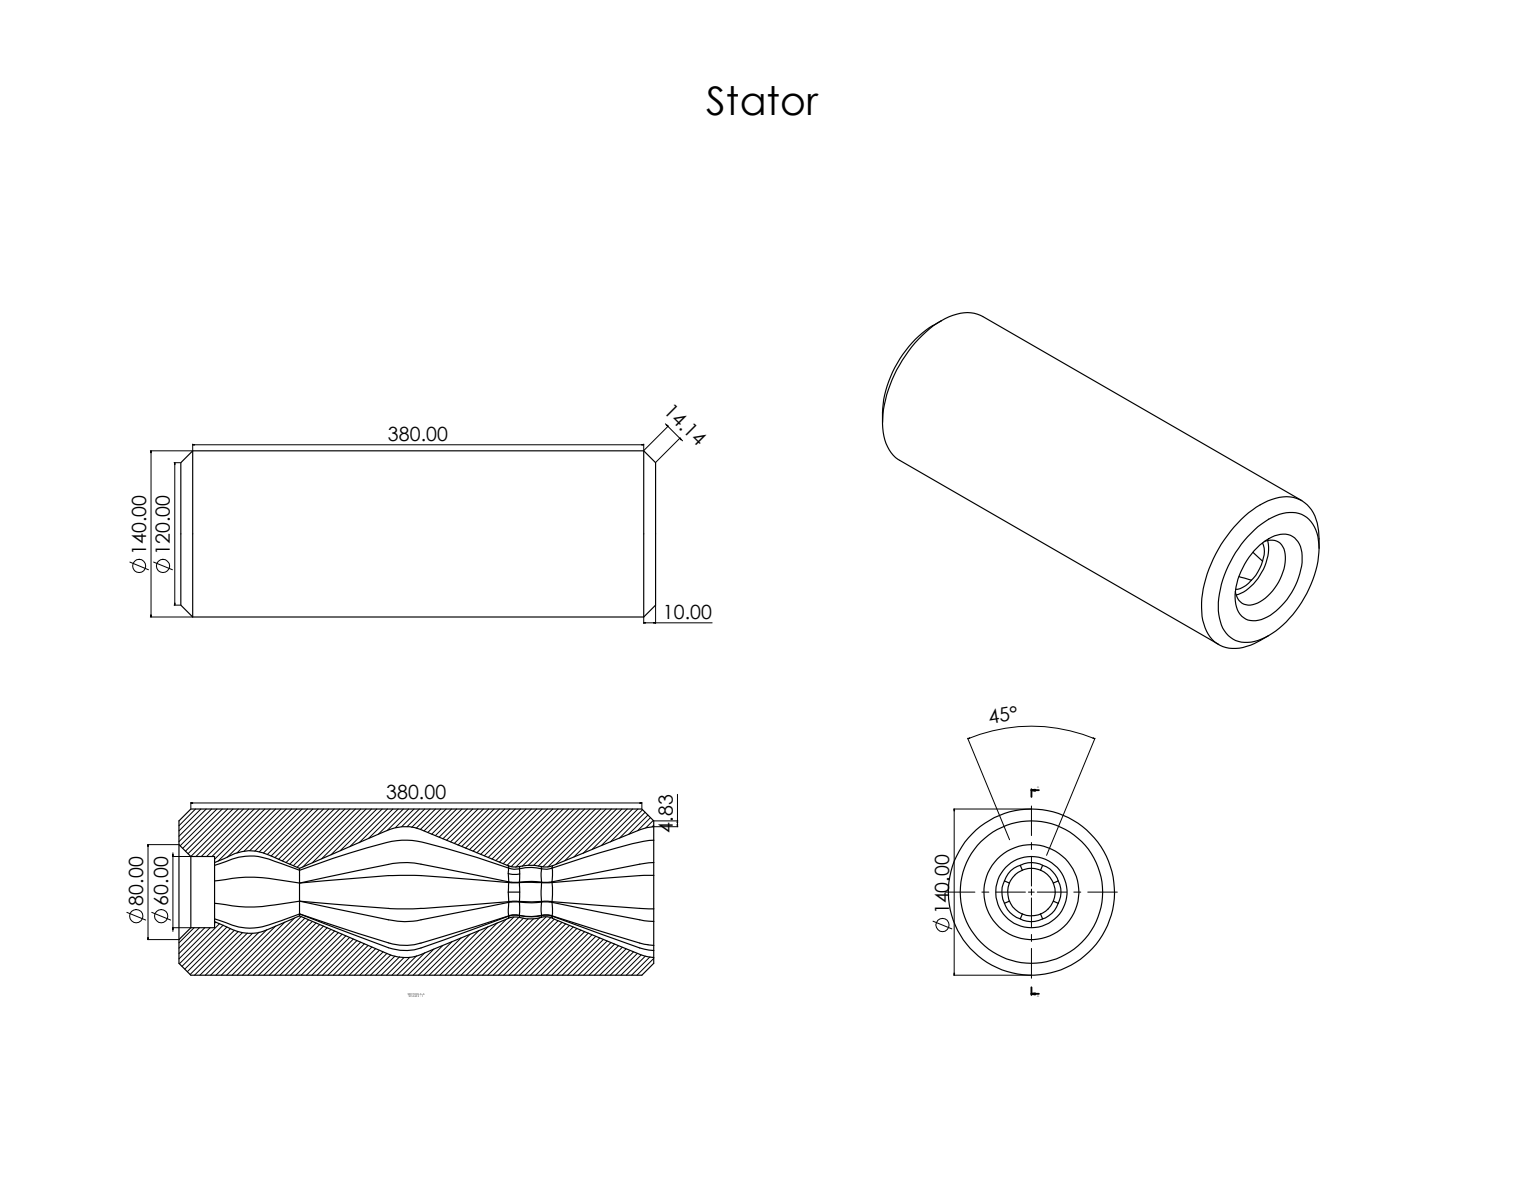
ISO-10303-21;
HEADER;
FILE_DESCRIPTION (('STEP AP214'),
    '1' );
FILE_NAME ('Stator.step',
    '2026-10-27T19:20:31',
    ( '' ),
    ( '' ),
    'SwSTEP 2.0',
    'SolidWorks 2025',
    '' );
FILE_SCHEMA (( 'AUTOMOTIVE_DESIGN' ));
ENDSEC;

DATA;
#1=CARTESIAN_POINT ( 'NONE',  ( 14.38125909742182529, -39.99999999999944578, -55.17850393971050238 ) ) ;
#2=CARTESIAN_POINT ( 'NONE',  ( -198.0356074513804572, -9.007331120208026888E-14, 15.37879056873070560 ) ) ;
#3=CARTESIAN_POINT ( 'NONE',  ( 4.995406935893293543, -15.24977328854832592, 0.000000000000000000 ) ) ;
#4=CARTESIAN_POINT ( 'NONE',  ( 163.1118516004056573, -9.006482792069636645, 9.006482792069567367 ) ) ;
#5=CARTESIAN_POINT ( 'NONE',  ( -259.2033419157646676, 9.517827891722584255, -0.000000000000000000 ) ) ;
#6=CARTESIAN_POINT ( 'NONE',  ( 0.2972598230770027716, -38.42060263243656237, -18.14793986248737667 ) ) ;
#10=CARTESIAN_POINT ( 'NONE',  ( 0.2972598230769957217, 1.502051041545559470E-13, -14.33493731733933352 ) ) ;
#11=CARTESIAN_POINT ( 'NONE',  ( 130.8568914410475372, 8.154165912415230659E-16, 5.949712681206690945 ) ) ;
#12=CARTESIAN_POINT ( 'NONE',  ( 184.8905102610680444, 13.49065550809807945, 13.49065550809809544 ) ) ;
#13=CARTESIAN_POINT ( 'NONE',  ( 146.6084372240433709, -3.800685668859084210, 52.76785682606516303 ) ) ;
#14=CARTESIAN_POINT ( 'NONE',  ( -190.0144721488653943, -13.91469502169275962, -47.57279682962041534 ) ) ;
#15=CARTESIAN_POINT ( 'NONE',  ( -198.0356074513804572, -39.15871834505905724, -17.40982414986491733 ) ) ;
#16=ORIENTED_EDGE ( 'NONE', *, *, #6629, .F. ) ;
#17=CARTESIAN_POINT ( 'NONE',  ( 146.6084372240433993, -24.48358557860353457, 24.48358557860296258 ) ) ;
#19=CARTESIAN_POINT ( 'NONE',  ( -192.9588430854689989, -14.46834944099973086, 0.000000000000000000 ) ) ;
#21=CARTESIAN_POINT ( 'NONE',  ( -100.7734535825088500, -44.31723036834885932, -12.25131212657538171 ) ) ;
#22=DIRECTION ( 'NONE',  ( 0.000000000000000000, 0.000000000000000000, 1.000000000000000000 ) ) ;
#23=CARTESIAN_POINT ( 'NONE',  ( -82.23866954411506924, 1.261533135296079022, 20.16514221458300682 ) ) ;
#26=CARTESIAN_POINT ( 'NONE',  ( 22.89172254855152389, -23.44749030158411074, 43.00256445985486664 ) ) ;
#27=CARTESIAN_POINT ( 'NONE',  ( -4.004886986946876171, 13.82996668233325721, 47.00296421444863171 ) ) ;
#29=ORIENTED_EDGE ( 'NONE', *, *, #2591, .T. ) ;
#30=CARTESIAN_POINT ( 'NONE',  ( -208.1127848780265026, 15.00245453012665564, 0.000000000000000000 ) ) ;
#33=CARTESIAN_POINT ( 'NONE',  ( -30.26275506840324070, 1.198031551616013601, 1.198031551616023371 ) ) ;
#35=CARTESIAN_POINT ( 'NONE',  ( 199.9999999999999432, -1.727494763561684666E-13, 20.00000000000010303 ) ) ;
#37=CARTESIAN_POINT ( 'NONE',  ( 170.0000000000000000, 1.183443619805854272E-13, -24.95097643317000546 ) ) ;
#41=CARTESIAN_POINT ( 'NONE',  ( 12.96694272553733107, -24.77464205076947223, -44.79869582454342236 ) ) ;
#42=CARTESIAN_POINT ( 'NONE',  ( -213.1075012329536946, -37.98287015391210275, -37.98287015391272092 ) ) ;
#43=EDGE_CURVE ( 'NONE', #19077, #10069, #15238, .T. ) ;
#44=CARTESIAN_POINT ( 'NONE',  ( -200.0000000000000000, 18.14877749763656212, 46.38610861938588670 ) ) ;
#45=CARTESIAN_POINT ( 'NONE',  ( 146.6084372240433709, -32.08495691632041513, -24.48358557860343154 ) ) ;
#46=CARTESIAN_POINT ( 'NONE',  ( -77.61444910505676376, 3.470426107442325048, 21.81614215779332966 ) ) ;
#47=CARTESIAN_POINT ( 'NONE',  ( -213.1075012329537230, -9.698598906450422774, -9.698598906450550672 ) ) ;
#48=CARTESIAN_POINT ( 'NONE',  ( -208.1127848780264742, -55.00245453012676222, -2.449293598294708485E-15 ) ) ;
#51=CIRCLE ( 'NONE', #14477, 30.00000000000003908 ) ;
#52=CARTESIAN_POINT ( 'NONE',  ( -192.9588430854689705, -54.46834944099975928, -2.449293598294708485E-15 ) ) ;
#53=AXIS2_PLACEMENT_3D ( 'NONE', #25264, #21266, #19008 ) ;
#54=CARTESIAN_POINT ( 'NONE',  ( -114.6180193230984372, 19.15387080987368762, 10.88873798880637622 ) ) ;
#55=CARTESIAN_POINT ( 'NONE',  ( -30.26275506840325136, 40.00000000000003553, -1.694272468445841007 ) ) ;
#56=EDGE_CURVE ( 'NONE', #12829, #11587, #7928, .T. ) ;
#57=CARTESIAN_POINT ( 'NONE',  ( -30.26275506840325136, 29.48230279907798135, -27.08623969584585112 ) ) ;
#58=EDGE_CURVE ( 'NONE', #18547, #5841, #11121, .T. ) ;
#59=CARTESIAN_POINT ( 'NONE',  ( -198.0356074513804572, 15.37879056873066830, -40.00000000000002132 ) ) ;
#61=VERTEX_POINT ( 'NONE', #13950 ) ;
#62=CARTESIAN_POINT ( 'NONE',  ( 146.6084372240433709, -34.62501878078303008, 40.00000000000002132 ) ) ;
#63=CARTESIAN_POINT ( 'NONE',  ( -86.86493150571118349, -7.943527260495776510, -19.77569912839190280 ) ) ;
#64=CARTESIAN_POINT ( 'NONE',  ( -259.2033419157646676, -40.00000000000017764, 30.48217210827725054 ) ) ;
#65=CIRCLE ( 'NONE', #6032, 14.99999999999999822 ) ;
#66=CARTESIAN_POINT ( 'NONE',  ( -259.2033419157646676, 21.55415060305860209, -21.55415060305812602 ) ) ;
#67=CARTESIAN_POINT ( 'NONE',  ( -280.0000000000000568, -20.00000000000006750, 40.00000000000002132 ) ) ;
#69=DIRECTION ( 'NONE',  ( 1.018913292508929218E-14, 1.000000000000000000, 8.144542348679703993E-15 ) ) ;
#72=CARTESIAN_POINT ( 'NONE',  ( 91.82158438592158234, 44.40256751092319121, 12.16597498400105515 ) ) ;
#73=CARTESIAN_POINT ( 'NONE',  ( -91.56559293963836410, -12.25131212657524138, 44.31723036834888774 ) ) ;
#75=CARTESIAN_POINT ( 'NONE',  ( 14.38125909742181108, 1.616281842095393922E-13, -15.17850393972633682 ) ) ;
#76=CARTESIAN_POINT ( 'NONE',  ( -198.0356074513804572, -67.44298959253333692, -10.87444709761016348 ) ) ;
#77=CARTESIAN_POINT ( 'NONE',  ( -87.08883615166502068, 12.58652615577663170, -17.39726528837345398 ) ) ;
#78=CARTESIAN_POINT ( 'NONE',  ( -213.1075012329537230, -18.58567234101155208, 37.98287015391234434 ) ) ;
#79=CARTESIAN_POINT ( 'NONE',  ( -100.7734535825088500, -12.25131212657462498, -44.31723036834905827 ) ) ;
#82=CARTESIAN_POINT ( 'NONE',  ( -208.1127848780265026, -2.327190355601776466E-13, 55.00245453012672670 ) ) ;
#85=CARTESIAN_POINT ( 'NONE',  ( 23.42154907652883011, 42.84253412640345715, -23.32998349128526883 ) ) ;
#86=CARTESIAN_POINT ( 'NONE',  ( 192.4448373802100889, 19.99999999996064304, 2.449293598294708485E-15 ) ) ;
#88=CARTESIAN_POINT ( 'NONE',  ( 192.4448373802100889, -14.14213562375876698, -14.14213562375885047 ) ) ;
#89=CARTESIAN_POINT ( 'NONE',  ( -62.79433447042063676, -25.93934121795946268, 9.335111860881914581 ) ) ;
#90=CARTESIAN_POINT ( 'NONE',  ( -280.0000000000000568, 19.99999999999995737, 40.00000000000002132 ) ) ;
#92=CARTESIAN_POINT ( 'NONE',  ( 12.01361959687201519, 24.84115733209565136, -44.88892880200794622 ) ) ;
#94=CARTESIAN_POINT ( 'NONE',  ( 20.91285618074969221, -23.84652503050088512, 43.54130497316993598 ) ) ;
#95=CARTESIAN_POINT ( 'NONE',  ( -2.164901439630326330, 23.84421257770968339, -43.53794903252429549 ) ) ;
#98=CARTESIAN_POINT ( 'NONE',  ( 151.7948205124836250, -3.202120068677277203E-13, 33.23291073765553705 ) ) ;
#99=CARTESIAN_POINT ( 'NONE',  ( 154.0339099654741801, -28.18615453125293513, 11.67508747798861002 ) ) ;
#100=CARTESIAN_POINT ( 'NONE',  ( -166.3490736466491740, -19.13702016930768579, 36.43932733844285821 ) ) ;
#101=CARTESIAN_POINT ( 'NONE',  ( 163.1118516004056573, 9.006482792069759213, -9.006482792069505194 ) ) ;
#103=CARTESIAN_POINT ( 'NONE',  ( -188.4265466358324090, 13.83489705870430519, -47.03621809928684172 ) ) ;
#104=CARTESIAN_POINT ( 'NONE',  ( 91.82158438592158234, -12.16597498397778843, 12.16597498397750954 ) ) ;
#105=CARTESIAN_POINT ( 'NONE',  ( -56.48582580120559271, -6.472252184284276844, 6.472252184284108978 ) ) ;
#106=CARTESIAN_POINT ( 'NONE',  ( 91.82158438592159655, -22.79471317813468545, -40.00000000000002132 ) ) ;
#107=CARTESIAN_POINT ( 'NONE',  ( -208.1127848780264742, 55.00245453010919050, -40.00000000000002132 ) ) ;
#108=CARTESIAN_POINT ( 'NONE',  ( -105.3755690713226585, -40.00000000000027711, 21.75974354311608749 ) ) ;
#109=CARTESIAN_POINT ( 'NONE',  ( 0.2972598230770011618, 10.13633138497462305, 66.70487387989858519 ) ) ;
#110=CARTESIAN_POINT ( 'NONE',  ( -96.94475454975007267, 20.58449551010169998, -9.001119816636389714 ) ) ;
#111=CARTESIAN_POINT ( 'NONE',  ( 130.8568914410475372, -4.207082182992785135, -4.207082182992884611 ) ) ;
#113=CARTESIAN_POINT ( 'NONE',  ( 0.2972598230769938343, 10.13633138497472252, 10.13633138497475628 ) ) ;
#114=CARTESIAN_POINT ( 'NONE',  ( -97.73806390046776471, 8.581719943994480460, 20.71810467721184423 ) ) ;
#116=ORIENTED_EDGE ( 'NONE', *, *, #25089, .T. ) ;
#119=B_SPLINE_CURVE_WITH_KNOTS ( 'NONE', 3,
 ( #4293, #2821, #10524, #19041, #16643, #4682, #8526, #24772, #8927, #6525, #20776, #20510, #2282, #14636, #22773, #8662, #10391, #6395, #24904, #14511, #14774, #22904, #12785, #20912, #2691, #18907, #15039, #23170, #13054, #25298, #21172, #4948, #17164, #2945 ),
 .UNSPECIFIED., .F., .F.,
 ( 4, 2, 2, 2, 2, 2, 2, 2, 2, 2, 2, 2, 2, 2, 2, 2, 4 ),
 ( -5.298243351204090312E-05, 0.01887868273877536807, 0.02834451532491907844, 0.03071097347145498174, 0.03307743161799089199, 0.03544388976452679529, 0.03781034791106269860, 0.04254326420413442889, 0.04727618049720615223, 0.04964263864374202084, 0.05200909679027788945, 0.05674201308334969607, 0.05910847122988561325, 0.06029170030315351980, 0.06147492937642144023, 0.06620784566949308725, 0.07567367825563638128 ),
 .UNSPECIFIED. ) ;
#120=CARTESIAN_POINT ( 'NONE',  ( 57.59792236341147031, -26.56190807104670171, -30.00663442387710234 ) ) ;
#121=CARTESIAN_POINT ( 'NONE',  ( 22.75882399337409367, -43.17886244245828919, -17.88527043150862283 ) ) ;
#123=CARTESIAN_POINT ( 'NONE',  ( 151.7948205124836250, -33.23291073765550863, 0.000000000000000000 ) ) ;
#124=CARTESIAN_POINT ( 'NONE',  ( -77.90255099906771363, -8.644468104261237684, -20.04994828523970440 ) ) ;
#125=ORIENTED_EDGE ( 'NONE', *, *, #9291, .T. ) ;
#128=CARTESIAN_POINT ( 'NONE',  ( -83.21262154144230294, -33.12752917117752105, 13.72187187063023472 ) ) ;
#129=CARTESIAN_POINT ( 'NONE',  ( -86.96347745069644475, 12.89780903124410472, -43.67073346367977393 ) ) ;
#130=CARTESIAN_POINT ( 'NONE',  ( -187.8779108535587739, -43.02987313851080131, -17.82355704116172745 ) ) ;
#131=CARTESIAN_POINT ( 'NONE',  ( 0.2972598230770030492, -40.00000000000007816, 14.33493731733919496 ) ) ;
#132=CARTESIAN_POINT ( 'NONE',  ( 4.995406935893288214, 15.24977328854832770, 0.000000000000000000 ) ) ;
#135=CARTESIAN_POINT ( 'NONE',  ( 200.0000000000000000, -39.99999999999991473, -20.00000000000024514 ) ) ;
#136=CARTESIAN_POINT ( 'NONE',  ( 192.4448373802100889, -3.692737725850373501E-14, 19.99999999996060751 ) ) ;
#137=CARTESIAN_POINT ( 'NONE',  ( -100.7734535825088500, 40.00000000000008527, -22.67402823373177512 ) ) ;
#138=CARTESIAN_POINT ( 'NONE',  ( -30.26275506840324425, -1.694272468446265334, -40.00000000000002132 ) ) ;
#139=CARTESIAN_POINT ( 'NONE',  ( 200.0000000000000000, -42.42640687119269671, -14.14213562373124766 ) ) ;
#140=CARTESIAN_POINT ( 'NONE',  ( 192.4448373802100889, 20.00000000003945644, 0.000000000000000000 ) ) ;
#142=CARTESIAN_POINT ( 'NONE',  ( -56.48582580120558561, -21.81201906317785699, 21.81201906317761896 ) ) ;
#145=CARTESIAN_POINT ( 'NONE',  ( 57.59792236341147031, 40.00000000000042633, -37.56421063658144277 ) ) ;
#146=CARTESIAN_POINT ( 'NONE',  ( 184.8905102610680444, -40.00000000000005684, 19.07866798485543569 ) ) ;
#147=CARTESIAN_POINT ( 'NONE',  ( -259.2033419157646676, 21.55415060305839958, -35.01439189186541512 ) ) ;
#148=CARTESIAN_POINT ( 'NONE',  ( -114.7173660547197045, 17.99555204289530863, 12.80183536318784299 ) ) ;
#149=CARTESIAN_POINT ( 'NONE',  ( -193.3669098795559194, -18.32287322058442314, -44.23532903077867218 ) ) ;
#150=CARTESIAN_POINT ( 'NONE',  ( 91.82158438592159655, -44.40256751092324095, -12.16597498400075139 ) ) ;
#151=VERTEX_POINT ( 'NONE', #13812 ) ;
#152=CARTESIAN_POINT ( 'NONE',  ( -192.9588430854690273, -18.05360324515400094, -38.51493924976961836 ) ) ;
#154=CARTESIAN_POINT ( 'NONE',  ( -30.26275506840324425, -1.694272468446265334, -40.00000000000002132 ) ) ;
#156=CARTESIAN_POINT ( 'NONE',  ( -259.2033419157646676, -6.730120644403663199, 6.730120644403451813 ) ) ;
#157=ORIENTED_EDGE ( 'NONE', *, *, #1849, .F. ) ;
#161=CARTESIAN_POINT ( 'NONE',  ( -7.769366557097702852, 22.72119856430158791, 41.90323276218021675 ) ) ;
#162=VERTEX_POINT ( 'NONE', #11961 ) ;
#164=CARTESIAN_POINT ( 'NONE',  ( -198.0356074513804572, 10.87444709759714989, 10.87444709759722450 ) ) ;
#166=CARTESIAN_POINT ( 'NONE',  ( -77.58504658647395047, -13.57342497464155429, -17.50304285594473086 ) ) ;
#167=CARTESIAN_POINT ( 'NONE',  ( 14.38125909742180752, 10.73282306404720465, 10.73282306404724018 ) ) ;
#168=CARTESIAN_POINT ( 'NONE',  ( 0.2972598230770030492, 5.716321584140269555E-13, -54.33493731733936016 ) ) ;
#173=CARTESIAN_POINT ( 'NONE',  ( -183.6284948306234810, 17.34366805700532410, 41.87131864452296526 ) ) ;
#174=CARTESIAN_POINT ( 'NONE',  ( 23.37583784646126617, -23.33923448557677105, -42.85659535397680031 ) ) ;
#175=CARTESIAN_POINT ( 'NONE',  ( 57.59792236341148453, -26.56190807104663421, -26.56190807104710672 ) ) ;
#176=CARTESIAN_POINT ( 'NONE',  ( -94.58366989427224780, 20.58370269626824012, -9.000605044545586964 ) ) ;
#177=CARTESIAN_POINT ( 'NONE',  ( -280.0000000000000000, -14.14213562373108779, 14.14213562373088529 ) ) ;
#179=CARTESIAN_POINT ( 'NONE',  ( 19.06497207195982924, -54.19242893257843008, -2.449293598294708485E-15 ) ) ;
#180=FACE_OUTER_BOUND ( 'NONE', #16206, .T. ) ;
#181=CARTESIAN_POINT ( 'NONE',  ( -208.1127848780264742, -55.00245453012676222, -2.449293598294708485E-15 ) ) ;
#182=CARTESIAN_POINT ( 'NONE',  ( -114.6133217222730991, 10.93740326486608083, 19.07173553325018389 ) ) ;
#183=CARTESIAN_POINT ( 'NONE',  ( -105.3755690713226585, 40.00000000000019185, -18.24025645688310249 ) ) ;
#184=CARTESIAN_POINT ( 'NONE',  ( -259.2033419157646676, -6.730120644403570829, -6.730120644403545960 ) ) ;
#185=CARTESIAN_POINT ( 'NONE',  ( -91.56559293963834989, -22.67402823373193499, -40.00000000000002132 ) ) ;
#189=CARTESIAN_POINT ( 'NONE',  ( -280.0000000000000568, 19.99999999999995737, 40.00000000000002132 ) ) ;
#191=CARTESIAN_POINT ( 'NONE',  ( -56.48582580120559982, 50.09629031063956717, 6.472252184284792875 ) ) ;
#192=CARTESIAN_POINT ( 'NONE',  ( -110.0685463886591293, -19.46857821975389058, -5.325649136242457615 ) ) ;
#198=ADVANCED_FACE ( 'NONE', ( #23801 ), #14342, .T. ) ;
#199=ADVANCED_FACE ( 'NONE', ( #14088 ), #12427, .T. ) ;
#201=CARTESIAN_POINT ( 'NONE',  ( 136.1360204305621551, 31.79587985999232558, 24.77266263493161702 ) ) ;
#202=CARTESIAN_POINT ( 'NONE',  ( 184.8905102610680444, -41.77492675556007384, 14.79361573936348684 ) ) ;
#203=DIRECTION ( 'NONE',  ( -0.2259624730582342200, 0.000000000000000000, -0.9741360073261878805 ) ) ;
#204=CARTESIAN_POINT ( 'NONE',  ( 19.06497207195979726, 40.00000000000017053, -14.19242893257798599 ) ) ;
#205=CARTESIAN_POINT ( 'NONE',  ( 146.6084372240433993, -3.800685668858596156, -3.800685668858692967 ) ) ;
#206=CARTESIAN_POINT ( 'NONE',  ( 163.1118516004056573, -19.27778845538787422, 19.27778845538743724 ) ) ;
#207=CARTESIAN_POINT ( 'NONE',  ( -198.0356074513804572, -17.40982414986482141, 39.15871834505909987 ) ) ;
#208=CARTESIAN_POINT ( 'NONE',  ( 163.1118516004056573, -9.006482792073960297, -47.56205970284963769 ) ) ;
#211=CARTESIAN_POINT ( 'NONE',  ( -100.7734535825088500, 39.99999999999994316, 17.32597176626825686 ) ) ;
#213=CARTESIAN_POINT ( 'NONE',  ( 19.94008347562116512, 43.76810615267693549, -24.01421467034480273 ) ) ;
#214=CARTESIAN_POINT ( 'NONE',  ( -135.8532207217289738, -9.153146818113595984, -40.00000000000002132 ) ) ;
#215=CARTESIAN_POINT ( 'NONE',  ( 8.517493242715996615, -24.85395068094629067, -44.90626920808422540 ) ) ;
#216=CARTESIAN_POINT ( 'NONE',  ( -4.082462733454099713, -46.97557262069199879, 13.82507958736570153 ) ) ;
#217=CARTESIAN_POINT ( 'NONE',  ( 130.8568914410475088, 5.949712681206712261, 40.00000000000002132 ) ) ;
#219=CARTESIAN_POINT ( 'NONE',  ( 7.307793593482434957, 24.85783611765758039, -44.91153572052478893 ) ) ;
#220=CARTESIAN_POINT ( 'NONE',  ( -259.2033419157646676, -35.01439189186554302, 21.55415060305832498 ) ) ;
#221=CARTESIAN_POINT ( 'NONE',  ( -16.87994666136603072, -20.93785811888612258, 39.19724034055838757 ) ) ;
#223=CARTESIAN_POINT ( 'NONE',  ( -3.696864809820620934, 13.84627154338459931, -47.11278487914880486 ) ) ;
#225=EDGE_CURVE ( 'NONE', #2033, #22654, #7079, .T. ) ;
#226=CARTESIAN_POINT ( 'NONE',  ( -56.48582580120559271, -1.062504017861011783E-13, 9.153146818113587102 ) ) ;
#227=CARTESIAN_POINT ( 'NONE',  ( 167.0466155511621480, -23.44215416552593467, 9.710058186601612462 ) ) ;
#228=CARTESIAN_POINT ( 'NONE',  ( -188.6890294954723117, -13.84869711777589885, 47.12920239600079242 ) ) ;
#229=CARTESIAN_POINT ( 'NONE',  ( 14.38125909742181463, 10.73282306403652875, -67.30136555895941797 ) ) ;
#230=CARTESIAN_POINT ( 'NONE',  ( -100.7734535825088500, 22.67402823373189591, -0.000000000000000000 ) ) ;
#233=CARTESIAN_POINT ( 'NONE',  ( -194.7884774423580154, 18.40784251727735565, -44.44046305924767637 ) ) ;
#234=CARTESIAN_POINT ( 'NONE',  ( -135.8532207217289738, -6.472252184284280396, 6.472252184284099208 ) ) ;
#235=CARTESIAN_POINT ( 'NONE',  ( -135.8532207217289738, 50.09629031063956006, 6.472252184284782217 ) ) ;
#236=CARTESIAN_POINT ( 'NONE',  ( -100.7734535825088500, -17.32597176626813251, 40.00000000000002132 ) ) ;
#237=CARTESIAN_POINT ( 'NONE',  ( 146.6084372240433993, 5.374981219216999229, 2.449293598294708485E-15 ) ) ;
#238=CARTESIAN_POINT ( 'NONE',  ( 4.995406935893290878, 1.606505379428369110E-13, -15.24977328854832592 ) ) ;
#239=CARTESIAN_POINT ( 'NONE',  ( 136.1360204305621551, -24.77266263493126885, 31.79587985999256006 ) ) ;
#240=CARTESIAN_POINT ( 'NONE',  ( -94.58414068580489698, 20.73981583682122576, -8.590713000717968839 ) ) ;
#241=CARTESIAN_POINT ( 'NONE',  ( 184.8905102610680444, 43.07788698682591644, -13.49065550809769221 ) ) ;
#242=CARTESIAN_POINT ( 'NONE',  ( -213.1075012329537230, -9.698598906450557777, 9.698598906450415669 ) ) ;
#245=CARTESIAN_POINT ( 'NONE',  ( 151.7948205124836534, -51.78348778862535795, 4.785054706298367044 ) ) ;
#248=CARTESIAN_POINT ( 'NONE',  ( -200.0000000000001421, -14.17215463606902404, -49.28189405767602693 ) ) ;
#249=CARTESIAN_POINT ( 'NONE',  ( -91.56559293963834989, 6.234561990864368500E-14, -22.67402823373191723 ) ) ;
#250=CARTESIAN_POINT ( 'NONE',  ( 91.82158438592159655, 12.16597498400028776, 44.40256751092339016 ) ) ;
#251=CARTESIAN_POINT ( 'NONE',  ( -3.379936260374155399, -43.32059152999958940, -17.94397654175126888 ) ) ;
#252=EDGE_LOOP ( 'NONE', ( #14876, #22901, #13781, #8671 ) ) ;
#259=CARTESIAN_POINT ( 'NONE',  ( 184.8905102610680444, -14.79361573936379415, -14.79361573936387941 ) ) ;
#260=CARTESIAN_POINT ( 'NONE',  ( -188.3066136396997479, -46.99300418776440580, -13.82848859481202553 ) ) ;
#261=CARTESIAN_POINT ( 'NONE',  ( -208.1127848780265026, -2.327190355601776466E-13, 55.00245453012672670 ) ) ;
#262=CARTESIAN_POINT ( 'NONE',  ( 163.1118516004056573, 12.73709011382477918, 40.00000000000002132 ) ) ;
#266=CARTESIAN_POINT ( 'NONE',  ( -192.9588430854690273, -40.00000000000024158, 54.46834944101708231 ) ) ;
#267=CARTESIAN_POINT ( 'NONE',  ( 170.2234770963711128, 40.00000000000000000, 15.44714144992830462 ) ) ;
#268=CARTESIAN_POINT ( 'NONE',  ( -208.1127848780265026, -9.061048840815752106E-14, 15.00245453012669472 ) ) ;
#270=CARTESIAN_POINT ( 'NONE',  ( 14.38125909742182884, -55.17850393972636169, -2.449293598294708485E-15 ) ) ;
#271=CARTESIAN_POINT ( 'NONE',  ( -238.4067589809705794, -0.6820004458488042598, 57.25054294077229855 ) ) ;
#272=CARTESIAN_POINT ( 'NONE',  ( -280.0000000000000000, -2.609240458947769655E-13, 20.00000000000001421 ) ) ;
#273=CARTESIAN_POINT ( 'NONE',  ( 1.564252679174732208, -48.56509332159251358, 14.06374044400967271 ) ) ;
#274=CARTESIAN_POINT ( 'NONE',  ( 136.1360204305621266, 7.947488714877270288E-14, -4.966164525587064560 ) ) ;
#275=CARTESIAN_POINT ( 'NONE',  ( -100.7734535825088500, -40.00000000000009948, 17.32597176626796909 ) ) ;
#276=CARTESIAN_POINT ( 'NONE',  ( -259.2033419157646676, -6.730120644403570829, -6.730120644403545960 ) ) ;
#278=CARTESIAN_POINT ( 'NONE',  ( -188.2995950289364941, -46.99046209955426434, -13.82811170417247126 ) ) ;
#279=CARTESIAN_POINT ( 'NONE',  ( -97.72675010090328840, -8.987772175319422630, -20.56394680065913505 ) ) ;
#280=CARTESIAN_POINT ( 'NONE',  ( 200.0000000000000000, -42.42640687119269671, -14.14213562373124766 ) ) ;
#282=CARTESIAN_POINT ( 'NONE',  ( 151.7948205124836534, -23.49921654115981084, -33.06932595376387951 ) ) ;
#284=CARTESIAN_POINT ( 'NONE',  ( -91.56559293963834989, -17.32597176626812185, -40.00000000000002132 ) ) ;
#285=CARTESIAN_POINT ( 'NONE',  ( -114.4364955367336449, 20.04994829326807348, -8.644468109231272734 ) ) ;
#286=CARTESIAN_POINT ( 'NONE',  ( -259.2033419157646676, -9.517827891722680178, 0.000000000000000000 ) ) ;
#290=CARTESIAN_POINT ( 'NONE',  ( -97.73860346102746632, 8.987542150733535351, -20.56359266934956764 ) ) ;
#292=CARTESIAN_POINT ( 'NONE',  ( 23.36462152322931374, 23.34178792078241216, 42.86003749000698804 ) ) ;
#293=ORIENTED_EDGE ( 'NONE', *, *, #21671, .T. ) ;
#294=AXIS2_PLACEMENT_3D ( 'NONE', #8252, #14768, #20771 ) ;
#297=CARTESIAN_POINT ( 'NONE',  ( -91.56559293963834989, -16.03295912088706388, -16.03295912088710651 ) ) ;
#301=CARTESIAN_POINT ( 'NONE',  ( 35.93702930694564657, 42.26928858314015258, -12.87541766278293665 ) ) ;
#302=CARTESIAN_POINT ( 'NONE',  ( -280.0000000000000568, 14.14213562373097943, -42.42640687119285303 ) ) ;
#305=CARTESIAN_POINT ( 'NONE',  ( -94.58414068588150769, -8.590713000723692261, -20.73981583676798124 ) ) ;
#306=EDGE_CURVE ( 'NONE', #14634, #3360, #8864, .T. ) ;
#307=CARTESIAN_POINT ( 'NONE',  ( -280.0000000000000568, 40.00000000000017764, -19.99999999999959144 ) ) ;
#308=CARTESIAN_POINT ( 'NONE',  ( 4.995406935893283773, 40.00000000000017764, -15.24977328854790848 ) ) ;
#312=CARTESIAN_POINT ( 'NONE',  ( -188.2652133075334291, 23.44262061655307505, 42.99509596150254964 ) ) ;
#313=CARTESIAN_POINT ( 'NONE',  ( 163.1118516004056573, -9.006482792074626431, 47.56205970284951690 ) ) ;
#315=CARTESIAN_POINT ( 'NONE',  ( -199.9999999999998579, 24.82633483071252201, 44.86878812508700776 ) ) ;
#316=CARTESIAN_POINT ( 'NONE',  ( 19.06497207195980792, 18.24870850772737185, 38.31983398719634692 ) ) ;
#318=CARTESIAN_POINT ( 'NONE',  ( -86.96347745069643054, 15.38646221621821297, -41.18208027870583265 ) ) ;
#320=CARTESIAN_POINT ( 'NONE',  ( 57.59792236341147031, 2.435789363418170872, 40.00000000000002132 ) ) ;
#321=CARTESIAN_POINT ( 'NONE',  ( 151.7948205124836250, 23.49921654116361225, -23.49921654116333514 ) ) ;
#323=CARTESIAN_POINT ( 'NONE',  ( 163.1118516004056573, 27.26290988616876021, 40.00000000000002132 ) ) ;
#325=CARTESIAN_POINT ( 'NONE',  ( -86.96347745069645896, 39.99999999999977973, 21.75974354311691883 ) ) ;
#326=CARTESIAN_POINT ( 'NONE',  ( 19.06497207195980792, 10.03556273973433299, 10.03556273973436319 ) ) ;
#327=CARTESIAN_POINT ( 'NONE',  ( 146.5090579137181237, -12.40347562390472191, 29.94463907179402185 ) ) ;
#328=EDGE_LOOP ( 'NONE', ( #16904, #25782, #2991, #623 ) ) ;
#329=ORIENTED_EDGE ( 'NONE', *, *, #13669, .T. ) ;
#330=CARTESIAN_POINT ( 'NONE',  ( 136.1360204305621551, -35.03383547441293899, 40.00000000000002132 ) ) ;
#332=CARTESIAN_POINT ( 'NONE',  ( -105.3755690713226585, 41.18208027870575449, 15.38646221621837107 ) ) ;
#333=CARTESIAN_POINT ( 'NONE',  ( 83.01683444495014896, 24.01517293246239859, -9.947410331382577908 ) ) ;
#334=B_SPLINE_CURVE_WITH_KNOTS ( 'NONE', 3,
 ( #4512, #20114, #6492, #14604, #8355, #6621, #19974, #12614, #1625, #16476, #1755, #1891, #10626, #24601 ),
 .UNSPECIFIED., .F., .F.,
 ( 4, 2, 2, 2, 2, 2, 4 ),
 ( 0.0003132551814620533593, 0.004485169056169878432, 0.006571125993523792459, 0.008657082930877708221, 0.01282899680558553628, 0.01491495374293945290, 0.01700091068029336780 ),
 .UNSPECIFIED. ) ;
#335=CARTESIAN_POINT ( 'NONE',  ( -175.9234121933940003, -12.95566993500714581, -42.70618342224702957 ) ) ;
#336=CARTESIAN_POINT ( 'NONE',  ( -175.9235632145383477, 21.03681926525754164, 39.35891845724489002 ) ) ;
#339=CARTESIAN_POINT ( 'NONE',  ( -192.9588430854690273, 10.23066800229588758, -66.79921049721882298 ) ) ;
#340=CARTESIAN_POINT ( 'NONE',  ( 57.59792236341147031, -26.56190807104712448, 30.00663442387673285 ) ) ;
#342=CARTESIAN_POINT ( 'NONE',  ( -213.1075012329537230, 40.00000000000055422, -53.71589010953623244 ) ) ;
#343=CARTESIAN_POINT ( 'NONE',  ( 130.8568914410475088, -32.49135343045495006, 24.07718906446878648 ) ) ;
#344=CARTESIAN_POINT ( 'NONE',  ( 130.8568914410475372, 34.05028731879791337, 0.000000000000000000 ) ) ;
#345=CARTESIAN_POINT ( 'NONE',  ( -77.90255099907052738, 8.064892378688679031, 20.29001641119211641 ) ) ;
#346=CARTESIAN_POINT ( 'NONE',  ( -198.0356074513804572, -67.44298959250878056, 10.87444709758448447 ) ) ;
#347=CARTESIAN_POINT ( 'NONE',  ( -198.0356074513804572, -15.37879056873074290, 0.000000000000000000 ) ) ;
#348=EDGE_CURVE ( 'NONE', #21839, #25714, #6340, .T. ) ;
#350=CARTESIAN_POINT ( 'NONE',  ( -259.2033419157646676, 39.99999999999987210, 30.48217210827754542 ) ) ;
#352=CARTESIAN_POINT ( 'NONE',  ( 27.00968939604439711, 41.97305875715863976, -17.38581019152421447 ) ) ;
#353=CARTESIAN_POINT ( 'NONE',  ( 146.6084372240433709, 5.374981219217002781, -40.00000000000002132 ) ) ;
#354=CARTESIAN_POINT ( 'NONE',  ( -162.0762913951020892, 1.198031840385716418, 1.198031840385750169 ) ) ;
#355=CARTESIAN_POINT ( 'NONE',  ( -100.7734535825088358, -22.67402823373193499, 0.000000000000000000 ) ) ;
#356=ADVANCED_FACE ( 'NONE', ( #16743 ), #4299, .T. ) ;
#357=CARTESIAN_POINT ( 'NONE',  ( -77.90255099906768521, -20.04994828523980743, 8.644468104261049390 ) ) ;
#358=CARTESIAN_POINT ( 'NONE',  ( -30.26275506840324070, 41.69427246844628598, 2.449293598294708485E-15 ) ) ;
#359=ADVANCED_FACE ( 'NONE', ( #19844 ), #15148, .T. ) ;
#360=ORIENTED_EDGE ( 'NONE', *, *, #13600, .F. ) ;
#362=CARTESIAN_POINT ( 'NONE',  ( -77.80451652700847376, 19.69389078277757577, 9.718324738897942794 ) ) ;
#363=CARTESIAN_POINT ( 'NONE',  ( -4.660840668353244176, -23.32816686155642572, 42.82207049670917343 ) ) ;
#364=CARTESIAN_POINT ( 'NONE',  ( -3.786831587087438500, 23.50387725152274143, -43.07879808621805040 ) ) ;
#366=CARTESIAN_POINT ( 'NONE',  ( -188.2995950289364089, 46.99046209955525200, -13.82811170417133617 ) ) ;
#367=CARTESIAN_POINT ( 'NONE',  ( -53.37686176745582145, -27.95807077219591008, -13.65870576116551405 ) ) ;
#368=CIRCLE ( 'NONE', #25453, 69.99999999999994316 ) ;
#369=CARTESIAN_POINT ( 'NONE',  ( -197.6433718613984638, -18.53520099271227650, 44.74793361791267188 ) ) ;
#370=CARTESIAN_POINT ( 'NONE',  ( 0.2972598230769990524, -18.14793986248671231, -38.42060263243687501 ) ) ;
#371=CARTESIAN_POINT ( 'NONE',  ( -105.3755690713226869, 21.75974354311648540, -0.000000000000000000 ) ) ;
#372=CARTESIAN_POINT ( 'NONE',  ( -188.3509229510973171, 17.87648076835260724, -43.15764231845668775 ) ) ;
#373=CARTESIAN_POINT ( 'NONE',  ( -198.0356074513804572, 10.87444709759730088, -10.87444709759707173 ) ) ;
#374=CARTESIAN_POINT ( 'NONE',  ( 163.1118516004056573, -19.27778845538787422, 19.27778845538743724 ) ) ;
#375=CARTESIAN_POINT ( 'NONE',  ( 146.6084372240433993, -5.374981219216945938, -2.449293598294708485E-15 ) ) ;
#376=CARTESIAN_POINT ( 'NONE',  ( 136.1360204305621266, 4.966164525587089429, 2.449293598294708485E-15 ) ) ;
#377=CARTESIAN_POINT ( 'NONE',  ( -91.56559293963834989, -2.543181659092656077E-13, 22.67402823373191723 ) ) ;
#378=CARTESIAN_POINT ( 'NONE',  ( 4.995406935893290878, 39.06748935135185263, 39.06748935135198764 ) ) ;
#379=EDGE_CURVE ( 'NONE', #9180, #11184, #24378, .T. ) ;
#380=CARTESIAN_POINT ( 'NONE',  ( -88.38011430142853442, 20.03522014474807733, -8.298859908977320288 ) ) ;
#381=CARTESIAN_POINT ( 'NONE',  ( -30.26275506840322649, -29.48230279907769358, -29.48230279907820162 ) ) ;
#382=CARTESIAN_POINT ( 'NONE',  ( 151.7948205124836250, 23.49921654116361225, -23.49921654116333514 ) ) ;
#384=CARTESIAN_POINT ( 'NONE',  ( 136.1360204305621551, -53.05693388239313890, 3.511608612530593199 ) ) ;
#385=CARTESIAN_POINT ( 'NONE',  ( -102.4294859495257981, 8.407280617713011495, 20.29697089052800862 ) ) ;
#386=CARTESIAN_POINT ( 'NONE',  ( 19.06497207195981858, -10.03556273973469715, 66.60410523465813526 ) ) ;
#387=CARTESIAN_POINT ( 'NONE',  ( 6.984886629841083661, -44.84679502273381502, -24.81009932001601825 ) ) ;
#388=EDGE_CURVE ( 'NONE', #22654, #12121, #26200, .T. ) ;
#391=CARTESIAN_POINT ( 'NONE',  ( 0.4226707250630000745, -48.37218667320258447, -14.03458789212649016 ) ) ;
#395=B_SPLINE_CURVE_WITH_KNOTS ( 'NONE', 3,
 ( #13531, #13284, #23906, #9540, #17397, #9292 ),
 .UNSPECIFIED., .F., .F.,
 ( 4, 2, 4 ),
 ( 0.0003134720024621259586, 0.004478974658733396105, 0.008644477315004665818 ),
 .UNSPECIFIED. ) ;
#397=CARTESIAN_POINT ( 'NONE',  ( -114.4364955367323091, -20.29001642039124675, -8.064892380834873364 ) ) ;
#399=CARTESIAN_POINT ( 'NONE',  ( -189.1288815661592650, -43.24061771116329567, -23.62384257861769754 ) ) ;
#400=CARTESIAN_POINT ( 'NONE',  ( -192.9588430854689989, -2.280704836619014309E-13, 54.46834944099972375 ) ) ;
#401=B_SPLINE_CURVE_WITH_KNOTS ( 'NONE', 3,
 ( #4947, #19166, #10663, #18773, #12921, #12650, #4553, #6791, #22903, #10796, #25038, #22772 ),
 .UNSPECIFIED., .F., .F.,
 ( 4, 2, 2, 2, 2, 4 ),
 ( 5.605063087764202676E-17, 0.005971652981263785541, 0.008957479471895606754, 0.01045039271721155509, 0.01119684933986949023, 0.01194330596252742363 ),
 .UNSPECIFIED. ) ;
#402=CARTESIAN_POINT ( 'NONE',  ( -238.4067589809705794, 40.96449427998256709, 2.449293598294708485E-15 ) ) ;
#405=CARTESIAN_POINT ( 'NONE',  ( -105.3755690713226585, -40.00000000000010658, 18.24025645688337249 ) ) ;
#406=CARTESIAN_POINT ( 'NONE',  ( 19.06497207195979726, 39.99999999999997158, 14.19242893257854554 ) ) ;
#409=CARTESIAN_POINT ( 'NONE',  ( -100.7734535825088500, -17.32597176626812185, -40.00000000000002132 ) ) ;
#410=CARTESIAN_POINT ( 'NONE',  ( 184.8905102610680444, -13.49065550809810965, 13.49065550809799596 ) ) ;
#411=CARTESIAN_POINT ( 'NONE',  ( 19.06497207195981147, 1.521599808664285085E-13, -14.19242893257840521 ) ) ;
#412=CARTESIAN_POINT ( 'NONE',  ( -114.4364955367327070, -8.644468109209471507, 20.04994829327649342 ) ) ;
#413=CARTESIAN_POINT ( 'NONE',  ( 170.2234770963711128, 40.00000000000021316, -15.44714144992773797 ) ) ;
#414=CARTESIAN_POINT ( 'NONE',  ( -162.0762913951020892, 39.99999999999985079, 41.69427287692695216 ) ) ;
#416=CARTESIAN_POINT ( 'NONE',  ( -114.7826396787322665, 2.171560191748074081E-13, -22.13135001986799111 ) ) ;
#417=CARTESIAN_POINT ( 'NONE',  ( -93.02511667906946968, -8.946512270084925333, -20.50052124204830761 ) ) ;
#418=CARTESIAN_POINT ( 'NONE',  ( 146.6084372240433709, -32.08495691632041513, -24.48358557860343154 ) ) ;
#422=CARTESIAN_POINT ( 'NONE',  ( -162.0762913951020607, -41.69427287682838568, -2.449293598294708485E-15 ) ) ;
#424=CARTESIAN_POINT ( 'NONE',  ( -138.9613198122422375, -27.95779845120239671, 13.65853124629192017 ) ) ;
#425=FACE_OUTER_BOUND ( 'NONE', #10801, .T. ) ;
#427=ORIENTED_EDGE ( 'NONE', *, *, #15865, .F. ) ;
#429=SPHERICAL_SURFACE ( 'NONE', #21501, 15.00000000000000000 ) ;
#430=CARTESIAN_POINT ( 'NONE',  ( -97.73806390048314086, 8.581719943918708182, -20.71810467719452120 ) ) ;
#431=CARTESIAN_POINT ( 'NONE',  ( 19.94008347562546390, 13.96811062196290010, 47.92933869853475670 ) ) ;
#434=CARTESIAN_POINT ( 'NONE',  ( -135.8532207217289738, -6.472252184284287502, 50.09629031063965243 ) ) ;
#436=CARTESIAN_POINT ( 'NONE',  ( -110.0947178155009141, 2.529241932053376551, 20.04333087343293940 ) ) ;
#437=CARTESIAN_POINT ( 'NONE',  ( -109.1264249741459338, -33.12752917269534692, -13.72187187123280161 ) ) ;
#438=CARTESIAN_POINT ( 'NONE',  ( 91.82158438592158234, -12.16597498397761967, -12.16597498397768007 ) ) ;
#443=CARTESIAN_POINT ( 'NONE',  ( 200.0000000000000000, 40.00000000000026290, -19.99999999999950617 ) ) ;
#444=CARTESIAN_POINT ( 'NONE',  ( 163.1118516004056573, -2.556006622855449647E-13, 27.26290988616872824 ) ) ;
#448=CARTESIAN_POINT ( 'NONE',  ( -188.3610564113327825, 23.46269903113395827, 43.02325945309083011 ) ) ;
#449=CARTESIAN_POINT ( 'NONE',  ( -105.3755690713226585, -12.89780903124444578, 43.67073346367968156 ) ) ;
#450=( BOUNDED_CURVE ( )  B_SPLINE_CURVE ( 3, ( #3461, #19679, #15943, #11828 ),
 .UNSPECIFIED., .F., .F. ) 
 B_SPLINE_CURVE_WITH_KNOTS ( ( 4, 4 ),
 ( 0.004183487405659383311, 0.01388163287021833628 ),
 .UNSPECIFIED. ) 
 CURVE ( )  GEOMETRIC_REPRESENTATION_ITEM ( )  RATIONAL_B_SPLINE_CURVE ( ( 0.6809743333591558034, 0.7608653435686151267, 0.8672072324488965256, 1.000000000000000000 ) ) 
 REPRESENTATION_ITEM ( '' )  );
#452=CARTESIAN_POINT ( 'NONE',  ( 14.38125909742182529, -39.01709431150933938, 39.01709431150894147 ) ) ;
#454=CARTESIAN_POINT ( 'NONE',  ( 192.4448373802101173, 14.14213562375922884, -42.42640687116488607 ) ) ;
#456=CARTESIAN_POINT ( 'NONE',  ( 163.1118516004056573, 27.26290988616875310, 0.000000000000000000 ) ) ;
#457=CARTESIAN_POINT ( 'NONE',  ( -192.9588430854690273, 66.79921049724377724, -10.23066800231904239 ) ) ;
#458=CARTESIAN_POINT ( 'NONE',  ( -100.7734535825088500, 22.67402823373189591, -0.000000000000000000 ) ) ;
#460=CARTESIAN_POINT ( 'NONE',  ( -91.56559293963834989, -39.99999999999985789, -17.32597176626853042 ) ) ;
#463=ORIENTED_EDGE ( 'NONE', *, *, #25346, .F. ) ;
#466=ORIENTED_EDGE ( 'NONE', *, *, #16953, .T. ) ;
#467=CARTESIAN_POINT ( 'NONE',  ( -86.96347745069644475, -21.75974354311651737, 0.000000000000000000 ) ) ;
#469=CARTESIAN_POINT ( 'NONE',  ( 0.2972598230769907257, 66.70487387989869887, -10.13633138497392494 ) ) ;
#470=CARTESIAN_POINT ( 'NONE',  ( -114.4364955367305896, -20.29001642037712827, 8.064892380866057309 ) ) ;
#474=CARTESIAN_POINT ( 'NONE',  ( 170.0000000000000000, -6.285860131565354614, 24.25569233607177111 ) ) ;
#475=CIRCLE ( 'NONE', #21717, 14.99999999999999822 ) ;
#476=CARTESIAN_POINT ( 'NONE',  ( 136.1360204305621551, -53.05693388239309627, -3.511608612531332163 ) ) ;
#477=CARTESIAN_POINT ( 'NONE',  ( -56.48582580120559271, 6.472252184284121412, 6.472252184284244869 ) ) ;
#479=CARTESIAN_POINT ( 'NONE',  ( 151.7948205124836534, 40.00000000000012079, -6.767089262348609857 ) ) ;
#480=CARTESIAN_POINT ( 'NONE',  ( 184.8905102610680444, -13.49065550809840630, 43.07788698682565354 ) ) ;
#481=CARTESIAN_POINT ( 'NONE',  ( -83.21262154144251610, -13.72187187061536484, 33.12752917118401541 ) ) ;
#482=CARTESIAN_POINT ( 'NONE',  ( -30.26275506840324070, 1.198031551616013601, 1.198031551616023371 ) ) ;
#483=CARTESIAN_POINT ( 'NONE',  ( -213.1075012329537230, -9.698598906438496314, 66.26714140136188291 ) ) ;
#486=CARTESIAN_POINT ( 'NONE',  ( 184.8905102610680444, -40.00000000000005684, 19.07866798485543569 ) ) ;
#488=CARTESIAN_POINT ( 'NONE',  ( 23.38399212876566580, 42.85408588822684806, -23.33762193384624695 ) ) ;
#489=CARTESIAN_POINT ( 'NONE',  ( -91.56559293963834989, 17.32597176626809699, -40.00000000000002132 ) ) ;
#490=CARTESIAN_POINT ( 'NONE',  ( -280.0000000000000568, -42.42640687119295251, 14.14213562373088351 ) ) ;
#491=CARTESIAN_POINT ( 'NONE',  ( -56.48582580120559982, 30.84685318188643421, 40.00000000000002132 ) ) ;
#492=CARTESIAN_POINT ( 'NONE',  ( -5.787027468455986146, -42.67020100828555940, 17.67457596681778043 ) ) ;
#493=AXIS2_PLACEMENT_3D ( 'NONE', #19176, #9563, #1212 ) ;
#494=CARTESIAN_POINT ( 'NONE',  ( -238.4067589809705794, 40.96449427990177128, 40.00000000000002132 ) ) ;
#496=CARTESIAN_POINT ( 'NONE',  ( -198.0012279766650067, -49.19397028317939657, -14.15883993157146215 ) ) ;
#498=CARTESIAN_POINT ( 'NONE',  ( -77.55640685876515761, 16.67541351910017866, 14.62304181636398148 ) ) ;
#499=CARTESIAN_POINT ( 'NONE',  ( -4.076660308449182146, -23.44206949513782945, 42.99426297939349695 ) ) ;
#500=CARTESIAN_POINT ( 'NONE',  ( -4.660840668352557614, 13.78427145221092154, -46.77528141313259624 ) ) ;
#502=CARTESIAN_POINT ( 'NONE',  ( -238.4067589809705794, 28.96627169325285678, 27.60227080167094726 ) ) ;
#503=CARTESIAN_POINT ( 'NONE',  ( -82.30220482034343377, -18.74474319042090542, 7.441767004327110691 ) ) ;
#505=CARTESIAN_POINT ( 'NONE',  ( -188.4702232936788278, -23.48628015402999836, 43.05505437950382941 ) ) ;
#506=CARTESIAN_POINT ( 'NONE',  ( 192.4448373802100889, 14.14213562375873678, 14.14213562375894817 ) ) ;
#507=CARTESIAN_POINT ( 'NONE',  ( -100.7734535825088500, -44.31723036834885932, -12.25131212657538171 ) ) ;
#508=CARTESIAN_POINT ( 'NONE',  ( -198.0356074513804572, -10.87444709759714634, -10.87444709759729911 ) ) ;
#510=CARTESIAN_POINT ( 'NONE',  ( 19.06497207195981147, -10.03556273973425483, -10.03556273973443247 ) ) ;
#511=CARTESIAN_POINT ( 'NONE',  ( 4.995406935893290878, 39.06748935135239265, -39.06748935135144762 ) ) ;
#512=CARTESIAN_POINT ( 'NONE',  ( -86.96347745069644475, 12.89780903124349898, 43.67073346367994446 ) ) ;
#513=CARTESIAN_POINT ( 'NONE',  ( -100.7734535825088358, -17.32597176626813251, -2.449293598294708485E-15 ) ) ;
#514=CARTESIAN_POINT ( 'NONE',  ( 91.82158438592158234, 22.79471317813471742, 40.00000000000002132 ) ) ;
#515=CARTESIAN_POINT ( 'NONE',  ( -56.48582580120558561, -40.00000000000012790, 9.153146818113166105 ) ) ;
#516=CARTESIAN_POINT ( 'NONE',  ( -91.56559293963834989, 12.25131212657490209, -44.31723036834897300 ) ) ;
#518=CARTESIAN_POINT ( 'NONE',  ( 14.38125909742181996, -10.73282306405815234, -67.30136555898266693 ) ) ;
#519=CARTESIAN_POINT ( 'NONE',  ( -56.48582580120559271, 6.472252184284211118, -6.472252184284153387 ) ) ;
#520=ORIENTED_EDGE ( 'NONE', *, *, #25095, .F. ) ;
#521=CARTESIAN_POINT ( 'NONE',  ( 192.4448373802101173, -14.14213562375886291, 42.42640687116498555 ) ) ;
#522=CARTESIAN_POINT ( 'NONE',  ( 169.9999999999999432, 22.62041470344884075, 9.369682556672378482 ) ) ;
#523=CARTESIAN_POINT ( 'NONE',  ( -100.7734535825088500, 16.03295912088683295, 40.53558337403684675 ) ) ;
#524=CARTESIAN_POINT ( 'NONE',  ( 7.112934525950139530, -44.84100494512853885, -18.57375239871706185 ) ) ;
#525=VERTEX_POINT ( 'NONE', #9736 ) ;
#527=CARTESIAN_POINT ( 'NONE',  ( -90.07798792367799479, -15.74993999324178162, -15.74993999324182248 ) ) ;
#530=CIRCLE ( 'NONE', #25177, 14.99999999999999822 ) ;
#533=CARTESIAN_POINT ( 'NONE',  ( 192.4448373802101173, 19.99999999996063949, 40.00000000000002132 ) ) ;
#536=EDGE_CURVE ( 'NONE', #22653, #12962, #21308, .T. ) ;
#537=CARTESIAN_POINT ( 'NONE',  ( -162.0762913951020607, -57.76657433537922515, -1.198031840455874963 ) ) ;
#538=CARTESIAN_POINT ( 'NONE',  ( 184.8905102610680444, -40.00000000000005684, 19.07866798485543569 ) ) ;
#539=CARTESIAN_POINT ( 'NONE',  ( 0.2972598230769883387, 39.99999999999997158, 14.33493731733947563 ) ) ;
#541=CARTESIAN_POINT ( 'NONE',  ( 14.38125909742181285, -15.17850393972633505, 0.000000000000000000 ) ) ;
#543=EDGE_CURVE ( 'NONE', #14909, #16811, #17780, .T. ) ;
#544=CARTESIAN_POINT ( 'NONE',  ( -100.7734535825088358, -17.32597176626813251, -2.449293598294708485E-15 ) ) ;
#546=CARTESIAN_POINT ( 'NONE',  ( -208.1127848780264742, -38.89260858015758515, 38.89260858015713751 ) ) ;
#547=CARTESIAN_POINT ( 'NONE',  ( -114.4364955367327354, 8.064892380842190178, 20.29001642038852182 ) ) ;
#548=CARTESIAN_POINT ( 'NONE',  ( -105.2109270643250909, 16.13380223203129304, -14.21138704485549731 ) ) ;
#549=CARTESIAN_POINT ( 'NONE',  ( -56.48582580120558561, 3.151766524733697544E-13, -30.84685318188644132 ) ) ;
#550=CARTESIAN_POINT ( 'NONE',  ( 192.4448373802100889, -3.692737725850373501E-14, 19.99999999996060751 ) ) ;
#551=CARTESIAN_POINT ( 'NONE',  ( 200.0000000000000000, 14.14213562373100608, -42.42640687119291698 ) ) ;
#554=CARTESIAN_POINT ( 'NONE',  ( 91.82158438592156813, -16.11829626348402655, -40.45024623143966380 ) ) ;
#558=CARTESIAN_POINT ( 'NONE',  ( 136.1360204305621551, -4.966164525587036138, -40.00000000000002132 ) ) ;
#559=CARTESIAN_POINT ( 'NONE',  ( -87.11144460191506766, -21.34775735502242000, -2.726834743463422583 ) ) ;
#560=CARTESIAN_POINT ( 'NONE',  ( -192.9588430854689989, 10.23066800230756712, -10.23066800230735396 ) ) ;
#562=( BOUNDED_SURFACE ( )  B_SPLINE_SURFACE ( 3, 3, ( 
 ( #2606, #10719, #25098, #14964, #10577, #12567, #4870, #12974, #18828, #18692, #24826, #608, #21097, #477, #6579, #2877, #10985, #19095, #25223, #21357, #5129, #15468, #11229, #7110, #25867, #3126, #9623, #19347, #17216, #13603 ),
 ( #19602, #9489, #1388, #7611, #11353, #15726, #21861, #23597, #25355, #13235, #11607, #5376, #7356, #11742, #23851, #17347, #19730, #17470, #25612, #9360, #23476, #13480, #9106, #21602, #9240, #3375, #1256, #11474, #17593, #3637 ),
 ( #15221, #21732, #1136, #23352, #25733, #5248, #3508, #7484, #15596, #19862, #5502, #23721, #1517, #17726, #5629, #25483, #13735, #7232, #15352, #13352, #21474, #3249, #19469, #20137, #9888, #2051, #13871, #14143, #16407, #3918 ),
 ( #6164, #5899, #24128, #42, #8018, #22275, #18261, #16001, #10290, #7880, #1915, #5763, #6291, #12409, #4049, #17856, #6037, #12150, #12281, #175, #22004, #24535, #4319, #20272, #8155, #26137, #14008, #26279, #10158, #3775 ),
 ( #1784, #16269, #14409, #24398, #17990, #22410, #14274, #11878, #10020, #26007, #4186, #19998, #16133, #20408, #12017, #2182, #22539, #23984, #1647, #18398, #24264, #15855, #8281, #9755, #18129, #7743, #22137, #4712, #19064, #22802 ),
 ( #25199, #12816, #18663, #6422, #10822, #2305, #20806, #23194, #24800, #449, #10414, #8956, #16799, #14800, #8821, #20939, #8553, #4579, #2717, #24936, #2577, #18935, #847, #18532, #17065, #313, #25067, #24665, #8415, #717 ),
 ( #18803, #16932, #6946, #6818, #6686, #22932, #12948, #23071, #10551, #14935, #2439, #583, #15064, #16537, #14540, #22670, #12676, #16669, #4842, #4442, #21064, #4975, #10691, #20534, #6552, #12536, #2850, #14662, #20670, #10958 ) ),
 .UNSPECIFIED., .T., .F., .F. ) 
 B_SPLINE_SURFACE_WITH_KNOTS ( ( 4, 3, 4 ),
 ( 4, 2, 2, 2, 2, 2, 2, 2, 2, 2, 2, 2, 2, 2, 4 ),
 ( 0.000000000000000000, 0.5000000000000000000, 1.000000000000000000 ),
 ( 0.000000000000000000, 0.1357259735107005372, 0.1651108541090157700, 0.1944957347073310028, 0.3598804999793158710, 0.3867117631979620773, 0.4135430264166082281, 0.5789277916885930964, 0.6062785021374117456, 0.6336292125862302838, 0.8508620842112317728, 0.8814014469398914198, 0.9119408096685510667, 0.9559704048342755334, 1.000000000000000000 ),
 .UNSPECIFIED. ) 
 GEOMETRIC_REPRESENTATION_ITEM ( )  RATIONAL_B_SPLINE_SURFACE ( (
 ( 1.000000000000000000, 1.000000000000000000, 1.000000000000000000, 1.000000000000000000, 1.000000000000000000, 1.000000000000000000, 1.000000000000000000, 1.000000000000000000, 1.000000000000000000, 1.000000000000000000, 1.000000000000000000, 1.000000000000000000, 1.000000000000000000, 1.000000000000000000, 1.000000000000000000, 1.000000000000000000, 1.000000000000000000, 1.000000000000000000, 1.000000000000000000, 1.000000000000000000, 1.000000000000000000, 1.000000000000000000, 1.000000000000000000, 1.000000000000000000, 1.000000000000000000, 1.000000000000000000, 1.000000000000000000, 1.000000000000000000, 1.000000000000000000, 1.000000000000000000),
 ( 0.3333333333333333703, 0.3333333333333333703, 0.3333333333333333703, 0.3333333333333333703, 0.3333333333333333703, 0.3333333333333333703, 0.3333333333333333703, 0.3333333333333333703, 0.3333333333333333703, 0.3333333333333333703, 0.3333333333333333703, 0.3333333333333333703, 0.3333333333333333703, 0.3333333333333333703, 0.3333333333333333703, 0.3333333333333333703, 0.3333333333333333703, 0.3333333333333333703, 0.3333333333333333703, 0.3333333333333333703, 0.3333333333333333703, 0.3333333333333333703, 0.3333333333333333703, 0.3333333333333333703, 0.3333333333333333703, 0.3333333333333333703, 0.3333333333333333703, 0.3333333333333333703, 0.3333333333333333703, 0.3333333333333333703),
 ( 0.3333333333333333703, 0.3333333333333333703, 0.3333333333333333703, 0.3333333333333333703, 0.3333333333333333703, 0.3333333333333333703, 0.3333333333333333703, 0.3333333333333333703, 0.3333333333333333703, 0.3333333333333333703, 0.3333333333333333703, 0.3333333333333333703, 0.3333333333333333703, 0.3333333333333333703, 0.3333333333333333703, 0.3333333333333333703, 0.3333333333333333703, 0.3333333333333333703, 0.3333333333333333703, 0.3333333333333333703, 0.3333333333333333703, 0.3333333333333333703, 0.3333333333333333703, 0.3333333333333333703, 0.3333333333333333703, 0.3333333333333333703, 0.3333333333333333703, 0.3333333333333333703, 0.3333333333333333703, 0.3333333333333333703),
 ( 1.000000000000000000, 1.000000000000000000, 1.000000000000000000, 1.000000000000000000, 1.000000000000000000, 1.000000000000000000, 1.000000000000000000, 1.000000000000000000, 1.000000000000000000, 1.000000000000000000, 1.000000000000000000, 1.000000000000000000, 1.000000000000000000, 1.000000000000000000, 1.000000000000000000, 1.000000000000000000, 1.000000000000000000, 1.000000000000000000, 1.000000000000000000, 1.000000000000000000, 1.000000000000000000, 1.000000000000000000, 1.000000000000000000, 1.000000000000000000, 1.000000000000000000, 1.000000000000000000, 1.000000000000000000, 1.000000000000000000, 1.000000000000000000, 1.000000000000000000),
 ( 0.3333333333333333703, 0.3333333333333333703, 0.3333333333333333703, 0.3333333333333333703, 0.3333333333333333703, 0.3333333333333333703, 0.3333333333333333703, 0.3333333333333333703, 0.3333333333333333703, 0.3333333333333333703, 0.3333333333333333703, 0.3333333333333333703, 0.3333333333333333703, 0.3333333333333333703, 0.3333333333333333703, 0.3333333333333333703, 0.3333333333333333703, 0.3333333333333333703, 0.3333333333333333703, 0.3333333333333333703, 0.3333333333333333703, 0.3333333333333333703, 0.3333333333333333703, 0.3333333333333333703, 0.3333333333333333703, 0.3333333333333333703, 0.3333333333333333703, 0.3333333333333333703, 0.3333333333333333703, 0.3333333333333333703),
 ( 0.3333333333333333703, 0.3333333333333333703, 0.3333333333333333703, 0.3333333333333333703, 0.3333333333333333703, 0.3333333333333333703, 0.3333333333333333703, 0.3333333333333333703, 0.3333333333333333703, 0.3333333333333333703, 0.3333333333333333703, 0.3333333333333333703, 0.3333333333333333703, 0.3333333333333333703, 0.3333333333333333703, 0.3333333333333333703, 0.3333333333333333703, 0.3333333333333333703, 0.3333333333333333703, 0.3333333333333333703, 0.3333333333333333703, 0.3333333333333333703, 0.3333333333333333703, 0.3333333333333333703, 0.3333333333333333703, 0.3333333333333333703, 0.3333333333333333703, 0.3333333333333333703, 0.3333333333333333703, 0.3333333333333333703),
 ( 1.000000000000000000, 1.000000000000000000, 1.000000000000000000, 1.000000000000000000, 1.000000000000000000, 1.000000000000000000, 1.000000000000000000, 1.000000000000000000, 1.000000000000000000, 1.000000000000000000, 1.000000000000000000, 1.000000000000000000, 1.000000000000000000, 1.000000000000000000, 1.000000000000000000, 1.000000000000000000, 1.000000000000000000, 1.000000000000000000, 1.000000000000000000, 1.000000000000000000, 1.000000000000000000, 1.000000000000000000, 1.000000000000000000, 1.000000000000000000, 1.000000000000000000, 1.000000000000000000, 1.000000000000000000, 1.000000000000000000, 1.000000000000000000, 1.000000000000000000) ) ) 
 REPRESENTATION_ITEM ( '' )  SURFACE ( )  );
#565=CARTESIAN_POINT ( 'NONE',  ( -103.9663809733945499, 8.026122151960143114, -20.15238534321454367 ) ) ;
#566=CARTESIAN_POINT ( 'NONE',  ( 23.26364522859735828, 23.36474233297307990, 42.89098160628132916 ) ) ;
#569=CARTESIAN_POINT ( 'NONE',  ( 136.1360204305621551, -53.05693388239313890, 3.511608612530593199 ) ) ;
#571=CARTESIAN_POINT ( 'NONE',  ( -110.1018001840315321, 0.6219992248577108640, 20.19553435165690658 ) ) ;
#572=CARTESIAN_POINT ( 'NONE',  ( 192.4448373802100889, -14.14213562375876698, -14.14213562375885047 ) ) ;
#574=CARTESIAN_POINT ( 'NONE',  ( -208.1127848780264742, 39.99999999999992895, 15.00245453012683683 ) ) ;
#577=CARTESIAN_POINT ( 'NONE',  ( -198.0356074513804572, 40.00000000000056843, -55.37879056871282302 ) ) ;
#578=CARTESIAN_POINT ( 'NONE',  ( -259.2033419157646676, 39.99999999999987921, 9.517827891723049660 ) ) ;
#582=CARTESIAN_POINT ( 'NONE',  ( -188.9266304146001971, 17.94050393342739014, 43.31220791188948738 ) ) ;
#583=CARTESIAN_POINT ( 'NONE',  ( -91.56559293963836410, 16.03295912088692177, 16.03295912088721664 ) ) ;
#585=CARTESIAN_POINT ( 'NONE',  ( -56.48582580120558561, 6.472252184283903809, 50.09629031063968796 ) ) ;
#587=CARTESIAN_POINT ( 'NONE',  ( -105.3755690713226727, -12.89780903124395550, -12.89780903124416511 ) ) ;
#588=CARTESIAN_POINT ( 'NONE',  ( -199.9999999999998010, 49.28189405767604114, -14.17215463606931181 ) ) ;
#589=CARTESIAN_POINT ( 'NONE',  ( 91.82158438592158234, 17.20528682183301683, 0.000000000000000000 ) ) ;
#590=CARTESIAN_POINT ( 'NONE',  ( 136.1360204305621266, -24.77266263493151044, 24.77266263493093135 ) ) ;
#591=CARTESIAN_POINT ( 'NONE',  ( -259.2033419157646676, 9.517827891722584255, -0.000000000000000000 ) ) ;
#593=ORIENTED_EDGE ( 'NONE', *, *, #11245, .T. ) ;
#594=CARTESIAN_POINT ( 'NONE',  ( -162.0762913951020892, -39.99999999999961631, -41.69427287692722928 ) ) ;
#596=CARTESIAN_POINT ( 'NONE',  ( 137.0939645874030361, -12.56330697291285681, 30.33050608226178468 ) ) ;
#597=ORIENTED_EDGE ( 'NONE', *, *, #20606, .T. ) ;
#598=ORIENTED_EDGE ( 'NONE', *, *, #21416, .F. ) ;
#599=CARTESIAN_POINT ( 'NONE',  ( -280.0000000000000000, 19.99999999999996092, 2.449293598294708485E-15 ) ) ;
#601=CARTESIAN_POINT ( 'NONE',  ( -114.7824662269243561, -22.13040512707748064, -1.403530270405573210 ) ) ;
#602=CARTESIAN_POINT ( 'NONE',  ( 107.5473083967388277, -16.96446921415041587, -16.96446921415049403 ) ) ;
#603=( BOUNDED_CURVE ( )  B_SPLINE_CURVE ( 3, ( #11156, #15517, #13403, #11526 ),
 .UNSPECIFIED., .F., .F. ) 
 B_SPLINE_CURVE_WITH_KNOTS ( ( 4, 4 ),
 ( 0.01577215542394082640, 0.02369175774463767523 ),
 .UNSPECIFIED. ) 
 CURVE ( )  GEOMETRIC_REPRESENTATION_ITEM ( )  RATIONAL_B_SPLINE_CURVE ( ( 0.5197830649482693133, 0.5065943549827455206, 0.4999999999999891198, 0.5000000000000001110 ) ) 
 REPRESENTATION_ITEM ( '' )  );
#606=CARTESIAN_POINT ( 'NONE',  ( -105.4741150117382062, 7.943527260750565588, -19.77569912955109288 ) ) ;
#607=CARTESIAN_POINT ( 'NONE',  ( -105.3755690713226585, -43.67073346367964604, -12.89780903124457545 ) ) ;
#608=CARTESIAN_POINT ( 'NONE',  ( -91.56559293963836410, 16.03295912088692177, 16.03295912088721664 ) ) ;
#610=CARTESIAN_POINT ( 'NONE',  ( -192.9588430854690273, 40.00000000000055422, -54.46834944101679810 ) ) ;
#611=CARTESIAN_POINT ( 'NONE',  ( -88.39148973765144035, -8.027153355909462107, 20.15708830332390988 ) ) ;
#613=CARTESIAN_POINT ( 'NONE',  ( -238.4067589809705794, -0.9644942799826262680, 0.000000000000000000 ) ) ;
#614=CARTESIAN_POINT ( 'NONE',  ( 163.1118516004056573, -19.27778845538761132, -19.27778845538770724 ) ) ;
#615=CARTESIAN_POINT ( 'NONE',  ( 146.6084372240433709, -32.08495691632041513, -24.48358557860343154 ) ) ;
#618=CARTESIAN_POINT ( 'NONE',  ( -208.1127848780265026, -9.061048840815752106E-14, 15.00245453012669472 ) ) ;
#619=CARTESIAN_POINT ( 'NONE',  ( 36.66494225463969059, 39.17447069122760439, -16.22659705898878002 ) ) ;
#620=CARTESIAN_POINT ( 'NONE',  ( 91.82158438592158234, -17.20528682183298486, -40.00000000000002132 ) ) ;
#621=CARTESIAN_POINT ( 'NONE',  ( 192.4448373802101173, -42.42640687122073473, 14.14213562370301780 ) ) ;
#622=CARTESIAN_POINT ( 'NONE',  ( 130.8568914410475372, -34.05028731879786363, 0.000000000000000000 ) ) ;
#623=ORIENTED_EDGE ( 'NONE', *, *, #25019, .T. ) ;
#624=CARTESIAN_POINT ( 'NONE',  ( 6.615221834168117709, -44.82734842560460464, 24.79576599681886151 ) ) ;
#625=CARTESIAN_POINT ( 'NONE',  ( -30.26275506840324425, 41.69427246844627177, 40.00000000000002132 ) ) ;
#628=CARTESIAN_POINT ( 'NONE',  ( -199.9999999999998579, 24.82633483071252201, 44.86878812508700776 ) ) ;
#629=CARTESIAN_POINT ( 'NONE',  ( 199.9999999999999432, -14.14213562373096345, -14.14213562373104871 ) ) ;
#630=CARTESIAN_POINT ( 'NONE',  ( -39.81953879995582213, -16.38089232936994222, 32.18669035977284665 ) ) ;
#632=CARTESIAN_POINT ( 'NONE',  ( -4.151555265633182223, 23.42746911247800057, -42.97219445042047425 ) ) ;
#634=CARTESIAN_POINT ( 'NONE',  ( -259.2033419157646676, 21.55415060305790931, 35.01439189186571355 ) ) ;
#635=CARTESIAN_POINT ( 'NONE',  ( -77.59415595804631494, -21.92621357339736221, 2.768978254285019425 ) ) ;
#637=CARTESIAN_POINT ( 'NONE',  ( -190.7346372394937077, -13.94676542150760312, 47.78727444208784192 ) ) ;
#638=CARTESIAN_POINT ( 'NONE',  ( -280.0000000000000000, 14.14213562373078581, 14.14213562373108424 ) ) ;
#639=ADVANCED_FACE ( 'NONE', ( #7380 ), #10777, .T. ) ;
#640=CARTESIAN_POINT ( 'NONE',  ( 4.995406935893287326, 17.50105314357170627, 39.06748935135200895 ) ) ;
#641=CARTESIAN_POINT ( 'NONE',  ( -280.0000000000000000, -14.14213562373118549, 14.14213562373078936 ) ) ;
#642=CARTESIAN_POINT ( 'NONE',  ( -91.56559293963836410, 16.03295912088692177, 16.03295912088721664 ) ) ;
#643=CARTESIAN_POINT ( 'NONE',  ( -238.4067589809705794, 27.60227080167080160, -28.96627169325299533 ) ) ;
#644=CARTESIAN_POINT ( 'NONE',  ( -100.7734535825088358, 12.25131212657497848, -12.25131212657469604 ) ) ;
#645=CARTESIAN_POINT ( 'NONE',  ( -259.2033419157646676, 49.83842185052017015, 6.730120644404137487 ) ) ;
#646=CARTESIAN_POINT ( 'NONE',  ( 136.1360204305621266, 35.03383547441298163, 40.00000000000002132 ) ) ;
#647=CARTESIAN_POINT ( 'NONE',  ( -213.1075012329537230, 13.71589010951907817, -40.00000000000002132 ) ) ;
#648=CARTESIAN_POINT ( 'NONE',  ( -238.4067589809705794, 28.96627169325324758, -27.60227080167054581 ) ) ;
#649=CARTESIAN_POINT ( 'NONE',  ( -102.4294859495854411, 20.29697089060380222, -8.407280617849153259 ) ) ;
#650=CARTESIAN_POINT ( 'NONE',  ( -213.1075012329536946, -37.98287015391210275, -37.98287015391272092 ) ) ;
#651=CARTESIAN_POINT ( 'NONE',  ( -151.7004365444681468, 32.50163950438717109, -13.46261988206755333 ) ) ;
#652=ORIENTED_EDGE ( 'NONE', *, *, #9331, .F. ) ;
#653=CARTESIAN_POINT ( 'NONE',  ( -213.1075012329537230, 66.26714140136188291, 9.698598906438215650 ) ) ;
#654=CARTESIAN_POINT ( 'NONE',  ( -86.86493150570990451, 7.943527260495432785, 19.77569912839167898 ) ) ;
#655=CARTESIAN_POINT ( 'NONE',  ( -135.8532207217289738, -21.81201906317788186, 21.81201906317762962 ) ) ;
#656=CARTESIAN_POINT ( 'NONE',  ( 16.03312633933773768, -44.50221493480259483, -18.43342098165166121 ) ) ;
#657=ORIENTED_EDGE ( 'NONE', *, *, #3627, .F. ) ;
#661=CARTESIAN_POINT ( 'NONE',  ( -114.5523123854244716, -20.89198064830845425, 6.807555700458482129 ) ) ;
#662=CARTESIAN_POINT ( 'NONE',  ( 91.82158438592158234, 22.79471317813472098, 2.449293598294708485E-15 ) ) ;
#663=CARTESIAN_POINT ( 'NONE',  ( -105.4894168351564048, 19.67999904371083275, 8.151722511394638104 ) ) ;
#666=CARTESIAN_POINT ( 'NONE',  ( 130.8568914410475088, -4.207082182990058428, 52.36146031193416661 ) ) ;
#667=CARTESIAN_POINT ( 'NONE',  ( 91.82158438592158234, -6.516925787240506436E-14, 22.79471317813470321 ) ) ;
#668=CARTESIAN_POINT ( 'NONE',  ( 57.59792236341146321, 40.00000000000004263, -2.435789363418021214 ) ) ;
#670=CARTESIAN_POINT ( 'NONE',  ( -30.26275506840322649, -41.69427246844630019, -2.449293598294708485E-15 ) ) ;
#671=CARTESIAN_POINT ( 'NONE',  ( 23.42154907652910012, -13.79745687233715046, -46.79103593565392316 ) ) ;
#672=CARTESIAN_POINT ( 'NONE',  ( 19.06497207195981147, -10.03556273973439517, 10.03556273973429214 ) ) ;
#673=CARTESIAN_POINT ( 'NONE',  ( 200.0000000000000000, -19.99999999999988631, -40.00000000000002132 ) ) ;
#674=CARTESIAN_POINT ( 'NONE',  ( 163.1118516004056573, 19.27778845539212327, 37.29075403953164169 ) ) ;
#675=CARTESIAN_POINT ( 'NONE',  ( 156.1979191798867248, -11.34289806466571271, -27.38417834433185760 ) ) ;
#677=CARTESIAN_POINT ( 'NONE',  ( -91.56559293963834989, 1.671088883502053755E-13, -17.32597176626811120 ) ) ;
#678=CARTESIAN_POINT ( 'NONE',  ( 14.38125909742180930, 39.99999999999982947, 55.17850393971022527 ) ) ;
#679=CARTESIAN_POINT ( 'NONE',  ( 130.8568914410475088, 4.207082182989741348, -52.36146031193420924 ) ) ;
#681=CARTESIAN_POINT ( 'NONE',  ( -86.86493150571116928, -8.366608963953867217, -19.60045294882765887 ) ) ;
#682=CARTESIAN_POINT ( 'NONE',  ( 14.38125909742182529, -39.01709431150933938, 39.01709431150894147 ) ) ;
#683=ORIENTED_EDGE ( 'NONE', *, *, #9481, .F. ) ;
#684=CARTESIAN_POINT ( 'NONE',  ( -192.9588430854689989, -10.23066800230742501, -10.23066800230756712 ) ) ;
#686=CARTESIAN_POINT ( 'NONE',  ( 163.1118516004056573, -12.73709011382471878, -40.00000000000002132 ) ) ;
#688=CARTESIAN_POINT ( 'NONE',  ( -114.6679276626366430, 11.81543316366880525, -18.60595090114481920 ) ) ;
#689=CARTESIAN_POINT ( 'NONE',  ( 151.7948205124836250, -23.49921654116371883, 23.49921654116317526 ) ) ;
#691=ORIENTED_EDGE ( 'NONE', *, *, #23589, .F. ) ;
#696=DIRECTION ( 'NONE',  ( 1.000000000000000000, 0.000000000000000000, 0.000000000000000000 ) ) ;
#697=EDGE_CURVE ( 'NONE', #5841, #23332, #14292, .T. ) ;
#698=ORIENTED_EDGE ( 'NONE', *, *, #18324, .T. ) ;
#699=ORIENTED_EDGE ( 'NONE', *, *, #4311, .T. ) ;
#700=CARTESIAN_POINT ( 'NONE',  ( -280.0000000000000568, -42.42640687119295251, 14.14213562373088351 ) ) ;
#704=EDGE_CURVE ( 'NONE', #13948, #1209, #14934, .T. ) ;
#706=CARTESIAN_POINT ( 'NONE',  ( -105.3755690713226585, -15.38646221621796251, 41.18208027870593924 ) ) ;
#707=CARTESIAN_POINT ( 'NONE',  ( 14.38125909742180752, 10.73282306404720465, 10.73282306404724018 ) ) ;
#708=CARTESIAN_POINT ( 'NONE',  ( 146.6084372240433709, 40.00000000000017053, -34.62501878078291639 ) ) ;
#709=CARTESIAN_POINT ( 'NONE',  ( -114.4364955367328491, -20.29001642038857156, 8.064892380842218600 ) ) ;
#711=CARTESIAN_POINT ( 'NONE',  ( 14.38125909742181818, 5.830552384690105017E-13, -55.17850393972636880 ) ) ;
#712=CARTESIAN_POINT ( 'NONE',  ( 0.2972598230769957217, 1.502051041545559470E-13, -14.33493731733933352 ) ) ;
#714=CARTESIAN_POINT ( 'NONE',  ( -87.13361725327075646, -16.16779225783700724, -14.22820416757983253 ) ) ;
#716=CARTESIAN_POINT ( 'NONE',  ( -190.0144222803280627, 13.91469272132741963, 47.57278142030602908 ) ) ;
#717=CARTESIAN_POINT ( 'NONE',  ( 200.0000000000000000, -14.14213562373122457, 42.42640687119282461 ) ) ;
#718=CARTESIAN_POINT ( 'NONE',  ( -93.02511667907126025, 8.946512270084744145, 20.50052124204852078 ) ) ;
#719=CARTESIAN_POINT ( 'NONE',  ( 200.0000000000000000, 14.14213562373083022, 42.42640687119289566 ) ) ;
#720=CARTESIAN_POINT ( 'NONE',  ( -77.55743582226475041, 22.12574471220127137, 0.8414656003864237066 ) ) ;
#721=CARTESIAN_POINT ( 'NONE',  ( 163.1118516004056573, 19.27778845539265618, -37.29075403953135037 ) ) ;
#723=CARTESIAN_POINT ( 'NONE',  ( -135.8532207217289738, 9.153146818113546246, -0.000000000000000000 ) ) ;
#725=CARTESIAN_POINT ( 'NONE',  ( -100.7734535825088500, 12.25131212657428748, 44.31723036834913643 ) ) ;
#726=CARTESIAN_POINT ( 'NONE',  ( 57.59792236341147031, 2.435789363418170872, 40.00000000000002132 ) ) ;
#729=ORIENTED_EDGE ( 'NONE', *, *, #3071, .F. ) ;
#730=CARTESIAN_POINT ( 'NONE',  ( 0.2972598230770103767, -39.99999999999945288, -54.33493731733979359 ) ) ;
#736=CARTESIAN_POINT ( 'NONE',  ( 130.8568914410475088, 5.949712681206712261, 40.00000000000002132 ) ) ;
#738=CARTESIAN_POINT ( 'NONE',  ( -100.0968563617347797, -20.72609133250457703, -8.149320301440017289 ) ) ;
#739=CARTESIAN_POINT ( 'NONE',  ( -105.4741150117382489, -19.77569912955116749, -7.943527260750408381 ) ) ;
#741=CARTESIAN_POINT ( 'NONE',  ( 146.6084372240433993, -24.48358557860319706, -24.48358557860330720 ) ) ;
#742=CARTESIAN_POINT ( 'NONE',  ( -30.26275506840324070, -1.147469862568086380E-14, 1.694272468446259783 ) ) ;
#745=CARTESIAN_POINT ( 'NONE',  ( 0.2972598230770011618, 10.13633138497555919, -66.70487387989845729 ) ) ;
#746=CARTESIAN_POINT ( 'NONE',  ( 146.6084372240433709, -3.800685668859084210, 52.76785682606516303 ) ) ;
#747=DIRECTION ( 'NONE',  ( 1.000000000000000000, 1.836970198721030181E-16, 0.000000000000000000 ) ) ;
#748=CARTESIAN_POINT ( 'NONE',  ( -162.0762913951021176, 40.00000000000001421, -1.694272876827905394 ) ) ;
#750=CARTESIAN_POINT ( 'NONE',  ( -135.8532207217289738, 9.153146818113546246, -0.000000000000000000 ) ) ;
#751=CARTESIAN_POINT ( 'NONE',  ( -280.0000000000000568, 14.14213562373067745, 42.42640687119295251 ) ) ;
#754=CARTESIAN_POINT ( 'NONE',  ( -87.13361725327074225, -15.19799821270821560, -15.19799821270861884 ) ) ;
#755=CARTESIAN_POINT ( 'NONE',  ( -192.9588430854689989, 14.46834944099965981, 0.000000000000000000 ) ) ;
#756=CARTESIAN_POINT ( 'NONE',  ( 151.7948205124836250, -23.49921654116339553, -23.49921654116350211 ) ) ;
#757=CARTESIAN_POINT ( 'NONE',  ( 163.1118516004056573, -27.26290988616869626, 0.000000000000000000 ) ) ;
#759=CARTESIAN_POINT ( 'NONE',  ( 17.65190074001006693, -48.50354960737486465, 14.05440436229930867 ) ) ;
#760=CARTESIAN_POINT ( 'NONE',  ( -192.9588430854690273, 14.46834944099966336, -40.00000000000002132 ) ) ;
#762=CARTESIAN_POINT ( 'NONE',  ( -105.2334157265390502, 16.99665894158216872, -13.14152336620543338 ) ) ;
#763=CARTESIAN_POINT ( 'NONE',  ( -56.48582580120559982, -34.75652343174615311, 21.81201906317766870 ) ) ;
#764=CARTESIAN_POINT ( 'NONE',  ( -70.30307074955213409, -8.711708290686113187, 23.14841683089695934 ) ) ;
#765=CARTESIAN_POINT ( 'NONE',  ( -82.26600655510863191, 19.56860215688234561, -4.953608811515387345 ) ) ;
#766=CARTESIAN_POINT ( 'NONE',  ( -5.859158571312478081, 23.09435402965887363, -42.46836465824239326 ) ) ;
#768=CARTESIAN_POINT ( 'NONE',  ( 130.8568914410475088, 4.207082182989012153, 52.36146031193425188 ) ) ;
#769=CARTESIAN_POINT ( 'NONE',  ( -87.13361725327075646, -21.49321519333432207, -1.155557966632341512E-30 ) ) ;
#771=CARTESIAN_POINT ( 'NONE',  ( -188.4265466358341428, -13.83489705870445263, 47.03621809928723252 ) ) ;
#772=CARTESIAN_POINT ( 'NONE',  ( 184.8905102610680444, 14.79361573936375507, 14.79361573936398067 ) ) ;
#773=CARTESIAN_POINT ( 'NONE',  ( -105.3755690713226727, 15.38646221621793231, -15.38646221621779020 ) ) ;
#774=CARTESIAN_POINT ( 'NONE',  ( -280.0000000000000568, -42.42640687119276066, -14.14213562373147148 ) ) ;
#775=CARTESIAN_POINT ( 'NONE',  ( -86.86493150571114086, -7.943527260496002107, 19.77569912839178912 ) ) ;
#776=LINE ( 'NONE', #12604, #24053 ) ;
#777=CARTESIAN_POINT ( 'NONE',  ( 146.6084372240433709, 32.08495691632030145, 24.48358557860365181 ) ) ;
#778=CARTESIAN_POINT ( 'NONE',  ( 130.8568914410475372, 4.207082182992923691, -4.207082182992794017 ) ) ;
#779=CARTESIAN_POINT ( 'NONE',  ( 170.2234770963711128, 24.55285855007190676, 40.00000000000002132 ) ) ;
#780=CARTESIAN_POINT ( 'NONE',  ( 192.4448373802101173, 19.99999999996065014, -40.00000000000002132 ) ) ;
#781=CARTESIAN_POINT ( 'NONE',  ( 91.82158438592158234, 16.11829626348434630, -40.45024623143955012 ) ) ;
#784=CARTESIAN_POINT ( 'NONE',  ( 0.2972598230770027716, -38.42060263243681817, 18.14793986248684377 ) ) ;
#785=CARTESIAN_POINT ( 'NONE',  ( -184.9729924864344355, 42.02333070177955676, -22.80024897327513500 ) ) ;
#787=CARTESIAN_POINT ( 'NONE',  ( 19.06497207195981858, 10.03556273973424062, 66.60410523465820631 ) ) ;
#788=CARTESIAN_POINT ( 'NONE',  ( -86.95457011089800403, -19.12034330075778854, -9.640471311020448297 ) ) ;
#790=CARTESIAN_POINT ( 'NONE',  ( 199.9999999999999432, -14.14213562373093680, 14.14213562373082311 ) ) ;
#791=CARTESIAN_POINT ( 'NONE',  ( 9.345847406375622057, -49.32890504404500831, -14.17927947630055741 ) ) ;
#792=EDGE_LOOP ( 'NONE', ( #18200, #12963, #12220, #17200 ) ) ;
#793=DIRECTION ( 'NONE',  ( -0.01051738777840850216, -0.9307051272558640731, 0.3656191333258757004 ) ) ;
#794=CARTESIAN_POINT ( 'NONE',  ( -110.0738206587849390, -10.29063887146194034, -17.41030175792333168 ) ) ;
#797=CARTESIAN_POINT ( 'NONE',  ( -114.6679276626352788, -21.51116696530653627, -4.801621139945174477 ) ) ;
#798=CARTESIAN_POINT ( 'NONE',  ( -86.96347745069644475, 18.24025645688350750, -40.00000000000002132 ) ) ;
#801=CARTESIAN_POINT ( 'NONE',  ( 57.59792236341147031, -26.56190807104712448, 30.00663442387673285 ) ) ;
#802=CARTESIAN_POINT ( 'NONE',  ( -208.1127848780265026, -2.327190355601776466E-13, 55.00245453012672670 ) ) ;
#803=CARTESIAN_POINT ( 'NONE',  ( -30.26275506840324425, 39.99999999999987210, 41.69427246844643520 ) ) ;
#804=CARTESIAN_POINT ( 'NONE',  ( 184.8905102610680444, 1.070102760522089011E-13, -20.92133201514444352 ) ) ;
#805=CARTESIAN_POINT ( 'NONE',  ( -280.0000000000000568, -20.00000000000006395, -40.00000000000002132 ) ) ;
#806=CARTESIAN_POINT ( 'NONE',  ( 25.62979979008735043, -22.88075396656093830, -42.16299361905900867 ) ) ;
#808=CARTESIAN_POINT ( 'NONE',  ( -213.1075012329537230, -53.71589010953668719, -40.00000000000002132 ) ) ;
#809=CARTESIAN_POINT ( 'NONE',  ( 14.38125909742180752, 17.55144818341448953, 39.01709431150923280 ) ) ;
#810=CARTESIAN_POINT ( 'NONE',  ( 167.0466155511619490, -9.710058186601607133, -23.44215416552599152 ) ) ;
#812=CARTESIAN_POINT ( 'NONE',  ( 4.995406935893306866, -39.99999999999944578, -55.24977328856505920 ) ) ;
#814=CARTESIAN_POINT ( 'NONE',  ( 155.1202959361052365, -27.79909075771130844, -11.51476041348459667 ) ) ;
#816=CARTESIAN_POINT ( 'NONE',  ( -86.96347745069643054, 15.38646221621763210, 41.18208027870604582 ) ) ;
#817=VERTEX_POINT ( 'NONE', #14658 ) ;
#818=CARTESIAN_POINT ( 'NONE',  ( -77.79405973474302982, -6.791823288762519617, -20.85724814835166896 ) ) ;
#819=CARTESIAN_POINT ( 'NONE',  ( -7.769366557093614567, 45.69637362129925862, -13.56374645825293257 ) ) ;
#821=CARTESIAN_POINT ( 'NONE',  ( 130.8568914410475088, -5.949712681206671405, 40.00000000000002132 ) ) ;
#824=CARTESIAN_POINT ( 'NONE',  ( -188.3392535381696007, 47.00481007172025727, -13.83023904993444120 ) ) ;
#826=ORIENTED_EDGE ( 'NONE', *, *, #944, .T. ) ;
#828=CARTESIAN_POINT ( 'NONE',  ( 85.88525995973293448, -8.769880560541459147, 23.37195345519199563 ) ) ;
#829=CARTESIAN_POINT ( 'NONE',  ( 98.29820294267858571, 2.581272653895909208, 20.00000000000376588 ) ) ;
#830=EDGE_LOOP ( 'NONE', ( #20781, #4653, #520, #427 ) ) ;
#832=CARTESIAN_POINT ( 'NONE',  ( 146.6084372240433993, -24.48358557860319706, -24.48358557860330720 ) ) ;
#835=CARTESIAN_POINT ( 'NONE',  ( 91.82158438592158234, -40.45024623143958564, 16.11829626348418998 ) ) ;
#836=CARTESIAN_POINT ( 'NONE',  ( -135.8532207217289738, -6.472252184284190690, -6.472252184284188914 ) ) ;
#837=CARTESIAN_POINT ( 'NONE',  ( 91.82158438592156813, 39.99999999999995737, 22.79471317813484887 ) ) ;
#838=CARTESIAN_POINT ( 'NONE',  ( -199.9999999999999716, -22.84381638316559204, 44.98788141756676140 ) ) ;
#839=CARTESIAN_POINT ( 'NONE',  ( -199.9999999999999432, 10.02640517461945890, 53.44529986889378392 ) ) ;
#840=CARTESIAN_POINT ( 'NONE',  ( -30.26275506840324070, -40.00000000000001421, -1.694272468446678559 ) ) ;
#841=CARTESIAN_POINT ( 'NONE',  ( -30.26275506840323359, 4.336144384597734078E-13, -41.69427246844629309 ) ) ;
#842=CARTESIAN_POINT ( 'NONE',  ( -110.0368417077420560, -18.51665893310633848, 7.992411109433169791 ) ) ;
#843=CARTESIAN_POINT ( 'NONE',  ( -87.13361725327075646, 15.19799821270843765, 15.19799821270837015 ) ) ;
#846=CARTESIAN_POINT ( 'NONE',  ( -86.96347745069644475, 15.38646221621793586, -15.38646221621778842 ) ) ;
#847=CARTESIAN_POINT ( 'NONE',  ( 136.1360204305621266, -3.511608612531119000, 53.05693388239312469 ) ) ;
#849=CARTESIAN_POINT ( 'NONE',  ( 146.6084372240433993, -3.800685668858652999, 3.800685668858636568 ) ) ;
#850=CARTESIAN_POINT ( 'NONE',  ( -280.0000000000000568, 14.14213562373127431, -42.42640687119274645 ) ) ;
#852=CARTESIAN_POINT ( 'NONE',  ( -198.0356074513804572, -15.37879056873074290, 40.00000000000002132 ) ) ;
#853=B_SPLINE_CURVE_WITH_KNOTS ( 'NONE', 3,
 ( #22849, #4624, #12724, #20848, #2626, #10738 ),
 .UNSPECIFIED., .F., .F.,
 ( 4, 2, 4 ),
 ( -0.0001050551439129801008, 0.04006586859759233427, 0.08023679233909764008 ),
 .UNSPECIFIED. ) ;
#855=CARTESIAN_POINT ( 'NONE',  ( -56.48582580120559982, 50.09629031063956717, 6.472252184284792875 ) ) ;
#856=CARTESIAN_POINT ( 'NONE',  ( 151.7948205124835681, 33.23291073765556547, 40.00000000000002132 ) ) ;
#858=VERTEX_POINT ( 'NONE', #4575 ) ;
#859=CARTESIAN_POINT ( 'NONE',  ( 19.06497207195981858, 5.735870351258996432E-13, -54.19242893257843008 ) ) ;
#863=ORIENTED_EDGE ( 'NONE', *, *, #704, .T. ) ;
#864=ORIENTED_EDGE ( 'NONE', *, *, #26060, .T. ) ;
#865=CARTESIAN_POINT ( 'NONE',  ( -213.1075012329537230, 53.71589010953660193, 40.00000000000002132 ) ) ;
#866=CARTESIAN_POINT ( 'NONE',  ( -105.4732637872227770, -19.68494377761401992, -8.153770687239941140 ) ) ;
#868=DIRECTION ( 'NONE',  ( 0.000000000000000000, 0.7071067811865434649, 0.7071067811865516806 ) ) ;
#870=CARTESIAN_POINT ( 'NONE',  ( -114.4364955367327070, -8.644468109209471507, 20.04994829327649342 ) ) ;
#871=CARTESIAN_POINT ( 'NONE',  ( -56.48582580120559271, 2.158176344243877536E-14, -9.153146818113587102 ) ) ;
#874=CARTESIAN_POINT ( 'NONE',  ( -56.48582580120559982, -34.75652343174584047, -21.81201906317815187 ) ) ;
#875=CARTESIAN_POINT ( 'NONE',  ( -280.0000000000000000, 14.14213562373078581, 14.14213562373108424 ) ) ;
#877=CARTESIAN_POINT ( 'NONE',  ( 4.995406935893298872, 5.820775922023080204E-13, -55.24977328854835434 ) ) ;
#881=ADVANCED_FACE ( 'NONE', ( #17061 ), #19573, .T. ) ;
#882=CARTESIAN_POINT ( 'NONE',  ( 4.995406935893310418, -67.35176059880237176, 10.78321810387813429 ) ) ;
#886=CARTESIAN_POINT ( 'NONE',  ( 130.8568914410475088, 40.00000000000015632, -34.05028731879774284 ) ) ;
#887=CARTESIAN_POINT ( 'NONE',  ( -56.48582580120559982, -9.153146818113595984, -40.00000000000002132 ) ) ;
#888=CARTESIAN_POINT ( 'NONE',  ( -259.2033419157646676, -6.730120644403667640, 49.83842185052029805 ) ) ;
#889=CARTESIAN_POINT ( 'NONE',  ( 192.4448373802100889, -20.00000000003938538, 0.000000000000000000 ) ) ;
#891=CARTESIAN_POINT ( 'NONE',  ( -1.087763065927232153, -43.78960619332504223, 24.03018639662561640 ) ) ;
#892=CARTESIAN_POINT ( 'NONE',  ( 192.4448373802101173, 19.99999999996065014, -40.00000000000002132 ) ) ;
#894=CARTESIAN_POINT ( 'NONE',  ( -238.4067589809705794, 28.96627169325315165, 28.96627169325329731 ) ) ;
#895=CARTESIAN_POINT ( 'NONE',  ( -213.1075012329537230, -40.00000000000011369, 13.71589010951897691 ) ) ;
#896=CARTESIAN_POINT ( 'NONE',  ( -86.86493150571119770, 19.77569912839179622, -7.943527260495995002 ) ) ;
#897=CARTESIAN_POINT ( 'NONE',  ( -1.818469002956039970, -13.93708913181221298, -47.72215409237463035 ) ) ;
#899=CARTESIAN_POINT ( 'NONE',  ( -238.4067589809705794, 57.25054294065799354, -0.6820004457334954973 ) ) ;
#900=CARTESIAN_POINT ( 'NONE',  ( -82.23726319249652761, -20.19517362732918642, -9.977985540125272163E-16 ) ) ;
#903=CARTESIAN_POINT ( 'NONE',  ( 136.1360204305621266, 24.77266263493104148, 24.77266263493145004 ) ) ;
#904=CARTESIAN_POINT ( 'NONE',  ( 136.1360204305621551, 24.77266263493108411, 31.79587985999273769 ) ) ;
#905=CARTESIAN_POINT ( 'NONE',  ( -82.30220482034344798, 7.992411108777224271, -18.51665893431685461 ) ) ;
#906=CARTESIAN_POINT ( 'NONE',  ( -208.1127848780265026, -10.60833733269537227, -10.60833733269551793 ) ) ;
#907=CARTESIAN_POINT ( 'NONE',  ( -91.56559293963836410, 44.31723036834908669, -12.25131212657445801 ) ) ;
#908=CARTESIAN_POINT ( 'NONE',  ( -100.7734535825088500, 40.53558337403654832, 16.03295912088756481 ) ) ;
#909=CARTESIAN_POINT ( 'NONE',  ( -208.1127848780265026, 38.89260858015777700, -38.89260858015687461 ) ) ;
#910=CARTESIAN_POINT ( 'NONE',  ( 19.06497207195980792, 54.19242893257844429, -40.00000000000002132 ) ) ;
#911=CARTESIAN_POINT ( 'NONE',  ( -105.3755690713226727, -15.38646221621786481, -15.38646221621789856 ) ) ;
#913=CARTESIAN_POINT ( 'NONE',  ( 19.06497207195982924, -66.60410523465809263, -10.03556273973493163 ) ) ;
#915=CARTESIAN_POINT ( 'NONE',  ( -188.2956751479420063, 46.98904240251129494, -13.82790121914899117 ) ) ;
#917=CARTESIAN_POINT ( 'NONE',  ( -238.4067589809705794, 28.96627169325315165, 28.96627169325329731 ) ) ;
#919=AXIS2_PLACEMENT_3D ( 'NONE', #13697, #7318, #23809 ) ;
#920=CARTESIAN_POINT ( 'NONE',  ( -100.7734535825088500, 44.31723036834890905, 12.25131212657507795 ) ) ;
#921=CARTESIAN_POINT ( 'NONE',  ( -16.87994666138489208, -42.52193590801358170, -12.91133298919152139 ) ) ;
#922=ORIENTED_EDGE ( 'NONE', *, *, #11815, .T. ) ;
#923=CARTESIAN_POINT ( 'NONE',  ( -188.8842190493880651, -43.30124183641380142, 17.93596163623971407 ) ) ;
#924=B_SPLINE_CURVE_WITH_KNOTS ( 'NONE', 3,
 ( #606, #10717, #18826, #24964, #6711, #14825 ),
 .UNSPECIFIED., .F., .F.,
 ( 4, 2, 4 ),
 ( 0.0002283555316178395036, 0.004316741542439621673, 0.008405127553261403789 ),
 .UNSPECIFIED. ) ;
#926=CARTESIAN_POINT ( 'NONE',  ( 27.79909650602726856, -13.47302921521705699, 45.20561170653579097 ) ) ;
#927=CARTESIAN_POINT ( 'NONE',  ( 192.4448373802101173, 19.99999999996065014, -40.00000000000002132 ) ) ;
#928=CARTESIAN_POINT ( 'NONE',  ( 67.90397382965308282, 10.29861769495212798, -30.27708616508716233 ) ) ;
#931=CARTESIAN_POINT ( 'NONE',  ( 136.1360204305621551, -31.79587985999279454, 24.77266263493094911 ) ) ;
#932=CARTESIAN_POINT ( 'NONE',  ( 57.59792236341149163, -40.00000000000014211, 37.56421063658172699 ) ) ;
#933=CARTESIAN_POINT ( 'NONE',  ( 0.2972598230769957217, -4.999556039334937811E-14, 14.33493731733933352 ) ) ;
#934=CARTESIAN_POINT ( 'NONE',  ( -99.21568817060989431, 16.03295912088713848, -16.03295912088698927 ) ) ;
#935=CARTESIAN_POINT ( 'NONE',  ( 146.6084372240433709, 34.62501878078307982, -40.00000000000002132 ) ) ;
#936=CARTESIAN_POINT ( 'NONE',  ( 23.49666234703804690, -23.31470603676250164, -42.81942870555072744 ) ) ;
#938=CARTESIAN_POINT ( 'NONE',  ( 184.8905102610680444, 20.92133201514447194, 40.00000000000002132 ) ) ;
#939=CARTESIAN_POINT ( 'NONE',  ( 4.995406935893287326, 17.50105314357170627, 39.06748935135200895 ) ) ;
#940=CARTESIAN_POINT ( 'NONE',  ( -208.1127848780264742, 40.00000000000055422, -55.00245453014380814 ) ) ;
#942=CARTESIAN_POINT ( 'NONE',  ( 91.82158438592159655, -39.99999999999976552, -22.79471317813512599 ) ) ;
#944=EDGE_CURVE ( 'NONE', #14912, #4726, #12582, .T. ) ;
#945=CARTESIAN_POINT ( 'NONE',  ( 141.7942202792037563, -30.38864012024685479, -12.58738687988142857 ) ) ;
#947=CARTESIAN_POINT ( 'NONE',  ( 184.8905102610680444, -13.49065550809810965, 13.49065550809799596 ) ) ;
#949=CARTESIAN_POINT ( 'NONE',  ( -87.04503123322959368, 18.12276621389070286, -11.46092073712416060 ) ) ;
#950=CARTESIAN_POINT ( 'NONE',  ( -4.558244102846366275, 46.81081390833239197, -13.79151199599547439 ) ) ;
#952=CARTESIAN_POINT ( 'NONE',  ( -100.7734535825088500, 22.67402823373189946, 40.00000000000002132 ) ) ;
#954=CARTESIAN_POINT ( 'NONE',  ( -114.7539998840377962, 2.778767434142399573, -21.97438023164994192 ) ) ;
#957=ORIENTED_EDGE ( 'NONE', *, *, #6304, .F. ) ;
#959=CARTESIAN_POINT ( 'NONE',  ( 35.93675087521947376, -12.87543817712692729, 42.26938917674299034 ) ) ;
#960=CARTESIAN_POINT ( 'NONE',  ( 132.4338126186515581, 12.33615677966353452, -29.78211700502412285 ) ) ;
#961=VERTEX_POINT ( 'NONE', #7078 ) ;
#962=ORIENTED_EDGE ( 'NONE', *, *, #25597, .T. ) ;
#966=CARTESIAN_POINT ( 'NONE',  ( -91.56559293963834989, -44.31723036834903695, 12.25131212657476709 ) ) ;
#967=CARTESIAN_POINT ( 'NONE',  ( 130.8568914410475372, -24.07718906447222551, -24.07718906447233209 ) ) ;
#968=CARTESIAN_POINT ( 'NONE',  ( -208.1127848780264742, 39.99999999999979394, 55.00245453010936103 ) ) ;
#969=CARTESIAN_POINT ( 'NONE',  ( -199.9999999999999432, -45.65206365911544850, 19.98641303047035223 ) ) ;
#970=EDGE_CURVE ( 'NONE', #17072, #2955, #7897, .T. ) ;
#972=CARTESIAN_POINT ( 'NONE',  ( -238.4067589809705794, -39.99999999999963762, -40.96449428006383187 ) ) ;
#973=CARTESIAN_POINT ( 'NONE',  ( -100.7734535825088500, 40.00000000000017764, -17.32597176626768487 ) ) ;
#974=DIRECTION ( 'NONE',  ( 0.9352143323239811012, 0.1355013636757285422, 0.3271292299043733198 ) ) ;
#975=CARTESIAN_POINT ( 'NONE',  ( -200.0000000000000284, 19.96680831879919538, -45.63305559644798137 ) ) ;
#976=CARTESIAN_POINT ( 'NONE',  ( 192.4448373802100889, 14.14213562375893574, -14.14213562375874922 ) ) ;
#977=CARTESIAN_POINT ( 'NONE',  ( -88.39148973765020401, 8.027153355909049992, 20.15708830332377133 ) ) ;
#980=FACE_OUTER_BOUND ( 'NONE', #4167, .T. ) ;
#981=CARTESIAN_POINT ( 'NONE',  ( -91.56559293963834989, -40.53558337403692491, 16.03295912088671571 ) ) ;
#982=CARTESIAN_POINT ( 'NONE',  ( -184.9730489278823882, -22.80026000644736328, -42.02334742172997295 ) ) ;
#985=CARTESIAN_POINT ( 'NONE',  ( 170.2234770963711128, 10.92277846919147066, 45.64576402573197811 ) ) ;
#986=CARTESIAN_POINT ( 'NONE',  ( 23.37394308801977871, -23.33966569535098046, 42.85717664514577763 ) ) ;
#988=ORIENTED_EDGE ( 'NONE', *, *, #20698, .F. ) ;
#989=CARTESIAN_POINT ( 'NONE',  ( 130.8568914410475088, -39.99999999999992895, -5.949712681207114606 ) ) ;
#991=CARTESIAN_POINT ( 'NONE',  ( -199.9999999999999432, 4.865628651907057289, -55.16984130226895644 ) ) ;
#994=ORIENTED_EDGE ( 'NONE', *, *, #17258, .F. ) ;
#995=CARTESIAN_POINT ( 'NONE',  ( -238.4067589809705794, 40.96449428006337001, -40.00000000000002132 ) ) ;
#998=CARTESIAN_POINT ( 'NONE',  ( -77.58523997990643295, -17.50224656896021003, 13.57278374160384260 ) ) ;
#999=CARTESIAN_POINT ( 'NONE',  ( -208.1127848780265026, -9.061048840815752106E-14, 15.00245453012669472 ) ) ;
#1002=CARTESIAN_POINT ( 'NONE',  ( 170.2234770963711128, -17.36149277827010096, 17.36149277826970660 ) ) ;
#1005=CARTESIAN_POINT ( 'NONE',  ( -238.4067589809705794, 3.877349844572403567E-13, -40.96449427998260973 ) ) ;
#1006=CARTESIAN_POINT ( 'NONE',  ( -99.29480781227053399, -8.165122821357890359, 20.80016781325164388 ) ) ;
#1007=CARTESIAN_POINT ( 'NONE',  ( 146.6084372240433709, 34.62501878078307982, -40.00000000000002132 ) ) ;
#1008=CARTESIAN_POINT ( 'NONE',  ( -162.0762913951020892, -29.48230308784785692, 29.48230308784751230 ) ) ;
#1009=CARTESIAN_POINT ( 'NONE',  ( 0.2972598230769983307, -14.33493731733933352, 0.000000000000000000 ) ) ;
#1011=CARTESIAN_POINT ( 'NONE',  ( 14.38125909742180220, 39.99999999999997158, 15.17850393972647716 ) ) ;
#1012=CARTESIAN_POINT ( 'NONE',  ( 163.1118516004056573, -27.26290988616869626, 0.000000000000000000 ) ) ;
#1013=CARTESIAN_POINT ( 'NONE',  ( -208.1127848780264742, -17.67593391476659548, 38.89260858015730804 ) ) ;
#1014=CARTESIAN_POINT ( 'NONE',  ( -280.0000000000000568, -20.00000000000006750, 40.00000000000002132 ) ) ;
#1016=ADVANCED_FACE ( 'NONE', ( #17315 ), #3265, .T. ) ;
#1017=CARTESIAN_POINT ( 'NONE',  ( 5.823571940253325252, -49.16771748718758062, 14.15488761397359418 ) ) ;
#1018=CARTESIAN_POINT ( 'NONE',  ( -91.56559293963834989, 17.32597176626809699, -40.00000000000002132 ) ) ;
#1020=EDGE_CURVE ( 'NONE', #4727, #14641, #4162, .T. ) ;
#1021=CARTESIAN_POINT ( 'NONE',  ( -238.4067589809705794, 0.6820004457340470561, 57.25054294065803617 ) ) ;
#1022=CARTESIAN_POINT ( 'NONE',  ( 192.4448373802100889, 1.051811698935164031E-13, -20.00000000003942091 ) ) ;
#1023=CARTESIAN_POINT ( 'NONE',  ( -82.25099254137421667, 19.89874485163253581, 3.429530458953132133 ) ) ;
#1024=EDGE_CURVE ( 'NONE', #19288, #5841, #13481, .T. ) ;
#1026=CARTESIAN_POINT ( 'NONE',  ( -3.071327051952971399, -13.87830843099562728, -47.32824404903816173 ) ) ;
#1028=CARTESIAN_POINT ( 'NONE',  ( 200.0000000000000000, 14.14213562373041455, 42.42640687119311593 ) ) ;
#1029=CARTESIAN_POINT ( 'NONE',  ( -82.25678930352327711, -4.084640388374164210, -19.77202877180203089 ) ) ;
#1030=CARTESIAN_POINT ( 'NONE',  ( 160.7895100360958622, -28.48799984206438296, 0.000000000000000000 ) ) ;
#1031=CARTESIAN_POINT ( 'NONE',  ( 199.9999999999999432, -1.727494763561684666E-13, 20.00000000000010303 ) ) ;
#1032=CARTESIAN_POINT ( 'NONE',  ( -198.0356074513804572, 17.40982414986446969, 39.15871834505921356 ) ) ;
#1033=CARTESIAN_POINT ( 'NONE',  ( -82.24857225179439979, 11.87278284862390976, -16.34324723835692694 ) ) ;
#1034=CARTESIAN_POINT ( 'NONE',  ( -105.3755690713226727, 15.38646221621771737, 15.38646221621800514 ) ) ;
#1035=CARTESIAN_POINT ( 'NONE',  ( -198.9233928135151928, 14.16707757974149828, -49.24835219441582979 ) ) ;
#1036=CARTESIAN_POINT ( 'NONE',  ( 163.1118516004056573, -47.56205970284945295, -9.006482792074823607 ) ) ;
#1037=CARTESIAN_POINT ( 'NONE',  ( 19.06497207195981147, 38.31983398719673772, -38.31983398719579981 ) ) ;
#1038=CARTESIAN_POINT ( 'NONE',  ( -86.96347745069644475, -21.75974354311652093, -40.00000000000002132 ) ) ;
#1039=CARTESIAN_POINT ( 'NONE',  ( -192.9588430854689989, 10.23066800230742679, 10.23066800230749607 ) ) ;
#1040=CARTESIAN_POINT ( 'NONE',  ( -198.0356074513804572, -9.007331120208026888E-14, 15.37879056873070560 ) ) ;
#1041=CARTESIAN_POINT ( 'NONE',  ( -100.7734535825088500, -40.53558337403692491, 16.03295912088671571 ) ) ;
#1042=CARTESIAN_POINT ( 'NONE',  ( -144.1957000271909806, 30.13184844835543075, -12.48102028634719396 ) ) ;
#1043=ORIENTED_EDGE ( 'NONE', *, *, #3287, .F. ) ;
#1044=CARTESIAN_POINT ( 'NONE',  ( 146.6084372240433993, 3.800685668858676980, 3.800685668858667210 ) ) ;
#1046=CARTESIAN_POINT ( 'NONE',  ( -4.039451493210490796, 46.99046209229823745, -13.82811171175438147 ) ) ;
#1047=CARTESIAN_POINT ( 'NONE',  ( 17.24092899311760263, 18.36647614518702198, 44.34059580268282730 ) ) ;
#1048=CARTESIAN_POINT ( 'NONE',  ( -62.69292774209023378, -24.97541154601726632, -11.76166271901563576 ) ) ;
#1050=CARTESIAN_POINT ( 'NONE',  ( -173.7925187075031204, -38.69492115326026038, 20.60915802515858886 ) ) ;
#1052=CARTESIAN_POINT ( 'NONE',  ( 23.84827734669584487, -23.24317830786080208, 42.71123329578262684 ) ) ;
#1054=CARTESIAN_POINT ( 'NONE',  ( 98.29820294267322822, 7.653668647304298744, -18.47759065023114999 ) ) ;
#1056=CARTESIAN_POINT ( 'NONE',  ( -259.2033419157646676, -21.55415060305872998, 35.01439189186525880 ) ) ;
#1057=CARTESIAN_POINT ( 'NONE',  ( 0.2972598230769883387, 39.99999999999997158, 14.33493731733947563 ) ) ;
#1058=CARTESIAN_POINT ( 'NONE',  ( 130.8568914410475372, 1.429239637432775288E-13, -34.05028731879788495 ) ) ;
#1060=CARTESIAN_POINT ( 'NONE',  ( -259.2033419157646676, -30.48217210827744239, -2.449293598294708485E-15 ) ) ;
#1061=CARTESIAN_POINT ( 'NONE',  ( 27.55177309528516361, -13.49150912998400287, -45.29548561696848452 ) ) ;
#1062=CARTESIAN_POINT ( 'NONE',  ( -86.96347745069644475, 15.38646221621793586, -15.38646221621778842 ) ) ;
#1063=CARTESIAN_POINT ( 'NONE',  ( -162.0762913951020607, -41.69427287692683848, 40.00000000000002132 ) ) ;
#1064=CARTESIAN_POINT ( 'NONE',  ( 184.8905102610680444, 43.07788698682572459, 13.49065550809829439 ) ) ;
#1065=CARTESIAN_POINT ( 'NONE',  ( -192.9588430854690273, 40.00000000000055422, -54.46834944101679810 ) ) ;
#1067=CARTESIAN_POINT ( 'NONE',  ( -280.0000000000000568, -39.99999999999987210, -20.00000000000043343 ) ) ;
#1068=CARTESIAN_POINT ( 'NONE',  ( 144.1614306663417722, -30.21666801910898315, -12.51615370324033272 ) ) ;
#1070=CARTESIAN_POINT ( 'NONE',  ( 146.6084372240433709, 24.48358557860311180, 32.08495691632071356 ) ) ;
#1071=ORIENTED_EDGE ( 'NONE', *, *, #14110, .F. ) ;
#1072=CARTESIAN_POINT ( 'NONE',  ( -86.86493150571116928, 19.60045294882758071, -8.366608963953975575 ) ) ;
#1073=CARTESIAN_POINT ( 'NONE',  ( 12.96694272559474648, 44.79869582453754617, -24.77464205076245207 ) ) ;
#1074=CARTESIAN_POINT ( 'NONE',  ( -198.0356074513804572, -15.37879056873074290, 40.00000000000002132 ) ) ;
#1078=VERTEX_POINT ( 'NONE', #6512 ) ;
#1080=CARTESIAN_POINT ( 'NONE',  ( -105.3755690713226727, 15.38646221621793231, -15.38646221621779020 ) ) ;
#1082=CARTESIAN_POINT ( 'NONE',  ( 165.3321726438082351, 1.230175059844345975E-13, -26.53500608755492252 ) ) ;
#1083=ORIENTED_EDGE ( 'NONE', *, *, #23767, .F. ) ;
#1088=CARTESIAN_POINT ( 'NONE',  ( 136.1360204305621551, -53.05693388239313890, 3.511608612530593199 ) ) ;
#1090=CARTESIAN_POINT ( 'NONE',  ( 146.6084372240433993, 1.478241399363601114E-13, -34.62501878078305850 ) ) ;
#1092=CARTESIAN_POINT ( 'NONE',  ( 130.8568914410475088, -40.00000000000036238, 34.05028731879746573 ) ) ;
#1093=CARTESIAN_POINT ( 'NONE',  ( 57.59792236341147742, 4.064940816252731242E-13, -37.56421063658186199 ) ) ;
#1095=CARTESIAN_POINT ( 'NONE',  ( -280.0000000000000568, -42.42640687119285303, -14.14213562373118371 ) ) ;
#1096=CARTESIAN_POINT ( 'NONE',  ( -77.90255099906767100, 8.064892378658102601, -20.29001641120677846 ) ) ;
#1097=CARTESIAN_POINT ( 'NONE',  ( -213.1075012329537230, -9.698598906450557777, 9.698598906450415669 ) ) ;
#1098=CARTESIAN_POINT ( 'NONE',  ( 126.3230993689412571, 28.30579214049041070, 11.72464299830500067 ) ) ;
#1101=CARTESIAN_POINT ( 'NONE',  ( -77.58512834293978244, -17.50146741023962349, 13.57440574222109397 ) ) ;
#1102=CARTESIAN_POINT ( 'NONE',  ( 192.4448373802101173, -14.14213562375886291, 42.42640687116498555 ) ) ;
#1104=AXIS2_PLACEMENT_3D ( 'NONE', #14806, #22938, #4718 ) ;
#1105=CARTESIAN_POINT ( 'NONE',  ( -259.2033419157646676, -49.83842185052040463, 6.730120644403092101 ) ) ;
#1106=CARTESIAN_POINT ( 'NONE',  ( -187.8779108535657372, -17.82355704115960648, -43.02987313851341611 ) ) ;
#1108=EDGE_LOOP ( 'NONE', ( #7564, #21544, #5228, #9146 ) ) ;
#1109=CARTESIAN_POINT ( 'NONE',  ( -30.26275506840324070, 1.198031551616724366, -57.76657404653984429 ) ) ;
#1111=CARTESIAN_POINT ( 'NONE',  ( 169.9999999999674571, -17.64300463372919836, -17.64300463252165585 ) ) ;
#1114=CARTESIAN_POINT ( 'NONE',  ( -56.48582580120559271, -1.062504017861011783E-13, 9.153146818113587102 ) ) ;
#1115=CARTESIAN_POINT ( 'NONE',  ( -3.555049149807529396, -23.55301256057176573, 43.14507846637736321 ) ) ;
#1117=CIRCLE ( 'NONE', #11762, 60.00000000000000000 ) ;
#1120=CARTESIAN_POINT ( 'NONE',  ( 170.2234770963711128, 15.44714144992819094, 2.449293598294708485E-15 ) ) ;
#1124=CARTESIAN_POINT ( 'NONE',  ( -56.48582580120559271, 6.472252184284211118, -6.472252184284153387 ) ) ;
#1125=CARTESIAN_POINT ( 'NONE',  ( -86.96347745069645896, 40.00000000000008527, -21.75974354311636461 ) ) ;
#1128=ADVANCED_FACE ( 'NONE', ( #14498 ), #20591, .T. ) ;
#1129=AXIS2_PLACEMENT_3D ( 'NONE', #12944, #974, #3215 ) ;
#1130=CARTESIAN_POINT ( 'NONE',  ( -199.9999999999999432, 43.68705981750494516, 18.09577267661451927 ) ) ;
#1131=CARTESIAN_POINT ( 'NONE',  ( -100.7734535825088358, 6.065416334915073333E-14, -22.67402823373191723 ) ) ;
#1133=AXIS2_PLACEMENT_3D ( 'NONE', #3305, #1186, #21785 ) ;
#1135=CARTESIAN_POINT ( 'NONE',  ( -24.88648382749666155, -19.35593139216429037, -36.77569126519823328 ) ) ;
#1136=CARTESIAN_POINT ( 'NONE',  ( -238.4067589809705794, -0.6820004457337348613, -57.25054294065803617 ) ) ;
#1137=CARTESIAN_POINT ( 'NONE',  ( -97.74230697482651919, 20.71358501227901883, 8.579847837454130044 ) ) ;
#1138=CARTESIAN_POINT ( 'NONE',  ( -238.4067589809705794, -39.99999999999963762, -40.96449428006383187 ) ) ;
#1140=CARTESIAN_POINT ( 'NONE',  ( 146.6084372240433709, -5.374981219216942385, -40.00000000000002132 ) ) ;
#1141=CARTESIAN_POINT ( 'NONE',  ( -30.26275506840325136, 27.08623969584573388, 29.48230279907808793 ) ) ;
#1142=CARTESIAN_POINT ( 'NONE',  ( 151.7948205124835681, 33.23291073765556547, -40.00000000000002132 ) ) ;
#1143=CARTESIAN_POINT ( 'NONE',  ( 98.29820294272737158, 10.21753654889138652, 17.41560179325824009 ) ) ;
#1144=CARTESIAN_POINT ( 'NONE',  ( 170.2234770963711128, 40.00000000000014211, -24.55285855007172913 ) ) ;
#1147=CARTESIAN_POINT ( 'NONE',  ( -105.3755690713226727, 12.89780903124400879, 12.89780903124407452 ) ) ;
#1148=CARTESIAN_POINT ( 'NONE',  ( 4.995406935893288214, 55.24977328854835434, 2.449293598294708485E-15 ) ) ;
#1149=ORIENTED_EDGE ( 'NONE', *, *, #9291, .F. ) ;
#1150=CARTESIAN_POINT ( 'NONE',  ( 23.17367289775286210, -42.91822977676378770, 23.38495170326197226 ) ) ;
#1151=CARTESIAN_POINT ( 'NONE',  ( -105.4741150117365009, 19.60045294981777531, -8.366608964619008049 ) ) ;
#1153=CARTESIAN_POINT ( 'NONE',  ( -192.9588430854689989, 38.51493924976929861, 38.51493924976947625 ) ) ;
#1154=CARTESIAN_POINT ( 'NONE',  ( -259.2033419157646676, -1.438356298054549103E-14, -9.517827891722632216 ) ) ;
#1155=CARTESIAN_POINT ( 'NONE',  ( -77.55800104386271698, 22.12266577817424817, 0.9110312510734462910 ) ) ;
#1156=CARTESIAN_POINT ( 'NONE',  ( 20.59573805978978811, -13.93986955483911849, -47.74081960064690833 ) ) ;
#1159=CARTESIAN_POINT ( 'NONE',  ( -82.23866184897889298, 1.260276691160380436, -20.16530832601847933 ) ) ;
#1160=CARTESIAN_POINT ( 'NONE',  ( -192.9588430854690273, 38.51493924976913519, 18.05360324515490333 ) ) ;
#1161=CARTESIAN_POINT ( 'NONE',  ( 192.4448373802101173, 14.14213562375922884, -42.42640687116488607 ) ) ;
#1162=EDGE_CURVE ( 'NONE', #1634, #13223, #20018, .T. ) ;
#1163=CARTESIAN_POINT ( 'NONE',  ( 91.82158438592156813, 40.45024623143950038, 16.11829626348447420 ) ) ;
#1165=CARTESIAN_POINT ( 'NONE',  ( -280.0000000000000568, 14.14213562373127431, -42.42640687119274645 ) ) ;
#1166=CARTESIAN_POINT ( 'NONE',  ( 0.2972598230770048811, -10.13633138497415942, -66.70487387989865624 ) ) ;
#1167=CARTESIAN_POINT ( 'NONE',  ( -91.56559293963834989, -16.03295912088659492, -40.53558337403696044 ) ) ;
#1168=CARTESIAN_POINT ( 'NONE',  ( 163.1118516004056573, 37.29075403953132906, 19.27778845539275565 ) ) ;
#1169=CARTESIAN_POINT ( 'NONE',  ( 130.8568914410475088, -34.05028731879786363, -40.00000000000002132 ) ) ;
#1170=CARTESIAN_POINT ( 'NONE',  ( 130.8568914410475372, 34.05028731879791337, 0.000000000000000000 ) ) ;
#1171=VECTOR ( 'NONE', #14693, 1000.000000000000114 ) ;
#1173=CARTESIAN_POINT ( 'NONE',  ( 0.2972598230770153171, -66.70487387989849992, -10.13633138497533004 ) ) ;
#1174=CARTESIAN_POINT ( 'NONE',  ( -173.7925187078953115, 41.93431653924884017, -12.78856575083363722 ) ) ;
#1175=ORIENTED_EDGE ( 'NONE', *, *, #25415, .F. ) ;
#1176=CARTESIAN_POINT ( 'NONE',  ( 136.1360204305621551, 31.79587985999267374, -24.77266263493117293 ) ) ;
#1178=CARTESIAN_POINT ( 'NONE',  ( 23.17367289775146943, 23.38495170326214989, 42.91822977676415718 ) ) ;
#1179=CARTESIAN_POINT ( 'NONE',  ( -87.08870976744167081, -21.20092391029482926, 3.405966936733633155 ) ) ;
#1181=CARTESIAN_POINT ( 'NONE',  ( -105.2527671768314548, 17.45248019613228863, 12.50784186996179059 ) ) ;
#1183=CARTESIAN_POINT ( 'NONE',  ( 22.92196489052106401, -23.44087486047334323, 42.99364193793560673 ) ) ;
#1186=DIRECTION ( 'NONE',  ( 1.000000000000000000, 1.836970198721025990E-16, 0.000000000000000000 ) ) ;
#1187=CARTESIAN_POINT ( 'NONE',  ( -192.9588430854690273, 39.99999999999992895, 14.46834944099983922 ) ) ;
#1189=EDGE_CURVE ( 'NONE', #23238, #6963, #17697, .T. ) ;
#1191=CARTESIAN_POINT ( 'NONE',  ( -135.8532207217289738, -30.84685318188647685, -2.449293598294708485E-15 ) ) ;
#1192=CARTESIAN_POINT ( 'NONE',  ( 60.14720761601253685, -15.75494750867305704, -31.22869220293659609 ) ) ;
#1194=EDGE_CURVE ( 'NONE', #8799, #7462, #15578, .T. ) ;
#1195=CARTESIAN_POINT ( 'NONE',  ( 136.1360204305621551, -4.966164525587043244, 40.00000000000002132 ) ) ;
#1196=FACE_OUTER_BOUND ( 'NONE', #11209, .T. ) ;
#1197=CARTESIAN_POINT ( 'NONE',  ( 136.1360204305621551, 40.00000000000009948, -4.966164525586641787 ) ) ;
#1198=CARTESIAN_POINT ( 'NONE',  ( 170.2234770963711128, -40.00000000000024158, 24.55285855007145202 ) ) ;
#1199=CARTESIAN_POINT ( 'NONE',  ( 156.5534228368365177, -27.23630265682181673, -11.28164594935398668 ) ) ;
#1201=EDGE_CURVE ( 'NONE', #20449, #5206, #6685, .T. ) ;
#1204=CARTESIAN_POINT ( 'NONE',  ( -4.027137536849638266, 43.00884733904534585, -23.45200847982327730 ) ) ;
#1205=CARTESIAN_POINT ( 'NONE',  ( -213.1075012329537230, -13.71589010951915810, 40.00000000000002132 ) ) ;
#1207=CARTESIAN_POINT ( 'NONE',  ( -192.9370391625991772, 44.11033075278052706, -24.26711063095028109 ) ) ;
#1209=VERTEX_POINT ( 'NONE', #25254 ) ;
#1210=ORIENTED_EDGE ( 'NONE', *, *, #56, .F. ) ;
#1211=CARTESIAN_POINT ( 'NONE',  ( 146.6084372240433993, 24.48358557860341733, -24.48358557860313311 ) ) ;
#1212=DIRECTION ( 'NONE',  ( 0.000000000000000000, 1.000000000000000000, 0.000000000000000000 ) ) ;
#1216=CARTESIAN_POINT ( 'NONE',  ( -199.9999999999999432, 14.17215463606929227, 49.28189405767592746 ) ) ;
#1217=CARTESIAN_POINT ( 'NONE',  ( 57.59792236341147031, 26.56190807104684382, 26.56190807104692553 ) ) ;
#1219=CARTESIAN_POINT ( 'NONE',  ( -100.7734535825088358, 6.065416334915073333E-14, -22.67402823373191723 ) ) ;
#1221=CARTESIAN_POINT ( 'NONE',  ( 98.29820294267867098, 17.44908643998556741, 10.13669746063099275 ) ) ;
#1222=CARTESIAN_POINT ( 'NONE',  ( -259.2033419157646676, -40.00000000000017053, 9.517827891722212996 ) ) ;
#1223=CARTESIAN_POINT ( 'NONE',  ( -213.1075012329537230, 5.259461644596141978E-13, -53.71589010951915100 ) ) ;
#1224=CARTESIAN_POINT ( 'NONE',  ( -110.0904723790854689, -16.34339323353421136, 11.87257855583943922 ) ) ;
#1225=CARTESIAN_POINT ( 'NONE',  ( -105.3755690713226727, 15.38646221621793231, -15.38646221621779020 ) ) ;
#1226=CARTESIAN_POINT ( 'NONE',  ( 14.38125909742181108, -5.035366881890652543E-14, 15.17850393972633682 ) ) ;
#1227=CARTESIAN_POINT ( 'NONE',  ( 19.06497207195981147, -10.03556273973439517, 10.03556273973429214 ) ) ;
#1228=CARTESIAN_POINT ( 'NONE',  ( 132.4338126186516718, 29.78211700502412995, 12.33615677966351676 ) ) ;
#1230=CARTESIAN_POINT ( 'NONE',  ( -77.70896657118139217, 18.93513500903836899, -11.20032855621326995 ) ) ;
#1231=CARTESIAN_POINT ( 'NONE',  ( 184.8905102610680444, 14.79361573936396113, -14.79361573936377461 ) ) ;
#1232=CARTESIAN_POINT ( 'NONE',  ( -87.04313178897470493, -18.12206666836609159, 11.44454159255920445 ) ) ;
#1233=CARTESIAN_POINT ( 'NONE',  ( 136.1360204305621551, -53.05693388239313890, 3.511608612530593199 ) ) ;
#1234=CARTESIAN_POINT ( 'NONE',  ( -86.96347745069644475, -12.89780903124395195, -12.89780903124416511 ) ) ;
#1235=CARTESIAN_POINT ( 'NONE',  ( -174.2682069747397975, -16.26528465553820268, -39.26787081120916412 ) ) ;
#1236=CARTESIAN_POINT ( 'NONE',  ( -77.55640685876514340, 14.66025428152425469, 16.63820105393991611 ) ) ;
#1238=CARTESIAN_POINT ( 'NONE',  ( 57.59792236341147031, 54.84617931850878136, 1.722363176415705910 ) ) ;
#1244=CARTESIAN_POINT ( 'NONE',  ( 12.01676469546555559, -44.88780742856556571, 24.84032989753427501 ) ) ;
#1247=CARTESIAN_POINT ( 'NONE',  ( -192.9588430854690273, -38.51493924976932703, -18.05360324515463688 ) ) ;
#1248=CARTESIAN_POINT ( 'NONE',  ( -238.4067589809705794, 39.99999999999997158, 0.9644942799827220803 ) ) ;
#1249=CARTESIAN_POINT ( 'NONE',  ( -93.01854144614549114, -20.65013722621582914, -8.553566904110464719 ) ) ;
#1252=CARTESIAN_POINT ( 'NONE',  ( -213.1075012329537230, -40.00000000000011369, 13.71589010951897691 ) ) ;
#1254=CARTESIAN_POINT ( 'NONE',  ( -77.70092540962068028, 11.20694785794322179, 18.98758604048486731 ) ) ;
#1255=CARTESIAN_POINT ( 'NONE',  ( -39.84211263226702471, -13.56589830548555398, -32.75097567531932441 ) ) ;
#1256=CARTESIAN_POINT ( 'NONE',  ( 170.2234770963711128, 45.64576402573196390, -10.92277846919159856 ) ) ;
#1258=CARTESIAN_POINT ( 'NONE',  ( 170.2234770963711128, 40.00000000000021316, -15.44714144992773797 ) ) ;
#1259=CARTESIAN_POINT ( 'NONE',  ( 170.0000000000000000, -24.95097643316998415, 3.062538285713072295 ) ) ;
#1260=CARTESIAN_POINT ( 'NONE',  ( -56.48582580120559271, 9.153146818113576444, -0.000000000000000000 ) ) ;
#1261=CARTESIAN_POINT ( 'NONE',  ( 192.4448373802100889, 20.00000000003945644, 0.000000000000000000 ) ) ;
#1262=CARTESIAN_POINT ( 'NONE',  ( 91.82158438592156813, 40.45024623143950038, 16.11829626348447420 ) ) ;
#1263=CARTESIAN_POINT ( 'NONE',  ( -86.96347745069645896, 21.75974354311648895, -40.00000000000002132 ) ) ;
#1264=EDGE_CURVE ( 'NONE', #11892, #19940, #5795, .T. ) ;
#1265=CARTESIAN_POINT ( 'NONE',  ( -1.255560987024270991, -43.73013506549190765, -23.98612781107773984 ) ) ;
#1267=CARTESIAN_POINT ( 'NONE',  ( -105.3755690713226727, -2.472783935621397949E-13, 21.75974354311649961 ) ) ;
#1268=CARTESIAN_POINT ( 'NONE',  ( 151.7948205124836534, 33.06932595376365924, -23.49921654116018743 ) ) ;
#1269=CARTESIAN_POINT ( 'NONE',  ( 192.4448373802100889, 19.99999999996064304, 2.449293598294708485E-15 ) ) ;
#1270=EDGE_LOOP ( 'NONE', ( #6729, #18877, #7061, #15213, #21211, #293, #7924 ) ) ;
#1271=CARTESIAN_POINT ( 'NONE',  ( 23.46661716383116669, -42.82867125331067371, 23.32081713244396681 ) ) ;
#1272=CARTESIAN_POINT ( 'NONE',  ( 170.0000000000427178, -17.64300463311358769, 17.64300463311318268 ) ) ;
#1273=CARTESIAN_POINT ( 'NONE',  ( 151.7948205124836534, -51.78348778862535795, 4.785054706298367044 ) ) ;
#1275=CARTESIAN_POINT ( 'NONE',  ( -77.93819491933658128, 20.10517996227020987, 8.440354353651857267 ) ) ;
#1276=CARTESIAN_POINT ( 'NONE',  ( 17.75917311731580739, -14.04884443869862487, -48.46615948699207621 ) ) ;
#1279=FACE_OUTER_BOUND ( 'NONE', #20923, .T. ) ;
#1280=CARTESIAN_POINT ( 'NONE',  ( -100.7734535825088358, -16.03295912088728770, 16.03295912088687913 ) ) ;
#1281=CARTESIAN_POINT ( 'NONE',  ( 19.06497207195980792, 18.24870850772790831, -38.31983398719609824 ) ) ;
#1283=CARTESIAN_POINT ( 'NONE',  ( -77.78698591354267933, -20.89067208891385974, -6.810288896245590529 ) ) ;
#1285=CARTESIAN_POINT ( 'NONE',  ( -30.26275506840323359, -1.198031551615522439, -57.76657404653986561 ) ) ;
#1286=CARTESIAN_POINT ( 'NONE',  ( -259.2033419157646676, -21.55415060305824326, -21.55415060305857367 ) ) ;
#1287=CARTESIAN_POINT ( 'NONE',  ( -208.1127848780264742, 10.60833733268383483, -67.17687982760675425 ) ) ;
#1288=CARTESIAN_POINT ( 'NONE',  ( -56.48582580120559982, 50.09629031063956717, 6.472252184284792875 ) ) ;
#1289=CARTESIAN_POINT ( 'NONE',  ( -105.2054292635175017, -14.23158570603253459, 16.16441072137211066 ) ) ;
#1291=( BOUNDED_CURVE ( )  B_SPLINE_CURVE ( 3, ( #7283, #11398, #21403, #15399 ),
 .UNSPECIFIED., .F., .F. ) 
 B_SPLINE_CURVE_WITH_KNOTS ( ( 4, 4 ),
 ( 0.004183487405659152593, 0.01388163287021919670 ),
 .UNSPECIFIED. ) 
 CURVE ( )  GEOMETRIC_REPRESENTATION_ITEM ( )  RATIONAL_B_SPLINE_CURVE ( ( 0.6809743333591533609, 0.7608653435686130173, 0.8672072324488951933, 1.000000000000000000 ) ) 
 REPRESENTATION_ITEM ( '' )  );
#1292=CARTESIAN_POINT ( 'NONE',  ( 98.29820294272414571, 7.653668647302724892, 18.47759065022804137 ) ) ;
#1293=CARTESIAN_POINT ( 'NONE',  ( 192.4448373802101173, -14.14213562370342281, 42.42640687122062104 ) ) ;
#1294=CARTESIAN_POINT ( 'NONE',  ( 14.38125909742180752, 15.17850393972634038, 40.00000000000002132 ) ) ;
#1295=ORIENTED_EDGE ( 'NONE', *, *, #10302, .T. ) ;
#1296=CARTESIAN_POINT ( 'NONE',  ( -30.26275506840325136, 57.76657404653985139, 1.198031551616126178 ) ) ;
#1297=CARTESIAN_POINT ( 'NONE',  ( -87.11182023518614415, -17.01577573093364038, -13.17795446294752892 ) ) ;
#1299=CARTESIAN_POINT ( 'NONE',  ( -4.151555265633143144, -46.95165237383028511, -13.82020782288861049 ) ) ;
#1300=B_SPLINE_CURVE_WITH_KNOTS ( 'NONE', 3,
 ( #17774, #5676, #13782, #21915, #16582, #4097, #6334, #18444, #18306, #24984, #12323, #22585, #219, #92, #10469, #8332, #6211, #8734, #12197, #22712, #12591, #14188, #4363, #22321, #24844, #24714, #16852 ),
 .UNSPECIFIED., .F., .F.,
 ( 4, 2, 1, 1, 2, 2, 2, 2, 2, 2, 2, 2, 1, 2, 4 ),
 ( -6.000000000158344332E-08, 0.0002171475752860021037, 0.0004343551505720058027, 0.0008687703011440085386, 0.001737600602288021275, 0.003475261204576048698, 0.006950582409152100509, 0.01390122481830420413, 0.02085186722745631036, 0.02432718843203236087, 0.02606484903432039479, 0.02693367933546441523, 0.02736809448603642544, 0.02758530206132243576, 0.02780250963660844607 ),
 .UNSPECIFIED. ) ;
#1301=ORIENTED_EDGE ( 'NONE', *, *, #3436, .F. ) ;
#1302=CARTESIAN_POINT ( 'NONE',  ( -187.8778500559185431, -43.02985669704839466, 17.82355023088355495 ) ) ;
#1305=CARTESIAN_POINT ( 'NONE',  ( 98.29820294267315717, -7.653668647304116668, 18.47759065023120684 ) ) ;
#1308=CARTESIAN_POINT ( 'NONE',  ( -199.9999999999998010, 24.82633483071100500, -44.86878812508844305 ) ) ;
#1309=CARTESIAN_POINT ( 'NONE',  ( -135.8532207217289738, 40.00000000000002842, -9.153146818113432559 ) ) ;
#1311=CARTESIAN_POINT ( 'NONE',  ( 23.09931156284629239, 46.91113948292964864, -13.81622350327230109 ) ) ;
#1312=CARTESIAN_POINT ( 'NONE',  ( 199.9999999999999432, -19.99999999999988987, -2.449293598294708485E-15 ) ) ;
#1314=CARTESIAN_POINT ( 'NONE',  ( -183.1091233172942907, 22.43565125815459282, -41.47045062400935223 ) ) ;
#1316=CARTESIAN_POINT ( 'NONE',  ( 170.2234770963711128, -15.44714144992813409, 40.00000000000002132 ) ) ;
#1317=CARTESIAN_POINT ( 'NONE',  ( -198.0356074513804572, -15.37879056873074290, 0.000000000000000000 ) ) ;
#1319=CARTESIAN_POINT ( 'NONE',  ( 19.06497207195980792, 14.19242893257840699, 40.00000000000002132 ) ) ;
#1320=CARTESIAN_POINT ( 'NONE',  ( -100.7734535825088500, 39.99999999999976552, 22.67402823373233645 ) ) ;
#1322=CARTESIAN_POINT ( 'NONE',  ( 184.8905102610680444, -40.00000000000021316, 20.92133201514402430 ) ) ;
#1323=CARTESIAN_POINT ( 'NONE',  ( 98.93808658348716278, -18.71306740730482687, -7.751206313707100115 ) ) ;
#1324=ORIENTED_EDGE ( 'NONE', *, *, #12009, .T. ) ;
#1325=CARTESIAN_POINT ( 'NONE',  ( -86.94949953272028154, 20.30809431151143229, -6.679047987429632904 ) ) ;
#1326=CARTESIAN_POINT ( 'NONE',  ( -4.260882601030880679, 46.91379881627385373, -13.81249720866881248 ) ) ;
#1327=CARTESIAN_POINT ( 'NONE',  ( -213.1075012329537230, -53.71589010950170717, 40.00000000000002132 ) ) ;
#1329=B_SPLINE_CURVE_WITH_KNOTS ( 'NONE', 3,
 ( #21318, #7074, #19683, #19306, #11317, #969, #23682, #13073, #11071, #17180, #21189, #2961, #5332, #19557 ),
 .UNSPECIFIED., .F., .F.,
 ( 4, 2, 2, 2, 2, 2, 4 ),
 ( 1.040834085586084257E-17, 0.002941681445496978960, 0.004412522168245460417, 0.005883362890993943176, 0.008825044336490900018, 0.01029588505923937844, 0.01176672578198786033 ),
 .UNSPECIFIED. ) ;
#1330=CARTESIAN_POINT ( 'NONE',  ( -188.6013476421588564, 43.09288642756978760, -23.51433506917260630 ) ) ;
#1332=ORIENTED_EDGE ( 'NONE', *, *, #7657, .T. ) ;
#1334=FACE_OUTER_BOUND ( 'NONE', #18817, .T. ) ;
#1335=CARTESIAN_POINT ( 'NONE',  ( 164.1122551457364409, 10.10009781492438918, -24.38379312608493521 ) ) ;
#1342=CARTESIAN_POINT ( 'NONE',  ( -198.0356074513804572, 67.44298959253333692, 10.87444709760969452 ) ) ;
#1344=ADVANCED_FACE ( 'NONE', ( #18724 ), #13391, .T. ) ;
#1345=CARTESIAN_POINT ( 'NONE',  ( 170.0000000000000000, 24.95097643317003744, 0.000000000000000000 ) ) ;
#1346=CARTESIAN_POINT ( 'NONE',  ( -198.0356074513804572, -9.007331120208026888E-14, 15.37879056873070560 ) ) ;
#1347=CARTESIAN_POINT ( 'NONE',  ( -105.2276019129704991, -13.16696799169988452, -17.02331989733613327 ) ) ;
#1351=ADVANCED_FACE ( 'NONE', ( #8881 ), #18725, .T. ) ;
#1352=CARTESIAN_POINT ( 'NONE',  ( -77.90255099906853786, 8.644468104252323926, -20.04994828524279882 ) ) ;
#1353=CARTESIAN_POINT ( 'NONE',  ( -56.48582580120557850, -39.99999999999970868, -30.84685318188687120 ) ) ;
#1354=CARTESIAN_POINT ( 'NONE',  ( 184.8905102610680444, 2.362515690532070066E-13, -19.07866798485558490 ) ) ;
#1355=CARTESIAN_POINT ( 'NONE',  ( -114.6821015619795645, -12.10555619827156626, 18.42370988052079284 ) ) ;
#1356=CARTESIAN_POINT ( 'NONE',  ( 14.38125909742181818, -39.01709431150904095, -17.55144818341490165 ) ) ;
#1357=CARTESIAN_POINT ( 'NONE',  ( 151.7948205124836534, 40.00000000000017053, -33.23291073765538783 ) ) ;
#1358=CARTESIAN_POINT ( 'NONE',  ( -126.6834154283287575, 24.04426794716025739, -11.16464792285741403 ) ) ;
#1359=CARTESIAN_POINT ( 'NONE',  ( 155.1206158682454657, 27.79897307351018654, 11.51471166709261951 ) ) ;
#1360=CARTESIAN_POINT ( 'NONE',  ( -77.67292258764840085, 18.59814239105719125, -11.80983163631141863 ) ) ;
#1361=CARTESIAN_POINT ( 'NONE',  ( 170.2234770963711128, 45.64576402573181468, 10.92277846919223627 ) ) ;
#1362=CARTESIAN_POINT ( 'NONE',  ( 91.82158438592159655, -39.99999999999994316, -17.20528682183314118 ) ) ;
#1363=CARTESIAN_POINT ( 'NONE',  ( 91.82158438592158234, -12.16597498400057198, 44.40256751092329779 ) ) ;
#1365=CARTESIAN_POINT ( 'NONE',  ( -238.4067589809705794, -57.25054294077233408, -0.6820004458489551391 ) ) ;
#1367=CARTESIAN_POINT ( 'NONE',  ( 130.8568914410475372, -3.326198072800416995E-13, 34.05028731879788495 ) ) ;
#1368=ORIENTED_EDGE ( 'NONE', *, *, #8822, .F. ) ;
#1369=CARTESIAN_POINT ( 'NONE',  ( 130.8568914410475372, 4.207082182992923691, -4.207082182992794017 ) ) ;
#1372=ORIENTED_EDGE ( 'NONE', *, *, #13149, .T. ) ;
#1373=CARTESIAN_POINT ( 'NONE',  ( 200.0000000000000000, -40.00000000000019185, 19.99999999999968381 ) ) ;
#1374=CARTESIAN_POINT ( 'NONE',  ( -2.652172544013602362, -23.73409167602005354, 43.38951316025630689 ) ) ;
#1378=CARTESIAN_POINT ( 'NONE',  ( -86.96347745069645896, -12.89780903124382938, -43.67073346367985920 ) ) ;
#1379=CARTESIAN_POINT ( 'NONE',  ( -259.2033419157646676, 39.99999999999987210, 30.48217210827754542 ) ) ;
#1380=CARTESIAN_POINT ( 'NONE',  ( -114.7826396787323375, -16.63820453137681454, -14.66025082034670213 ) ) ;
#1382=CARTESIAN_POINT ( 'NONE',  ( 170.0000000000133014, 17.64300463311800016, 17.64300463311827016 ) ) ;
#1383=CARTESIAN_POINT ( 'NONE',  ( -213.1075012329537230, -2.291445344039133686E-13, 53.71589010951915100 ) ) ;
#1385=CARTESIAN_POINT ( 'NONE',  ( -105.3755690713226585, 40.00000000000007816, -21.75974354311636461 ) ) ;
#1387=CARTESIAN_POINT ( 'NONE',  ( -5.866564133085600652, -13.69896896866330849, -46.35727274689645583 ) ) ;
#1388=CARTESIAN_POINT ( 'NONE',  ( -238.4067589809705794, 27.60227080167080160, -28.96627169325299533 ) ) ;
#1390=CARTESIAN_POINT ( 'NONE',  ( 0.2972598230770103767, -39.99999999999945288, -54.33493731733979359 ) ) ;
#1391=CARTESIAN_POINT ( 'NONE',  ( 73.43468551893268170, -28.18272074650139203, -9.843145830824745701 ) ) ;
#1392=CARTESIAN_POINT ( 'NONE',  ( 163.1118516004056573, 27.26290988616876021, 40.00000000000002132 ) ) ;
#1393=CARTESIAN_POINT ( 'NONE',  ( 0.2972598230769983307, -14.33493731733933352, -40.00000000000002132 ) ) ;
#1394=CARTESIAN_POINT ( 'NONE',  ( 163.1118516004056573, 47.56205970284957374, 9.006482792074494981 ) ) ;
#1395=CARTESIAN_POINT ( 'NONE',  ( -30.26275506840324070, -1.694272468446265112, 0.000000000000000000 ) ) ;
#1396=CARTESIAN_POINT ( 'NONE',  ( 98.29820294272414571, 7.653668647302724892, 18.47759065022804137 ) ) ;
#1397=CARTESIAN_POINT ( 'NONE',  ( -86.86493150571116928, -8.366608963953867217, -19.60045294882765887 ) ) ;
#1399=CARTESIAN_POINT ( 'NONE',  ( 163.1118516004056573, 9.006482792069629539, 9.006482792069634868 ) ) ;
#1400=CARTESIAN_POINT ( 'NONE',  ( 136.1360204305621551, 4.966164525587093870, -40.00000000000002132 ) ) ;
#1402=CARTESIAN_POINT ( 'NONE',  ( 67.79414719545434309, -28.72755866870028285, 14.15005687161233361 ) ) ;
#1403=( BOUNDED_SURFACE ( )  B_SPLINE_SURFACE ( 3, 2, ( 
 ( #357, #24710, #8062 ),
 ( #14184, #6465, #14580 ),
 ( #22317, #18709, #89 ),
 ( #16178, #12587, #14714 ),
 ( #6080, #16709, #4621 ),
 ( #8461, #8198, #14318 ),
 ( #2351, #4094, #24841 ),
 ( #20717, #20316, #12194 ),
 ( #16314, #22709, #12720 ),
 ( #18172, #492, #2092 ),
 ( #12320, #24314, #14453 ),
 ( #10200, #1960, #22580 ),
 ( #18302, #4486, #24439 ),
 ( #10596, #4360, #8600 ),
 ( #6592, #6206, #22846 ),
 ( #22451, #4230, #18577 ),
 ( #2483, #10465, #10067 ),
 ( #16579, #26320, #20446 ),
 ( #2224, #10332, #216 ),
 ( #18441, #8327, #12451 ),
 ( #16451, #24575, #6331 ),
 ( #20578, #11243, #23366 ),
 ( #7124, #2621, #10735 ),
 ( #6861, #22976, #14843 ),
 ( #891, #8730, #25371 ),
 ( #16976, #19236, #9000 ),
 ( #2758, #24981, #21242 ),
 ( #5142, #21111, #1017 ),
 ( #624, #14978, #6731 ),
 ( #17230, #17105, #4753 ),
 ( #18980, #2890, #16848 ),
 ( #25237, #23112, #12859 ),
 ( #18846, #25112, #20845 ),
 ( #20977, #10861, #10998 ),
 ( #19107, #17361, #759 ),
 ( #15234, #8863, #13248 ),
 ( #4884, #6989, #9119 ),
 ( #11123, #12989, #5015 ),
 ( #23490, #9255, #15104 ),
 ( #23239, #13121, #3016 ),
 ( #21372, #3140, #19360 ),
 ( #1150, #25497, #7245 ),
 ( #15366, #5264, #9375 ),
 ( #17609, #11367, #17484 ),
 ( #13886, #1662, #25627 ),
 ( #21746, #13366, #23998 ),
 ( #7896, #13620, #23735 ),
 ( #3521, #9637, #26152 ),
 ( #5779, #3791, #11488 ),
 ( #1271, #22021, #16015 ),
 ( #7373, #1798, #24141 ),
 ( #21490, #23867, #5391 ),
 ( #11621, #25751, #19743 ),
 ( #13495, #15484, #23611 ),
 ( #9771, #3263, #9902 ),
 ( #11894, #21617, #20015 ),
 ( #3392, #25882, #7760 ),
 ( #18008, #19616, #19487 ),
 ( #1402, #26021, #9503 ),
 ( #7499, #7625, #15611 ),
 ( #5516, #1532, #17739 ),
 ( #15739, #15870, #5643 ) ),
 .UNSPECIFIED., .F., .F., .F. ) 
 B_SPLINE_SURFACE_WITH_KNOTS ( ( 4, 2, 2, 2, 2, 2, 2, 2, 2, 2, 2, 2, 2, 2, 2, 2, 2, 2, 2, 2, 2, 2, 2, 2, 2, 2, 2, 2, 2, 2, 4 ),
 ( 3, 3 ),
 ( 0.005118828937694837322, 0.02956064127319293564, 0.05400245360869103395, 0.07844426594418912879, 0.08149949248612639585, 0.08302710575709502938, 0.08379091239257935309, 0.08417281571032150800, 0.08436376736919258545, 0.08445924319862813112, 0.08450698111334589702, 0.08455471902806366291, 0.09066517211193818315, 0.09677562519581270339, 0.09983085173774997045, 0.1028860782796872375, 0.1089965313635617716, 0.1151069844474362919, 0.1181622109893735451, 0.1196898242603421786, 0.1204536308958265023, 0.1208355342135686572, 0.1208594031709275401, 0.1208832721282864231, 0.1209310100430041890, 0.1210264858724397347, 0.1212174375313108121, 0.1273278906151853462, 0.1517697029506834272, 0.1762115152861815359, 0.2006533276216796446 ),
 ( 0.000000000000000000, 1.000000000000000000 ),
 .UNSPECIFIED. ) 
 GEOMETRIC_REPRESENTATION_ITEM ( )  RATIONAL_B_SPLINE_SURFACE ( (
 ( 1.000000000000000000, 0.9997813423572990965, 1.000000000000000000),
 ( 1.000000000000000000, 0.9990919206318839008, 1.000000000000000000),
 ( 1.000000000000000000, 0.9967874177841469230, 1.000000000000000000),
 ( 1.000000000000000000, 0.9887544623280424272, 1.000000000000000000),
 ( 1.000000000000000000, 0.9830290792185782944, 1.000000000000000000),
 ( 1.000000000000000000, 0.9678345454235133261, 1.000000000000000000),
 ( 1.000000000000000000, 0.9583650305396005376, 1.000000000000000000),
 ( 1.000000000000000000, 0.9453335293272576711, 1.000000000000000000),
 ( 1.000000000000000000, 0.9438523872746900079, 1.000000000000000000),
 ( 1.000000000000000000, 0.9415799504610725679, 1.000000000000000000),
 ( 1.000000000000000000, 0.9408140170424496018, 1.000000000000000000),
 ( 1.000000000000000000, 0.9396523143998791738, 1.000000000000000000),
 ( 1.000000000000000000, 0.9392629463989451422, 1.000000000000000000),
 ( 1.000000000000000000, 0.9386756783046033004, 1.000000000000000000),
 ( 1.000000000000000000, 0.9384793862554601240, 1.000000000000000000),
 ( 1.000000000000000000, 0.9381841422087060511, 1.000000000000000000),
 ( 1.000000000000000000, 0.9380855931974548811, 1.000000000000000000),
 ( 1.000000000000000000, 0.9379375679425719925, 1.000000000000000000),
 ( 1.000000000000000000, 0.9378881925679177778, 1.000000000000000000),
 ( 1.000000000000000000, 0.9378140790407639704, 1.000000000000000000),
 ( 1.000000000000000000, 0.9377896949153107231, 1.000000000000000000),
 ( 1.000000000000000000, 0.9377409313168988403, 1.000000000000000000),
 ( 1.000000000000000000, 0.9377165729686763873, 1.000000000000000000),
 ( 1.000000000000000000, 0.9345773786260987981, 1.000000000000000000),
 ( 1.000000000000000000, 0.9318492984274224789, 1.000000000000000000),
 ( 1.000000000000000000, 0.9273872927429853696, 1.000000000000000000),
 ( 1.000000000000000000, 0.9256532593469947168, 1.000000000000000000),
 ( 1.000000000000000000, 0.9239357372751189068, 1.000000000000000000),
 ( 1.000000000000000000, 0.9235102113428168558, 1.000000000000000000),
 ( 1.000000000000000000, 0.9229728558028662544, 1.000000000000000000),
 ( 1.000000000000000000, 0.9228633126626074601, 1.000000000000000000),
 ( 1.000000000000000000, 0.9230139704737772011, 1.000000000000000000),
 ( 1.000000000000000000, 0.9237531682202682060, 1.000000000000000000),
 ( 1.000000000000000000, 0.9264156051932146418, 1.000000000000000000),
 ( 1.000000000000000000, 0.9283388455998524691, 1.000000000000000000),
 ( 1.000000000000000000, 0.9320050037531947273, 1.000000000000000000),
 ( 1.000000000000000000, 0.9333574575348377866, 1.000000000000000000),
 ( 1.000000000000000000, 0.9355411998009157681, 1.000000000000000000),
 ( 1.000000000000000000, 0.9362956009277125791, 1.000000000000000000),
 ( 1.000000000000000000, 0.9374637148015746435, 1.000000000000000000),
 ( 1.000000000000000000, 0.9378591705544939705, 1.000000000000000000),
 ( 1.000000000000000000, 0.9384610703419805633, 1.000000000000000000),
 ( 1.000000000000000000, 0.9386631562400454820, 1.000000000000000000),
 ( 1.000000000000000000, 0.9388793792114364933, 1.000000000000000000),
 ( 1.000000000000000000, 0.9388921037490475241, 1.000000000000000000),
 ( 1.000000000000000000, 0.9389175638858665573, 1.000000000000000000),
 ( 1.000000000000000000, 0.9389305010154709308, 1.000000000000000000),
 ( 1.000000000000000000, 0.9389691441648050363, 1.000000000000000000),
 ( 1.000000000000000000, 0.9389948969011622237, 1.000000000000000000),
 ( 1.000000000000000000, 0.9390721270299990930, 1.000000000000000000),
 ( 1.000000000000000000, 0.9391235763422335348, 1.000000000000000000),
 ( 1.000000000000000000, 0.9392778120326625846, 1.000000000000000000),
 ( 1.000000000000000000, 0.9393804861645765891, 1.000000000000000000),
 ( 1.000000000000000000, 0.9427638002347920043, 1.000000000000000000),
 ( 1.000000000000000000, 0.9458915987233171840, 1.000000000000000000),
 ( 1.000000000000000000, 0.9607963039206464106, 1.000000000000000000),
 ( 1.000000000000000000, 0.9703812854709539248, 1.000000000000000000),
 ( 1.000000000000000000, 0.9854660764533730299, 1.000000000000000000),
 ( 1.000000000000000000, 0.9909632567911320633, 1.000000000000000000),
 ( 1.000000000000000000, 0.9982308762617714271, 1.000000000000000000),
 ( 1.000000000000000000, 0.9999976772058264407, 1.000000000000000000),
 ( 1.000000000000000000, 1.000000000000000000, 1.000000000000000000) ) ) 
 REPRESENTATION_ITEM ( '' )  SURFACE ( )  );
#1405=CARTESIAN_POINT ( 'NONE',  ( -56.48582580120559982, -6.472252184284282173, 50.09629031063965243 ) ) ;
#1406=CARTESIAN_POINT ( 'NONE',  ( 184.8905102610680444, 1.070102760522089011E-13, -20.92133201514444352 ) ) ;
#1407=CARTESIAN_POINT ( 'NONE',  ( 151.7948205124836250, -23.49921654116371883, 23.49921654116317526 ) ) ;
#1408=CARTESIAN_POINT ( 'NONE',  ( 14.38125909742180752, 55.17850393971008316, -40.00000000000002132 ) ) ;
#1411=CARTESIAN_POINT ( 'NONE',  ( -82.23724611274339225, 0.6214486198419367780, -20.19553932739445656 ) ) ;
#1412=CARTESIAN_POINT ( 'NONE',  ( -162.0762913951021176, 29.48230308784730980, 27.08623940707652622 ) ) ;
#1413=CARTESIAN_POINT ( 'NONE',  ( -105.3755690713226585, 15.38646221621820764, -41.18208027870583265 ) ) ;
#1414=CARTESIAN_POINT ( 'NONE',  ( 19.06497207195981147, -10.03556273973439517, 10.03556273973429214 ) ) ;
#1415=CARTESIAN_POINT ( 'NONE',  ( 136.1360204305621266, -24.77266263493151044, 24.77266263493093135 ) ) ;
#1416=CARTESIAN_POINT ( 'NONE',  ( 146.6084372240433709, 52.76785682606523409, -3.800685668858194255 ) ) ;
#1417=CARTESIAN_POINT ( 'NONE',  ( 151.7948205124835681, 51.78348778862544322, -4.785054706298002891 ) ) ;
#1418=CARTESIAN_POINT ( 'NONE',  ( 19.06497207195980792, -18.24870850772710540, -38.31983398719647482 ) ) ;
#1419=CARTESIAN_POINT ( 'NONE',  ( -105.3755690713226727, -15.38646221621807619, 15.38646221621768362 ) ) ;
#1420=CARTESIAN_POINT ( 'NONE',  ( -114.5520595707410081, -6.810300319901277710, -20.89066663055196926 ) ) ;
#1421=CARTESIAN_POINT ( 'NONE',  ( 184.8905102610680444, -14.79361573936379415, -14.79361573936387941 ) ) ;
#1422=CARTESIAN_POINT ( 'NONE',  ( -30.26275506840324070, -40.00000000000003553, 1.694272468446120117 ) ) ;
#1423=CARTESIAN_POINT ( 'NONE',  ( 14.38125909742181285, -10.73282306404712472, -10.73282306404731301 ) ) ;
#1424=CARTESIAN_POINT ( 'NONE',  ( -192.9588430854689989, 54.46834944099968823, 2.449293598294708485E-15 ) ) ;
#1426=EDGE_CURVE ( 'NONE', #5206, #17844, #12718, .T. ) ;
#1427=CARTESIAN_POINT ( 'NONE',  ( 170.2234770963711128, 39.20704971665398375, -17.36149277826984871 ) ) ;
#1428=CARTESIAN_POINT ( 'NONE',  ( 18.43739873636958393, 43.10664370278630031, 17.85535645007986716 ) ) ;
#1429=CARTESIAN_POINT ( 'NONE',  ( 98.29820294267337033, 7.653668647303973671, 18.47759065023120328 ) ) ;
#1430=CARTESIAN_POINT ( 'NONE',  ( -87.12800209209288482, -21.45652401693875078, 1.368681197236398361 ) ) ;
#1433=CARTESIAN_POINT ( 'NONE',  ( -200.5022718138936284, -44.86987976039414860, 18.58571273880634322 ) ) ;
#1435=CARTESIAN_POINT ( 'NONE',  ( 23.54890483848222615, -13.78807129923187169, 46.74501720879658961 ) ) ;
#1436=EDGE_CURVE ( 'NONE', #20782, #10228, #1513, .T. ) ;
#1439=CARTESIAN_POINT ( 'NONE',  ( -87.13361725327072804, 21.49321519333427233, -1.448021113139547951E-30 ) ) ;
#1440=CARTESIAN_POINT ( 'NONE',  ( -86.96347745069645896, 40.00000000000008527, -21.75974354311636461 ) ) ;
#1441=CARTESIAN_POINT ( 'NONE',  ( -91.56559293963834989, 6.234561990864368500E-14, -22.67402823373191723 ) ) ;
#1442=( BOUNDED_CURVE ( )  B_SPLINE_CURVE ( 3, ( #15584, #17204, #991, #9096, #25341, #7098, #5235 ),
 .UNSPECIFIED., .F., .F. ) 
 B_SPLINE_CURVE_WITH_KNOTS ( ( 4, 3, 4 ),
 ( 0.007504621739143815112, 0.02318610956072928234, 0.03886759738231780614 ),
 .UNSPECIFIED. ) 
 CURVE ( )  GEOMETRIC_REPRESENTATION_ITEM ( )  RATIONAL_B_SPLINE_CURVE ( ( 0.5852718452494397594, 0.6660804010233953854, 0.8043231192735821322, 1.000000000000000000, 0.8043231192735440516, 0.6660804010233416506, 0.5852718452493926860 ) ) 
 REPRESENTATION_ITEM ( '' )  );
#1443=CARTESIAN_POINT ( 'NONE',  ( 22.82385994800816320, 47.01156385802210025, -13.83113328680595266 ) ) ;
#1444=CARTESIAN_POINT ( 'NONE',  ( 146.6084372240433993, -5.374981219216945938, -2.449293598294708485E-15 ) ) ;
#1445=CARTESIAN_POINT ( 'NONE',  ( -166.3490736462130144, 12.23457872939038715, -39.29841219616762515 ) ) ;
#1447=CARTESIAN_POINT ( 'NONE',  ( -135.8532207217289738, 9.153146818113546246, -0.000000000000000000 ) ) ;
#1448=CARTESIAN_POINT ( 'NONE',  ( 14.38125909742181285, -15.17850393972633505, 0.000000000000000000 ) ) ;
#1449=CARTESIAN_POINT ( 'NONE',  ( 0.2972598230769930017, 14.33493731733933352, 40.00000000000002132 ) ) ;
#1450=CARTESIAN_POINT ( 'NONE',  ( -135.8532207217289738, 40.00000000000031974, -30.84685318188603986 ) ) ;
#1452=CARTESIAN_POINT ( 'NONE',  ( 98.47991336697563725, -18.54450719071631681, -7.681386385922040816 ) ) ;
#1453=VERTEX_POINT ( 'NONE', #20834 ) ;
#1454=CARTESIAN_POINT ( 'NONE',  ( -87.04503123322955105, 20.91882565556252871, -4.710636111838677031 ) ) ;
#1455=CARTESIAN_POINT ( 'NONE',  ( 3.468680969976427608, 48.91035688725698805, -14.11592159092573162 ) ) ;
#1456=CARTESIAN_POINT ( 'NONE',  ( 146.6084372240433993, 34.62501878078308692, 0.000000000000000000 ) ) ;
#1460=ORIENTED_EDGE ( 'NONE', *, *, #20049, .T. ) ;
#1464=ORIENTED_EDGE ( 'NONE', *, *, #17113, .T. ) ;
#1466=ORIENTED_EDGE ( 'NONE', *, *, #15475, .T. ) ;
#1469=CARTESIAN_POINT ( 'NONE',  ( 170.2234770963711128, 39.20704971665398375, -17.36149277826984871 ) ) ;
#1471=CARTESIAN_POINT ( 'NONE',  ( 0.2972598230769957217, -4.999556039334937811E-14, 14.33493731733933352 ) ) ;
#1472=CARTESIAN_POINT ( 'NONE',  ( -190.6721700386038663, -23.91541588165673460, 43.63442057298713905 ) ) ;
#1475=CARTESIAN_POINT ( 'NONE',  ( 170.2234770963711128, -2.259079968736224833E-13, 24.55285855007187124 ) ) ;
#1476=CARTESIAN_POINT ( 'NONE',  ( -91.56559293963834989, -39.99999999999985789, -17.32597176626853042 ) ) ;
#1477=CARTESIAN_POINT ( 'NONE',  ( -199.9999999999999432, -45.63305559644809506, -19.96680831879890761 ) ) ;
#1478=CARTESIAN_POINT ( 'NONE',  ( 136.1360204305621266, -3.511608612530379592, -53.05693388239318153 ) ) ;
#1479=CARTESIAN_POINT ( 'NONE',  ( -200.0000000000000000, 18.59955921182038807, -46.19968414209451169 ) ) ;
#1480=CARTESIAN_POINT ( 'NONE',  ( 163.1118516004056573, -37.29075403953139300, -19.27778845539249630 ) ) ;
#1481=CARTESIAN_POINT ( 'NONE',  ( -102.4068193528150061, 8.088405365068718211, 20.44188272012853957 ) ) ;
#1483=CARTESIAN_POINT ( 'NONE',  ( -77.61378591600576726, 12.98772233503618878, -17.87002798532567027 ) ) ;
#1484=CARTESIAN_POINT ( 'NONE',  ( 57.59792236341147031, 1.722363176415065089, -1.722363176415036445 ) ) ;
#1485=CARTESIAN_POINT ( 'NONE',  ( 57.59792236341148453, -40.00000000000000000, -2.435789363418300546 ) ) ;
#1486=CARTESIAN_POINT ( 'NONE',  ( -213.1075012329537230, 9.698598906462684965, 66.26714140138669507 ) ) ;
#1487=CARTESIAN_POINT ( 'NONE',  ( -208.1127848780264742, -67.17687982760682530, -10.60833733268364298 ) ) ;
#1488=CARTESIAN_POINT ( 'NONE',  ( -183.1091233172618615, -13.45963571010332949, -45.18843800007923051 ) ) ;
#1491=CARTESIAN_POINT ( 'NONE',  ( 4.995406935893290878, 39.06748935135239265, -39.06748935135144762 ) ) ;
#1495=CARTESIAN_POINT ( 'NONE',  ( -213.1075012329537230, 9.698598906438871126, -66.26714140136179765 ) ) ;
#1498=CARTESIAN_POINT ( 'NONE',  ( 57.59792236341147031, -1.493297263419786540E-14, 2.435789363418160658 ) ) ;
#1501=CARTESIAN_POINT ( 'NONE',  ( -77.90255099907078318, 8.644468104260425889, 20.04994828523877359 ) ) ;
#1504=CARTESIAN_POINT ( 'NONE',  ( 184.8905102610680444, 19.07866798485562043, 2.449293598294708485E-15 ) ) ;
#1505=CARTESIAN_POINT ( 'NONE',  ( -195.1685814578493421, -48.78510996053816484, -14.09692187700277444 ) ) ;
#1506=CARTESIAN_POINT ( 'NONE',  ( 163.1118516004056573, 40.00000000000000711, 12.73709011382489642 ) ) ;
#1509=CARTESIAN_POINT ( 'NONE',  ( -135.8532207217289738, 39.99999999999990763, 9.153146818113990335 ) ) ;
#1510=CARTESIAN_POINT ( 'NONE',  ( -91.56559293963834989, -7.976292724337646577E-14, 17.32597176626811120 ) ) ;
#1513=CIRCLE ( 'NONE', #21880, 14.99999999999999645 ) ;
#1514=CARTESIAN_POINT ( 'NONE',  ( 200.0000000000000000, 40.00000000000012790, -19.99999999999996092 ) ) ;
#1516=CARTESIAN_POINT ( 'NONE',  ( -4.915070467875013449, -23.27857837409171182, -42.74707758271716074 ) ) ;
#1517=CARTESIAN_POINT ( 'NONE',  ( -86.96347745069643054, 15.38646221621821297, -41.18208027870583265 ) ) ;
#1518=DIRECTION ( 'NONE',  ( -1.511376984792852195E-16, -4.006716270543645993E-17, -1.000000000000000000 ) ) ;
#1519=CARTESIAN_POINT ( 'NONE',  ( -280.0000000000000568, -40.00000000000028422, 19.99999999999959499 ) ) ;
#1521=CARTESIAN_POINT ( 'NONE',  ( 57.59792236341147031, 2.435789363418171760, 0.000000000000000000 ) ) ;
#1522=CARTESIAN_POINT ( 'NONE',  ( -135.8532207217289738, 9.153146818113548022, -40.00000000000002132 ) ) ;
#1523=CARTESIAN_POINT ( 'NONE',  ( -56.48582580120559982, 34.75652343174597547, 21.81201906317791384 ) ) ;
#1525=CARTESIAN_POINT ( 'NONE',  ( 91.82158438592158234, 17.20528682183301683, 0.000000000000000000 ) ) ;
#1527=CARTESIAN_POINT ( 'NONE',  ( -114.5247552372686357, 20.75064880308619308, 7.059277231979386613 ) ) ;
#1528=CARTESIAN_POINT ( 'NONE',  ( -162.0762913951020892, 29.48230308784758691, 29.48230308784772191 ) ) ;
#1530=CARTESIAN_POINT ( 'NONE',  ( 170.2234770963711128, 15.44714144992819094, 2.449293598294708485E-15 ) ) ;
#1532=CARTESIAN_POINT ( 'NONE',  ( 90.68848423405329129, -21.28058941706692053, 8.814708751807811993 ) ) ;
#1534=CARTESIAN_POINT ( 'NONE',  ( 126.3230993689412855, 11.72464299830463652, 28.30579214049060610 ) ) ;
#1535=CARTESIAN_POINT ( 'NONE',  ( 4.995406935893283773, 39.06748935135195211, -17.50105314357185193 ) ) ;
#1536=CARTESIAN_POINT ( 'NONE',  ( 19.06497207195981858, -1.881589693694111225E-13, 54.19242893257843008 ) ) ;
#1537=CARTESIAN_POINT ( 'NONE',  ( -56.48582580120559982, 21.81201906317729922, 34.75652343174635917 ) ) ;
#1538=AXIS2_PLACEMENT_3D ( 'NONE', #24991, #24721, #9013 ) ;
#1539=CARTESIAN_POINT ( 'NONE',  ( 130.8568914410475088, -34.05028731879786363, -40.00000000000002132 ) ) ;
#1542=CARTESIAN_POINT ( 'NONE',  ( -86.86493150571115507, -7.943527260495787168, -19.77569912839188859 ) ) ;
#1543=CARTESIAN_POINT ( 'NONE',  ( -30.26275506840324070, 1.198031551616030033, -1.198031551616006496 ) ) ;
#1544=CARTESIAN_POINT ( 'NONE',  ( -91.56559293963834989, -12.25131212657475466, -12.25131212657495361 ) ) ;
#1545=CARTESIAN_POINT ( 'NONE',  ( 91.82158438592158234, 12.16597498397773869, -12.16597498397759303 ) ) ;
#1546=CARTESIAN_POINT ( 'NONE',  ( 91.82158438592158234, -1.633484621919921769E-13, 17.20528682183300262 ) ) ;
#1547=CARTESIAN_POINT ( 'NONE',  ( 91.82158438592156813, 40.45024623143973486, -16.11829626348390931 ) ) ;
#1549=CARTESIAN_POINT ( 'NONE',  ( -198.0356074513804288, -39.15871834505882276, -39.15871834505946936 ) ) ;
#1550=CARTESIAN_POINT ( 'NONE',  ( -86.96347745069644475, -43.67073346367964604, -12.89780903124457545 ) ) ;
#1551=CARTESIAN_POINT ( 'NONE',  ( 91.82158438592158234, -12.16597498399995203, -44.40256751092347542 ) ) ;
#1552=CARTESIAN_POINT ( 'NONE',  ( -259.2033419157646676, 6.730120644403521979, -6.730120644403498886 ) ) ;
#1553=CARTESIAN_POINT ( 'NONE',  ( 170.0000000000000000, 24.95097643317003744, 0.000000000000000000 ) ) ;
#1555=CARTESIAN_POINT ( 'NONE',  ( 184.8905102610680444, -39.99999999999991473, -20.92133201514458207 ) ) ;
#1556=CARTESIAN_POINT ( 'NONE',  ( -56.48582580120558561, 6.472252184283903809, 50.09629031063968796 ) ) ;
#1557=CARTESIAN_POINT ( 'NONE',  ( 199.9999999999999432, 14.14213562373093680, 14.14213562373114641 ) ) ;
#1558=CARTESIAN_POINT ( 'NONE',  ( 151.7948205124836534, 6.767089262349056611, 40.00000000000002132 ) ) ;
#1560=CARTESIAN_POINT ( 'NONE',  ( -162.0762913951020892, 1.198031840385716418, 1.198031840385750169 ) ) ;
#1561=CARTESIAN_POINT ( 'NONE',  ( -77.92915424793434909, 20.15198149301296482, 8.347224043097730473 ) ) ;
#1562=CARTESIAN_POINT ( 'NONE',  ( 98.29820294267334191, 7.653668647303994099, 18.47759065023120684 ) ) ;
#1563=CARTESIAN_POINT ( 'NONE',  ( 98.29820294267339875, -20.00000000000581224, -1.310413973304028090 ) ) ;
#1565=CARTESIAN_POINT ( 'NONE',  ( -200.4317933031552741, -49.29858032309926585, 14.17468109412851796 ) ) ;
#1567=CARTESIAN_POINT ( 'NONE',  ( -3.205219349397939510, -17.96245967913801778, 43.36521377095295549 ) ) ;
#1568=CARTESIAN_POINT ( 'NONE',  ( 22.79879570922453169, 17.88067497375744352, -43.16776802602858254 ) ) ;
#1571=CARTESIAN_POINT ( 'NONE',  ( -105.4741150117379789, -19.60045294982730724, -8.366608964594114184 ) ) ;
#1572=CARTESIAN_POINT ( 'NONE',  ( 14.38125909742180930, 39.99999999999982947, 55.17850393971022527 ) ) ;
#1573=CARTESIAN_POINT ( 'NONE',  ( -87.13361725327072804, -2.411356650979014119E-13, 21.49321519333428299 ) ) ;
#1575=CARTESIAN_POINT ( 'NONE',  ( 19.06497207195981147, 38.31983398719673772, -38.31983398719579981 ) ) ;
#1576=CARTESIAN_POINT ( 'NONE',  ( -105.3755690713226585, -18.24025645688355013, 40.00000000000002132 ) ) ;
#1580=CARTESIAN_POINT ( 'NONE',  ( 91.82158438592158234, 17.20528682183301683, 0.000000000000000000 ) ) ;
#1581=CARTESIAN_POINT ( 'NONE',  ( 130.8568914410475088, -34.05028731879786363, 40.00000000000002132 ) ) ;
#1582=CARTESIAN_POINT ( 'NONE',  ( 136.1360204305621551, -39.99999999999994316, -4.966164525587488221 ) ) ;
#1583=CARTESIAN_POINT ( 'NONE',  ( 98.29820294273281434, -7.653668647304240125, 18.47759065023114644 ) ) ;
#1584=CARTESIAN_POINT ( 'NONE',  ( -198.0356074513804572, 17.40982414986501325, -39.15871834505897198 ) ) ;
#1587=CARTESIAN_POINT ( 'NONE',  ( 170.2234770963711128, 24.55285855007190676, 40.00000000000002132 ) ) ;
#1588=EDGE_CURVE ( 'NONE', #11219, #16477, #2420, .T. ) ;
#1590=CARTESIAN_POINT ( 'NONE',  ( -88.37877758189179644, -8.026456974226181984, 20.15391234919130525 ) ) ;
#1592=ORIENTED_EDGE ( 'NONE', *, *, #17520, .T. ) ;
#1594=CARTESIAN_POINT ( 'NONE',  ( 91.82158438592159655, -44.40256751092324095, -12.16597498400075139 ) ) ;
#1595=CARTESIAN_POINT ( 'NONE',  ( 22.37977766478896058, -43.15105302556170130, -23.55755712318277162 ) ) ;
#1597=CARTESIAN_POINT ( 'NONE',  ( -208.1127848780264742, 15.00245453012665742, -40.00000000000002132 ) ) ;
#1598=CARTESIAN_POINT ( 'NONE',  ( -105.4741150117399684, -19.60045294982700170, 8.366608964593480025 ) ) ;
#1602=CARTESIAN_POINT ( 'NONE',  ( 170.2234770963711128, -17.36149277826995885, 39.20704971665388427 ) ) ;
#1603=B_SPLINE_CURVE_WITH_KNOTS ( 'NONE', 3,
 ( #9185, #3575, #17798, #3714, #5838, #9558, #1986, #13942, #3850, #25944, #17666, #5575 ),
 .UNSPECIFIED., .F., .F.,
 ( 4, 2, 2, 2, 2, 4 ),
 ( 0.000000000000000000, 0.005971690550335614737, 0.008957535825503465041, 0.01045045846308743052, 0.01119691978187945143, 0.01194338110067147407 ),
 .UNSPECIFIED. ) ;
#1605=( BOUNDED_SURFACE ( )  B_SPLINE_SURFACE ( 3, 2, ( 
 ( #13412, #17920, #25666 ),
 ( #7292, #11804, #22065 ),
 ( #19790, #21536, #13536 ),
 ( #7672, #7412, #21661 ),
 ( #15526, #15784, #11407 ),
 ( #19658, #19529, #1445 ),
 ( #19924, #7801, #24050 ),
 ( #1314, #23781, #13667 ),
 ( #19409, #21790, #3562 ),
 ( #11666, #1707, #9680 ),
 ( #22334, #372, #7941 ),
 ( #12073, #8476, #6093 ),
 ( #12208, #4109, #16594 ),
 ( #24727, #24185, #22201 ),
 ( #14465, #18594, #16466 ),
 ( #20066, #24590, #18455 ),
 ( #10215, #9944, #16059 ),
 ( #14200, #6483, #11940 ),
 ( #16328, #1842, #24457 ),
 ( #4245, #2106, #103 ),
 ( #4374, #2368, #20194 ),
 ( #8210, #20329, #18321 ),
 ( #1974, #24329, #14595 ),
 ( #12464, #20592, #18054 ),
 ( #26205, #14334, #6221 ),
 ( #10080, #22466, #22724 ),
 ( #12335, #5959, #16196 ),
 ( #14069, #18185, #20463 ),
 ( #3976, #2237, #26335 ),
 ( #8076, #233, #10345 ),
 ( #8345, #6346, #22598 ),
 ( #10480, #19255, #18862 ),
 ( #17124, #10613, #1035 ),
 ( #25255, #16726, #6878 ) ),
 .UNSPECIFIED., .F., .F., .F. ) 
 B_SPLINE_SURFACE_WITH_KNOTS ( ( 4, 2, 2, 2, 2, 2, 2, 2, 2, 2, 2, 2, 2, 2, 2, 2, 4 ),
 ( 3, 3 ),
 ( 0.005135431517081130715, 0.02907016617530081351, 0.05300490083352049631, 0.07693963549174018257, 0.08292331915629509720, 0.08441924007243381545, 0.08446598760106314996, 0.08448936136537782415, 0.08451273512969248447, 0.08460623018695115349, 0.08479322030146849154, 0.08516720053050318151, 0.08591516098857254757, 0.08890700282085001183, 0.09189884465312747608, 0.09489068648540494033, 0.1008743701499598550 ),
 ( 0.000000000000000000, 1.000000000000000000 ),
 .UNSPECIFIED. ) 
 GEOMETRIC_REPRESENTATION_ITEM ( )  RATIONAL_B_SPLINE_SURFACE ( (
 ( 1.000000000000000000, 0.9997813423552077694, 1.000000000000000000),
 ( 1.000000000000000000, 0.9991063894442805404, 1.000000000000000000),
 ( 1.000000000000000000, 0.9968824679670509337, 1.000000000000000000),
 ( 1.000000000000000000, 0.9891556708430848666, 1.000000000000000000),
 ( 1.000000000000000000, 0.9836552227697955564, 1.000000000000000000),
 ( 1.000000000000000000, 0.9690804699604719241, 1.000000000000000000),
 ( 1.000000000000000000, 0.9600093828083156033, 1.000000000000000000),
 ( 1.000000000000000000, 0.9461484455230979584, 1.000000000000000000),
 ( 1.000000000000000000, 0.9432496483671297671, 1.000000000000000000),
 ( 1.000000000000000000, 0.9394619383806620538, 1.000000000000000000),
 ( 1.000000000000000000, 0.9386961831920602739, 1.000000000000000000),
 ( 1.000000000000000000, 0.9378979462694526648, 1.000000000000000000),
 ( 1.000000000000000000, 0.9378737491732507259, 1.000000000000000000),
 ( 1.000000000000000000, 0.9378374413774228646, 1.000000000000000000),
 ( 1.000000000000000000, 0.9378252326299143515, 1.000000000000000000),
 ( 1.000000000000000000, 0.9378013115143155609, 1.000000000000000000),
 ( 1.000000000000000000, 0.9377893564346093669, 1.000000000000000000),
 ( 1.000000000000000000, 0.9377296084626354222, 1.000000000000000000),
 ( 1.000000000000000000, 0.9376818978498914214, 1.000000000000000000),
 ( 1.000000000000000000, 0.9375390306864402890, 1.000000000000000000),
 ( 1.000000000000000000, 0.9374441388111856011, 1.000000000000000000),
 ( 1.000000000000000000, 0.9371605328928512835, 1.000000000000000000),
 ( 1.000000000000000000, 0.9369728885716379629, 1.000000000000000000),
 ( 1.000000000000000000, 0.9364143219790427297, 1.000000000000000000),
 ( 1.000000000000000000, 0.9360477663173715213, 1.000000000000000000),
 ( 1.000000000000000000, 0.9342452504720836215, 1.000000000000000000),
 ( 1.000000000000000000, 0.9329001521054777202, 1.000000000000000000),
 ( 1.000000000000000000, 0.9304320728631004789, 1.000000000000000000),
 ( 1.000000000000000000, 0.9293115496650089513, 1.000000000000000000),
 ( 1.000000000000000000, 0.9273349178230613221, 1.000000000000000000),
 ( 1.000000000000000000, 0.9264755994061862898, 1.000000000000000000),
 ( 1.000000000000000000, 0.9243018539389631361, 1.000000000000000000),
 ( 1.000000000000000000, 0.9233922906946041564, 1.000000000000000000),
 ( 1.000000000000000000, 0.9230540990195960083, 1.000000000000000000) ) ) 
 REPRESENTATION_ITEM ( '' )  SURFACE ( )  );
#1609=CARTESIAN_POINT ( 'NONE',  ( -93.12335834970892279, -16.03295912088728414, 16.03295912088688269 ) ) ;
#1610=CARTESIAN_POINT ( 'NONE',  ( -280.0000000000000000, -2.609240458947769655E-13, 20.00000000000001421 ) ) ;
#1611=CARTESIAN_POINT ( 'NONE',  ( -114.4940140763160912, -9.297404372800567529, 19.81979918810025154 ) ) ;
#1612=CARTESIAN_POINT ( 'NONE',  ( 91.82158438592156813, -16.11829626348402655, -40.45024623143966380 ) ) ;
#1613=CARTESIAN_POINT ( 'NONE',  ( -259.2033419157646676, -30.48217210827743884, -40.00000000000002132 ) ) ;
#1614=CARTESIAN_POINT ( 'NONE',  ( -105.3755690713226585, -12.89780903124383471, -43.67073346367985920 ) ) ;
#1615=CARTESIAN_POINT ( 'NONE',  ( -96.93773665438791909, -9.001171854902402458, 20.58457565566394010 ) ) ;
#1617=CARTESIAN_POINT ( 'NONE',  ( -192.9588430854689989, 1.161019517985663313E-13, -14.46834944099969533 ) ) ;
#1618=CARTESIAN_POINT ( 'NONE',  ( 136.1360204305621266, 1.473277640373554421E-13, -35.03383547441296741 ) ) ;
#1619=CARTESIAN_POINT ( 'NONE',  ( 0.2972598230769990524, -18.14793986248724522, 38.42060263243662632 ) ) ;
#1620=CARTESIAN_POINT ( 'NONE',  ( -100.7734535825088500, 16.03295912088691821, 16.03295912088721309 ) ) ;
#1621=CARTESIAN_POINT ( 'NONE',  ( -195.5008451367478983, -18.44412755965894846, -44.52806290062954986 ) ) ;
#1622=CARTESIAN_POINT ( 'NONE',  ( -192.9588430854689989, -10.23066800230756890, 10.23066800230742501 ) ) ;
#1624=CARTESIAN_POINT ( 'NONE',  ( -238.4067589809705794, 28.96627169325354956, -28.96627169325289231 ) ) ;
#1625=CARTESIAN_POINT ( 'NONE',  ( -114.7537493279899223, -2.780162309571297286, 21.97305528828380261 ) ) ;
#1626=CARTESIAN_POINT ( 'NONE',  ( -105.3755690713226585, 21.75974354311648185, -40.00000000000002132 ) ) ;
#1628=CARTESIAN_POINT ( 'NONE',  ( 4.995406935893294431, -17.50105314357144337, -39.06748935135212264 ) ) ;
#1629=CARTESIAN_POINT ( 'NONE',  ( -77.59415595804735233, 2.768978254217757673, 21.92621357340613031 ) ) ;
#1631=CARTESIAN_POINT ( 'NONE',  ( -86.96347745069644475, -2.438961472018186339E-13, 21.75974354311649961 ) ) ;
#1632=CARTESIAN_POINT ( 'NONE',  ( 23.37394308801976806, -13.80096434448233111, -46.80823611210209378 ) ) ;
#1633=CARTESIAN_POINT ( 'NONE',  ( -16.78454218904764872, 16.41855578209794686, 39.63790004357517915 ) ) ;
#1634=VERTEX_POINT ( 'NONE', #15471 ) ;
#1635=ORIENTED_EDGE ( 'NONE', *, *, #25912, .T. ) ;
#1636=CARTESIAN_POINT ( 'NONE',  ( 146.6084372240433993, 5.374981219216999229, 2.449293598294708485E-15 ) ) ;
#1637=CARTESIAN_POINT ( 'NONE',  ( -198.0356074513804572, -10.87444709759729911, 10.87444709759714812 ) ) ;
#1638=CARTESIAN_POINT ( 'NONE',  ( -56.48582580120559982, 39.99999999999990763, 30.84685318188658698 ) ) ;
#1643=CARTESIAN_POINT ( 'NONE',  ( 151.7948205124836250, -3.202120068677277203E-13, 33.23291073765553705 ) ) ;
#1645=CARTESIAN_POINT ( 'NONE',  ( -129.2303492456788945, 9.309000511628456209, 25.82246949224157362 ) ) ;
#1646=CARTESIAN_POINT ( 'NONE',  ( -2.557884977122323100, -23.77085849408081231, -43.43882039326604882 ) ) ;
#1647=CARTESIAN_POINT ( 'NONE',  ( 19.06497207195982924, -66.60410523465809263, -10.03556273973493163 ) ) ;
#1648=DIRECTION ( 'NONE',  ( -1.000000000000000000, 0.000000000000000000, 1.511376984792852195E-16 ) ) ;
#1649=CARTESIAN_POINT ( 'NONE',  ( -198.0356074513804288, -39.15871834505936278, 39.15871834505892224 ) ) ;
#1650=CARTESIAN_POINT ( 'NONE',  ( 163.1118516004056573, -40.00000000000027711, 27.26290988616830546 ) ) ;
#1653=CARTESIAN_POINT ( 'NONE',  ( -86.96347745069644475, -18.24025645688354302, -2.449293598294708485E-15 ) ) ;
#1654=CARTESIAN_POINT ( 'NONE',  ( 19.06497207195980792, 18.24870850772737185, 38.31983398719634692 ) ) ;
#1655=CARTESIAN_POINT ( 'NONE',  ( 14.38125909742182884, -55.17850393971007605, 40.00000000000002132 ) ) ;
#1656=CARTESIAN_POINT ( 'NONE',  ( -3.069599232962560986, -43.28003856805334237, -23.65302469262813290 ) ) ;
#1657=CARTESIAN_POINT ( 'NONE',  ( 184.8905102610680444, -1.851754852062639767E-13, 20.92133201514444352 ) ) ;
#1658=CARTESIAN_POINT ( 'NONE',  ( 130.8568914410475088, 32.49135343045483637, -24.07718906446901030 ) ) ;
#1659=CARTESIAN_POINT ( 'NONE',  ( 192.4448373802100889, -20.00000000003938538, 0.000000000000000000 ) ) ;
#1662=CARTESIAN_POINT ( 'NONE',  ( 22.76403192593588543, -43.17745271018599595, 17.88468650128193715 ) ) ;
#1663=CARTESIAN_POINT ( 'NONE',  ( 104.1600437297061745, 8.548029202655486714, 20.63676802864342363 ) ) ;
#1665=CARTESIAN_POINT ( 'NONE',  ( -198.0356074513804572, 39.15871834505912119, -17.40982414986464377 ) ) ;
#1666=CARTESIAN_POINT ( 'NONE',  ( 184.8905102610680444, -39.99999999999991473, -20.92133201514458207 ) ) ;
#1667=CARTESIAN_POINT ( 'NONE',  ( -86.96347745069644475, -15.38646221621807442, 15.38646221621768184 ) ) ;
#1670=CARTESIAN_POINT ( 'NONE',  ( -30.26275506840324070, 1.694272468446254232, 0.000000000000000000 ) ) ;
#1673=EDGE_CURVE ( 'NONE', #19299, #23960, #24451, .T. ) ;
#1674=EDGE_CURVE ( 'NONE', #3292, #2226, #4485, .T. ) ;
#1676=CARTESIAN_POINT ( 'NONE',  ( -100.7734535825088500, 40.53558337403654832, 16.03295912088756481 ) ) ;
#1677=CARTESIAN_POINT ( 'NONE',  ( 136.1360204305621551, 24.77266263493153176, -31.79587985999237887 ) ) ;
#1679=CARTESIAN_POINT ( 'NONE',  ( -87.04313178894985015, 18.12206666836759084, -11.44454159254445891 ) ) ;
#1680=CARTESIAN_POINT ( 'NONE',  ( 163.1118516004056573, 19.27778845539265618, -37.29075403953135037 ) ) ;
#1681=CARTESIAN_POINT ( 'NONE',  ( 57.59792236341148453, 1.722363176415528940, -54.84617931850878136 ) ) ;
#1683=CARTESIAN_POINT ( 'NONE',  ( -238.4067589809705794, -27.60227080167029001, -28.96627169325357798 ) ) ;
#1688=CARTESIAN_POINT ( 'NONE',  ( -91.56559293963834989, -39.99999999999995737, -22.67402823373205933 ) ) ;
#1689=CARTESIAN_POINT ( 'NONE',  ( -162.0762913951020607, -1.198031840455708430, 57.76657433537920383 ) ) ;
#1691=CARTESIAN_POINT ( 'NONE',  ( -100.7734535825088500, 17.32597176626808988, 40.00000000000002132 ) ) ;
#1693=CARTESIAN_POINT ( 'NONE',  ( -238.4067589809705794, 28.96627169325324758, -27.60227080167054581 ) ) ;
#1696=CARTESIAN_POINT ( 'NONE',  ( 163.1118516004056573, -27.26290988616869626, 0.000000000000000000 ) ) ;
#1698=CARTESIAN_POINT ( 'NONE',  ( -192.1963514251730203, -43.96876056340474292, 24.16258207727632978 ) ) ;
#1700=CARTESIAN_POINT ( 'NONE',  ( -4.031723327955650582, -23.45082932595530423, 43.00750292060842384 ) ) ;
#1702=CARTESIAN_POINT ( 'NONE',  ( 23.35928221536270399, 23.34300348377183454, -42.86167611819463019 ) ) ;
#1705=CARTESIAN_POINT ( 'NONE',  ( 4.995406935893286438, 67.35176059880245703, -10.78321810387767066 ) ) ;
#1706=CARTESIAN_POINT ( 'NONE',  ( -56.48582580120558561, -30.84685318188645908, 40.00000000000002132 ) ) ;
#1707=CARTESIAN_POINT ( 'NONE',  ( -187.8779108535516400, 17.82355704116720574, -43.02987313850719886 ) ) ;
#1709=CARTESIAN_POINT ( 'NONE',  ( 130.8568914410475372, 34.05028731879791337, 0.000000000000000000 ) ) ;
#1710=CARTESIAN_POINT ( 'NONE',  ( 14.38125909742181285, -15.17850393972633505, -40.00000000000002132 ) ) ;
#1711=CARTESIAN_POINT ( 'NONE',  ( 14.38125909742180752, 15.17850393972634038, 40.00000000000002132 ) ) ;
#1712=CARTESIAN_POINT ( 'NONE',  ( 130.8568914410475372, 8.880724697947696879E-14, -5.949712681206690945 ) ) ;
#1713=CARTESIAN_POINT ( 'NONE',  ( -30.26275506840324070, 1.218738420030236455E-14, -1.694272468446259783 ) ) ;
#1714=CARTESIAN_POINT ( 'NONE',  ( -280.0000000000000000, 14.14213562373078581, 14.14213562373108424 ) ) ;
#1716=DIRECTION ( 'NONE',  ( -1.000000000000000000, -1.836970198721024264E-16, 0.000000000000000000 ) ) ;
#1717=CARTESIAN_POINT ( 'NONE',  ( -192.9588430854689989, 10.23066800230742679, 10.23066800230749607 ) ) ;
#1719=CARTESIAN_POINT ( 'NONE',  ( -102.4294859495866348, -8.407280617917511023, 20.29697089056567805 ) ) ;
#1722=ORIENTED_EDGE ( 'NONE', *, *, #12326, .T. ) ;
#1723=CARTESIAN_POINT ( 'NONE',  ( -91.56559293963834989, -40.53558337403669753, -16.03295912088728770 ) ) ;
#1724=CARTESIAN_POINT ( 'NONE',  ( 23.54890483848231852, -46.74501720879656119, -13.78807129923171892 ) ) ;
#1726=CARTESIAN_POINT ( 'NONE',  ( -135.8532207217289738, -9.153146818113595984, -40.00000000000002132 ) ) ;
#1731=CARTESIAN_POINT ( 'NONE',  ( 163.1118516004056573, 9.006482792069629539, 9.006482792069634868 ) ) ;
#1732=CARTESIAN_POINT ( 'NONE',  ( -188.9524938556045583, -43.19211203807761024, -23.58789616778846110 ) ) ;
#1733=CARTESIAN_POINT ( 'NONE',  ( -213.1075012329537230, -2.291445344039133686E-13, 53.71589010951915100 ) ) ;
#1734=CARTESIAN_POINT ( 'NONE',  ( 14.38125909742180752, 15.17850393972634038, 0.000000000000000000 ) ) ;
#1738=CARTESIAN_POINT ( 'NONE',  ( -30.26275506840324070, -1.147469862568086380E-14, 1.694272468446259783 ) ) ;
#1739=CARTESIAN_POINT ( 'NONE',  ( -280.0000000000000568, -40.00000000000028422, 19.99999999999959499 ) ) ;
#1741=CARTESIAN_POINT ( 'NONE',  ( -110.0723150831631330, -10.27950330707893656, 17.37189535808295915 ) ) ;
#1742=CARTESIAN_POINT ( 'NONE',  ( 151.7948205124836534, -33.06932595376343897, -23.49921654116042902 ) ) ;
#1743=CARTESIAN_POINT ( 'NONE',  ( -30.26275506840324070, -1.694272468446265112, 0.000000000000000000 ) ) ;
#1744=CARTESIAN_POINT ( 'NONE',  ( -213.1075012329537230, -37.98287015391232302, -18.58567234101164800 ) ) ;
#1745=CARTESIAN_POINT ( 'NONE',  ( -102.4068193528148356, -8.735227608997083948, 20.17396017424882260 ) ) ;
#1747=CARTESIAN_POINT ( 'NONE',  ( -208.1127848780264742, 40.00000000000014211, -15.00245453012627728 ) ) ;
#1748=CARTESIAN_POINT ( 'NONE',  ( 14.38125909742181818, -40.00000000000007816, 15.17850393972619649 ) ) ;
#1749=CARTESIAN_POINT ( 'NONE',  ( 130.8568914410475088, 32.49135343045483637, -24.07718906446901030 ) ) ;
#1750=CARTESIAN_POINT ( 'NONE',  ( -114.4955329334175786, 9.314646064825868876, 19.81372178018229135 ) ) ;
#1751=CARTESIAN_POINT ( 'NONE',  ( -188.3392995398488949, -13.83024151208627650, -47.00482667599261788 ) ) ;
#1754=CARTESIAN_POINT ( 'NONE',  ( 151.7948205124836534, -51.78348778862529400, -4.785054706299085581 ) ) ;
#1755=CARTESIAN_POINT ( 'NONE',  ( -114.6318783467511508, -5.473070270845196816, 21.31802243456079538 ) ) ;
#1756=CARTESIAN_POINT ( 'NONE',  ( 19.06497207195981503, -14.19242893257840166, 0.000000000000000000 ) ) ;
#1758=CARTESIAN_POINT ( 'NONE',  ( 170.2234770963711128, 10.92277846919216522, -10.92277846919186501 ) ) ;
#1763=CARTESIAN_POINT ( 'NONE',  ( 48.46046611906520241, -11.89583623498083575, -37.63122027851154172 ) ) ;
#1765=CARTESIAN_POINT ( 'NONE',  ( -4.027137536851070898, 23.45200847982306414, 43.00884733904467794 ) ) ;
#1768=EDGE_LOOP ( 'NONE', ( #17544, #2552, #14244, #8261 ) ) ;
#1769=CARTESIAN_POINT ( 'NONE',  ( -56.48582580120559271, -6.472252184284187138, -6.472252184284199572 ) ) ;
#1771=CARTESIAN_POINT ( 'NONE',  ( -77.55640685876514340, -14.66025389215425712, -16.63820144330994566 ) ) ;
#1773=CARTESIAN_POINT ( 'NONE',  ( -93.01741312761159008, -20.50009083235103446, -8.946232117463726041 ) ) ;
#1775=EDGE_CURVE ( 'NONE', #13725, #1634, #18127, .T. ) ;
#1776=CARTESIAN_POINT ( 'NONE',  ( 57.59792236341147031, -1.493297263419786540E-14, 2.435789363418160658 ) ) ;
#1779=AXIS2_PLACEMENT_3D ( 'NONE', #16083, #3998, #18078 ) ;
#1780=FACE_OUTER_BOUND ( 'NONE', #14683, .T. ) ;
#1782=CARTESIAN_POINT ( 'NONE',  ( -151.4802849345942093, 11.09498666340387096, 33.96623543969244707 ) ) ;
#1783=CARTESIAN_POINT ( 'NONE',  ( 5.823571940223073895, -24.75780943188384242, -44.77584346942393267 ) ) ;
#1784=CARTESIAN_POINT ( 'NONE',  ( -280.0000000000000568, -42.42640687119305198, 14.14213562373058686 ) ) ;
#1785=CARTESIAN_POINT ( 'NONE',  ( -86.94949953272053733, -19.08279132442580561, 9.637191076868178996 ) ) ;
#1786=CARTESIAN_POINT ( 'NONE',  ( -86.96347745069644475, -12.89780903124413491, 12.89780903124398037 ) ) ;
#1787=CARTESIAN_POINT ( 'NONE',  ( -100.7734535825088358, -2.560096224687585342E-13, 22.67402823373191723 ) ) ;
#1788=FACE_OUTER_BOUND ( 'NONE', #17941, .T. ) ;
#1789=CARTESIAN_POINT ( 'NONE',  ( -213.1075012329537230, 18.58567234101174037, -37.98287015391222354 ) ) ;
#1790=CARTESIAN_POINT ( 'NONE',  ( 151.7948205124836250, -6.767089262349004208, -2.449293598294708485E-15 ) ) ;
#1791=DIRECTION ( 'NONE',  ( 1.000000000000000000, 1.836970198721030181E-16, 0.000000000000000000 ) ) ;
#1792=CARTESIAN_POINT ( 'NONE',  ( -192.9588430854690273, -54.46834944098226572, 40.00000000000002132 ) ) ;
#1793=CARTESIAN_POINT ( 'NONE',  ( -105.3209481228352615, 10.91022678754919006, 18.42900430629945774 ) ) ;
#1794=CARTESIAN_POINT ( 'NONE',  ( 0.2972598230769956662, 40.00000000000058975, -54.33493731733894094 ) ) ;
#1795=CARTESIAN_POINT ( 'NONE',  ( -238.4067589809705794, 0.6820004457912757223, 0.6820004457913219076 ) ) ;
#1796=CARTESIAN_POINT ( 'NONE',  ( -30.26275506840324070, 1.694272468446254232, 0.000000000000000000 ) ) ;
#1798=CARTESIAN_POINT ( 'NONE',  ( 22.89778847645078486, -43.13990468001248502, 17.86913359794352019 ) ) ;
#1800=CARTESIAN_POINT ( 'NONE',  ( 140.2235668266256425, 12.60094438999802868, 30.42137084504315325 ) ) ;
#1801=CARTESIAN_POINT ( 'NONE',  ( 192.4448373802101173, 42.42640687116508502, -14.14213562375874567 ) ) ;
#1802=CARTESIAN_POINT ( 'NONE',  ( -238.4067589809705794, -40.00000000000021316, 40.96449427990166470 ) ) ;
#1803=CARTESIAN_POINT ( 'NONE',  ( -162.0762913951021176, 29.48230308784730980, 27.08623940707652622 ) ) ;
#1804=CARTESIAN_POINT ( 'NONE',  ( 199.9999999999999432, -1.727494763561684666E-13, 20.00000000000010303 ) ) ;
#1805=CARTESIAN_POINT ( 'NONE',  ( -238.4067589809705794, 0.9644942799825386714, 0.000000000000000000 ) ) ;
#1809=CARTESIAN_POINT ( 'NONE',  ( -198.0356074513804572, 67.44298959250878056, -10.87444709758402261 ) ) ;
#1810=CARTESIAN_POINT ( 'NONE',  ( 130.8568914410475372, -4.207082182992785135, -4.207082182992884611 ) ) ;
#1811=CARTESIAN_POINT ( 'NONE',  ( -110.0913210856344904, 19.97012681669859191, -3.048699489023670495 ) ) ;
#1812=CARTESIAN_POINT ( 'NONE',  ( -87.05569247516073972, 17.94468678732786060, -11.73639047247175604 ) ) ;
#1813=CARTESIAN_POINT ( 'NONE',  ( -91.56559293963834989, -40.53558337403692491, 16.03295912088671571 ) ) ;
#1814=CARTESIAN_POINT ( 'NONE',  ( 130.8568914410475372, -4.207082182992785135, -4.207082182992884611 ) ) ;
#1815=CARTESIAN_POINT ( 'NONE',  ( 192.4448373802100889, -14.14213562375896061, 14.14213562375865330 ) ) ;
#1816=CARTESIAN_POINT ( 'NONE',  ( 4.995406935893294431, -17.50105314357144337, -39.06748935135212264 ) ) ;
#1817=CARTESIAN_POINT ( 'NONE',  ( 146.6084372240433993, -34.62501878078303008, 0.000000000000000000 ) ) ;
#1821=CARTESIAN_POINT ( 'NONE',  ( -105.3755690713226585, -40.00000000000010658, 18.24025645688337249 ) ) ;
#1822=CARTESIAN_POINT ( 'NONE',  ( 146.6084372240433709, 52.76785682606519146, 3.800685668858932775 ) ) ;
#1824=CARTESIAN_POINT ( 'NONE',  ( 19.06497207195980792, 14.19242893257840699, 40.00000000000002132 ) ) ;
#1826=CARTESIAN_POINT ( 'NONE',  ( 170.2234770963711128, -17.36149277826985937, -17.36149277826995174 ) ) ;
#1827=ADVANCED_FACE ( 'NONE', ( #11882 ), #11690, .T. ) ;
#1828=CARTESIAN_POINT ( 'NONE',  ( 14.63649358215962515, 43.53262337840171625, 18.03180300901562916 ) ) ;
#1829=CARTESIAN_POINT ( 'NONE',  ( 59.93546481434775330, 13.19882033562931056, 31.86477106141393989 ) ) ;
#1830=CARTESIAN_POINT ( 'NONE',  ( -105.2054292635175585, -2.444554031225951202E-13, 21.49321519473985020 ) ) ;
#1831=ADVANCED_FACE ( 'NONE', ( #1788 ), #23328, .T. ) ;
#1833=CARTESIAN_POINT ( 'NONE',  ( -200.4317933031570647, -44.88237357214666901, 24.83634732651998789 ) ) ;
#1835=CARTESIAN_POINT ( 'NONE',  ( 19.66474694216432795, -18.18658454057326068, 43.90629905113207343 ) ) ;
#1836=CARTESIAN_POINT ( 'NONE',  ( 22.76838195347366067, 17.88421977190837708, -43.17632592580126527 ) ) ;
#1839=CARTESIAN_POINT ( 'NONE',  ( -184.9730489280271684, -13.59277546673063952, 45.83721239345848630 ) ) ;
#1840=CARTESIAN_POINT ( 'NONE',  ( 200.0000000000000000, 42.42640687119267540, 14.14213562373153543 ) ) ;
#1841=CARTESIAN_POINT ( 'NONE',  ( 4.995406935893309530, -55.24977328856464709, 40.00000000000002132 ) ) ;
#1842=CARTESIAN_POINT ( 'NONE',  ( -188.9478905404506577, 17.94277290414884973, -43.31768569177498307 ) ) ;
#1843=CARTESIAN_POINT ( 'NONE',  ( 136.1360204305621266, -24.77266263493151044, 24.77266263493093135 ) ) ;
#1844=CARTESIAN_POINT ( 'NONE',  ( -199.9999999999998579, 24.82633483071252201, 44.86878812508700776 ) ) ;
#1845=CARTESIAN_POINT ( 'NONE',  ( 163.1118516004056573, 27.26290988616875310, 0.000000000000000000 ) ) ;
#1846=CARTESIAN_POINT ( 'NONE',  ( 170.2234770963711128, -24.55285855007183926, 0.000000000000000000 ) ) ;
#1847=CARTESIAN_POINT ( 'NONE',  ( 146.6084372240433993, 8.568076647504290689E-14, -5.374981219216972583 ) ) ;
#1848=CARTESIAN_POINT ( 'NONE',  ( -30.26275506840324070, 1.198031551615912571, 57.76657404653985139 ) ) ;
#1849=EDGE_CURVE ( 'NONE', #25714, #12267, #18484, .T. ) ;
#1853=CARTESIAN_POINT ( 'NONE',  ( -30.26275506840324070, 1.198031551616013601, 1.198031551616023371 ) ) ;
#1854=B_SPLINE_CURVE_WITH_KNOTS ( 'NONE', 3,
 ( #21166, #21417, #23291, #17030, #5442, #1199, #15412, #2939, #814, #7049, #11049, #7170, #9053, #19160, #17535, #21294, #1068, #945, #19537, #21669, #17158, #11170, #3445, #19285, #9177, #8920, #11298, #17288, #3189, #15287, #25422, #11541, #9304, #17410, #5309, #13420, #21543, #3317, #1323, #9428, #1452, #18062, #10088 ),
 .UNSPECIFIED., .F., .F.,
 ( 4, 2, 2, 2, 2, 2, 2, 2, 2, 2, 2, 2, 2, 2, 2, 2, 2, 2, 1, 1, 1, 2, 4 ),
 ( 0.03014611463440037761, 0.03932844241433864491, 0.04391960630430777335, 0.04506739727680003638, 0.04621518824929229941, 0.04851077019427690873, 0.05310193408424610656, 0.05539751602923075058, 0.05769309797421538766, 0.06228426186418467569, 0.06687542575415394985, 0.06917100769913860081, 0.07146658964412323789, 0.07376217158910787497, 0.07605775353409251205, 0.08524008131403096322, 0.09442240909396941440, 0.09901357298393861917, 0.1013091549289232424, 0.1024569459014155609, 0.1030308413876617202, 0.1033177891307847929, 0.1036047368739078656 ),
 .UNSPECIFIED. ) ;
#1855=CARTESIAN_POINT ( 'NONE',  ( -162.0762913951020892, -1.694272876828353702, 0.000000000000000000 ) ) ;
#1856=CARTESIAN_POINT ( 'NONE',  ( -89.91498783732212985, -8.087768383116706872, 20.43892340025324117 ) ) ;
#1858=VERTEX_POINT ( 'NONE', #17248 ) ;
#1859=ORIENTED_EDGE ( 'NONE', *, *, #18389, .T. ) ;
#1860=CARTESIAN_POINT ( 'NONE',  ( -135.8532207217289738, -21.81201906317758343, -34.75652343174620995 ) ) ;
#1861=CARTESIAN_POINT ( 'NONE',  ( 45.01779936602802223, -36.09695843547836347, -18.90344565818509537 ) ) ;
#1864=CARTESIAN_POINT ( 'NONE',  ( 14.38125909742180752, 15.17850393972634038, -40.00000000000002132 ) ) ;
#1869=CARTESIAN_POINT ( 'NONE',  ( 184.8905102610680444, 13.49065550809817715, -43.07788698682574591 ) ) ;
#1870=CARTESIAN_POINT ( 'NONE',  ( -188.8842637254079193, -43.30125340596319461, -17.93596642850435785 ) ) ;
#1871=CARTESIAN_POINT ( 'NONE',  ( 19.06497207195981858, -40.00000000000007105, 14.19242893257826665 ) ) ;
#1872=CARTESIAN_POINT ( 'NONE',  ( -135.8532207217289738, -9.153146818113595984, 40.00000000000002132 ) ) ;
#1875=CARTESIAN_POINT ( 'NONE',  ( 19.06497207195981147, -4.605042221739098431E-14, 14.19242893257840521 ) ) ;
#1876=CARTESIAN_POINT ( 'NONE',  ( 146.6084372240433709, -40.00000000000036238, 34.62501878078263218 ) ) ;
#1877=CARTESIAN_POINT ( 'NONE',  ( -199.9999999999999716, -44.89135967046717468, -23.83302776610000961 ) ) ;
#1878=CARTESIAN_POINT ( 'NONE',  ( -280.0000000000000568, 14.14213562373067745, 42.42640687119295251 ) ) ;
#1879=CARTESIAN_POINT ( 'NONE',  ( -56.48582580120559982, -21.81201906317755501, -34.75652343174621706 ) ) ;
#1882=CARTESIAN_POINT ( 'NONE',  ( 151.7948205124836250, -3.202120068677277203E-13, 33.23291073765553705 ) ) ;
#1883=CARTESIAN_POINT ( 'NONE',  ( -86.96347745069644475, 5.999880687339585546E-14, -21.75974354311649961 ) ) ;
#1884=CARTESIAN_POINT ( 'NONE',  ( 57.59792236341147031, 26.56190807104684382, 26.56190807104692553 ) ) ;
#1885=CARTESIAN_POINT ( 'NONE',  ( 14.38125909742181818, -39.01709431150928253, 17.55144818341435808 ) ) ;
#1886=CARTESIAN_POINT ( 'NONE',  ( -191.2490444017885522, -18.16428715638061675, -43.85246840378096067 ) ) ;
#1887=CARTESIAN_POINT ( 'NONE',  ( 136.1360204305621266, -3.419521671106983309E-13, 35.03383547441296741 ) ) ;
#1889=CARTESIAN_POINT ( 'NONE',  ( -91.56559293963834989, -44.31723036834885932, -12.25131212657538171 ) ) ;
#1891=CARTESIAN_POINT ( 'NONE',  ( -114.5450021253300861, -6.791646844855799614, 20.85732849908779940 ) ) ;
#1892=CARTESIAN_POINT ( 'NONE',  ( -105.3755690713226869, 21.75974354311648540, -0.000000000000000000 ) ) ;
#1893=DIRECTION ( 'NONE',  ( 0.01051738792036196329, 0.9166396752537513404, 0.3995761383041158132 ) ) ;
#1894=CARTESIAN_POINT ( 'NONE',  ( -105.3755690713226585, -15.38646221621738164, -41.18208027870615240 ) ) ;
#1896=CARTESIAN_POINT ( 'NONE',  ( -77.58513204268632535, 2.423266694375444619, 21.97516623138666603 ) ) ;
#1899=CARTESIAN_POINT ( 'NONE',  ( -105.2334157265389507, -16.99665894158227175, 13.14152336620594141 ) ) ;
#1900=CARTESIAN_POINT ( 'NONE',  ( 1.925538622541579148, 14.07631154915297778, 48.64880301060233592 ) ) ;
#1902=VERTEX_POINT ( 'NONE', #9516 ) ;
#1904=CARTESIAN_POINT ( 'NONE',  ( -86.96347745069644475, -21.75974354311651737, 0.000000000000000000 ) ) ;
#1906=CARTESIAN_POINT ( 'NONE',  ( -192.1131137119205903, -43.98782916596421444, 24.17676406461175631 ) ) ;
#1908=CARTESIAN_POINT ( 'NONE',  ( -94.58360650945819259, -8.190527749723793605, -20.91945674500546559 ) ) ;
#1909=CARTESIAN_POINT ( 'NONE',  ( -192.9588430854689989, 1.161019517985663313E-13, -14.46834944099969533 ) ) ;
#1911=CARTESIAN_POINT ( 'NONE',  ( -83.21262154144253032, -13.72187187061456015, -33.12752917118434226 ) ) ;
#1913=CARTESIAN_POINT ( 'NONE',  ( -196.2219207559400047, 43.48224904004372604, 18.01093727487041107 ) ) ;
#1914=CARTESIAN_POINT ( 'NONE',  ( -4.915070467874963711, -13.76630780994289438, -46.68718905935000407 ) ) ;
#1915=CARTESIAN_POINT ( 'NONE',  ( -100.7734535825088358, -12.25131212657475643, -12.25131212657495539 ) ) ;
#1917=CARTESIAN_POINT ( 'NONE',  ( 136.1360204305621266, -3.511608612530379592, -53.05693388239318153 ) ) ;
#1918=CARTESIAN_POINT ( 'NONE',  ( 0.2972598230770030492, -39.99999999999987210, -14.33493731733975451 ) ) ;
#1919=CARTESIAN_POINT ( 'NONE',  ( -105.3755690713226727, 15.38646221621771737, 15.38646221621800514 ) ) ;
#1920=CARTESIAN_POINT ( 'NONE',  ( -259.2033419157646676, -30.48217210827744239, -2.449293598294708485E-15 ) ) ;
#1922=CARTESIAN_POINT ( 'NONE',  ( 146.6084372240433709, -5.374981219216942385, -40.00000000000002132 ) ) ;
#1923=CARTESIAN_POINT ( 'NONE',  ( -94.58366989427231886, 20.91926462023913658, -8.190486896678999429 ) ) ;
#1924=CARTESIAN_POINT ( 'NONE',  ( 184.8905102610680444, 40.00000000000025580, -19.07866798485515503 ) ) ;
#1925=CARTESIAN_POINT ( 'NONE',  ( 91.82158438592158234, -12.16597498397761967, -12.16597498397768007 ) ) ;
#1927=CARTESIAN_POINT ( 'NONE',  ( -105.3755690713226727, -21.75974354311652093, 0.000000000000000000 ) ) ;
#1929=EDGE_CURVE ( 'NONE', #15177, #10228, #3634, .T. ) ;
#1931=CARTESIAN_POINT ( 'NONE',  ( 14.38125909742180752, 15.17850393972634038, 40.00000000000002132 ) ) ;
#1932=CARTESIAN_POINT ( 'NONE',  ( -83.21262154144250189, -13.72187187061479641, 33.12752917118422857 ) ) ;
#1933=CARTESIAN_POINT ( 'NONE',  ( -135.8532207217289738, -40.00000000000014921, 30.84685318188631697 ) ) ;
#1935=CARTESIAN_POINT ( 'NONE',  ( -91.56559293963834989, 12.25131212657428748, 44.31723036834913643 ) ) ;
#1936=CARTESIAN_POINT ( 'NONE',  ( 57.59792236341147031, -2.435789363418150444, 0.000000000000000000 ) ) ;
#1937=CARTESIAN_POINT ( 'NONE',  ( 91.82158438592158234, -17.20528682183298486, 0.000000000000000000 ) ) ;
#1938=CARTESIAN_POINT ( 'NONE',  ( 169.9999999999999716, 22.62041470344888339, -9.369682556672254137 ) ) ;
#1941=CARTESIAN_POINT ( 'NONE',  ( 19.06497207195980792, 66.60410523465830579, -10.03556273973354251 ) ) ;
#1942=CARTESIAN_POINT ( 'NONE',  ( 4.995406935893305977, -39.06748935135157552, -39.06748935135225764 ) ) ;
#1944=CARTESIAN_POINT ( 'NONE',  ( -110.0687879519081918, 19.47486782027040775, 5.333724827205037933 ) ) ;
#1945=CARTESIAN_POINT ( 'NONE',  ( -77.56349232223030299, 14.64315958561415343, -16.60062240782661647 ) ) ;
#1946=CARTESIAN_POINT ( 'NONE',  ( 163.1118516004056573, -37.29075403953166301, 19.27778845539196695 ) ) ;
#1947=CARTESIAN_POINT ( 'NONE',  ( 57.59792236341147031, -1.722363176415055985, 1.722363176415024677 ) ) ;
#1948=CARTESIAN_POINT ( 'NONE',  ( 192.4448373802101173, -42.42640687122053578, -14.14213562370360577 ) ) ;
#1949=CARTESIAN_POINT ( 'NONE',  ( 91.82158438592158234, 12.16597498397773869, -12.16597498397759303 ) ) ;
#1952=CARTESIAN_POINT ( 'NONE',  ( -100.7734535825088500, -39.99999999999995737, -22.67402823373205578 ) ) ;
#1953=CIRCLE ( 'NONE', #12143, 14.99999999999999467 ) ;
#1954=CARTESIAN_POINT ( 'NONE',  ( 192.4448373802100889, 14.14213562375873678, 14.14213562375894817 ) ) ;
#1956=CARTESIAN_POINT ( 'NONE',  ( 22.90311673802928993, 42.99920082299722424, -23.44499648834960936 ) ) ;
#1957=CARTESIAN_POINT ( 'NONE',  ( -238.4067589809705794, 40.96449428006337001, -40.00000000000002132 ) ) ;
#1958=ORIENTED_EDGE ( 'NONE', *, *, #4931, .F. ) ;
#1959=CARTESIAN_POINT ( 'NONE',  ( -259.2033419157646676, -9.517827891722680178, 0.000000000000000000 ) ) ;
#1960=CARTESIAN_POINT ( 'NONE',  ( -4.580761711674998793, -42.99740816077039796, 17.81010960708318791 ) ) ;
#1961=CARTESIAN_POINT ( 'NONE',  ( -259.2033419157646676, -9.517827891722680178, 40.00000000000002132 ) ) ;
#1965=CARTESIAN_POINT ( 'NONE',  ( -190.7345856380928524, -43.65254615100791113, 23.92884448222190841 ) ) ;
#1968=CARTESIAN_POINT ( 'NONE',  ( -2.164901439740674505, -23.84421257765607294, 43.53794903249384873 ) ) ;
#1969=CARTESIAN_POINT ( 'NONE',  ( 23.30336656375570215, 23.35569295765361986, -42.87878279885786270 ) ) ;
#1972=CARTESIAN_POINT ( 'NONE',  ( 0.2972598230769959993, 38.42060263243713081, -38.42060263243619289 ) ) ;
#1973=CARTESIAN_POINT ( 'NONE',  ( -198.0356074513804572, -15.37879056873074290, 0.000000000000000000 ) ) ;
#1974=CARTESIAN_POINT ( 'NONE',  ( -188.6890294954694980, 23.53287096354939223, -43.11788624870165876 ) ) ;
#1975=CARTESIAN_POINT ( 'NONE',  ( 146.6084372240433993, -24.48358557860353457, 24.48358557860296258 ) ) ;
#1977=CARTESIAN_POINT ( 'NONE',  ( 184.8905102610680444, 20.92133201514447194, -40.00000000000002132 ) ) ;
#1978=CARTESIAN_POINT ( 'NONE',  ( 19.06497207195980792, 54.19242893257844429, 40.00000000000002132 ) ) ;
#1979=CARTESIAN_POINT ( 'NONE',  ( -135.8532207217289738, -39.99999999999972289, -30.84685318188688541 ) ) ;
#1980=CARTESIAN_POINT ( 'NONE',  ( -208.1127848780264742, 67.17687982760683951, 10.60833733268317403 ) ) ;
#1983=CARTESIAN_POINT ( 'NONE',  ( 0.2972598230769923355, 18.14793986248751168, -38.42060263243650553 ) ) ;
#1985=CARTESIAN_POINT ( 'NONE',  ( -105.3755690713226585, -43.67073346367983788, 12.89780903124397149 ) ) ;
#1986=CARTESIAN_POINT ( 'NONE',  ( -190.1935165880707075, 47.62328200654632582, -13.92226094463961594 ) ) ;
#1990=CARTESIAN_POINT ( 'NONE',  ( 184.8905102610680444, -41.77492675555986779, -14.79361573936407304 ) ) ;
#1991=CARTESIAN_POINT ( 'NONE',  ( 23.41418334855293537, -46.79369727367380705, -13.79799959793995079 ) ) ;
#1993=CARTESIAN_POINT ( 'NONE',  ( 163.1118516004056573, 12.73709011382478806, -40.00000000000002132 ) ) ;
#1995=EDGE_LOOP ( 'NONE', ( #11759, #20286, #16388, #3299 ) ) ;
#1998=CARTESIAN_POINT ( 'NONE',  ( 130.8568914410475088, 4.207082182989741348, -52.36146031193420924 ) ) ;
#1999=CARTESIAN_POINT ( 'NONE',  ( -188.4702232936773214, -43.05505437950338177, -23.48628015402992020 ) ) ;
#2002=CARTESIAN_POINT ( 'NONE',  ( 14.38125909742181818, -40.00000000000007816, 15.17850393972619649 ) ) ;
#2003=CARTESIAN_POINT ( 'NONE',  ( -56.48582580120559271, -9.153146818113595984, 0.000000000000000000 ) ) ;
#2007=B_SPLINE_CURVE_WITH_KNOTS ( 'NONE', 3,
 ( #3756, #20254, #16384, #24517, #6276, #14391 ),
 .UNSPECIFIED., .F., .F.,
 ( 4, 2, 4 ),
 ( -5.998621905616971167E-08, 0.03937827992696036478, 0.07875661984013977712 ),
 .UNSPECIFIED. ) ;
#2008=CARTESIAN_POINT ( 'NONE',  ( 151.7948205124836250, 1.439163438361279259E-13, -33.23291073765553705 ) ) ;
#2009=CARTESIAN_POINT ( 'NONE',  ( 151.7948205124836250, 1.807796684091926154E-15, 6.767089262349031742 ) ) ;
#2010=CARTESIAN_POINT ( 'NONE',  ( 0.2972598230770103767, -39.99999999999945288, -54.33493731733979359 ) ) ;
#2011=CARTESIAN_POINT ( 'NONE',  ( 192.4448373802101173, 39.99999999999998579, 19.99999999996075317 ) ) ;
#2012=CARTESIAN_POINT ( 'NONE',  ( 57.59792236341147031, 2.435789363418171760, 0.000000000000000000 ) ) ;
#2013=CARTESIAN_POINT ( 'NONE',  ( -259.2033419157646676, 6.730120644403214669, 49.83842185052034068 ) ) ;
#2015=CARTESIAN_POINT ( 'NONE',  ( 91.82158438592156813, 17.20528682183302038, -40.00000000000002132 ) ) ;
#2017=CARTESIAN_POINT ( 'NONE',  ( -105.3755690713226585, -41.18208027870589660, -15.38646221621809040 ) ) ;
#2018=CARTESIAN_POINT ( 'NONE',  ( -94.58366989427226201, -9.000605044545805455, 20.58370269626814775 ) ) ;
#2020=CARTESIAN_POINT ( 'NONE',  ( -259.2033419157646676, -1.473088368616265084E-13, 9.517827891722632216 ) ) ;
#2021=CARTESIAN_POINT ( 'NONE',  ( 199.9999999999999432, -3.553951640073651008E-14, 19.99999999999992539 ) ) ;
#2022=CARTESIAN_POINT ( 'NONE',  ( -238.4067589809705794, 57.25054294077225592, 0.6820004458485544596 ) ) ;
#2023=CARTESIAN_POINT ( 'NONE',  ( -114.7731140143791038, 16.71335482098725578, 14.51162400671975305 ) ) ;
#2024=CARTESIAN_POINT ( 'NONE',  ( -188.2652746676664606, -23.44263257803881118, -42.99511404082397092 ) ) ;
#2025=CARTESIAN_POINT ( 'NONE',  ( -30.26275506840324070, -1.198031551616032919, 1.198031551616014712 ) ) ;
#2026=VERTEX_POINT ( 'NONE', #15496 ) ;
#2027=CARTESIAN_POINT ( 'NONE',  ( 14.38125909742180752, 10.73282306404735387, -10.73282306404708919 ) ) ;
#2028=CARTESIAN_POINT ( 'NONE',  ( -79.35537823250633949, 19.65633339167321481, 8.141919877358327895 ) ) ;
#2029=CARTESIAN_POINT ( 'NONE',  ( -192.9588430854690273, -14.46834944099973264, -40.00000000000002132 ) ) ;
#2031=CARTESIAN_POINT ( 'NONE',  ( 146.6084372240433709, -24.48358557860284179, -32.08495691632087699 ) ) ;
#2033=VERTEX_POINT ( 'NONE', #21629 ) ;
#2035=CARTESIAN_POINT ( 'NONE',  ( -105.3175882261749194, -18.50843658929550983, 10.85998092706852347 ) ) ;
#2036=CARTESIAN_POINT ( 'NONE',  ( -3.439026802540597672, 17.93765581402023557, 43.30533194338860881 ) ) ;
#2037=ORIENTED_EDGE ( 'NONE', *, *, #17908, .T. ) ;
#2039=CARTESIAN_POINT ( 'NONE',  ( -162.0762913951020892, 1.694272876828294194, 0.000000000000000000 ) ) ;
#2042=CARTESIAN_POINT ( 'NONE',  ( -162.0762913951020892, 1.198031840385716418, 1.198031840385750169 ) ) ;
#2043=CARTESIAN_POINT ( 'NONE',  ( -102.4294859496168755, -8.407280617747138862, -20.29697089062620918 ) ) ;
#2044=CARTESIAN_POINT ( 'NONE',  ( 184.8905102610680444, -1.851754852062639767E-13, 20.92133201514444352 ) ) ;
#2046=CARTESIAN_POINT ( 'NONE',  ( -86.95455603114054099, -20.33687888584654857, -6.703476574496026963 ) ) ;
#2047=CARTESIAN_POINT ( 'NONE',  ( -109.1264249741455643, -33.12752917268982600, 13.72187187124576191 ) ) ;
#2050=CARTESIAN_POINT ( 'NONE',  ( 8.273828130702915118, -18.58906013839226645, -44.87796109789693588 ) ) ;
#2051=CARTESIAN_POINT ( 'NONE',  ( 163.1118516004056573, 19.27778845539265618, -37.29075403953135037 ) ) ;
#2052=CARTESIAN_POINT ( 'NONE',  ( -114.7826396787039727, 1.385190677998766828, -22.13135001985627426 ) ) ;
#2053=CARTESIAN_POINT ( 'NONE',  ( -198.0356074513804572, -67.44298959250878056, 10.87444709758448447 ) ) ;
#2055=CARTESIAN_POINT ( 'NONE',  ( -238.4067589809705794, -0.6820004457913585449, -0.6820004457913265705 ) ) ;
#2057=CARTESIAN_POINT ( 'NONE',  ( -192.9588430854689705, -54.46834944099975928, -2.449293598294708485E-15 ) ) ;
#2058=CARTESIAN_POINT ( 'NONE',  ( -259.2033419157646676, -6.730120644403663199, 6.730120644403451813 ) ) ;
#2059=CARTESIAN_POINT ( 'NONE',  ( 192.4448373802101173, -19.99999999996056843, -40.00000000000002132 ) ) ;
#2060=CARTESIAN_POINT ( 'NONE',  ( -105.3330350205445143, 18.67663213883233908, 10.55153823230807397 ) ) ;
#2061=CARTESIAN_POINT ( 'NONE',  ( -192.9588430854690273, 40.00000000000014211, -14.46834944099927966 ) ) ;
#2062=CARTESIAN_POINT ( 'NONE',  ( -135.8532207217289738, -6.472252184284190690, -6.472252184284188914 ) ) ;
#2063=CARTESIAN_POINT ( 'NONE',  ( -259.2033419157646676, -9.517827891722680178, 0.000000000000000000 ) ) ;
#2066=CARTESIAN_POINT ( 'NONE',  ( 200.0000000000000000, -20.00000000000006750, 40.00000000000002132 ) ) ;
#2067=CARTESIAN_POINT ( 'NONE',  ( -94.58366989427226201, -8.190486896679201934, -20.91926462023907263 ) ) ;
#2068=CARTESIAN_POINT ( 'NONE',  ( 192.4448373802101173, -40.00000000000005684, 19.99999999996046185 ) ) ;
#2069=CARTESIAN_POINT ( 'NONE',  ( 91.82158438592158234, 44.40256751092319121, 12.16597498400105515 ) ) ;
#2070=FACE_OUTER_BOUND ( 'NONE', #16181, .T. ) ;
#2075=CARTESIAN_POINT ( 'NONE',  ( -259.2033419157646676, -6.730120644402966867, -49.83842185052038332 ) ) ;
#2076=CARTESIAN_POINT ( 'NONE',  ( -192.9588430854690273, -38.51493924976957572, 18.05360324515410397 ) ) ;
#2078=CARTESIAN_POINT ( 'NONE',  ( 4.995406935893290878, 1.606505379428369110E-13, -15.24977328854832592 ) ) ;
#2079=CARTESIAN_POINT ( 'NONE',  ( 0.2972598230770153171, -66.70487387989849992, -10.13633138497533004 ) ) ;
#2080=ADVANCED_FACE ( 'NONE', ( #23626 ), #8039, .T. ) ;
#2082=CARTESIAN_POINT ( 'NONE',  ( -192.9588430854690273, -66.79921049724377724, 10.23066800231950069 ) ) ;
#2086=CARTESIAN_POINT ( 'NONE',  ( -238.4067589809705794, -1.892706720741712928E-13, 40.96449427998260973 ) ) ;
#2088=CARTESIAN_POINT ( 'NONE',  ( 20.17262239840771088, 43.80323544016827242, -18.14389419515791246 ) ) ;
#2089=CARTESIAN_POINT ( 'NONE',  ( 0.2972598230769930017, 54.33493731733938148, -40.00000000000002132 ) ) ;
#2091=CARTESIAN_POINT ( 'NONE',  ( -198.0356074513804572, 15.37879056873067007, 0.000000000000000000 ) ) ;
#2092=CARTESIAN_POINT ( 'NONE',  ( -6.342283169552854538, -46.19215417244088684, 13.66521761902479248 ) ) ;
#2093=CARTESIAN_POINT ( 'NONE',  ( 91.82158438592158234, -17.20528682183298486, 40.00000000000002132 ) ) ;
#2095=CARTESIAN_POINT ( 'NONE',  ( -188.2995950289364941, -46.99046209955426434, -13.82811170417247126 ) ) ;
#2097=CARTESIAN_POINT ( 'NONE',  ( -3.117754532603109308, -17.97158175134531533, 43.38723640139177462 ) ) ;
#2099=CARTESIAN_POINT ( 'NONE',  ( -4.076660308449107539, 13.82548859978937550, -46.97758120990494035 ) ) ;
#2101=CARTESIAN_POINT ( 'NONE',  ( 85.88498456125454084, -23.37206003943197175, 8.769910163431326566 ) ) ;
#2103=CARTESIAN_POINT ( 'NONE',  ( -144.0562696877088626, -10.50947022284602994, 31.27040355063070365 ) ) ;
#2104=CARTESIAN_POINT ( 'NONE',  ( -198.0356074513804572, 39.15871834505956173, -39.15871834505865223 ) ) ;
#2105=CARTESIAN_POINT ( 'NONE',  ( 170.0000000000000000, 24.95097643317004454, 3.062538285713123809 ) ) ;
#2106=CARTESIAN_POINT ( 'NONE',  ( -189.0115661350385494, 17.94954792649267716, -43.33404204260362746 ) ) ;
#2107=CARTESIAN_POINT ( 'NONE',  ( -238.4067589809705794, 28.96627169325285678, 27.60227080167094726 ) ) ;
#2109=CARTESIAN_POINT ( 'NONE',  ( -280.0000000000000568, -20.00000000000007105, 40.00000000000002132 ) ) ;
#2110=CARTESIAN_POINT ( 'NONE',  ( -259.2033419157646676, 30.48217210827735713, -40.00000000000002132 ) ) ;
#2111=CARTESIAN_POINT ( 'NONE',  ( -280.0000000000000000, -2.609240458947769655E-13, 20.00000000000001421 ) ) ;
#2112=CARTESIAN_POINT ( 'NONE',  ( 0.2972598230769907257, 66.70487387989857098, 10.13633138497486641 ) ) ;
#2113=CARTESIAN_POINT ( 'NONE',  ( 98.29820294270298575, 18.47759065022021474, -7.653668647299666894 ) ) ;
#2114=CARTESIAN_POINT ( 'NONE',  ( 184.8905102610680444, -13.49065550809791603, -13.49065550809818781 ) ) ;
#2115=ORIENTED_EDGE ( 'NONE', *, *, #11409, .F. ) ;
#2116=CARTESIAN_POINT ( 'NONE',  ( -208.1127848780264742, -17.67593391476659548, 38.89260858015730804 ) ) ;
#2121=CARTESIAN_POINT ( 'NONE',  ( -259.2033419157646676, -49.83842185052031937, -6.730120644403796426 ) ) ;
#2122=CARTESIAN_POINT ( 'NONE',  ( 23.30336656375535398, -46.83484695576522228, -13.80490921643035307 ) ) ;
#2124=CARTESIAN_POINT ( 'NONE',  ( -56.48582580120559982, 30.84685318188643777, -40.00000000000002132 ) ) ;
#2130=CARTESIAN_POINT ( 'NONE',  ( 14.38125909742180220, 39.01709431150916885, -17.55144818341463164 ) ) ;
#2131=CARTESIAN_POINT ( 'NONE',  ( -188.8948648269077921, -43.30399732969039661, -17.93710299892621052 ) ) ;
#2132=CARTESIAN_POINT ( 'NONE',  ( -238.4067589809705794, -40.00000000000007105, 0.9644942799824426372 ) ) ;
#2133=CARTESIAN_POINT ( 'NONE',  ( 130.8568914410475088, -34.05028731879786363, 40.00000000000002132 ) ) ;
#2136=CARTESIAN_POINT ( 'NONE',  ( -100.7734535825088358, 6.065416334915073333E-14, -22.67402823373191723 ) ) ;
#2137=CARTESIAN_POINT ( 'NONE',  ( 57.59792236341149163, -40.00000000000014211, 37.56421063658172699 ) ) ;
#2138=CARTESIAN_POINT ( 'NONE',  ( -91.56559293963834989, 6.234561990864368500E-14, -22.67402823373191723 ) ) ;
#2140=CARTESIAN_POINT ( 'NONE',  ( 19.06497207195982924, -66.60410523465823474, 10.03556273973400081 ) ) ;
#2141=CARTESIAN_POINT ( 'NONE',  ( -238.4067589809705794, -0.9644942799826262680, 0.000000000000000000 ) ) ;
#2142=CARTESIAN_POINT ( 'NONE',  ( -105.3755690713226585, 15.38646221621762678, 41.18208027870604582 ) ) ;
#2145=CARTESIAN_POINT ( 'NONE',  ( -1.258540240222666418, -47.88180740053034157, 13.96099832920793737 ) ) ;
#2146=CARTESIAN_POINT ( 'NONE',  ( 163.1118516004056573, -2.556006622855449647E-13, 27.26290988616872824 ) ) ;
#2147=CARTESIAN_POINT ( 'NONE',  ( 57.59792236341147742, -1.230234673553095937E-13, 37.56421063658186199 ) ) ;
#2148=CARTESIAN_POINT ( 'NONE',  ( -105.3755690713226585, 41.18208027870598187, -15.38646221621779731 ) ) ;
#2149=CARTESIAN_POINT ( 'NONE',  ( -114.6238578290137724, 19.10716134690576595, 10.97953394730984478 ) ) ;
#2150=CARTESIAN_POINT ( 'NONE',  ( -190.5535808404531508, -18.10342626499672036, -43.70553721438312778 ) ) ;
#2151=CARTESIAN_POINT ( 'NONE',  ( -56.48582580120558561, -21.81201906317785699, 21.81201906317761896 ) ) ;
#2153=CARTESIAN_POINT ( 'NONE',  ( -100.7734535825088358, -16.03295912088728770, 16.03295912088687913 ) ) ;
#2155=CARTESIAN_POINT ( 'NONE',  ( 184.8905102610680444, 20.92133201514447549, 0.000000000000000000 ) ) ;
#2156=ADVANCED_FACE ( 'NONE', ( #21760 ), #12275, .T. ) ;
#2157=( BOUNDED_SURFACE ( )  B_SPLINE_SURFACE ( 3, 3, ( 
 ( #5865, #2020, #20371, #7713, #4015, #3881, #1617, #18223, #15824, #12115, #13971, #8121, #10122, #6130, #19966, #10, #16238, #13833, #24367, #14112, #23954, #9724, #13708, #21968, #1882, #2146, #20105, #9986, #5601, #19831 ),
 ( #3602, #15965, #3740, #7843, #1747, #7981, #18097, #11711, #9855, #24231, #4154, #6004, #21833, #22378, #20239, #17694, #12249, #7583, #15695, #23819, #4285, #16761, #6784, #24764, #4674, #22507, #2681, #6387, #12776, #4545 ),
 ( #21030, #22765, #2406, #18898, #22634, #6650, #20631, #22895, #8653, #14765, #16899, #14374, #18365, #20903, #12643, #8517, #14503, #20768, #2538, #145, #10383, #10516, #16504, #14896, #18630, #10656, #413, #25031, #6261, #10788 ),
 ( #23036, #4409, #18765, #24629, #12503, #4811, #16635, #6517, #8249, #10256, #16366, #677, #14628, #549, #12913, #8786, #24500, #24895, #12374, #20502, #2274, #18494, #274, #8382, #8918, #7418, #19284, #13046, #13294, #23661 ),
 ( #1067, #7047, #21415, #15285, #19033, #2937, #3066, #9051, #25672, #11168, #5192, #13171, #17534, #25163, #5307, #21542, #812, #6914, #15031, #13542, #942, #15533, #17287, #17027, #5441, #17156, #5065, #23536, #3188, #3316 ),
 ( #25549, #15411, #2812, #13419, #23161, #10921, #9303, #9427, #23289, #4940, #21164, #17407, #7169, #11047, #23416, #19158, #11296, #9174, #25421, #11414, #25290, #15164, #7297, #19414, #21292, #19536, #1198, #1322, #9823, #12080 ),
 ( #15924, #3844, #7808, #9551, #11810, #5833, #23787, #19664, #13936, #26212, #15661, #9952, #19796, #11540, #1713, #3568, #22071, #10087, #7549, #19930, #21796, #3708, #7679, #11948, #20073, #5568, #15791, #25937, #8084, #11672 ) ),
 .UNSPECIFIED., .T., .F., .F. ) 
 B_SPLINE_SURFACE_WITH_KNOTS ( ( 4, 3, 4 ),
 ( 4, 2, 2, 2, 2, 2, 2, 2, 2, 2, 2, 2, 2, 2, 4 ),
 ( 0.000000000000000000, 0.5000000000000000000, 1.000000000000000000 ),
 ( 0.000000000000000000, 0.1357259735107005372, 0.1651108541090157700, 0.1944957347073310028, 0.3598804999793158710, 0.3867117631979620773, 0.4135430264166082281, 0.5789277916885930964, 0.6062785021374117456, 0.6336292125862302838, 0.8508620842112317728, 0.8814014469398914198, 0.9119408096685510667, 0.9559704048342755334, 1.000000000000000000 ),
 .UNSPECIFIED. ) 
 GEOMETRIC_REPRESENTATION_ITEM ( )  RATIONAL_B_SPLINE_SURFACE ( (
 ( 1.000000000000000000, 1.000000000000000000, 1.000000000000000000, 1.000000000000000000, 1.000000000000000000, 1.000000000000000000, 1.000000000000000000, 1.000000000000000000, 1.000000000000000000, 1.000000000000000000, 1.000000000000000000, 1.000000000000000000, 1.000000000000000000, 1.000000000000000000, 1.000000000000000000, 1.000000000000000000, 1.000000000000000000, 1.000000000000000000, 1.000000000000000000, 1.000000000000000000, 1.000000000000000000, 1.000000000000000000, 1.000000000000000000, 1.000000000000000000, 1.000000000000000000, 1.000000000000000000, 1.000000000000000000, 1.000000000000000000, 1.000000000000000000, 1.000000000000000000),
 ( 0.3333333333333333703, 0.3333333333333333703, 0.3333333333333333703, 0.3333333333333333703, 0.3333333333333333703, 0.3333333333333333703, 0.3333333333333333703, 0.3333333333333333703, 0.3333333333333333703, 0.3333333333333333703, 0.3333333333333333703, 0.3333333333333333703, 0.3333333333333333703, 0.3333333333333333703, 0.3333333333333333703, 0.3333333333333333703, 0.3333333333333333703, 0.3333333333333333703, 0.3333333333333333703, 0.3333333333333333703, 0.3333333333333333703, 0.3333333333333333703, 0.3333333333333333703, 0.3333333333333333703, 0.3333333333333333703, 0.3333333333333333703, 0.3333333333333333703, 0.3333333333333333703, 0.3333333333333333703, 0.3333333333333333703),
 ( 0.3333333333333333703, 0.3333333333333333703, 0.3333333333333333703, 0.3333333333333333703, 0.3333333333333333703, 0.3333333333333333703, 0.3333333333333333703, 0.3333333333333333703, 0.3333333333333333703, 0.3333333333333333703, 0.3333333333333333703, 0.3333333333333333703, 0.3333333333333333703, 0.3333333333333333703, 0.3333333333333333703, 0.3333333333333333703, 0.3333333333333333703, 0.3333333333333333703, 0.3333333333333333703, 0.3333333333333333703, 0.3333333333333333703, 0.3333333333333333703, 0.3333333333333333703, 0.3333333333333333703, 0.3333333333333333703, 0.3333333333333333703, 0.3333333333333333703, 0.3333333333333333703, 0.3333333333333333703, 0.3333333333333333703),
 ( 1.000000000000000000, 1.000000000000000000, 1.000000000000000000, 1.000000000000000000, 1.000000000000000000, 1.000000000000000000, 1.000000000000000000, 1.000000000000000000, 1.000000000000000000, 1.000000000000000000, 1.000000000000000000, 1.000000000000000000, 1.000000000000000000, 1.000000000000000000, 1.000000000000000000, 1.000000000000000000, 1.000000000000000000, 1.000000000000000000, 1.000000000000000000, 1.000000000000000000, 1.000000000000000000, 1.000000000000000000, 1.000000000000000000, 1.000000000000000000, 1.000000000000000000, 1.000000000000000000, 1.000000000000000000, 1.000000000000000000, 1.000000000000000000, 1.000000000000000000),
 ( 0.3333333333333333703, 0.3333333333333333703, 0.3333333333333333703, 0.3333333333333333703, 0.3333333333333333703, 0.3333333333333333703, 0.3333333333333333703, 0.3333333333333333703, 0.3333333333333333703, 0.3333333333333333703, 0.3333333333333333703, 0.3333333333333333703, 0.3333333333333333703, 0.3333333333333333703, 0.3333333333333333703, 0.3333333333333333703, 0.3333333333333333703, 0.3333333333333333703, 0.3333333333333333703, 0.3333333333333333703, 0.3333333333333333703, 0.3333333333333333703, 0.3333333333333333703, 0.3333333333333333703, 0.3333333333333333703, 0.3333333333333333703, 0.3333333333333333703, 0.3333333333333333703, 0.3333333333333333703, 0.3333333333333333703),
 ( 0.3333333333333333703, 0.3333333333333333703, 0.3333333333333333703, 0.3333333333333333703, 0.3333333333333333703, 0.3333333333333333703, 0.3333333333333333703, 0.3333333333333333703, 0.3333333333333333703, 0.3333333333333333703, 0.3333333333333333703, 0.3333333333333333703, 0.3333333333333333703, 0.3333333333333333703, 0.3333333333333333703, 0.3333333333333333703, 0.3333333333333333703, 0.3333333333333333703, 0.3333333333333333703, 0.3333333333333333703, 0.3333333333333333703, 0.3333333333333333703, 0.3333333333333333703, 0.3333333333333333703, 0.3333333333333333703, 0.3333333333333333703, 0.3333333333333333703, 0.3333333333333333703, 0.3333333333333333703, 0.3333333333333333703),
 ( 1.000000000000000000, 1.000000000000000000, 1.000000000000000000, 1.000000000000000000, 1.000000000000000000, 1.000000000000000000, 1.000000000000000000, 1.000000000000000000, 1.000000000000000000, 1.000000000000000000, 1.000000000000000000, 1.000000000000000000, 1.000000000000000000, 1.000000000000000000, 1.000000000000000000, 1.000000000000000000, 1.000000000000000000, 1.000000000000000000, 1.000000000000000000, 1.000000000000000000, 1.000000000000000000, 1.000000000000000000, 1.000000000000000000, 1.000000000000000000, 1.000000000000000000, 1.000000000000000000, 1.000000000000000000, 1.000000000000000000, 1.000000000000000000, 1.000000000000000000) ) ) 
 REPRESENTATION_ITEM ( '' )  SURFACE ( )  );
#2158=CARTESIAN_POINT ( 'NONE',  ( -87.13361725327075646, 15.19799821270843765, 15.19799821270837015 ) ) ;
#2159=CARTESIAN_POINT ( 'NONE',  ( -105.3755690713226727, -15.38646221621807619, 15.38646221621768362 ) ) ;
#2160=EDGE_LOOP ( 'NONE', ( #12063, #8625, #3993, #6401, #1324 ) ) ;
#2164=CARTESIAN_POINT ( 'NONE',  ( 3.774039766383602945, 18.47898247162966356, 44.61221010184721081 ) ) ;
#2167=EDGE_LOOP ( 'NONE', ( #7931, #12834, #17870, #16767 ) ) ;
#2168=CARTESIAN_POINT ( 'NONE',  ( -238.4067589809705794, 0.9644942799825386714, 0.000000000000000000 ) ) ;
#2170=CARTESIAN_POINT ( 'NONE',  ( -110.1017833367309890, -1.261434661933622303, -20.19517362623882306 ) ) ;
#2173=CARTESIAN_POINT ( 'NONE',  ( 48.46046611906923118, 37.63122027851007090, -11.89583623498074161 ) ) ;
#2175=CARTESIAN_POINT ( 'NONE',  ( 170.2234770963711128, 40.00000000000021316, -15.44714144992773797 ) ) ;
#2181=CARTESIAN_POINT ( 'NONE',  ( 11.28112952480041820, -18.58737866929310201, -44.87390167242637773 ) ) ;
#2182=CARTESIAN_POINT ( 'NONE',  ( 0.2972598230770153171, -66.70487387989849992, -10.13633138497533004 ) ) ;
#2183=CARTESIAN_POINT ( 'NONE',  ( -110.0368417077420418, 7.441767003006856562, -18.74474319002892031 ) ) ;
#2184=CARTESIAN_POINT ( 'NONE',  ( 170.2234770963711128, -39.20704971665379190, -17.36149277827012938 ) ) ;
#2185=CARTESIAN_POINT ( 'NONE',  ( -77.71518870763448206, 21.27450625603104939, 5.747100446277157104 ) ) ;
#2188=CARTESIAN_POINT ( 'NONE',  ( -238.4067589809705794, -40.96449428006345528, 40.00000000000002132 ) ) ;
#2189=CARTESIAN_POINT ( 'NONE',  ( 146.6084372240433993, 24.48358557860341733, -24.48358557860313311 ) ) ;
#2191=CARTESIAN_POINT ( 'NONE',  ( -213.1075012329536946, -53.71589010951918652, -2.449293598294708485E-15 ) ) ;
#2192=CARTESIAN_POINT ( 'NONE',  ( -105.2410663018207373, 17.15223596101294490, 12.91571364855967907 ) ) ;
#2194=CARTESIAN_POINT ( 'NONE',  ( -213.1075012329537230, 40.00000000000055422, -53.71589010953623244 ) ) ;
#2195=CARTESIAN_POINT ( 'NONE',  ( 0.2972598230769938343, 10.13633138497472252, 10.13633138497475628 ) ) ;
#2196=CARTESIAN_POINT ( 'NONE',  ( -86.96347745069644475, -21.75974354311651737, 0.000000000000000000 ) ) ;
#2197=ORIENTED_EDGE ( 'NONE', *, *, #2296, .F. ) ;
#2199=CARTESIAN_POINT ( 'NONE',  ( 14.38125909742180752, 15.17850393972634038, 0.000000000000000000 ) ) ;
#2200=CARTESIAN_POINT ( 'NONE',  ( -188.2995950289364089, -23.44932284465861727, -43.00522595870986464 ) ) ;
#2202=CARTESIAN_POINT ( 'NONE',  ( -280.0000000000000568, 42.42640687119265408, 14.14213562373147504 ) ) ;
#2203=CARTESIAN_POINT ( 'NONE',  ( -192.9588430854689989, 14.46834944099965981, 0.000000000000000000 ) ) ;
#2208=CARTESIAN_POINT ( 'NONE',  ( -238.4067589809705794, 28.96627169325354956, -28.96627169325289231 ) ) ;
#2209=CARTESIAN_POINT ( 'NONE',  ( -56.48582580120559982, -21.81201906317804173, 34.75652343174591152 ) ) ;
#2211=CARTESIAN_POINT ( 'NONE',  ( -259.2033419157646676, 39.99999999999987921, 9.517827891723049660 ) ) ;
#2212=CARTESIAN_POINT ( 'NONE',  ( 136.1360204305621266, -3.511608612530630058, -3.511608612530719764 ) ) ;
#2214=CARTESIAN_POINT ( 'NONE',  ( 4.995406935893289102, 10.78321810388998081, 10.78321810389001811 ) ) ;
#2215=CARTESIAN_POINT ( 'NONE',  ( 19.06497207195981147, -10.03556273973439517, 10.03556273973429214 ) ) ;
#2218=CARTESIAN_POINT ( 'NONE',  ( 146.6084372240433709, -40.00000000000001421, 5.374981219216829587 ) ) ;
#2221=CARTESIAN_POINT ( 'NONE',  ( 22.72189371636483557, 47.04833883278845974, -13.83659596078922682 ) ) ;
#2222=CARTESIAN_POINT ( 'NONE',  ( -135.8532207217289738, 30.84685318188643777, -40.00000000000002132 ) ) ;
#2223=CARTESIAN_POINT ( 'NONE',  ( 0.2972598230769930572, 14.33493731733933352, 0.000000000000000000 ) ) ;
#2224=CARTESIAN_POINT ( 'NONE',  ( -4.082462733454207182, -42.99255347688252726, 23.44093842354193313 ) ) ;
#2225=CARTESIAN_POINT ( 'NONE',  ( 4.995406935893288214, 15.24977328854832770, 40.00000000000002132 ) ) ;
#2226=VERTEX_POINT ( 'NONE', #12412 ) ;
#2228=CARTESIAN_POINT ( 'NONE',  ( 192.4448373802100889, -14.14213562375876698, -14.14213562375885047 ) ) ;
#2229=CARTESIAN_POINT ( 'NONE',  ( -70.28815428291109413, -9.450978460797621494, 22.81668038719991998 ) ) ;
#2230=CARTESIAN_POINT ( 'NONE',  ( -4.121597284766290059, 23.43330939486714470, -42.98102224344789590 ) ) ;
#2232=CARTESIAN_POINT ( 'NONE',  ( -114.4364955367336449, 20.04994829326807348, -8.644468109231272734 ) ) ;
#2233=CARTESIAN_POINT ( 'NONE',  ( 146.5090579137182090, -29.94463907179424211, 12.40347562390428138 ) ) ;
#2234=CARTESIAN_POINT ( 'NONE',  ( -183.1091233172535624, -13.45963571007644610, 45.18843800009203449 ) ) ;
#2235=CARTESIAN_POINT ( 'NONE',  ( -105.3755690713226727, -15.38646221621807619, 15.38646221621768362 ) ) ;
#2236=CARTESIAN_POINT ( 'NONE',  ( 170.2234770963711128, 24.55285855007190321, 0.000000000000000000 ) ) ;
#2237=CARTESIAN_POINT ( 'NONE',  ( -193.3669098795969319, 18.32287322059355361, -44.23532903078456968 ) ) ;
#2238=CARTESIAN_POINT ( 'NONE',  ( -208.1127848780265026, 10.60833733269551615, -10.60833733269529766 ) ) ;
#2239=CARTESIAN_POINT ( 'NONE',  ( 146.6084372240433709, 3.800685668858042821, 52.76785682606522698 ) ) ;
#2241=CARTESIAN_POINT ( 'NONE',  ( 184.8905102610680444, -19.07866798485555293, -2.449293598294708485E-15 ) ) ;
#2242=CARTESIAN_POINT ( 'NONE',  ( -91.56559293963834989, 17.32597176626809343, 2.449293598294708485E-15 ) ) ;
#2243=CARTESIAN_POINT ( 'NONE',  ( 14.38125909742181818, -39.99999999999986500, -15.17850393972675604 ) ) ;
#2244=CARTESIAN_POINT ( 'NONE',  ( 130.8568914410475372, 4.207082182992862407, 4.207082182992856190 ) ) ;
#2245=CARTESIAN_POINT ( 'NONE',  ( -99.31364972222439746, 20.79869444142039470, -8.164808577100629350 ) ) ;
#2246=CARTESIAN_POINT ( 'NONE',  ( 0.2972598230770100991, -38.42060263243632079, -38.42060263243699580 ) ) ;
#2248=CARTESIAN_POINT ( 'NONE',  ( -198.0356074513804572, -17.40982414986482141, 39.15871834505909987 ) ) ;
#2250=CARTESIAN_POINT ( 'NONE',  ( -91.56559293963834989, -12.25131212657492874, 12.25131212657477953 ) ) ;
#2251=CARTESIAN_POINT ( 'NONE',  ( -3.205219349396362993, -43.36521377095327523, -17.96245967913666064 ) ) ;
#2253=ORIENTED_EDGE ( 'NONE', *, *, #21362, .T. ) ;
#2254=CARTESIAN_POINT ( 'NONE',  ( 18.90082769090740555, -48.20711988125818692, -14.00978943384287767 ) ) ;
#2259=CYLINDRICAL_SURFACE ( 'NONE', #10711, 69.99999999999994316 ) ;
#2260=CARTESIAN_POINT ( 'NONE',  ( 130.8568914410475372, -24.07718906447222551, -24.07718906447233209 ) ) ;
#2261=CARTESIAN_POINT ( 'NONE',  ( -188.9478905404515103, -43.31768569177536676, -17.94277290414884618 ) ) ;
#2262=CARTESIAN_POINT ( 'NONE',  ( 151.7948205124836534, -40.00000000000001421, 6.767089262348889633 ) ) ;
#2263=CARTESIAN_POINT ( 'NONE',  ( -30.26275506840324425, 41.69427246844627177, 40.00000000000002132 ) ) ;
#2266=CARTESIAN_POINT ( 'NONE',  ( -192.9588430854689989, -8.596193650988133061E-14, 14.46834944099969533 ) ) ;
#2267=CARTESIAN_POINT ( 'NONE',  ( -162.0762913951021176, -40.00000000000019895, 41.69427287672974813 ) ) ;
#2268=CARTESIAN_POINT ( 'NONE',  ( 4.995406935893290878, -5.232665749138292703E-14, 15.24977328854832592 ) ) ;
#2270=CARTESIAN_POINT ( 'NONE',  ( -259.2033419157646676, -30.48217210827744950, 40.00000000000002132 ) ) ;
#2271=CARTESIAN_POINT ( 'NONE',  ( 14.38125909742182529, -39.01709431150933938, 39.01709431150894147 ) ) ;
#2272=CARTESIAN_POINT ( 'NONE',  ( 130.8888609958233076, -12.21841679119707891, -29.49786752803538548 ) ) ;
#2274=CARTESIAN_POINT ( 'NONE',  ( 91.82158438592158234, 2.580785920671402147E-13, -22.79471317813470321 ) ) ;
#2275=CARTESIAN_POINT ( 'NONE',  ( 163.1118516004056573, -1.695744499706194789E-14, 12.73709011382475254 ) ) ;
#2276=CARTESIAN_POINT ( 'NONE',  ( 91.82158438592158234, 16.11829626346139577, 16.11829626346143840 ) ) ;
#2278=CARTESIAN_POINT ( 'NONE',  ( -89.92902785008709543, -8.734793929541330826, -20.17328762787300533 ) ) ;
#2279=CARTESIAN_POINT ( 'NONE',  ( 130.8568914410475088, -32.49135343045460900, -24.07718906446924478 ) ) ;
#2281=CARTESIAN_POINT ( 'NONE',  ( 136.1360204305621551, -53.05693388239309627, -3.511608612531332163 ) ) ;
#2282=CARTESIAN_POINT ( 'NONE',  ( 133.2080217031555378, 29.90338805389124488, -12.38638889282725408 ) ) ;
#2283=CARTESIAN_POINT ( 'NONE',  ( 4.995406935893307754, -55.24977328854835434, -2.449293598294708485E-15 ) ) ;
#2284=CARTESIAN_POINT ( 'NONE',  ( -105.3220356878035915, 10.86389608387957395, 18.46482525816570330 ) ) ;
#2286=ORIENTED_EDGE ( 'NONE', *, *, #15342, .T. ) ;
#2289=CARTESIAN_POINT ( 'NONE',  ( 5.823571940223288834, 14.15488761396325046, 49.16771748719407498 ) ) ;
#2290=ORIENTED_EDGE ( 'NONE', *, *, #15245, .T. ) ;
#2291=ORIENTED_EDGE ( 'NONE', *, *, #1024, .F. ) ;
#2292=CARTESIAN_POINT ( 'NONE',  ( -198.0356074513804572, 15.37879056873067007, 0.000000000000000000 ) ) ;
#2294=CARTESIAN_POINT ( 'NONE',  ( -259.2033419157646676, 49.83842185052027673, -6.730120644403441155 ) ) ;
#2295=CARTESIAN_POINT ( 'NONE',  ( -196.0240701155048271, -24.63338802315931986, 44.60678452943332672 ) ) ;
#2296=EDGE_CURVE ( 'NONE', #858, #22654, #8641, .T. ) ;
#2298=CARTESIAN_POINT ( 'NONE',  ( -86.96347745069645896, 40.00000000000019895, -18.24025645688310249 ) ) ;
#2300=CARTESIAN_POINT ( 'NONE',  ( -238.4067589809705794, 39.99999999999999289, -0.9644942799821634161 ) ) ;
#2304=CARTESIAN_POINT ( 'NONE',  ( -188.2652133075138750, 13.82568790539370163, 46.97855991888750538 ) ) ;
#2305=CARTESIAN_POINT ( 'NONE',  ( -198.0356074513804572, -39.15871834505931304, 17.40982414986437377 ) ) ;
#2306=( BOUNDED_SURFACE ( )  B_SPLINE_SURFACE ( 3, 2, ( 
 ( #6998, #503, #23250 ),
 ( #24851, #15119, #4765 ),
 ( #13003, #23121, #14590 ),
 ( #22718, #12869, #16985 ),
 ( #2635, #13132, #18855 ),
 ( #635, #6603, #24990 ),
 ( #20987, #2768, #20728 ),
 ( #18718, #10877, #18589 ),
 ( #11007, #19117, #18992 ),
 ( #25122, #900, #769 ) ),
 .UNSPECIFIED., .F., .F., .T. ) 
 B_SPLINE_SURFACE_WITH_KNOTS ( ( 4, 2, 2, 2, 4 ),
 ( 3, 3 ),
 ( 0.04143701731398998639, 0.04847035109443004197, 0.05022868453954006107, 0.05198701798465007323, 0.05550368487487010449 ),
 ( 0.000000000000000000, 1.000000000000000000 ),
 .UNSPECIFIED. ) 
 GEOMETRIC_REPRESENTATION_ITEM ( )  RATIONAL_B_SPLINE_SURFACE ( (
 ( 1.000000000000000000, 0.9541700779530608578, 1.000000000000000000),
 ( 1.000000000000000000, 0.9520138072637328586, 1.000000000000000000),
 ( 1.000000000000000000, 0.9503242346237325000, 1.000000000000000000),
 ( 1.000000000000000000, 0.9488844900981833197, 1.000000000000000000),
 ( 1.000000000000000000, 0.9486296596067500531, 1.000000000000000000),
 ( 1.000000000000000000, 0.9481942170211148380, 1.000000000000000000),
 ( 1.000000000000000000, 0.9480132043934548225, 1.000000000000000000),
 ( 1.000000000000000000, 0.9475791817277525730, 1.000000000000000000),
 ( 1.000000000000000000, 0.9474351099636038054, 1.000000000000000000),
 ( 1.000000000000000000, 0.9474350314971538012, 1.000000000000000000) ) ) 
 REPRESENTATION_ITEM ( '' )  SURFACE ( )  );
#2307=CARTESIAN_POINT ( 'NONE',  ( -114.6380096433489797, -11.20642776433569665, -18.98727595036316984 ) ) ;
#2308=CARTESIAN_POINT ( 'NONE',  ( -86.96347745069645896, 43.67073346367970288, 12.89780903124427702 ) ) ;
#2309=CARTESIAN_POINT ( 'NONE',  ( -77.70130000790294389, 5.505113979798187174, 21.34877220993403313 ) ) ;
#2310=CARTESIAN_POINT ( 'NONE',  ( 0.2972598230770048811, -10.13633138497415942, -66.70487387989865624 ) ) ;
#2312=CARTESIAN_POINT ( 'NONE',  ( -91.56559293963836410, 22.67402823373190301, 40.00000000000002132 ) ) ;
#2314=CARTESIAN_POINT ( 'NONE',  ( -105.3755690713226727, -15.38646221621807619, 15.38646221621768362 ) ) ;
#2315=CARTESIAN_POINT ( 'NONE',  ( 184.8905102610680444, 20.92133201514447194, 40.00000000000002132 ) ) ;
#2316=CARTESIAN_POINT ( 'NONE',  ( -110.0880539878520352, 16.49558164034374741, 11.64549321196552256 ) ) ;
#2317=CARTESIAN_POINT ( 'NONE',  ( 91.82158438592156813, 40.00000000000027711, -22.79471317813428044 ) ) ;
#2318=CARTESIAN_POINT ( 'NONE',  ( -56.48582580120559271, -6.472252184284187138, -6.472252184284199572 ) ) ;
#2319=CARTESIAN_POINT ( 'NONE',  ( 132.4338126186516149, -12.33615677966369972, 29.78211700502403048 ) ) ;
#2320=ORIENTED_EDGE ( 'NONE', *, *, #25191, .F. ) ;
#2323=CARTESIAN_POINT ( 'NONE',  ( 199.9999999999999432, -20.00000000000006750, 0.000000000000000000 ) ) ;
#2324=CARTESIAN_POINT ( 'NONE',  ( -88.39148973765149719, -8.027153355909691257, -20.15708830332379975 ) ) ;
#2325=CARTESIAN_POINT ( 'NONE',  ( -91.56559293963834989, 12.25131212657497848, -12.25131212657469426 ) ) ;
#2327=EDGE_CURVE ( 'NONE', #7090, #61, #14669, .T. ) ;
#2328=CARTESIAN_POINT ( 'NONE',  ( -199.9999999999999147, -49.28189405767606956, -14.17215463606684089 ) ) ;
#2330=CARTESIAN_POINT ( 'NONE',  ( -126.6834154283331912, 11.16464792285796293, 24.04426794716179572 ) ) ;
#2333=CARTESIAN_POINT ( 'NONE',  ( -213.1075012329537230, 9.698598906450543566, -9.698598906450348167 ) ) ;
#2334=CARTESIAN_POINT ( 'NONE',  ( 14.38125909742181818, -39.01709431150928253, 17.55144818341435808 ) ) ;
#2335=CARTESIAN_POINT ( 'NONE',  ( -110.0946026131977789, 20.04280215252648034, 2.777995947984109648 ) ) ;
#2336=CARTESIAN_POINT ( 'NONE',  ( -56.48582580120560692, 39.99999999999991473, 9.153146818114004546 ) ) ;
#2337=CARTESIAN_POINT ( 'NONE',  ( 14.38125909742181818, -39.01709431150928253, 17.55144818341435808 ) ) ;
#2338=CARTESIAN_POINT ( 'NONE',  ( 3.854699808470062550, 14.12217777258775087, 48.95177852071779512 ) ) ;
#2339=CARTESIAN_POINT ( 'NONE',  ( 91.82158438592158234, -12.16597498397778843, 12.16597498397750954 ) ) ;
#2342=CARTESIAN_POINT ( 'NONE',  ( -91.56559293963836410, -12.25131212657462321, -44.31723036834905827 ) ) ;
#2345=CARTESIAN_POINT ( 'NONE',  ( 91.82158438592158234, -6.516925787240506436E-14, 22.79471317813470321 ) ) ;
#2347=CARTESIAN_POINT ( 'NONE',  ( 23.46661716383104590, 46.77475180958804657, -13.79413593526249926 ) ) ;
#2348=CARTESIAN_POINT ( 'NONE',  ( 57.59792236341147031, 37.56421063658187620, 2.449293598294708485E-15 ) ) ;
#2349=CARTESIAN_POINT ( 'NONE',  ( -238.4067589809705794, 0.6820004457912757223, 0.6820004457913219076 ) ) ;
#2350=CARTESIAN_POINT ( 'NONE',  ( 17.75917276260962296, -24.33671690504799656, -44.20478326162363913 ) ) ;
#2351=CARTESIAN_POINT ( 'NONE',  ( -17.28139728211570869, -39.07633224435642205, 20.85871090875331646 ) ) ;
#2353=CARTESIAN_POINT ( 'NONE',  ( 14.38125909742180752, 15.17850393972634038, 40.00000000000002132 ) ) ;
#2354=ORIENTED_EDGE ( 'NONE', *, *, #14093, .T. ) ;
#2355=CARTESIAN_POINT ( 'NONE',  ( -199.9999999999999432, 43.68705981750494516, 18.09577267661451927 ) ) ;
#2356=CARTESIAN_POINT ( 'NONE',  ( 91.82158438592158234, -40.45024623143958564, 16.11829626348418998 ) ) ;
#2357=CARTESIAN_POINT ( 'NONE',  ( -5.379830816902156698, -23.18791234549711788, 42.60994460517750326 ) ) ;
#2359=CARTESIAN_POINT ( 'NONE',  ( 9.345847406388463341, 24.85453859512489316, -44.90706793518255324 ) ) ;
#2361=CARTESIAN_POINT ( 'NONE',  ( 184.8905102610680444, -1.851754852062639767E-13, 20.92133201514444352 ) ) ;
#2363=CARTESIAN_POINT ( 'NONE',  ( -197.4153392276943748, -24.72549520223458330, 44.73189834455659764 ) ) ;
#2364=CARTESIAN_POINT ( 'NONE',  ( 151.7948205124836534, -23.49921654115981084, -33.06932595376387951 ) ) ;
#2365=CARTESIAN_POINT ( 'NONE',  ( -105.2940237833716282, 11.46076537571703646, -18.12284447397524190 ) ) ;
#2368=CARTESIAN_POINT ( 'NONE',  ( -189.0540493709910095, 17.95404051684933577, -43.34488811517292106 ) ) ;
#2369=CARTESIAN_POINT ( 'NONE',  ( -91.56559293963834989, -16.03295912088728414, 16.03295912088688269 ) ) ;
#2370=CARTESIAN_POINT ( 'NONE',  ( 184.8905102610680444, -14.79361573936399665, 14.79361573936367158 ) ) ;
#2371=CARTESIAN_POINT ( 'NONE',  ( -86.96347745069644475, -18.24025645688354302, -2.449293598294708485E-15 ) ) ;
#2372=CARTESIAN_POINT ( 'NONE',  ( -238.4067589809705794, 40.96449427998256709, 2.449293598294708485E-15 ) ) ;
#2373=CARTESIAN_POINT ( 'NONE',  ( -162.0762913951020892, -1.202636532414034422E-14, -1.694272876828323948 ) ) ;
#2374=CARTESIAN_POINT ( 'NONE',  ( 151.7948205124836534, -23.49921654116027980, 33.06932595376354556 ) ) ;
#2375=CARTESIAN_POINT ( 'NONE',  ( -188.2995950289364941, -13.82811170417257607, 46.99046209955427855 ) ) ;
#2376=CARTESIAN_POINT ( 'NONE',  ( -30.26275506840323359, -1.198031551615522439, -57.76657404653986561 ) ) ;
#2377=CARTESIAN_POINT ( 'NONE',  ( 130.8568914410475088, 52.36146031193420924, 4.207082182989907437 ) ) ;
#2380=CARTESIAN_POINT ( 'NONE',  ( 19.06497207195980792, 10.03556273973433299, 10.03556273973436319 ) ) ;
#2381=CARTESIAN_POINT ( 'NONE',  ( -196.0240701155051113, -14.12332411291384737, -48.96019554246502281 ) ) ;
#2382=CARTESIAN_POINT ( 'NONE',  ( 146.6084372240433709, 24.48358557860311180, 32.08495691632071356 ) ) ;
#2383=CARTESIAN_POINT ( 'NONE',  ( -3.921555385251674686, -43.03974577853533390, -23.47492146735003615 ) ) ;
#2386=CARTESIAN_POINT ( 'NONE',  ( -82.26522686998488609, -10.29055646685526426, -17.41035301669956681 ) ) ;
#2391=CARTESIAN_POINT ( 'NONE',  ( -190.0144721488881601, -47.57279682963539358, -13.91469502168864203 ) ) ;
#2392=CARTESIAN_POINT ( 'NONE',  ( 4.995406935893298872, -1.944352046434030652E-13, 55.24977328854835434 ) ) ;
#2393=CARTESIAN_POINT ( 'NONE',  ( -56.48582580120559982, 30.84685318188643777, -40.00000000000002132 ) ) ;
#2396=CIRCLE ( 'NONE', #1538, 15.00000000000000178 ) ;
#2397=CARTESIAN_POINT ( 'NONE',  ( 14.38125909742182529, -40.00000000000021316, 55.17850393974251944 ) ) ;
#2398=CARTESIAN_POINT ( 'NONE',  ( 184.8905102610680444, 40.00000000000013500, -20.92133201514430141 ) ) ;
#2399=CARTESIAN_POINT ( 'NONE',  ( -190.1760961843334030, -23.85870989132040521, -43.55713529792407002 ) ) ;
#2401=CARTESIAN_POINT ( 'NONE',  ( 199.9999999999999432, -19.99999999999988987, -2.449293598294708485E-15 ) ) ;
#2402=CARTESIAN_POINT ( 'NONE',  ( -198.0356074513804572, 17.40982414986446969, 39.15871834505921356 ) ) ;
#2403=CARTESIAN_POINT ( 'NONE',  ( -213.1075012329537230, 1.045191102001431893E-13, -13.71589010951911902 ) ) ;
#2406=CARTESIAN_POINT ( 'NONE',  ( -238.4067589809705794, 40.00000000000040501, -40.96449427990138759 ) ) ;
#2407=CARTESIAN_POINT ( 'NONE',  ( -213.1075012329537230, 39.99999999999979394, 53.71589010950180665 ) ) ;
#2411=CARTESIAN_POINT ( 'NONE',  ( -114.4364955367335881, -20.04994829326802019, 8.644468109231409514 ) ) ;
#2412=CARTESIAN_POINT ( 'NONE',  ( 151.7948205124835681, -4.785054706298153882, -51.78348778862540058 ) ) ;
#2413=ORIENTED_EDGE ( 'NONE', *, *, #2459, .T. ) ;
#2414=CARTESIAN_POINT ( 'NONE',  ( -24.88648382767190270, 36.77569126515872711, -19.35593139203984592 ) ) ;
#2416=CARTESIAN_POINT ( 'NONE',  ( 4.995406935893307754, -55.24977328853207581, -40.00000000000002132 ) ) ;
#2417=CARTESIAN_POINT ( 'NONE',  ( -114.7823189589621649, 14.64951506468985798, -16.64646944818631980 ) ) ;
#2418=CARTESIAN_POINT ( 'NONE',  ( 19.06497207195980792, 10.03556273973447155, -10.03556273973422286 ) ) ;
#2420=( BOUNDED_CURVE ( )  B_SPLINE_CURVE ( 3, ( #25615, #21605, #1259, #9760 ),
 .UNSPECIFIED., .F., .F. ) 
 B_SPLINE_CURVE_WITH_KNOTS ( ( 4, 4 ),
 ( 0.004183487405659177746, 0.01388163287021749320 ),
 .UNSPECIFIED. ) 
 CURVE ( )  GEOMETRIC_REPRESENTATION_ITEM ( )  RATIONAL_B_SPLINE_CURVE ( ( 0.6809743333591599113, 0.7608653435686186794, 0.8672072324488987460, 1.000000000000000000 ) ) 
 REPRESENTATION_ITEM ( '' )  );
#2423=CARTESIAN_POINT ( 'NONE',  ( -99.31364972216337605, 8.164808577109676335, -20.79869444142046575 ) ) ;
#2424=CARTESIAN_POINT ( 'NONE',  ( 23.35901252181146859, 23.34306388117459008, 42.86175755505350793 ) ) ;
#2426=ORIENTED_EDGE ( 'NONE', *, *, #1020, .T. ) ;
#2427=CARTESIAN_POINT ( 'NONE',  ( 4.995406935893294431, -17.50105314357198694, 39.06748935135188816 ) ) ;
#2429=CARTESIAN_POINT ( 'NONE',  ( -110.0822598093780300, -4.084357705409311201, 19.77208535310552051 ) ) ;
#2430=CARTESIAN_POINT ( 'NONE',  ( -30.26275506840325136, 57.76657404653985139, 1.198031551616126178 ) ) ;
#2431=CARTESIAN_POINT ( 'NONE',  ( -105.2054292635175727, 7.329160573984922335E-13, -21.49321519473985020 ) ) ;
#2433=CARTESIAN_POINT ( 'NONE',  ( -198.0356074513804572, 5.461327841961909642E-13, -55.37879056873073580 ) ) ;
#2434=CARTESIAN_POINT ( 'NONE',  ( 200.0000000000000000, 39.99999999999985079, 20.00000000000052225 ) ) ;
#2435=CARTESIAN_POINT ( 'NONE',  ( -163.5815475687401204, 38.33196416463010081, -12.03526863292965388 ) ) ;
#2438=CARTESIAN_POINT ( 'NONE',  ( -188.3392535381826178, 23.45796413245995282, 43.01687576774276778 ) ) ;
#2439=CARTESIAN_POINT ( 'NONE',  ( -100.7734535825088500, 16.03295912088691821, 16.03295912088721309 ) ) ;
#2440=CARTESIAN_POINT ( 'NONE',  ( 98.29820294267865677, 17.41560179325850655, -10.21753654889061202 ) ) ;
#2441=CARTESIAN_POINT ( 'NONE',  ( -192.9588430854690273, 18.05360324515418924, 38.51493924976949756 ) ) ;
#2443=CARTESIAN_POINT ( 'NONE',  ( 130.8568914410475088, 24.07718906446937623, -32.49135343045455215 ) ) ;
#2444=CARTESIAN_POINT ( 'NONE',  ( -200.0000000000000000, 45.81998439131063350, -19.51623549979301586 ) ) ;
#2445=CARTESIAN_POINT ( 'NONE',  ( 130.8568914410475372, 34.05028731879791337, 0.000000000000000000 ) ) ;
#2446=B_SPLINE_CURVE_WITH_KNOTS ( 'NONE', 3,
 ( #22171, #12847, #14965, #2607, #25356, #1137, #12704, #18829, #3127, #17348, #6977, #21229 ),
 .UNSPECIFIED., .F., .F.,
 ( 4, 2, 2, 2, 2, 4 ),
 ( 0.004260855364862041646, 0.008951250736248025225, 0.01129644842194101745, 0.01364164610763400967, 0.01833204147901999065, 0.02302243685040597510 ),
 .UNSPECIFIED. ) ;
#2447=CARTESIAN_POINT ( 'NONE',  ( 136.1360204305621551, 3.511608612530062512, 53.05693388239318864 ) ) ;
#2448=CARTESIAN_POINT ( 'NONE',  ( -91.56559293963836410, 22.67402823373189946, -0.000000000000000000 ) ) ;
#2451=CARTESIAN_POINT ( 'NONE',  ( -100.7734535825088358, 1.654174317907124744E-13, -17.32597176626811120 ) ) ;
#2454=ORIENTED_EDGE ( 'NONE', *, *, #3381, .F. ) ;
#2456=CARTESIAN_POINT ( 'NONE',  ( 0.2972598230769930572, 14.33493731733933352, 0.000000000000000000 ) ) ;
#2458=CARTESIAN_POINT ( 'NONE',  ( 14.38125909742181108, 39.01709431150961649, -39.01709431150867147 ) ) ;
#2459=EDGE_CURVE ( 'NONE', #13654, #22653, #3464, .T. ) ;
#2460=CARTESIAN_POINT ( 'NONE',  ( 98.29820294267332770, 18.47759065023125302, -7.653668647303920380 ) ) ;
#2461=CARTESIAN_POINT ( 'NONE',  ( -188.2995950289364089, -43.00522595870943832, -23.44932284466036521 ) ) ;
#2462=( BOUNDED_SURFACE ( )  B_SPLINE_SURFACE ( 3, 2, ( 
 ( #21358, #8851, #14699 ),
 ( #3002, #8988, #10720 ),
 ( #16833, #15091, #4871 ),
 ( #11230, #15222, #5003 ),
 ( #16961, #12975, #21098 ),
 ( #17092, #24967, #23353 ) ),
 .UNSPECIFIED., .F., .F., .F. ) 
 B_SPLINE_SURFACE_WITH_KNOTS ( ( 4, 2, 4 ),
 ( 3, 3 ),
 ( 0.04143195986178510593, 0.04845790097403032681, 0.05548384208627555464 ),
 ( 0.000000000000000000, 1.000000000000000000 ),
 .UNSPECIFIED. ) 
 GEOMETRIC_REPRESENTATION_ITEM ( )  RATIONAL_B_SPLINE_SURFACE ( (
 ( 1.000000000000000000, 0.9541700777564472435, 1.000000000000000000),
 ( 1.000000000000000000, 0.9520117016571142399, 1.000000000000000000),
 ( 1.000000000000000000, 0.9503157806795483609, 1.000000000000000000),
 ( 1.000000000000000000, 0.9480088156006571953, 1.000000000000000000),
 ( 1.000000000000000000, 0.9474362554090329791, 1.000000000000000000),
 ( 1.000000000000000000, 0.9474350312570024579, 1.000000000000000000) ) ) 
 REPRESENTATION_ITEM ( '' )  SURFACE ( )  );
#2463=CARTESIAN_POINT ( 'NONE',  ( -83.28983882461058386, -1.484402994022060711E-13, 35.99236576815652455 ) ) ;
#2465=CARTESIAN_POINT ( 'NONE',  ( 170.0000000000000000, -2.301191124287261779E-13, 24.95097643317000546 ) ) ;
#2466=CARTESIAN_POINT ( 'NONE',  ( -100.7734535825088500, -16.03295912088659492, -40.53558337403696044 ) ) ;
#2467=CARTESIAN_POINT ( 'NONE',  ( 163.1118516004056573, -9.006482792074626431, 47.56205970284951690 ) ) ;
#2469=CARTESIAN_POINT ( 'NONE',  ( 136.1360204305621551, 40.00000000000009948, -4.966164525586641787 ) ) ;
#2471=CARTESIAN_POINT ( 'NONE',  ( -3.071327051952974063, 13.87830843099595057, 47.32824404903805515 ) ) ;
#2472=CARTESIAN_POINT ( 'NONE',  ( -86.96347745069644475, -15.38646221621786125, -15.38646221621789856 ) ) ;
#2473=CARTESIAN_POINT ( 'NONE',  ( 146.6084372240433709, -3.800685668858344801, -52.76785682606520567 ) ) ;
#2476=CARTESIAN_POINT ( 'NONE',  ( -56.48582580120559982, 39.99999999999990763, 30.84685318188658698 ) ) ;
#2478=CARTESIAN_POINT ( 'NONE',  ( 23.26364522860148654, 42.89098160628032730, -23.36474233297085945 ) ) ;
#2479=CARTESIAN_POINT ( 'NONE',  ( 136.1360204305621266, 4.966164525587089429, 2.449293598294708485E-15 ) ) ;
#2480=CARTESIAN_POINT ( 'NONE',  ( -135.8532207217289738, -34.75652343174615311, 21.81201906317767936 ) ) ;
#2481=CARTESIAN_POINT ( 'NONE',  ( -105.3755690713226585, 18.24025645688349684, 40.00000000000002132 ) ) ;
#2483=CARTESIAN_POINT ( 'NONE',  ( -4.201409602816726263, -42.95750343186489317, 23.41774994521231790 ) ) ;
#2484=CARTESIAN_POINT ( 'NONE',  ( 163.1118516004056573, 12.73709011382477918, 40.00000000000002132 ) ) ;
#2485=EDGE_CURVE ( 'NONE', #7299, #6050, #16556, .T. ) ;
#2488=CARTESIAN_POINT ( 'NONE',  ( -280.0000000000000000, -14.14213562373098831, -14.14213562373098654 ) ) ;
#2490=ADVANCED_FACE ( 'NONE', ( #980 ), #8909, .T. ) ;
#2491=ADVANCED_FACE ( 'NONE', ( #19068 ), #11608, .T. ) ;
#2492=CARTESIAN_POINT ( 'NONE',  ( -4.421177063218397763, 13.80119274858276590, -46.85829989839402288 ) ) ;
#2494=CARTESIAN_POINT ( 'NONE',  ( -100.7734535825088500, 12.25131212657428748, 44.31723036834913643 ) ) ;
#2498=CARTESIAN_POINT ( 'NONE',  ( -189.1288815661663989, -23.62384257861548775, 43.24061771116531361 ) ) ;
#2500=CARTESIAN_POINT ( 'NONE',  ( 136.1360204305621551, -24.77266263493081766, -31.79587985999290112 ) ) ;
#2501=CARTESIAN_POINT ( 'NONE',  ( -105.4741150117369273, 8.366608964608960974, -19.60045294982168329 ) ) ;
#2502=DIRECTION ( 'NONE',  ( -0.3301743753965505901, 0.9439199552035636431, 0.000000000000000000 ) ) ;
#2503=CARTESIAN_POINT ( 'NONE',  ( 57.59792236341147031, 26.56190807104720975, -26.56190807104655249 ) ) ;
#2504=CARTESIAN_POINT ( 'NONE',  ( 19.06497207195980792, 10.03556273973447155, -10.03556273973422286 ) ) ;
#2505=CARTESIAN_POINT ( 'NONE',  ( -91.56559293963834989, -17.32597176626812896, 40.00000000000002132 ) ) ;
#2506=CARTESIAN_POINT ( 'NONE',  ( 163.1118516004056573, 12.73709011382478273, 2.449293598294708485E-15 ) ) ;
#2507=CARTESIAN_POINT ( 'NONE',  ( -100.7734535825088358, -2.560096224687585342E-13, 22.67402823373191723 ) ) ;
#2508=CARTESIAN_POINT ( 'NONE',  ( 136.1360204305621551, 31.79587985999267374, -24.77266263493117293 ) ) ;
#2509=CARTESIAN_POINT ( 'NONE',  ( -86.86578273022546171, 19.68494377654086591, -8.153770686795049016 ) ) ;
#2510=CARTESIAN_POINT ( 'NONE',  ( -100.7734535825088500, 16.03295912088740494, -40.53558337403661938 ) ) ;
#2511=CARTESIAN_POINT ( 'NONE',  ( -198.0356074513804572, -10.87444709759729911, 10.87444709759714812 ) ) ;
#2512=ORIENTED_EDGE ( 'NONE', *, *, #10872, .F. ) ;
#2513=CARTESIAN_POINT ( 'NONE',  ( 199.9999999999999432, 14.14213562373090838, 14.14213562373092437 ) ) ;
#2516=CARTESIAN_POINT ( 'NONE',  ( 146.6084372240433993, -3.800685668858652999, 3.800685668858636568 ) ) ;
#2517=CARTESIAN_POINT ( 'NONE',  ( 16.38602454699831057, -48.74566733939990826, -14.09104119327536786 ) ) ;
#2519=CARTESIAN_POINT ( 'NONE',  ( 19.06497207195980792, 14.19242893257840876, 0.000000000000000000 ) ) ;
#2521=CIRCLE ( 'NONE', #5914, 30.00000000000003908 ) ;
#2525=CARTESIAN_POINT ( 'NONE',  ( -192.9588430854689989, 54.46834944099968823, 2.449293598294708485E-15 ) ) ;
#2528=CARTESIAN_POINT ( 'NONE',  ( -198.0356074513804572, -67.44298959253333692, -10.87444709761016348 ) ) ;
#2529=CARTESIAN_POINT ( 'NONE',  ( -192.9588430854690273, 39.99999999999980105, 54.46834944098235809 ) ) ;
#2530=CARTESIAN_POINT ( 'NONE',  ( -213.1075012329537230, 39.99999999999979394, 53.71589010950180665 ) ) ;
#2531=CARTESIAN_POINT ( 'NONE',  ( 199.9999999999999432, 1.065690307512836407E-13, -20.00000000000010303 ) ) ;
#2532=CARTESIAN_POINT ( 'NONE',  ( -280.0000000000000000, 19.99999999999996092, -0.000000000000000000 ) ) ;
#2534=CARTESIAN_POINT ( 'NONE',  ( -30.26275506840323004, -41.69427246844627888, -40.00000000000002132 ) ) ;
#2535=CARTESIAN_POINT ( 'NONE',  ( -162.0762913951020607, -1.198031840455708430, 57.76657433537920383 ) ) ;
#2536=CARTESIAN_POINT ( 'NONE',  ( 110.0479209278586552, -9.419601331808673095, -22.74092928740049402 ) ) ;
#2537=CARTESIAN_POINT ( 'NONE',  ( -105.2333497862813374, 16.99530394074077222, -13.14348404881843280 ) ) ;
#2538=CARTESIAN_POINT ( 'NONE',  ( 19.06497207195980792, 40.00000000000059686, -54.19242893257802507 ) ) ;
#2539=CARTESIAN_POINT ( 'NONE',  ( -259.2033419157646676, 39.99999999999987210, 30.48217210827754542 ) ) ;
#2540=CARTESIAN_POINT ( 'NONE',  ( 184.8905102610680444, 13.49065550809817715, -43.07788698682574591 ) ) ;
#2543=CARTESIAN_POINT ( 'NONE',  ( -198.0356074513804572, -67.44298959250878056, 10.87444709758448447 ) ) ;
#2547=CARTESIAN_POINT ( 'NONE',  ( 163.1118516004056573, 27.26290988616876021, -40.00000000000002132 ) ) ;
#2549=CARTESIAN_POINT ( 'NONE',  ( -105.2940152837819454, 11.46092073792507193, 18.12276621495183804 ) ) ;
#2552=ORIENTED_EDGE ( 'NONE', *, *, #25597, .F. ) ;
#2555=CARTESIAN_POINT ( 'NONE',  ( 126.3230993689413708, 11.72464299830509482, -28.30579214049042847 ) ) ;
#2556=CARTESIAN_POINT ( 'NONE',  ( 6.762329110783161568, 18.56720258519183986, 44.82519229650664983 ) ) ;
#2559=PRODUCT_DEFINITION_SHAPE ( 'NONE', 'NONE',  #14914 ) ;
#2560=CARTESIAN_POINT ( 'NONE',  ( -135.8532207217289738, -34.75652343174615311, 21.81201906317767936 ) ) ;
#2563=CARTESIAN_POINT ( 'NONE',  ( -213.1075012329537230, -18.58567234101155208, 37.98287015391234434 ) ) ;
#2565=CARTESIAN_POINT ( 'NONE',  ( -86.96347745069645896, 40.00000000000008527, -21.75974354311636461 ) ) ;
#2566=CIRCLE ( 'NONE', #26311, 69.99999999999994316 ) ;
#2570=CONICAL_SURFACE ( 'NONE', #19542, 60.00000000000009948, 0.7853981633974479459 ) ;
#2571=CARTESIAN_POINT ( 'NONE',  ( -100.7734535825088500, 40.00000000000017764, -17.32597176626768487 ) ) ;
#2572=CARTESIAN_POINT ( 'NONE',  ( -30.26275506840324070, 1.218738420030236455E-14, -1.694272468446259783 ) ) ;
#2574=CARTESIAN_POINT ( 'NONE',  ( -87.13361725327074225, -15.19799821270821560, -15.19799821270861884 ) ) ;
#2576=CARTESIAN_POINT ( 'NONE',  ( -188.6013476421465782, 13.84412643133159904, 47.09841799633510817 ) ) ;
#2577=CARTESIAN_POINT ( 'NONE',  ( 91.82158438592156813, -16.11829626348459144, 40.45024623143943643 ) ) ;
#2579=CARTESIAN_POINT ( 'NONE',  ( 163.1118516004056573, 19.27778845539212327, 37.29075403953164169 ) ) ;
#2581=CARTESIAN_POINT ( 'NONE',  ( 146.6084372240433709, 24.48358557860356655, -32.08495691632035118 ) ) ;
#2583=CARTESIAN_POINT ( 'NONE',  ( 184.8905102610680444, 20.92133201514447549, 0.000000000000000000 ) ) ;
#2584=EDGE_CURVE ( 'NONE', #8799, #25674, #25753, .T. ) ;
#2585=CARTESIAN_POINT ( 'NONE',  ( 163.1118516004056573, -19.27778845538787422, 19.27778845538743724 ) ) ;
#2586=CARTESIAN_POINT ( 'NONE',  ( -105.3755690713226585, 21.75974354311648185, 40.00000000000002132 ) ) ;
#2589=CARTESIAN_POINT ( 'NONE',  ( 170.2234770963711128, -39.99999999999982947, -15.44714144992858529 ) ) ;
#2591=EDGE_CURVE ( 'NONE', #8524, #3196, #14957, .T. ) ;
#2596=CARTESIAN_POINT ( 'NONE',  ( -100.7734535825088500, 17.32597176626808988, 40.00000000000002132 ) ) ;
#2599=CARTESIAN_POINT ( 'NONE',  ( 98.29820294267329928, 18.47759065023126013, -7.653668647303936368 ) ) ;
#2600=CARTESIAN_POINT ( 'NONE',  ( -77.65678946166502783, -18.42186864997352913, 12.10857941958507134 ) ) ;
#2605=CARTESIAN_POINT ( 'NONE',  ( -280.0000000000000568, -42.42640687119276066, -14.14213562373147148 ) ) ;
#2606=CARTESIAN_POINT ( 'NONE',  ( -280.0000000000000000, 14.14213562373078581, 14.14213562373108424 ) ) ;
#2607=CARTESIAN_POINT ( 'NONE',  ( -100.0993625062911150, 20.55804859447406230, 8.515422543756583806 ) ) ;
#2608=CARTESIAN_POINT ( 'NONE',  ( -238.4067589809705794, 40.00000000000040501, -40.96449427990138759 ) ) ;
#2610=CARTESIAN_POINT ( 'NONE',  ( 21.15737826136109234, 13.91467835516651164, 47.57244852138558144 ) ) ;
#2611=CARTESIAN_POINT ( 'NONE',  ( 199.9999999999999432, -14.14213562373096345, -14.14213562373104871 ) ) ;
#2612=CARTESIAN_POINT ( 'NONE',  ( -213.1075012329536946, -37.98287015391263566, 37.98287015391218802 ) ) ;
#2615=CARTESIAN_POINT ( 'NONE',  ( 170.2234770963711128, -2.511315425431857630E-14, 15.44714144992816074 ) ) ;
#2616=CARTESIAN_POINT ( 'NONE',  ( 44.82887508605028160, 38.96139886172597500, -12.17256213098433548 ) ) ;
#2617=CARTESIAN_POINT ( 'NONE',  ( 19.06497207195980792, 14.19242893257840876, 0.000000000000000000 ) ) ;
#2618=CARTESIAN_POINT ( 'NONE',  ( -56.48582580120559982, -6.472252184284282173, 50.09629031063965243 ) ) ;
#2619=CARTESIAN_POINT ( 'NONE',  ( -30.26275506840324425, 1.694272468446254232, 40.00000000000002132 ) ) ;
#2620=ORIENTED_EDGE ( 'NONE', *, *, #697, .T. ) ;
#2621=CARTESIAN_POINT ( 'NONE',  ( -3.406542234095978561, -43.31371932780104572, 17.94112998239678447 ) ) ;
#2623=CARTESIAN_POINT ( 'NONE',  ( -280.0000000000000000, 19.99999999999996092, 2.449293598294708485E-15 ) ) ;
#2624=B_SPLINE_CURVE_WITH_KNOTS ( 'NONE', 3,
 ( #23453, #15575, #3484, #5227, #9088, #25332 ),
 .UNSPECIFIED., .F., .F.,
 ( 4, 2, 4 ),
 ( 0.3689590070116581244, 0.3867117631979620773, 0.4044645193949217288 ),
 .UNSPECIFIED. ) ;
#2626=CARTESIAN_POINT ( 'NONE',  ( 35.93739820529123818, -20.78453043059072769, -38.99308227228176094 ) ) ;
#2628=( BOUNDED_SURFACE ( )  B_SPLINE_SURFACE ( 3, 2, ( 
 ( #16950, #866, #2870 ),
 ( #25347, #8976, #10840 ),
 ( #4729, #7103, #18957 ),
 ( #738, #23343, #5122 ),
 ( #13226, #7225, #25473 ),
 ( #5240, #13729, #7869 ),
 ( #21854, #19462, #19988 ),
 ( #11868, #13593, #25605 ),
 ( #23977, #1249, #1773 ),
 ( #3763, #15461, #19854 ),
 ( #17586, #9353, #9878 ),
 ( #21594, #9482, #15716 ) ),
 .UNSPECIFIED., .F., .F., .F. ) 
 B_SPLINE_SURFACE_WITH_KNOTS ( ( 4, 2, 2, 2, 2, 4 ),
 ( 3, 3 ),
 ( 0.006022589392326875915, 0.01254516766564483035, 0.01580645680230381017, 0.01906774593896278652, 0.02559032421228074269, 0.03211290248559869887 ),
 ( 0.000000000000000000, 1.000000000000000000 ),
 .UNSPECIFIED. ) 
 GEOMETRIC_REPRESENTATION_ITEM ( )  RATIONAL_B_SPLINE_SURFACE ( (
 ( 1.000000000000000000, 0.9998834880171258988, 1.000000000000000000),
 ( 1.000000000000000000, 0.9998139205011338237, 1.000000000000000000),
 ( 1.000000000000000000, 0.9997315632445886724, 1.000000000000000000),
 ( 1.000000000000000000, 0.9996405464946352959, 1.000000000000000000),
 ( 1.000000000000000000, 0.9996155081776924023, 1.000000000000000000),
 ( 1.000000000000000000, 0.9995814087511104562, 1.000000000000000000),
 ( 1.000000000000000000, 0.9995724100939918921, 1.000000000000000000),
 ( 1.000000000000000000, 0.9995726760936894939, 1.000000000000000000),
 ( 1.000000000000000000, 0.9996103361816741639, 1.000000000000000000),
 ( 1.000000000000000000, 0.9997312749796802844, 1.000000000000000000),
 ( 1.000000000000000000, 0.9998135910914284219, 1.000000000000000000),
 ( 1.000000000000000000, 0.9998834880173383954, 1.000000000000000000) ) ) 
 REPRESENTATION_ITEM ( '' )  SURFACE ( )  );
#2629=CARTESIAN_POINT ( 'NONE',  ( 4.995406935893294431, -17.50105314357198694, 39.06748935135188816 ) ) ;
#2630=CARTESIAN_POINT ( 'NONE',  ( -24.53392603781537318, -12.34411287792658563, 39.81639166308519151 ) ) ;
#2631=B_SPLINE_CURVE_WITH_KNOTS ( 'NONE', 3,
 ( #7303, #5076, #21677, #11177, #15417, #11546 ),
 .UNSPECIFIED., .F., .F.,
 ( 4, 2, 4 ),
 ( -5.999999988291011724E-08, 0.03937727647058182623, 0.07875461294116353761 ),
 .UNSPECIFIED. ) ;
#2632=CARTESIAN_POINT ( 'NONE',  ( -3.379936260373888501, 17.94397654175175205, -43.32059152999933360 ) ) ;
#2634=CARTESIAN_POINT ( 'NONE',  ( -135.8532207217289738, 21.81201906317729566, 34.75652343174635917 ) ) ;
#2635=CARTESIAN_POINT ( 'NONE',  ( -77.61595200903875025, -21.80829238163389405, 3.459815247604749011 ) ) ;
#2637=CARTESIAN_POINT ( 'NONE',  ( -189.1816166312677581, -17.96744819724865039, 43.37725711903350856 ) ) ;
#2638=CARTESIAN_POINT ( 'NONE',  ( 0.2972598230769976091, -10.13633138497465147, -10.13633138497482733 ) ) ;
#2640=CARTESIAN_POINT ( 'NONE',  ( 151.7948205124836250, -4.785054706301671068, 4.785054706301645311 ) ) ;
#2641=CARTESIAN_POINT ( 'NONE',  ( -198.0356074513804572, -17.40982414986427429, -39.15871834505933435 ) ) ;
#2642=CARTESIAN_POINT ( 'NONE',  ( 184.8905102610680444, 14.79361573936375507, 14.79361573936398067 ) ) ;
#2644=CARTESIAN_POINT ( 'NONE',  ( -213.1075012329537230, -9.698598906450422774, -9.698598906450550672 ) ) ;
#2645=CARTESIAN_POINT ( 'NONE',  ( 151.7948205124836534, 33.06932595376333239, 23.49921654116065284 ) ) ;
#2646=CARTESIAN_POINT ( 'NONE',  ( -91.56559293963834989, 12.25131212657428748, 44.31723036834913643 ) ) ;
#2647=CARTESIAN_POINT ( 'NONE',  ( -162.0762913951020607, -41.69427287692683848, 40.00000000000002132 ) ) ;
#2648=CARTESIAN_POINT ( 'NONE',  ( -259.2033419157646676, -9.517827891722680178, -40.00000000000002132 ) ) ;
#2649=CARTESIAN_POINT ( 'NONE',  ( -105.3755690713226727, -2.472783935621397949E-13, 21.75974354311649961 ) ) ;
#2650=CARTESIAN_POINT ( 'NONE',  ( -198.0356074513804572, 10.87444709759714989, 10.87444709759722450 ) ) ;
#2651=CARTESIAN_POINT ( 'NONE',  ( -86.86493150571116928, 19.77569912839187083, -7.943527260495796050 ) ) ;
#2652=CARTESIAN_POINT ( 'NONE',  ( 192.4448373802101173, 42.42640687122089815, -14.14213562370272470 ) ) ;
#2653=EDGE_CURVE ( 'NONE', #9180, #21913, #21069, .T. ) ;
#2654=CARTESIAN_POINT ( 'NONE',  ( -166.3490444793987422, 39.29840179260881428, -12.23457652165070186 ) ) ;
#2656=CARTESIAN_POINT ( 'NONE',  ( -86.96347745069644475, -15.38646221621796073, 41.18208027870593924 ) ) ;
#2657=CARTESIAN_POINT ( 'NONE',  ( -94.58414068589586066, 8.590713000693110502, 20.73981583682890317 ) ) ;
#2658=CARTESIAN_POINT ( 'NONE',  ( 151.7948205124836250, -4.785054706301671068, 4.785054706301645311 ) ) ;
#2659=CARTESIAN_POINT ( 'NONE',  ( -3.488770945845510063, -43.29206711590405376, -17.93216134257416527 ) ) ;
#2660=ORIENTED_EDGE ( 'NONE', *, *, #58, .T. ) ;
#2661=CARTESIAN_POINT ( 'NONE',  ( -94.58366989427186411, -20.91926462023914013, 8.190486896679004758 ) ) ;
#2662=CARTESIAN_POINT ( 'NONE',  ( -110.0574606394870329, -9.172127818399005150, -18.01698387425555481 ) ) ;
#2666=CARTESIAN_POINT ( 'NONE',  ( -30.26275506840324070, 41.69427246844628598, 2.449293598294708485E-15 ) ) ;
#2669=CARTESIAN_POINT ( 'NONE',  ( 170.2234770963711128, -39.20704971665404059, 17.36149277826957160 ) ) ;
#2670=CARTESIAN_POINT ( 'NONE',  ( -280.0000000000000000, -1.237140859393462838E-13, 20.00000000000001421 ) ) ;
#2671=CARTESIAN_POINT ( 'NONE',  ( 200.0000000000000000, 40.00000000000012790, -19.99999999999996092 ) ) ;
#2674=CARTESIAN_POINT ( 'NONE',  ( -192.9588430854689705, -54.46834944099975928, -2.449293598294708485E-15 ) ) ;
#2675=CARTESIAN_POINT ( 'NONE',  ( 23.26364522860124140, -13.80713620122686436, -46.84987168986906170 ) ) ;
#2677=CARTESIAN_POINT ( 'NONE',  ( 136.1360204305621551, -4.966164525587036138, -40.00000000000002132 ) ) ;
#2678=CARTESIAN_POINT ( 'NONE',  ( -213.1075012329537230, -9.698598906438496314, 66.26714140136188291 ) ) ;
#2679=CARTESIAN_POINT ( 'NONE',  ( 130.1167162091013267, -12.15076864148440983, -29.33455044752963659 ) ) ;
#2680=CARTESIAN_POINT ( 'NONE',  ( -110.0685463886750313, 10.00056106073172479, -17.53216629774168567 ) ) ;
#2681=CARTESIAN_POINT ( 'NONE',  ( 170.2234770963711128, 39.99999999999980105, 24.55285855007229401 ) ) ;
#2682=CARTESIAN_POINT ( 'NONE',  ( -30.26275506840324425, 39.99999999999987210, 41.69427246844643520 ) ) ;
#2683=CARTESIAN_POINT ( 'NONE',  ( 199.9999999999999432, -14.14213562373096345, -14.14213562373104871 ) ) ;
#2686=CARTESIAN_POINT ( 'NONE',  ( 192.4448373802101173, -42.42640687116490028, -14.14213562375904942 ) ) ;
#2689=CARTESIAN_POINT ( 'NONE',  ( -87.13361725327074225, 15.19799821270847850, -15.19799821270833284 ) ) ;
#2690=CARTESIAN_POINT ( 'NONE',  ( 192.4448373802100889, -14.14213562375896061, 14.14213562375865330 ) ) ;
#2691=CARTESIAN_POINT ( 'NONE',  ( 154.0339099654741233, 28.18615453125291381, -11.67508747798877344 ) ) ;
#2692=CARTESIAN_POINT ( 'NONE',  ( 170.2234770963711128, 24.55285855007190676, -40.00000000000002132 ) ) ;
#2693=CARTESIAN_POINT ( 'NONE',  ( -87.13361725327072804, 5.903697393916396424E-14, -21.49321519333428299 ) ) ;
#2700=CARTESIAN_POINT ( 'NONE',  ( 19.44355705751405239, 18.20455056366773405, 43.94967286773182025 ) ) ;
#2701=ORIENTED_EDGE ( 'NONE', *, *, #10106, .F. ) ;
#2703=CARTESIAN_POINT ( 'NONE',  ( -213.1075012329537230, -18.58567234101155208, 37.98287015391234434 ) ) ;
#2705=CARTESIAN_POINT ( 'NONE',  ( -105.4293522941591590, -7.324187428699950431, 20.05597878319033356 ) ) ;
#2706=CARTESIAN_POINT ( 'NONE',  ( -135.8532207217289738, -6.472252184284287502, 50.09629031063965243 ) ) ;
#2707=CARTESIAN_POINT ( 'NONE',  ( 199.9999999999999432, -14.14213562373096345, -14.14213562373104871 ) ) ;
#2708=CARTESIAN_POINT ( 'NONE',  ( -238.4067589809705794, 39.99999999999983658, 40.96449428006354765 ) ) ;
#2710=CARTESIAN_POINT ( 'NONE',  ( -86.86493150571121191, -8.366608963954089262, -19.60045294882756295 ) ) ;
#2711=CARTESIAN_POINT ( 'NONE',  ( -213.1075012329537230, 40.00000000000055422, -53.71589010953623244 ) ) ;
#2712=CARTESIAN_POINT ( 'NONE',  ( 19.06497207195981147, 1.521599808664285085E-13, -14.19242893257840521 ) ) ;
#2716=CARTESIAN_POINT ( 'NONE',  ( -188.2506440019711818, 13.82466072834903770, 46.97351617221500675 ) ) ;
#2717=CARTESIAN_POINT ( 'NONE',  ( 19.06497207195981858, -38.31983398719641087, 18.24870850772724040 ) ) ;
#2718=CARTESIAN_POINT ( 'NONE',  ( 190.0000000000001137, 3.490243377569959927E-14, 0.000000000000000000 ) ) ;
#2719=CARTESIAN_POINT ( 'NONE',  ( 136.1360204305621551, 24.77266263493108411, 31.79587985999273769 ) ) ;
#2720=CARTESIAN_POINT ( 'NONE',  ( -77.58208867533490150, 21.99046547477049174, -2.676519792206656589 ) ) ;
#2721=CARTESIAN_POINT ( 'NONE',  ( -280.0000000000000000, -14.14213562373088706, -14.14213562373108424 ) ) ;
#2723=CARTESIAN_POINT ( 'NONE',  ( -208.1127848780265026, -15.00245453012673202, 0.000000000000000000 ) ) ;
#2724=CARTESIAN_POINT ( 'NONE',  ( -192.9588430854690273, 38.51493924976913519, 18.05360324515490333 ) ) ;
#2725=CARTESIAN_POINT ( 'NONE',  ( 146.6084372240433993, 34.62501878078308692, 0.000000000000000000 ) ) ;
#2728=CARTESIAN_POINT ( 'NONE',  ( 199.9999999999999432, 2.486775779033024914E-13, -19.99999999999992539 ) ) ;
#2731=ORIENTED_EDGE ( 'NONE', *, *, #5807, .F. ) ;
#2732=ORIENTED_EDGE ( 'NONE', *, *, #12326, .F. ) ;
#2734=CARTESIAN_POINT ( 'NONE',  ( -105.3755690713226585, 18.24025645688349684, 40.00000000000002132 ) ) ;
#2736=CARTESIAN_POINT ( 'NONE',  ( 83.06440094959391729, 24.44702070089013901, -9.006081069718883114 ) ) ;
#2739=CARTESIAN_POINT ( 'NONE',  ( 146.6084372240433993, 1.478241399363601114E-13, -34.62501878078305850 ) ) ;
#2742=CARTESIAN_POINT ( 'NONE',  ( 19.06497207195980792, -18.24870850772710540, -38.31983398719647482 ) ) ;
#2743=CARTESIAN_POINT ( 'NONE',  ( -86.96347745069644475, 15.38646221621772092, 15.38646221621800336 ) ) ;
#2744=DIRECTION ( 'NONE',  ( 1.000000000000000000, 0.000000000000000000, 0.000000000000000000 ) ) ;
#2745=CARTESIAN_POINT ( 'NONE',  ( -100.7734535825088500, 40.00000000000017764, -17.32597176626768487 ) ) ;
#2746=CARTESIAN_POINT ( 'NONE',  ( -102.4068193528145940, -8.088405365069414543, 20.44188272012834418 ) ) ;
#2747=CARTESIAN_POINT ( 'NONE',  ( -162.0762913951020892, -1.694272876828353702, 0.000000000000000000 ) ) ;
#2748=CARTESIAN_POINT ( 'NONE',  ( -135.8532207217289738, 21.81201906317767936, 21.81201906317778239 ) ) ;
#2749=CARTESIAN_POINT ( 'NONE',  ( 170.2234770963711128, -10.92277846919202666, 10.92277846919193962 ) ) ;
#2753=CARTESIAN_POINT ( 'NONE',  ( 199.9999999999999432, 1.065690307512836407E-13, -20.00000000000010303 ) ) ;
#2755=CARTESIAN_POINT ( 'NONE',  ( 170.2234770963711128, -45.64576402573183600, 10.92277846919191653 ) ) ;
#2756=CARTESIAN_POINT ( 'NONE',  ( -91.56559293963834989, -22.67402823373193499, 40.00000000000002132 ) ) ;
#2758=CARTESIAN_POINT ( 'NONE',  ( 3.468680970029910604, -44.56630890487710417, 24.60338114560769185 ) ) ;
#2759=CARTESIAN_POINT ( 'NONE',  ( -198.0356074513804572, 15.37879056873066830, -40.00000000000002132 ) ) ;
#2761=CARTESIAN_POINT ( 'NONE',  ( -87.13361725327075646, -14.71749760135919161, 15.67849882405766770 ) ) ;
#2762=CARTESIAN_POINT ( 'NONE',  ( -56.48582580120559271, -6.472252184284187138, -6.472252184284199572 ) ) ;
#2763=CARTESIAN_POINT ( 'NONE',  ( -3.473570583883154317, -17.93385599103746486, 43.29615835920800748 ) ) ;
#2764=CARTESIAN_POINT ( 'NONE',  ( -259.2033419157646676, 21.55415060305839958, -35.01439189186541512 ) ) ;
#2767=CARTESIAN_POINT ( 'NONE',  ( 19.06497207195980792, 10.03556273973447155, -10.03556273973422286 ) ) ;
#2768=CARTESIAN_POINT ( 'NONE',  ( -82.24289765310217604, -20.07413437147977575, 2.209159509587613535 ) ) ;
#2769=CARTESIAN_POINT ( 'NONE',  ( 107.5473083967386572, -23.99138244111233220, 0.000000000000000000 ) ) ;
#2770=CARTESIAN_POINT ( 'NONE',  ( -188.3392995398478149, -23.45797413244888929, 43.01688924973637285 ) ) ;
#2771=CARTESIAN_POINT ( 'NONE',  ( 4.995406935893293543, -10.78321810388990265, -10.78321810389009272 ) ) ;
#2772=CARTESIAN_POINT ( 'NONE',  ( 146.6084372240433709, 52.76785682606519146, 3.800685668858932775 ) ) ;
#2773=CARTESIAN_POINT ( 'NONE',  ( -86.96347745069644475, -15.38646221621738164, -41.18208027870615240 ) ) ;
#2774=DIRECTION ( 'NONE',  ( 1.000000000000000000, 1.836970198721030181E-16, 0.000000000000000000 ) ) ;
#2775=CARTESIAN_POINT ( 'NONE',  ( -208.1127848780264742, 17.67593391476678377, -38.89260858015718014 ) ) ;
#2776=CARTESIAN_POINT ( 'NONE',  ( -135.8532207217289738, 50.09629031063956006, 6.472252184284782217 ) ) ;
#2777=CARTESIAN_POINT ( 'NONE',  ( -213.1075012329537230, 37.98287015391211696, 18.58567234101190735 ) ) ;
#2778=CARTESIAN_POINT ( 'NONE',  ( -135.8532207217289738, 9.153146818113546246, -0.000000000000000000 ) ) ;
#2779=CARTESIAN_POINT ( 'NONE',  ( 0.2972598230769930017, 54.33493731733938148, -40.00000000000002132 ) ) ;
#2780=CARTESIAN_POINT ( 'NONE',  ( -162.0762913951021176, 29.48230308784768638, -27.08623940707612121 ) ) ;
#2782=CARTESIAN_POINT ( 'NONE',  ( -162.0762913951020607, -57.76657433537922515, -1.198031840455874963 ) ) ;
#2784=VERTEX_POINT ( 'NONE', #24888 ) ;
#2785=CARTESIAN_POINT ( 'NONE',  ( -259.2033419157646676, 21.55415060305830366, 21.55415060305842800 ) ) ;
#2787=CARTESIAN_POINT ( 'NONE',  ( -192.9588430854690273, -10.23066800229550388, 66.79921049721887982 ) ) ;
#2788=CARTESIAN_POINT ( 'NONE',  ( -2.164901439684538076, -47.64638340558528284, -13.92557459409770892 ) ) ;
#2789=EDGE_LOOP ( 'NONE', ( #9312, #7216, #10203, #17169 ) ) ;
#2790=CARTESIAN_POINT ( 'NONE',  ( -173.7925187073452946, -41.93431653918364788, 12.78856575065205270 ) ) ;
#2791=CARTESIAN_POINT ( 'NONE',  ( -110.1017833366170748, -14.28014421838192405, -14.28014421838201820 ) ) ;
#2795=CARTESIAN_POINT ( 'NONE',  ( -162.0762913951020892, 41.69427287692678163, -40.00000000000002132 ) ) ;
#2800=CARTESIAN_POINT ( 'NONE',  ( 19.06497207195982924, -66.60410523465809263, -10.03556273973493163 ) ) ;
#2801=CARTESIAN_POINT ( 'NONE',  ( -100.7734535825088358, -8.145438380286941744E-14, 17.32597176626811120 ) ) ;
#2802=CARTESIAN_POINT ( 'NONE',  ( 200.0000000000000000, 39.99999999999999289, 20.00000000000007105 ) ) ;
#2803=CARTESIAN_POINT ( 'NONE',  ( -102.2610585947573441, 15.74993999358161112, -15.74993999358146191 ) ) ;
#2804=CARTESIAN_POINT ( 'NONE',  ( 91.82158438592159655, -22.79471317813468545, -40.00000000000002132 ) ) ;
#2805=CARTESIAN_POINT ( 'NONE',  ( 17.24092899317993144, -18.36647614517220006, -44.34059580268279888 ) ) ;
#2807=CARTESIAN_POINT ( 'NONE',  ( -91.56559293963834989, -17.32597176626812896, -2.449293598294708485E-15 ) ) ;
#2808=CARTESIAN_POINT ( 'NONE',  ( 200.0000000000000000, 42.42640687119290988, 14.14213562373111976 ) ) ;
#2810=CARTESIAN_POINT ( 'NONE',  ( -138.9613198120156881, 10.11110880661586719, 29.42718893709540851 ) ) ;
#2811=CARTESIAN_POINT ( 'NONE',  ( -126.6834156230552679, -11.16464796290101802, 24.04426801068220598 ) ) ;
#2812=CARTESIAN_POINT ( 'NONE',  ( -238.4067589809705794, -40.00000000000005684, -0.9644942799830014124 ) ) ;
#2814=CARTESIAN_POINT ( 'NONE',  ( 192.4448373802100889, -14.14213562375876698, -14.14213562375885047 ) ) ;
#2816=CARTESIAN_POINT ( 'NONE',  ( -100.0753760173619185, -8.894334231739314589, -20.41987330121788702 ) ) ;
#2817=CARTESIAN_POINT ( 'NONE',  ( 151.7948205124836534, 23.49921654116009506, 33.06932595376371609 ) ) ;
#2819=CARTESIAN_POINT ( 'NONE',  ( -77.58523997990613452, -2.778549811635243838, -21.97336465817913975 ) ) ;
#2820=CARTESIAN_POINT ( 'NONE',  ( -7.769366557094080861, 41.90323276218152415, -22.72119856430118645 ) ) ;
#2821=CARTESIAN_POINT ( 'NONE',  ( 104.1600437297061603, 20.63676802888582884, -8.548029202070297927 ) ) ;
#2822=CARTESIAN_POINT ( 'NONE',  ( 0.2972598230770130412, -54.33493731733936016, -2.449293598294708485E-15 ) ) ;
#2823=CARTESIAN_POINT ( 'NONE',  ( 170.0000000000000284, -15.47746304364901171, -19.80854622259142417 ) ) ;
#2824=CARTESIAN_POINT ( 'NONE',  ( -188.4701769959784770, 43.05504096897865907, -23.48627020870706161 ) ) ;
#2826=ORIENTED_EDGE ( 'NONE', *, *, #15195, .T. ) ;
#2827=CIRCLE ( 'NONE', #6201, 14.99999999999999467 ) ;
#2828=DIRECTION ( 'NONE',  ( 1.000000000000000000, 0.000000000000000000, 0.000000000000000000 ) ) ;
#2829=CARTESIAN_POINT ( 'NONE',  ( -86.86578273022558960, 8.153770686795043687, -19.68494377654074157 ) ) ;
#2833=CARTESIAN_POINT ( 'NONE',  ( 170.2234770963711128, -45.64576402573183600, 10.92277846919191653 ) ) ;
#2835=CARTESIAN_POINT ( 'NONE',  ( -114.6097568999503125, -5.809233881211882888, 21.20070836100120815 ) ) ;
#2836=EDGE_CURVE ( 'NONE', #4035, #6176, #5428, .T. ) ;
#2837=CARTESIAN_POINT ( 'NONE',  ( 200.0000000000000000, -42.42640687119293119, 14.14213562373082134 ) ) ;
#2838=CARTESIAN_POINT ( 'NONE',  ( -238.4067589809705794, 0.6820004457912757223, 0.6820004457913219076 ) ) ;
#2839=CARTESIAN_POINT ( 'NONE',  ( -162.0762913951020892, 39.99999999999985079, 41.69427287692695216 ) ) ;
#2840=CARTESIAN_POINT ( 'NONE',  ( -192.1167141818823154, -24.15421809699817501, 43.95739236919496307 ) ) ;
#2843=CARTESIAN_POINT ( 'NONE',  ( -200.0000000000000000, -10.02640517461745517, 53.44529986889241968 ) ) ;
#2844=CARTESIAN_POINT ( 'NONE',  ( -91.56559293963834989, -39.99999999999985789, -17.32597176626853042 ) ) ;
#2845=CARTESIAN_POINT ( 'NONE',  ( 130.8568914410475088, 39.99999999999969447, 34.05028731879830417 ) ) ;
#2846=CARTESIAN_POINT ( 'NONE',  ( -77.63478802649954957, 18.14812407464349064, 12.54968118178400083 ) ) ;
#2847=CARTESIAN_POINT ( 'NONE',  ( -87.02160625236410851, 10.86264740421045083, 18.50711184548089960 ) ) ;
#2849=CARTESIAN_POINT ( 'NONE',  ( -188.6013476421563553, 23.51433506916966110, 43.09288642756894205 ) ) ;
#2850=CARTESIAN_POINT ( 'NONE',  ( 170.2234770963711128, 17.36149277826980253, 17.36149277827007253 ) ) ;
#2851=CARTESIAN_POINT ( 'NONE',  ( -198.0012400611978194, -49.19397081476451206, 14.15884001207462184 ) ) ;
#2852=CARTESIAN_POINT ( 'NONE',  ( -162.0762913951020607, -1.198031840455708430, 57.76657433537920383 ) ) ;
#2853=CARTESIAN_POINT ( 'NONE',  ( -87.13348102040650645, -16.17099723934745015, 14.22374190074250855 ) ) ;
#2854=CARTESIAN_POINT ( 'NONE',  ( -56.48582580120558561, 6.472252184284607246, -50.09629031063960269 ) ) ;
#2855=CARTESIAN_POINT ( 'NONE',  ( -200.0000000000000000, 44.96258949770069790, -22.85346793133681942 ) ) ;
#2856=CARTESIAN_POINT ( 'NONE',  ( -162.0762913951021176, -1.694272876828353702, 40.00000000000002132 ) ) ;
#2859=CARTESIAN_POINT ( 'NONE',  ( -105.3755690713226585, 41.18208027870575449, 15.38646221621837107 ) ) ;
#2860=CARTESIAN_POINT ( 'NONE',  ( 146.6084372240433709, 34.62501878078307982, 40.00000000000002132 ) ) ;
#2863=CARTESIAN_POINT ( 'NONE',  ( -162.0762913951021176, -40.00000000000003553, -1.694272876828743168 ) ) ;
#2866=EDGE_LOOP ( 'NONE', ( #15413, #13992, #1635, #20909 ) ) ;
#2868=ORIENTED_EDGE ( 'NONE', *, *, #18344, .F. ) ;
#2869=CARTESIAN_POINT ( 'NONE',  ( 192.4448373802100889, 19.99999999996064304, 2.449293598294708485E-15 ) ) ;
#2870=CARTESIAN_POINT ( 'NONE',  ( -105.4741150117382773, -19.60045294982706920, -8.366608964594435704 ) ) ;
#2871=B_SPLINE_CURVE_WITH_KNOTS ( 'NONE', 3,
 ( #11575, #19442, #3601, #11710, #15823, #13832, #21967, #2145, #18096, #273, #8120, #11844, #6260, #16365, #26104, #10255, #7842, #16237, #18364, #7980, #16098, #9854, #22377, #20238, #18222, #10382 ),
 .UNSPECIFIED., .F., .F.,
 ( 4, 2, 1, 2, 2, 2, 2, 2, 2, 2, 2, 1, 2, 4 ),
 ( -5.999999999281531560E-08, 0.0004354487530732486806, 0.0008709575061464901744, 0.001741975012292972837, 0.003484010024585937945, 0.006968080049171867726, 0.01045215007375779881, 0.01393622009834372642, 0.02090436014751559032, 0.02438843017210151967, 0.02613046518439449128, 0.02700148269054098230, 0.02743699144361422607, 0.02787250019668746984 ),
 .UNSPECIFIED. ) ;
#2872=CARTESIAN_POINT ( 'NONE',  ( -110.0723150831393582, -19.55249150545847314, -5.015078513992241582 ) ) ;
#2876=CARTESIAN_POINT ( 'NONE',  ( 4.995406935893294431, -17.50105314357144337, -39.06748935135212264 ) ) ;
#2877=CARTESIAN_POINT ( 'NONE',  ( 0.2972598230769976091, -10.13633138497465147, -10.13633138497482733 ) ) ;
#2878=CARTESIAN_POINT ( 'NONE',  ( -77.78698662148927667, -19.58754019070067542, -9.956326400803837018 ) ) ;
#2879=CARTESIAN_POINT ( 'NONE',  ( -208.1127848780265026, 5.403397259664334602E-13, -55.00245453012672670 ) ) ;
#2881=CARTESIAN_POINT ( 'NONE',  ( 14.38125909742181285, -15.17850393972633505, 0.000000000000000000 ) ) ;
#2882=CARTESIAN_POINT ( 'NONE',  ( -100.7734535825088500, 16.03295912088683295, 40.53558337403684675 ) ) ;
#2885=CARTESIAN_POINT ( 'NONE',  ( -91.56559293963836410, 40.00000000000008527, -22.67402823373177867 ) ) ;
#2886=CARTESIAN_POINT ( 'NONE',  ( 184.8905102610680444, -20.92133201514440799, -40.00000000000002132 ) ) ;
#2887=CARTESIAN_POINT ( 'NONE',  ( 184.8905102610680444, -43.07788698682576722, 13.49065550809799063 ) ) ;
#2888=CARTESIAN_POINT ( 'NONE',  ( -135.8532207217289738, 30.84685318188643421, 40.00000000000002132 ) ) ;
#2889=VERTEX_POINT ( 'NONE', #13163 ) ;
#2890=CARTESIAN_POINT ( 'NONE',  ( 9.028290303213244883, -44.88859993224341594, 18.59346688786898483 ) ) ;
#2891=CARTESIAN_POINT ( 'NONE',  ( 146.6084372240433709, 5.374981219217002781, -40.00000000000002132 ) ) ;
#2893=CARTESIAN_POINT ( 'NONE',  ( 19.06497207195981147, 38.31983398719620482, 38.31983398719633271 ) ) ;
#2894=CARTESIAN_POINT ( 'NONE',  ( 170.2234770963711128, 1.169953928977015745E-13, -24.55285855007187124 ) ) ;
#2895=CARTESIAN_POINT ( 'NONE',  ( -77.72572481383096488, 21.21966553434844727, -5.751841496721930014 ) ) ;
#2896=B_SPLINE_CURVE_WITH_KNOTS ( 'NONE', 3,
 ( #23764, #9667, #21521, #11391, #17771, #13779 ),
 .UNSPECIFIED., .F., .F.,
 ( 4, 2, 4 ),
 ( 3.570546400823084320E-15, 0.03937634048171164552, 0.07875268096341971058 ),
 .UNSPECIFIED. ) ;
#2897=CARTESIAN_POINT ( 'NONE',  ( 23.09931156284629949, -13.81622350327199378, -46.91113948292964864 ) ) ;
#2900=CARTESIAN_POINT ( 'NONE',  ( -280.0000000000000568, 42.42640687119265408, 14.14213562373147504 ) ) ;
#2901=CARTESIAN_POINT ( 'NONE',  ( -87.12800209209292746, 1.368681197224306478, 21.45652401693913092 ) ) ;
#2902=CARTESIAN_POINT ( 'NONE',  ( -188.3120606736018772, -23.45204117844399860, 43.00889065702907033 ) ) ;
#2903=CARTESIAN_POINT ( 'NONE',  ( -259.2033419157646676, 6.730120644403426944, 6.730120644403592145 ) ) ;
#2904=CARTESIAN_POINT ( 'NONE',  ( -208.1127848780264742, 17.67593391476624021, 38.89260858015742883 ) ) ;
#2905=CARTESIAN_POINT ( 'NONE',  ( 130.8568914410475372, -24.07718906447255947, 24.07718906447199458 ) ) ;
#2906=CARTESIAN_POINT ( 'NONE',  ( -30.26275506840325136, 27.08623969584614244, -29.48230279907770779 ) ) ;
#2907=CARTESIAN_POINT ( 'NONE',  ( 184.8905102610680444, 14.79361573936375507, 14.79361573936398067 ) ) ;
#2908=CARTESIAN_POINT ( 'NONE',  ( 200.0000000000000000, 14.14213562373041455, 42.42640687119311593 ) ) ;
#2909=CARTESIAN_POINT ( 'NONE',  ( -213.1075012329537230, 9.698598906438871126, -66.26714140136179765 ) ) ;
#2910=CARTESIAN_POINT ( 'NONE',  ( -208.1127848780264742, 15.00245453012665742, -40.00000000000002132 ) ) ;
#2911=CARTESIAN_POINT ( 'NONE',  ( 91.82158438592158234, 44.40256751092336884, -12.16597498400043342 ) ) ;
#2913=CARTESIAN_POINT ( 'NONE',  ( -135.8532207217289738, -50.09629031063973770, 6.472252184283735943 ) ) ;
#2914=CARTESIAN_POINT ( 'NONE',  ( -188.9001212172966007, 43.30535683045355455, -17.93766612258001913 ) ) ;
#2916=CARTESIAN_POINT ( 'NONE',  ( 170.2234770963711128, -17.36149277826995885, 39.20704971665388427 ) ) ;
#2917=CARTESIAN_POINT ( 'NONE',  ( -77.55640685885761343, -16.62871490253266771, -14.66974043287744323 ) ) ;
#2918=CARTESIAN_POINT ( 'NONE',  ( -162.0762913951021176, 27.08623940707598265, 29.48230308784781428 ) ) ;
#2920=ORIENTED_EDGE ( 'NONE', *, *, #20292, .T. ) ;
#2921=CARTESIAN_POINT ( 'NONE',  ( -188.2652133075326049, -42.99509596150239332, 23.44262061655336993 ) ) ;
#2924=CARTESIAN_POINT ( 'NONE',  ( 4.995406935893288214, 15.24977328854832770, 0.000000000000000000 ) ) ;
#2927=CARTESIAN_POINT ( 'NONE',  ( 91.82158438592156813, -16.11829626348459144, 40.45024623143943643 ) ) ;
#2928=CARTESIAN_POINT ( 'NONE',  ( 136.1360204305621551, -40.00000000000001421, 4.966164525586921563 ) ) ;
#2929=CARTESIAN_POINT ( 'NONE',  ( 4.995406935893290878, -5.232665749138292703E-14, 15.24977328854832592 ) ) ;
#2930=CARTESIAN_POINT ( 'NONE',  ( -2.654373026594475160, 47.46285323120928723, -13.89837698318162218 ) ) ;
#2931=CARTESIAN_POINT ( 'NONE',  ( 14.38125909742181285, -15.17850393972633505, -40.00000000000002132 ) ) ;
#2932=CARTESIAN_POINT ( 'NONE',  ( 23.46661716383010088, -13.79413593526223103, -46.77475180958838052 ) ) ;
#2933=CARTESIAN_POINT ( 'NONE',  ( 57.59792236341147031, 1.722363176415065089, -1.722363176415036445 ) ) ;
#2934=CARTESIAN_POINT ( 'NONE',  ( 0.2972598230769983307, -14.33493731733933352, 40.00000000000002132 ) ) ;
#2935=CARTESIAN_POINT ( 'NONE',  ( 57.59792236341146321, 40.00000000000000711, 2.435789363418579434 ) ) ;
#2936=CARTESIAN_POINT ( 'NONE',  ( -110.1017491837771303, 13.37584907585219440, -15.18340520632207102 ) ) ;
#2937=CARTESIAN_POINT ( 'NONE',  ( -198.0356074513804572, -39.99999999999948130, -55.37879056874863437 ) ) ;
#2938=CARTESIAN_POINT ( 'NONE',  ( -238.4067589809705794, 0.6820004457912757223, 0.6820004457913219076 ) ) ;
#2939=CARTESIAN_POINT ( 'NONE',  ( 155.4806860510508670, -27.66458559364820857, -11.45904655032044239 ) ) ;
#2941=CARTESIAN_POINT ( 'NONE',  ( 57.59792236341147031, 30.00663442387683588, 26.56190807104703211 ) ) ;
#2943=CARTESIAN_POINT ( 'NONE',  ( -135.8532207217289738, 6.472252184284096543, 6.472252184284234211 ) ) ;
#2944=CARTESIAN_POINT ( 'NONE',  ( -5.866564133099172018, 46.35727274689134703, -13.69896896866313796 ) ) ;
#2945=CARTESIAN_POINT ( 'NONE',  ( 169.9999999999999716, 22.62041470344888339, -9.369682556672254137 ) ) ;
#2946=CARTESIAN_POINT ( 'NONE',  ( -30.26275506840324425, -1.694272468446265334, 40.00000000000002132 ) ) ;
#2948=CARTESIAN_POINT ( 'NONE',  ( -190.0144222802854586, 47.57278142029252166, -13.91469272132485280 ) ) ;
#2953=CARTESIAN_POINT ( 'NONE',  ( 170.0000000000000853, 9.369682556672316309, -22.62041470344884075 ) ) ;
#2954=CARTESIAN_POINT ( 'NONE',  ( -198.0012401002533409, 44.79720214428365921, -24.77357857137243613 ) ) ;
#2955=VERTEX_POINT ( 'NONE', #11160 ) ;
#2958=CARTESIAN_POINT ( 'NONE',  ( -198.0356074513804572, 10.87444709758468875, 67.44298959250869530 ) ) ;
#2959=CARTESIAN_POINT ( 'NONE',  ( -83.21262154144073975, 13.72187187061437541, 33.12752917118392304 ) ) ;
#2960=CARTESIAN_POINT ( 'NONE',  ( -30.26275506840324425, 39.99999999999987210, 41.69427246844643520 ) ) ;
#2961=CARTESIAN_POINT ( 'NONE',  ( -199.9999999999999432, -48.59548038928831204, 14.89048929005521416 ) ) ;
#2963=CARTESIAN_POINT ( 'NONE',  ( -208.1127848780264742, -39.99999999999990763, -15.00245453012711394 ) ) ;
#2964=CARTESIAN_POINT ( 'NONE',  ( 130.8568914410475088, 40.00000000000011369, -5.949712681206269949 ) ) ;
#2966=FACE_OUTER_BOUND ( 'NONE', #1995, .T. ) ;
#2967=CARTESIAN_POINT ( 'NONE',  ( -199.9999999999999716, 14.87399974031265337, -48.57705986237285600 ) ) ;
#2968=CARTESIAN_POINT ( 'NONE',  ( 130.8568914410475372, 24.07718906447243867, -24.07718906447216156 ) ) ;
#2969=CARTESIAN_POINT ( 'NONE',  ( 146.5090579137181805, 29.94463907179409290, 12.40347562390452651 ) ) ;
#2973=CARTESIAN_POINT ( 'NONE',  ( 136.1360204305621266, 53.05693388239316022, 3.511608612530967566 ) ) ;
#2974=CARTESIAN_POINT ( 'NONE',  ( -77.70606139385991185, 21.32448501951759923, -5.419212411896500825 ) ) ;
#2975=CARTESIAN_POINT ( 'NONE',  ( -280.0000000000000568, -14.14213562373137556, 42.42640687119276066 ) ) ;
#2977=CARTESIAN_POINT ( 'NONE',  ( 1.564253033640323531, 24.39614062124472937, 44.28527310957323238 ) ) ;
#2978=ORIENTED_EDGE ( 'NONE', *, *, #9553, .T. ) ;
#2979=CARTESIAN_POINT ( 'NONE',  ( 4.995406935893286438, 67.35176059880245703, -10.78321810387767066 ) ) ;
#2984=CARTESIAN_POINT ( 'NONE',  ( -238.4067589809705794, -40.00000000000005684, -0.9644942799830014124 ) ) ;
#2990=ORIENTED_EDGE ( 'NONE', *, *, #13522, .F. ) ;
#2991=ORIENTED_EDGE ( 'NONE', *, *, #24197, .T. ) ;
#2992=CARTESIAN_POINT ( 'NONE',  ( 199.9999999999999432, 19.99999999999996092, 2.449293598294708485E-15 ) ) ;
#2995=CIRCLE ( 'NONE', #13180, 15.00000000000000355 ) ;
#2997=CARTESIAN_POINT ( 'NONE',  ( 170.2234770963711128, 1.169953928977015745E-13, -24.55285855007187124 ) ) ;
#2999=CARTESIAN_POINT ( 'NONE',  ( 151.7948205124836250, -23.49921654116371883, 23.49921654116317526 ) ) ;
#3000=CARTESIAN_POINT ( 'NONE',  ( -56.48582580120559271, 6.472252184284121412, 6.472252184284244869 ) ) ;
#3001=EDGE_CURVE ( 'NONE', #3196, #9833, #7031, .T. ) ;
#3002=CARTESIAN_POINT ( 'NONE',  ( -105.3844635030161641, -19.12027419152980556, -9.640654680272803034 ) ) ;
#3003=CARTESIAN_POINT ( 'NONE',  ( 136.1360204305621551, -39.99999999999994316, -4.966164525587488221 ) ) ;
#3004=CARTESIAN_POINT ( 'NONE',  ( 192.4448373802101173, -14.14213562370342281, 42.42640687122062104 ) ) ;
#3005=CARTESIAN_POINT ( 'NONE',  ( 170.2234770963711128, 24.55285855007190676, -40.00000000000002132 ) ) ;
#3006=CARTESIAN_POINT ( 'NONE',  ( -30.26275506840323359, -1.198031551616339341, 57.76657404653985139 ) ) ;
#3010=CARTESIAN_POINT ( 'NONE',  ( -259.2033419157646676, 40.00000000000000711, -9.517827891722491884 ) ) ;
#3011=CARTESIAN_POINT ( 'NONE',  ( 91.82158438592158234, -17.20528682183298486, 0.000000000000000000 ) ) ;
#3012=CARTESIAN_POINT ( 'NONE',  ( 146.6084372240433709, -52.76785682606516303, 3.800685668858563737 ) ) ;
#3013=EDGE_CURVE ( 'NONE', #5580, #5450, #16402, .T. ) ;
#3014=CARTESIAN_POINT ( 'NONE',  ( -259.2033419157646676, -9.517827891722680178, 40.00000000000002132 ) ) ;
#3015=EDGE_LOOP ( 'NONE', ( #9374, #9694, #24059, #25401, #24348, #5735 ) ) ;
#3016=CARTESIAN_POINT ( 'NONE',  ( 22.72189371636510202, -47.04833883279060558, 13.83659596078687493 ) ) ;
#3017=CARTESIAN_POINT ( 'NONE',  ( 130.8568914410475088, -34.05028731879786363, -40.00000000000002132 ) ) ;
#3018=CARTESIAN_POINT ( 'NONE',  ( 169.9999999999999716, -22.62041470344880523, -9.369682556672316309 ) ) ;
#3019=CARTESIAN_POINT ( 'NONE',  ( 151.7948205124836250, 4.785054706301690608, 4.785054706301682614 ) ) ;
#3021=CARTESIAN_POINT ( 'NONE',  ( -86.91081356576945893, 20.06298749293320682, -7.308700132831655871 ) ) ;
#3025=CARTESIAN_POINT ( 'NONE',  ( 163.1118516004056573, 9.006482792073693844, 47.56205970284970164 ) ) ;
#3026=CARTESIAN_POINT ( 'NONE',  ( 146.6084372240433993, -34.62501878078303008, 0.000000000000000000 ) ) ;
#3027=CARTESIAN_POINT ( 'NONE',  ( 151.7948205124836250, -3.202120068677277203E-13, 33.23291073765553705 ) ) ;
#3028=CARTESIAN_POINT ( 'NONE',  ( -259.2033419157646676, 35.01439189186528722, 21.55415060305857011 ) ) ;
#3031=CARTESIAN_POINT ( 'NONE',  ( 199.9999999999999432, 14.14213562373093680, 14.14213562373114641 ) ) ;
#3032=CARTESIAN_POINT ( 'NONE',  ( 146.6084372240433993, 3.800685668858732935, -3.800685668858610367 ) ) ;
#3033=CARTESIAN_POINT ( 'NONE',  ( -162.0762913951020892, 1.198031840456041497, -57.76657433537918251 ) ) ;
#3034=CARTESIAN_POINT ( 'NONE',  ( 200.0000000000000000, -20.00000000000006750, -40.00000000000002132 ) ) ;
#3035=CARTESIAN_POINT ( 'NONE',  ( -86.96347745069644475, -15.38646221621786125, -15.38646221621789856 ) ) ;
#3037=CARTESIAN_POINT ( 'NONE',  ( -192.9588430854690273, -66.79921049721887982, -10.23066800229569040 ) ) ;
#3039=CARTESIAN_POINT ( 'NONE',  ( -121.8425418703243110, 22.74408241228373484, -9.420907402774027162 ) ) ;
#3040=VERTEX_POINT ( 'NONE', #22202 ) ;
#3041=CARTESIAN_POINT ( 'NONE',  ( 0.2972598230770011618, 10.13633138497462305, 66.70487387989858519 ) ) ;
#3044=CARTESIAN_POINT ( 'NONE',  ( -3.534370630407282832, -43.27979241395900090, -17.92707699455385750 ) ) ;
#3046=CARTESIAN_POINT ( 'NONE',  ( -114.4388184736424705, -20.16431396440406232, 8.352332320010008360 ) ) ;
#3048=CARTESIAN_POINT ( 'NONE',  ( 25.88393124174758597, -13.61573025394965164, 45.90075965688545523 ) ) ;
#3052=ADVANCED_FACE ( 'NONE', ( #24186 ), #26266, .T. ) ;
#3053=CARTESIAN_POINT ( 'NONE',  ( -105.3755690713226585, -41.18208027870611687, 15.38646221621750954 ) ) ;
#3054=CARTESIAN_POINT ( 'NONE',  ( -280.0000000000000000, 1.839446121267387017E-14, -20.00000000000001421 ) ) ;
#3058=CARTESIAN_POINT ( 'NONE',  ( -280.0000000000000000, -20.00000000000006750, -2.449293598294708485E-15 ) ) ;
#3059=CARTESIAN_POINT ( 'NONE',  ( 23.36462152323027297, -13.80148662728946896, -46.81175967489690493 ) ) ;
#3061=CARTESIAN_POINT ( 'NONE',  ( 136.1360204305621266, 35.03383547441298163, 40.00000000000002132 ) ) ;
#3063=CARTESIAN_POINT ( 'NONE',  ( -198.0356074513804572, -10.87444709759729911, 10.87444709759714812 ) ) ;
#3064=CARTESIAN_POINT ( 'NONE',  ( -30.26275506840325136, 40.00000000000003553, -1.694272468445841007 ) ) ;
#3065=CARTESIAN_POINT ( 'NONE',  ( -110.0368417077424681, 7.992411109430601179, -18.51665893310733324 ) ) ;
#3066=CARTESIAN_POINT ( 'NONE',  ( -192.9588430854690273, -39.99999999999948841, -54.46834944098263520 ) ) ;
#3070=CARTESIAN_POINT ( 'NONE',  ( -91.56559293963836410, 44.31723036834890905, 12.25131212657507795 ) ) ;
#3071=EDGE_CURVE ( 'NONE', #10709, #25674, #16221, .T. ) ;
#3072=ORIENTED_EDGE ( 'NONE', *, *, #11755, .F. ) ;
#3074=CARTESIAN_POINT ( 'NONE',  ( -2.004660104950324762, 43.67474423979815867, -18.09067139733604179 ) ) ;
#3075=CARTESIAN_POINT ( 'NONE',  ( 57.59792236341148453, -37.56421063658185489, 40.00000000000002132 ) ) ;
#3077=CARTESIAN_POINT ( 'NONE',  ( -190.5535326093529704, 43.70552662393590282, -18.10342187829310134 ) ) ;
#3083=FACE_OUTER_BOUND ( 'NONE', #3494, .T. ) ;
#3084=CARTESIAN_POINT ( 'NONE',  ( 160.7895100360958622, 1.290018736498604486E-13, -28.48799984206441138 ) ) ;
#3088=CARTESIAN_POINT ( 'NONE',  ( -100.7734535825088500, -16.03295912088716335, 40.53558337403673306 ) ) ;
#3089=CARTESIAN_POINT ( 'NONE',  ( -192.9588430854689989, 10.23066800230742679, 10.23066800230749607 ) ) ;
#3090=CARTESIAN_POINT ( 'NONE',  ( 151.7948205124836534, 40.00000000000017053, -33.23291073765538783 ) ) ;
#3093=CARTESIAN_POINT ( 'NONE',  ( -280.0000000000000568, -39.99999999999987210, -20.00000000000043343 ) ) ;
#3094=CARTESIAN_POINT ( 'NONE',  ( -105.3755690713226727, 1.741486606973311632E-13, -18.24025645688352881 ) ) ;
#3095=CARTESIAN_POINT ( 'NONE',  ( -114.4364955367319965, -20.04994829327483075, 8.644468109212210649 ) ) ;
#3096=CARTESIAN_POINT ( 'NONE',  ( 91.82158438592158234, 12.16597498397773869, -12.16597498397759303 ) ) ;
#3098=CARTESIAN_POINT ( 'NONE',  ( 167.0466155511619775, 23.44215416552593823, 9.710058186601706609 ) ) ;
#3099=CARTESIAN_POINT ( 'NONE',  ( -189.4799703873392787, -47.39666448643377805, 13.88847319136879221 ) ) ;
#3101=CARTESIAN_POINT ( 'NONE',  ( -82.23724611271893536, -13.84097227486369874, 14.71983334136218602 ) ) ;
#3102=CARTESIAN_POINT ( 'NONE',  ( 0.2972598230770153171, -66.70487387989849992, -10.13633138497533004 ) ) ;
#3104=CARTESIAN_POINT ( 'NONE',  ( -77.55640685876518603, 15.64922766773203122, 15.64922766773211471 ) ) ;
#3106=CARTESIAN_POINT ( 'NONE',  ( -135.8532207217289738, -6.472252184283586729, -50.09629031063973770 ) ) ;
#3110=CARTESIAN_POINT ( 'NONE',  ( 91.82158438592159655, -40.00000000000017764, 17.20528682183258340 ) ) ;
#3112=CARTESIAN_POINT ( 'NONE',  ( 17.75917276260962652, -44.20478326162357519, 24.33671690504831986 ) ) ;
#3115=CARTESIAN_POINT ( 'NONE',  ( -259.2033419157646676, 30.48217210827734647, 40.00000000000002132 ) ) ;
#3116=CARTESIAN_POINT ( 'NONE',  ( 19.06497207195981147, -10.03556273973439517, 10.03556273973429214 ) ) ;
#3121=CARTESIAN_POINT ( 'NONE',  ( -259.2033419157646676, -40.00000000000003553, -9.517827891722768996 ) ) ;
#3124=CARTESIAN_POINT ( 'NONE',  ( -82.24286370861491946, 12.41698901658174137, 15.97557204291290134 ) ) ;
#3125=CARTESIAN_POINT ( 'NONE',  ( -40.07203023092246497, -11.15662918578760632, -34.25109662816847589 ) ) ;
#3126=CARTESIAN_POINT ( 'NONE',  ( 163.1118516004056573, 19.27778845538753316, 19.27778845538783870 ) ) ;
#3127=CARTESIAN_POINT ( 'NONE',  ( -93.01806789315402568, 20.64606681690898782, 8.551880885224901974 ) ) ;
#3128=CARTESIAN_POINT ( 'NONE',  ( 170.2234770963711128, -39.99999999999982947, -15.44714144992858529 ) ) ;
#3130=CARTESIAN_POINT ( 'NONE',  ( 19.06497207195982924, -54.19242893257843008, -40.00000000000002132 ) ) ;
#3131=CARTESIAN_POINT ( 'NONE',  ( 163.1118516004056573, -9.006482792069636645, 9.006482792069567367 ) ) ;
#3133=CARTESIAN_POINT ( 'NONE',  ( -91.56559293963834989, -17.32597176626812185, -40.00000000000002132 ) ) ;
#3134=CARTESIAN_POINT ( 'NONE',  ( -3.971463587453694988, -43.02522237043177000, -23.46415232635092707 ) ) ;
#3135=CARTESIAN_POINT ( 'NONE',  ( -86.96347745069644475, 5.999880687339585546E-14, -21.75974354311649961 ) ) ;
#3136=CARTESIAN_POINT ( 'NONE',  ( -91.56559293963834989, -22.67402823373193499, 0.000000000000000000 ) ) ;
#3137=CARTESIAN_POINT ( 'NONE',  ( -135.8532207217289738, 21.81201906317767936, 21.81201906317778239 ) ) ;
#3138=CARTESIAN_POINT ( 'NONE',  ( 163.1118516004056573, 12.73709011382477918, 40.00000000000002132 ) ) ;
#3140=CARTESIAN_POINT ( 'NONE',  ( 22.31419732600847539, -43.29699898481722187, 17.93420418956550222 ) ) ;
#3141=DIRECTION ( 'NONE',  ( -0.01051738777840945799, 0.9307051272558533039, 0.3656191333259035670 ) ) ;
#3142=EDGE_CURVE ( 'NONE', #22654, #26074, #22271, .T. ) ;
#3143=CARTESIAN_POINT ( 'NONE',  ( 91.82158438592158234, -12.16597498400057198, 44.40256751092329779 ) ) ;
#3144=CARTESIAN_POINT ( 'NONE',  ( -91.56559293963834989, 6.234561990864368500E-14, -22.67402823373191723 ) ) ;
#3147=CARTESIAN_POINT ( 'NONE',  ( -77.90255099906865155, 8.644468104261473940, -20.04994828523921058 ) ) ;
#3152=DIRECTION ( 'NONE',  ( 0.000000000000000000, 1.000000000000000000, 0.000000000000000000 ) ) ;
#3153=CARTESIAN_POINT ( 'NONE',  ( 163.1118516004056573, 9.006482792073693844, 47.56205970284970164 ) ) ;
#3154=CARTESIAN_POINT ( 'NONE',  ( 200.0000000000000000, 42.42640687119310172, -14.14213562373052646 ) ) ;
#3155=CARTESIAN_POINT ( 'NONE',  ( 200.0000000000000000, 14.14213562373083022, 42.42640687119289566 ) ) ;
#3156=CARTESIAN_POINT ( 'NONE',  ( 19.06497207195980792, 10.03556273973447155, -10.03556273973422286 ) ) ;
#3158=CARTESIAN_POINT ( 'NONE',  ( 184.8905102610680444, 43.07788698682591644, -13.49065550809769221 ) ) ;
#3159=CARTESIAN_POINT ( 'NONE',  ( 151.7948205124836534, -51.78348778862529400, -4.785054706299085581 ) ) ;
#3160=CARTESIAN_POINT ( 'NONE',  ( -135.8532207217289738, 21.81201906317798134, -21.81201906317747685 ) ) ;
#3161=CARTESIAN_POINT ( 'NONE',  ( 14.38125909742180752, 15.17850393972634038, -40.00000000000002132 ) ) ;
#3163=( BOUNDED_CURVE ( )  B_SPLINE_CURVE ( 3, ( #17693, #21446, #11326, #21832 ),
 .UNSPECIFIED., .F., .F. ) 
 B_SPLINE_CURVE_WITH_KNOTS ( ( 4, 4 ),
 ( 0.03952673792116803697, 0.04745072232834487980 ),
 .UNSPECIFIED. ) 
 CURVE ( )  GEOMETRIC_REPRESENTATION_ITEM ( )  RATIONAL_B_SPLINE_CURVE ( ( 0.5000000000000000000, 0.4999999999999885647, 0.5065943549827448544, 0.5197830649482689802 ) ) 
 REPRESENTATION_ITEM ( '' )  );
#3164=CARTESIAN_POINT ( 'NONE',  ( -56.48582580120559271, 2.158176344243877536E-14, -9.153146818113587102 ) ) ;
#3165=CARTESIAN_POINT ( 'NONE',  ( 4.995406935893297984, -39.06748935135205869, 17.50105314357158193 ) ) ;
#3166=CARTESIAN_POINT ( 'NONE',  ( -188.8531444083254485, 43.29283928523322800, -17.93248118558230431 ) ) ;
#3168=CARTESIAN_POINT ( 'NONE',  ( -91.56559293963834989, 40.53558337403677569, -16.03295912088699993 ) ) ;
#3170=CARTESIAN_POINT ( 'NONE',  ( 15.76057515043981638, 18.44716516375474313, 44.53539632574958063 ) ) ;
#3171=CARTESIAN_POINT ( 'NONE',  ( -4.421177063219556835, -46.85829989839349707, -13.80119274858244793 ) ) ;
#3173=CARTESIAN_POINT ( 'NONE',  ( -166.7090608783924210, -37.06260950138378973, 15.35183551239266997 ) ) ;
#3175=CARTESIAN_POINT ( 'NONE',  ( 23.30336656375548188, -23.35569295765331788, 42.87878279885809718 ) ) ;
#3176=CARTESIAN_POINT ( 'NONE',  ( 98.29820294267324243, 7.653668647304287198, -18.47759065023114999 ) ) ;
#3178=CARTESIAN_POINT ( 'NONE',  ( 130.1167162091013267, -29.33455044752969343, 12.15076864148434943 ) ) ;
#3179=CARTESIAN_POINT ( 'NONE',  ( 57.59792236341147031, 39.99999999999990763, 37.56421063658199699 ) ) ;
#3181=CARTESIAN_POINT ( 'NONE',  ( -200.0000000000000000, -18.14877749763631343, -46.38610861938597907 ) ) ;
#3182=CARTESIAN_POINT ( 'NONE',  ( -238.4067589809705510, -40.96449427998265946, -2.449293598294708485E-15 ) ) ;
#3183=CARTESIAN_POINT ( 'NONE',  ( 23.58679727197023368, -13.78527791281898374, -46.73132340480074021 ) ) ;
#3185=CARTESIAN_POINT ( 'NONE',  ( 184.8905102610680444, -19.07866798485554938, 40.00000000000002132 ) ) ;
#3186=CARTESIAN_POINT ( 'NONE',  ( -213.1075012329537230, -9.698598906450557777, 9.698598906450415669 ) ) ;
#3187=CARTESIAN_POINT ( 'NONE',  ( 91.82158438592156813, 40.00000000000027711, -22.79471317813428044 ) ) ;
#3188=CARTESIAN_POINT ( 'NONE',  ( 192.4448373802101173, -39.99999999999977973, -19.99999999996102673 ) ) ;
#3189=CARTESIAN_POINT ( 'NONE',  ( 125.5822694977128435, -28.05278406097506050, -11.61984362037969554 ) ) ;
#3190=ORIENTED_EDGE ( 'NONE', *, *, #8835, .T. ) ;
#3192=CARTESIAN_POINT ( 'NONE',  ( -3.615356597029523389, 43.25798660799116391, -17.91804473398302733 ) ) ;
#3193=CARTESIAN_POINT ( 'NONE',  ( -238.4067589809705794, -0.9644942799826263791, 40.00000000000002132 ) ) ;
#3195=CARTESIAN_POINT ( 'NONE',  ( -191.2489946134048182, 43.85245824700246686, -18.16428294930772580 ) ) ;
#3196=VERTEX_POINT ( 'NONE', #20835 ) ;
#3197=EDGE_LOOP ( 'NONE', ( #8537, #5709, #360, #14901, #14125, #8295, #1175 ) ) ;
#3198=CARTESIAN_POINT ( 'NONE',  ( 130.8568914410475372, 24.07718906447243867, -24.07718906447216156 ) ) ;
#3199=CARTESIAN_POINT ( 'NONE',  ( 90.71510531243710318, -21.27078368575422118, -8.810647086396985017 ) ) ;
#3205=CARTESIAN_POINT ( 'NONE',  ( -163.5815439468655939, 18.59457101073966712, -35.61501074489178365 ) ) ;
#3206=CARTESIAN_POINT ( 'NONE',  ( -135.8532207217289738, 50.09629031063965243, -6.472252184284084109 ) ) ;
#3207=CARTESIAN_POINT ( 'NONE',  ( -129.2303573025683079, -24.84170326008768370, -11.67678754045152800 ) ) ;
#3208=CARTESIAN_POINT ( 'NONE',  ( -280.0000000000000568, -40.00000000000000000, -20.00000000000015277 ) ) ;
#3211=EDGE_CURVE ( 'NONE', #7311, #5206, #7063, .T. ) ;
#3212=CARTESIAN_POINT ( 'NONE',  ( 170.2234770963711128, -40.00000000000024158, 24.55285855007145202 ) ) ;
#3213=CARTESIAN_POINT ( 'NONE',  ( 192.4448373802100889, -20.00000000003938538, 0.000000000000000000 ) ) ;
#3214=CARTESIAN_POINT ( 'NONE',  ( 91.82158438592158234, 2.580785920671402147E-13, -22.79471317813470321 ) ) ;
#3215=DIRECTION ( 'NONE',  ( 0.3301743753966839834, 0.000000000000000000, -0.9439199552035171248 ) ) ;
#3216=CARTESIAN_POINT ( 'NONE',  ( -208.1127848780264742, -38.89260858015728672, -17.67593391476669851 ) ) ;
#3217=CARTESIAN_POINT ( 'NONE',  ( 192.4448373802100889, 1.051811698935164031E-13, -20.00000000003942091 ) ) ;
#3218=CARTESIAN_POINT ( 'NONE',  ( -199.0731274800458834, 18.57195892579281704, 44.83667511838283559 ) ) ;
#3219=CARTESIAN_POINT ( 'NONE',  ( 121.8740240556053323, 26.81399039734613865, 11.10671848392282079 ) ) ;
#3220=CARTESIAN_POINT ( 'NONE',  ( -77.72892396114366420, 19.09609284692255571, -10.88898768916570603 ) ) ;
#3221=CARTESIAN_POINT ( 'NONE',  ( -91.56559293963836410, 16.03295912088714203, -16.03295912088699282 ) ) ;
#3222=CARTESIAN_POINT ( 'NONE',  ( -87.10570614285154534, -13.14378919784947364, 16.99508527299667193 ) ) ;
#3223=CARTESIAN_POINT ( 'NONE',  ( -91.56559293963834989, -44.31723036834903695, 12.25131212657476709 ) ) ;
#3225=AXIS2_PLACEMENT_3D ( 'NONE', #18624, #4927, #14497 ) ;
#3226=CARTESIAN_POINT ( 'NONE',  ( -91.56559293963836410, -12.25131212657524138, 44.31723036834888774 ) ) ;
#3227=CARTESIAN_POINT ( 'NONE',  ( -151.4802930569921955, -16.17241674341475033, -31.86309827676130624 ) ) ;
#3229=EDGE_LOOP ( 'NONE', ( #13277, #22786, #5608, #7278, #3262, #6501 ) ) ;
#3230=CARTESIAN_POINT ( 'NONE',  ( -91.56559293963834989, 12.25131212657497848, -12.25131212657469426 ) ) ;
#3232=CARTESIAN_POINT ( 'NONE',  ( -16.41654234116891686, 12.95560590050290806, -42.70586891546086861 ) ) ;
#3234=CARTESIAN_POINT ( 'NONE',  ( 163.1118516004056573, -40.00000000000027711, 27.26290988616830546 ) ) ;
#3240=CARTESIAN_POINT ( 'NONE',  ( 57.59792236341147031, 1.722363176415065089, -1.722363176415036445 ) ) ;
#3241=CARTESIAN_POINT ( 'NONE',  ( -280.0000000000000568, 40.00000000000004263, -19.99999999999987210 ) ) ;
#3245=CARTESIAN_POINT ( 'NONE',  ( -100.7734535825088500, -39.99999999999995737, -22.67402823373205578 ) ) ;
#3247=DIRECTION ( 'NONE',  ( 0.000000000000000000, 1.000000000000000000, 0.000000000000000000 ) ) ;
#3248=CARTESIAN_POINT ( 'NONE',  ( 146.6084372240433993, -24.48358557860353457, 24.48358557860296258 ) ) ;
#3249=CARTESIAN_POINT ( 'NONE',  ( 130.8568914410475088, 24.07718906446937623, -32.49135343045455215 ) ) ;
#3250=CARTESIAN_POINT ( 'NONE',  ( -77.56366795221720167, -22.09173432935364190, 1.395416561028956393 ) ) ;
#3251=CARTESIAN_POINT ( 'NONE',  ( 91.82158438592158234, 2.580785920671402147E-13, -22.79471317813470321 ) ) ;
#3252=CARTESIAN_POINT ( 'NONE',  ( -105.2054292635177006, -21.49321519473982889, -1.366713675288041330 ) ) ;
#3253=CARTESIAN_POINT ( 'NONE',  ( -213.1075012329537230, -13.71589010951915810, 0.000000000000000000 ) ) ;
#3254=CARTESIAN_POINT ( 'NONE',  ( 130.8568914410475088, -5.949712681206664300, -40.00000000000002132 ) ) ;
#3255=CARTESIAN_POINT ( 'NONE',  ( 130.8568914410475088, 52.36146031193420924, 4.207082182989907437 ) ) ;
#3256=CARTESIAN_POINT ( 'NONE',  ( -91.56559293963836410, 22.67402823373190301, -40.00000000000002132 ) ) ;
#3257=CARTESIAN_POINT ( 'NONE',  ( -105.2054292635175585, -2.444554031225951202E-13, 21.49321519473985020 ) ) ;
#3259=FACE_OUTER_BOUND ( 'NONE', #17549, .T. ) ;
#3260=CARTESIAN_POINT ( 'NONE',  ( 91.82158438592158234, 16.11829626346139577, 16.11829626346143840 ) ) ;
#3261=CARTESIAN_POINT ( 'NONE',  ( 170.2234770963711128, 15.44714144992818738, 40.00000000000002132 ) ) ;
#3262=ORIENTED_EDGE ( 'NONE', *, *, #9386, .F. ) ;
#3263=CARTESIAN_POINT ( 'NONE',  ( 27.00968939605193953, -41.97305875717999157, 17.38581019152067597 ) ) ;
#3264=B_SPLINE_CURVE_WITH_KNOTS ( 'NONE', 3,
 ( #15275, #15520, #25925, #17916, #5430, #7666, #15778, #7159, #5181, #3178, #26201, #16462, #16191, #13925, #22196, #11935, #6217, #14462, #24584, #2233, #3833, #14064, #4104, #22328, #99, #18181, #18316, #12204, #20062, #18048, #22593, #20187, #227, #8341 ),
 .UNSPECIFIED., .F., .F.,
 ( 4, 2, 2, 2, 2, 2, 2, 2, 2, 2, 2, 2, 2, 2, 2, 2, 4 ),
 ( -5.298243351207237208E-05, 0.01887868273877487887, 0.02834451532491835332, 0.03071097347145420459, 0.03307743161799005932, 0.03544388976452591405, 0.03781034791106176185, 0.04254326420413346438, 0.04727618049720517385, 0.04964263864374102164, 0.05200909679027687638, 0.05674201308334866217, 0.05910847122988456548, 0.06029170030315254142, 0.06147492937642052430, 0.06620784566949247663, 0.07567367825563638128 ),
 .UNSPECIFIED. ) ;
#3265=( BOUNDED_SURFACE ( )  B_SPLINE_SURFACE ( 3, 2, ( 
 ( #3095, #842, #15060 ),
 ( #11076, #15314, #25447 ),
 ( #4969, #7199, #11321 ),
 ( #19437, #1224, #9583 ),
 ( #7449, #7975, #14104 ),
 ( #19563, #15818, #20099 ),
 ( #3340, #9849, #17688 ),
 ( #15563, #11704, #7576 ),
 ( #25967, #7707, #9980 ),
 ( #1355, #11441, #9454 ),
 ( #11570, #19689, #19825 ),
 ( #3734, #1741, #23813 ),
 ( #25831, #23688, #26240 ),
 ( #17560, #3873, #23945 ),
 ( #1611, #5723, #13701 ),
 ( #18089, #25698, #5466 ) ),
 .UNSPECIFIED., .F., .F., .F. ) 
 B_SPLINE_SURFACE_WITH_KNOTS ( ( 4, 2, 2, 2, 2, 2, 2, 4 ),
 ( 3, 3 ),
 ( 0.04143342415526168887, 0.04844520228007725970, 0.05195109134248504512, 0.05545698040489283054, 0.06246875852970840137, 0.06422170306091229408, 0.06597464759211618679, 0.06948053665452397221 ),
 ( 0.000000000000000000, 1.000000000000000000 ),
 .UNSPECIFIED. ) 
 GEOMETRIC_REPRESENTATION_ITEM ( )  RATIONAL_B_SPLINE_SURFACE ( (
 ( 1.000000000000000000, 0.9541700777564554592, 1.000000000000000000),
 ( 1.000000000000000000, 0.9520170179160407642, 1.000000000000000000),
 ( 1.000000000000000000, 0.9503264940267092120, 1.000000000000000000),
 ( 1.000000000000000000, 0.9485966650357087193, 1.000000000000000000),
 ( 1.000000000000000000, 0.9481601953989508003, 1.000000000000000000),
 ( 1.000000000000000000, 0.9475786562869455976, 1.000000000000000000),
 ( 1.000000000000000000, 0.9474333041665753408, 1.000000000000000000),
 ( 1.000000000000000000, 0.9474385324112287732, 1.000000000000000000),
 ( 1.000000000000000000, 0.9480205960586695069, 1.000000000000000000),
 ( 1.000000000000000000, 0.9494433550395400268, 1.000000000000000000),
 ( 1.000000000000000000, 0.9497628485351724548, 1.000000000000000000),
 ( 1.000000000000000000, 0.9504717112746540186, 1.000000000000000000),
 ( 1.000000000000000000, 0.9508623530685325065, 1.000000000000000000),
 ( 1.000000000000000000, 0.9521262215761925329, 1.000000000000000000),
 ( 1.000000000000000000, 0.9530922057189646912, 1.000000000000000000),
 ( 1.000000000000000000, 0.9541700777564678937, 1.000000000000000000) ) ) 
 REPRESENTATION_ITEM ( '' )  SURFACE ( )  );
#3269=CARTESIAN_POINT ( 'NONE',  ( 184.8905102610680444, -43.07788698682576722, 13.49065550809799063 ) ) ;
#3273=CARTESIAN_POINT ( 'NONE',  ( -47.45115950045327224, 14.84795788661607929, -29.80449331798435608 ) ) ;
#3276=CARTESIAN_POINT ( 'NONE',  ( -82.27051431266434633, -5.326770061496585384, -19.46826128364778086 ) ) ;
#3277=CARTESIAN_POINT ( 'NONE',  ( 19.06497207195980792, 10.03556273973447155, -10.03556273973422286 ) ) ;
#3278=CARTESIAN_POINT ( 'NONE',  ( 130.8568914410475088, 52.36146031193427319, -4.207082182989173802 ) ) ;
#3279=CARTESIAN_POINT ( 'NONE',  ( -110.0954903719524935, 20.05999989284160634, -2.400669240794628401 ) ) ;
#3280=CARTESIAN_POINT ( 'NONE',  ( 14.38125909742180752, 10.73282306404735387, -10.73282306404708919 ) ) ;
#3281=CARTESIAN_POINT ( 'NONE',  ( 14.38125909742182529, -39.01709431150879936, -39.01709431150948859 ) ) ;
#3282=CARTESIAN_POINT ( 'NONE',  ( -192.9588430854689705, -38.51493924976909966, -38.51493924976973915 ) ) ;
#3283=CARTESIAN_POINT ( 'NONE',  ( 4.995406935893297984, 10.78321810390233892, -67.35176059882522281 ) ) ;
#3284=CARTESIAN_POINT ( 'NONE',  ( -30.26275506840325136, 57.76657404653985139, -1.198031551615314161 ) ) ;
#3285=CARTESIAN_POINT ( 'NONE',  ( -213.1075012329537230, -9.698598906450557777, 9.698598906450415669 ) ) ;
#3287=EDGE_CURVE ( 'NONE', #26074, #19299, #4849, .T. ) ;
#3288=CARTESIAN_POINT ( 'NONE',  ( 14.38125909742181108, -5.035366881890652543E-14, 15.17850393972633682 ) ) ;
#3289=CARTESIAN_POINT ( 'NONE',  ( 200.0000000000000000, -14.14213562373122457, 42.42640687119282461 ) ) ;
#3290=ADVANCED_FACE ( 'NONE', ( #17095 ), #16203, .T. ) ;
#3291=CARTESIAN_POINT ( 'NONE',  ( 170.2234770963711128, 15.44714144992818738, 40.00000000000002132 ) ) ;
#3292=VERTEX_POINT ( 'NONE', #6692 ) ;
#3293=CARTESIAN_POINT ( 'NONE',  ( 91.82158438592158234, 16.11829626348434630, -40.45024623143955012 ) ) ;
#3294=CARTESIAN_POINT ( 'NONE',  ( -103.9474983245022344, -20.15710290851514586, -8.027156558344424653 ) ) ;
#3295=CARTESIAN_POINT ( 'NONE',  ( 25.62979979007943498, 13.63460241475089951, 45.99287499157590275 ) ) ;
#3296=CARTESIAN_POINT ( 'NONE',  ( -77.90255099906873681, -20.04994828523928163, -8.644468104261223473 ) ) ;
#3297=EDGE_CURVE ( 'NONE', #12216, #8800, #5759, .T. ) ;
#3298=EDGE_CURVE ( 'NONE', #4428, #12165, #2827, .T. ) ;
#3299=ORIENTED_EDGE ( 'NONE', *, *, #25921, .F. ) ;
#3300=CARTESIAN_POINT ( 'NONE',  ( -188.2956751479426885, -46.98904240251139441, 13.82790121914922388 ) ) ;
#3302=CARTESIAN_POINT ( 'NONE',  ( 22.95085416411796331, -17.86294511971716048, 43.12496437194802468 ) ) ;
#3303=CARTESIAN_POINT ( 'NONE',  ( 37.37129771754243279, 20.48130208294292842, -38.51719860168416432 ) ) ;
#3305=CARTESIAN_POINT ( 'NONE',  ( 190.0000000000001137, 3.490243377569959927E-14, 0.000000000000000000 ) ) ;
#3306=CARTESIAN_POINT ( 'NONE',  ( -162.0762913951021176, 39.99999999999998579, 1.694272876828463614 ) ) ;
#3307=CARTESIAN_POINT ( 'NONE',  ( -87.11181979037108647, -2.713702011544433912, 21.35018875643972081 ) ) ;
#3308=( BOUNDED_SURFACE ( )  B_SPLINE_SURFACE ( 3, 2, ( 
 ( #17755, #18020, #13900 ),
 ( #11633, #13634, #19756 ),
 ( #13505, #23880, #11377 ),
 ( #3806, #1811, #7637 ),
 ( #5792, #3279, #5657 ),
 ( #13763, #19498, #9391 ),
 ( #25638, #15495, #23625 ),
 ( #5405, #21628, #3404 ),
 ( #11505, #19630, #6449 ),
 ( #20162, #26304, #10578 ),
 ( #14436, #2335, #20300 ),
 ( #12179, #12304, #8183 ),
 ( #12042, #1944, #10051 ),
 ( #4344, #20564, #18693 ),
 ( #3945, #6190, #24694 ),
 ( #18158, #6316, #8047 ) ),
 .UNSPECIFIED., .F., .F., .F. ) 
 B_SPLINE_SURFACE_WITH_KNOTS ( ( 4, 2, 2, 2, 2, 2, 2, 4 ),
 ( 3, 3 ),
 ( 0.04143342415524681882, 0.04862317170365706986, 0.05221804547786219192, 0.05401548236496475641, 0.05581291925206731397, 0.06300266680047755807, 0.06659754057468268706, 0.07019241434888781606 ),
 ( 0.000000000000000000, 1.000000000000000000 ),
 .UNSPECIFIED. ) 
 GEOMETRIC_REPRESENTATION_ITEM ( )  RATIONAL_B_SPLINE_SURFACE ( (
 ( 1.000000000000000000, 0.9541700777564458003, 1.000000000000000000),
 ( 1.000000000000000000, 0.9519624585090378233, 1.000000000000000000),
 ( 1.000000000000000000, 0.9502408728421397610, 1.000000000000000000),
 ( 1.000000000000000000, 0.9485093239120891973, 1.000000000000000000),
 ( 1.000000000000000000, 0.9480808157489741816, 1.000000000000000000),
 ( 1.000000000000000000, 0.9476673512789849374, 1.000000000000000000),
 ( 1.000000000000000000, 0.9475676663659571286, 1.000000000000000000),
 ( 1.000000000000000000, 0.9474462208978693400, 1.000000000000000000),
 ( 1.000000000000000000, 0.9474241303505198664, 1.000000000000000000),
 ( 1.000000000000000000, 0.9475034751962024826, 1.000000000000000000),
 ( 1.000000000000000000, 0.9481710333135665580, 1.000000000000000000),
 ( 1.000000000000000000, 0.9500557947230517941, 1.000000000000000000),
 ( 1.000000000000000000, 0.9508368636698915077, 1.000000000000000000),
 ( 1.000000000000000000, 0.9526500836528452032, 1.000000000000000000),
 ( 1.000000000000000000, 0.9536844903836366738, 1.000000000000000000),
 ( 1.000000000000000000, 0.9548353292492207656, 1.000000000000000000) ) ) 
 REPRESENTATION_ITEM ( '' )  SURFACE ( )  );
#3309=CARTESIAN_POINT ( 'NONE',  ( 18.89824444022306338, 48.20791849611975266, -14.00990882958417671 ) ) ;
#3310=CARTESIAN_POINT ( 'NONE',  ( -162.0762913951020607, -41.69427287692683848, 40.00000000000002132 ) ) ;
#3311=CARTESIAN_POINT ( 'NONE',  ( 37.15749683987841223, -12.76981037570312694, -41.79699086507935135 ) ) ;
#3313=CARTESIAN_POINT ( 'NONE',  ( -30.26275506840324425, -1.694272468446265334, 40.00000000000002132 ) ) ;
#3314=CARTESIAN_POINT ( 'NONE',  ( -135.8532207217289738, 9.153146818113546246, -0.000000000000000000 ) ) ;
#3315=CARTESIAN_POINT ( 'NONE',  ( 170.2234770963711128, -2.259079968736224833E-13, 24.55285855007187124 ) ) ;
#3316=CARTESIAN_POINT ( 'NONE',  ( 200.0000000000000000, -39.99999999999977973, -20.00000000000034817 ) ) ;
#3317=CARTESIAN_POINT ( 'NONE',  ( 99.57966121244446356, -18.94872250966755090, -7.848817853148193358 ) ) ;
#3320=CARTESIAN_POINT ( 'NONE',  ( 6.011245401515337150, 44.78331514753590881, -18.54985650214099380 ) ) ;
#3321=CARTESIAN_POINT ( 'NONE',  ( 130.8568914410475372, -5.949712681206667853, -2.449293598294708485E-15 ) ) ;
#3323=CARTESIAN_POINT ( 'NONE',  ( -189.0115211946964848, 43.33403054566065293, -17.94954316430204955 ) ) ;
#3325=ORIENTED_EDGE ( 'NONE', *, *, #11896, .T. ) ;
#3327=CARTESIAN_POINT ( 'NONE',  ( 163.1118516004056573, 19.27778845538780317, -19.27778845538757224 ) ) ;
#3333=CARTESIAN_POINT ( 'NONE',  ( -213.1075012329537230, 66.26714140136188291, 9.698598906438215650 ) ) ;
#3334=CARTESIAN_POINT ( 'NONE',  ( -105.2054292635174733, -1.371496932086386566, -21.49321519473988573 ) ) ;
#3335=CARTESIAN_POINT ( 'NONE',  ( 170.2234770963711128, 1.169953928977015745E-13, -24.55285855007187124 ) ) ;
#3336=CARTESIAN_POINT ( 'NONE',  ( -105.3841224671147216, -9.645501175099258973, -19.11844758208756545 ) ) ;
#3338=CARTESIAN_POINT ( 'NONE',  ( 184.8905102610680444, -39.99999999999978684, -19.07866798485600768 ) ) ;
#3339=CARTESIAN_POINT ( 'NONE',  ( 91.82158438592156813, 40.00000000000027711, -22.79471317813428044 ) ) ;
#3340=CARTESIAN_POINT ( 'NONE',  ( -114.7827252410686754, -16.13252424103086824, 15.16659028666128073 ) ) ;
#3341=CARTESIAN_POINT ( 'NONE',  ( -213.1075012329537230, -37.98287015391232302, -18.58567234101164800 ) ) ;
#3342=CARTESIAN_POINT ( 'NONE',  ( 91.82158438592158234, 7.693928927950222250E-14, -17.20528682183300262 ) ) ;
#3343=CARTESIAN_POINT ( 'NONE',  ( 136.1360204305621266, 24.77266263493138965, -24.77266263493110188 ) ) ;
#3344=CARTESIAN_POINT ( 'NONE',  ( 149.5797498300189261, 29.41965740490872250, 12.18602109748340290 ) ) ;
#3346=CARTESIAN_POINT ( 'NONE',  ( -77.65678946166460150, 18.42186864996805440, -12.10857941959429596 ) ) ;
#3347=CARTESIAN_POINT ( 'NONE',  ( 130.8568914410475372, 24.07718906447243867, -24.07718906447216156 ) ) ;
#3348=CARTESIAN_POINT ( 'NONE',  ( 19.06497207195981147, -4.605042221739098431E-14, 14.19242893257840521 ) ) ;
#3349=CARTESIAN_POINT ( 'NONE',  ( 170.2234770963711128, -45.64576402573183600, 10.92277846919191653 ) ) ;
#3350=CARTESIAN_POINT ( 'NONE',  ( 91.82158438592159655, -16.11829626346125011, -16.11829626346154853 ) ) ;
#3351=CARTESIAN_POINT ( 'NONE',  ( -121.8425463773527326, -9.420908034907393258, -22.74408395655231274 ) ) ;
#3352=ORIENTED_EDGE ( 'NONE', *, *, #17746, .F. ) ;
#3353=CARTESIAN_POINT ( 'NONE',  ( 57.59792236341147031, -1.722363176414363206, -54.84617931850881689 ) ) ;
#3357=CARTESIAN_POINT ( 'NONE',  ( -192.9588430854689989, 1.161019517985663313E-13, -14.46834944099969533 ) ) ;
#3359=CARTESIAN_POINT ( 'NONE',  ( -62.79433447051992090, 11.74096317487346042, 24.94280497462943558 ) ) ;
#3360=VERTEX_POINT ( 'NONE', #14942 ) ;
#3361=ORIENTED_EDGE ( 'NONE', *, *, #5308, .F. ) ;
#3362=CARTESIAN_POINT ( 'NONE',  ( -192.9370379452147972, -48.35015161802368056, -14.03127537977354855 ) ) ;
#3364=CARTESIAN_POINT ( 'NONE',  ( 136.1360204305621551, 40.00000000000002842, 4.966164525587208445 ) ) ;
#3368=CARTESIAN_POINT ( 'NONE',  ( -30.26275506840323359, -40.00000000000017053, 41.69427246844613677 ) ) ;
#3370=CARTESIAN_POINT ( 'NONE',  ( -30.26275506840325136, 40.00000000000001421, 1.694272468446399227 ) ) ;
#3371=B_SPLINE_CURVE_WITH_KNOTS ( 'NONE', 3,
 ( #315, #18533, #4188, #4444, #22540, #8416, #6039, #44, #20138, #12537, #7882, #12410, #24129, #20409 ),
 .UNSPECIFIED., .F., .F.,
 ( 4, 2, 2, 2, 2, 2, 4 ),
 ( 6.938893903907228378E-18, 0.002941681445496991537, 0.004412522168245485571, 0.005883362890993980472, 0.008825044336490969407, 0.01029588505923945650, 0.01176672578198794533 ),
 .UNSPECIFIED. ) ;
#3372=EDGE_CURVE ( 'NONE', #12121, #6926, #20388, .T. ) ;
#3374=CARTESIAN_POINT ( 'NONE',  ( -7.233308327731263532, -17.51119053152957150, -42.27575367454436872 ) ) ;
#3375=CARTESIAN_POINT ( 'NONE',  ( 163.1118516004056573, 47.56205970284970164, -9.006482792073828847 ) ) ;
#3377=CARTESIAN_POINT ( 'NONE',  ( 184.8905102610680444, 40.00000000000025580, -19.07866798485515503 ) ) ;
#3379=CARTESIAN_POINT ( 'NONE',  ( 0.2972598230769983307, -14.33493731733933352, 40.00000000000002132 ) ) ;
#3380=CARTESIAN_POINT ( 'NONE',  ( -100.7734535825088500, 22.67402823373189946, -40.00000000000002132 ) ) ;
#3381=EDGE_CURVE ( 'NONE', #8098, #817, #24818, .T. ) ;
#3382=CARTESIAN_POINT ( 'NONE',  ( -100.7734535825088500, 16.03295912088713848, -16.03295912088698927 ) ) ;
#3383=CARTESIAN_POINT ( 'NONE',  ( 0.2972598230769983307, -14.33493731733933352, -40.00000000000002132 ) ) ;
#3384=CARTESIAN_POINT ( 'NONE',  ( 20.59039453120236018, -43.61606461192724282, -23.90179120638650900 ) ) ;
#3385=CARTESIAN_POINT ( 'NONE',  ( -86.84962968273566730, 19.67999904273991163, 8.151722510992470916 ) ) ;
#3386=CARTESIAN_POINT ( 'NONE',  ( -114.6415077203361221, 21.36885048555677358, -5.448690899135370636 ) ) ;
#3387=CARTESIAN_POINT ( 'NONE',  ( -91.56559293963834989, 40.53558337403677569, -16.03295912088699993 ) ) ;
#3388=CARTESIAN_POINT ( 'NONE',  ( 57.59792236341147031, 37.56421063658187620, 2.449293598294708485E-15 ) ) ;
#3389=EDGE_LOOP ( 'NONE', ( #826, #17331, #17714, #7244 ) ) ;
#3392=CARTESIAN_POINT ( 'NONE',  ( 44.82887508589845993, -36.15717056698611742, 18.94256811206760105 ) ) ;
#3394=CARTESIAN_POINT ( 'NONE',  ( 136.1360204305621551, -53.05693388239313890, 3.511608612530593199 ) ) ;
#3395=CARTESIAN_POINT ( 'NONE',  ( -105.3755690713226585, -39.99999999999996447, -21.75974354311664527 ) ) ;
#3396=CARTESIAN_POINT ( 'NONE',  ( -82.26983156992163515, 19.48351608823322678, -5.272298809006593423 ) ) ;
#3397=CARTESIAN_POINT ( 'NONE',  ( -259.2033419157646676, -9.517827891722680178, 0.000000000000000000 ) ) ;
#3400=CARTESIAN_POINT ( 'NONE',  ( 170.0000000000000284, 15.47746304364896019, 19.80854622259152720 ) ) ;
#3401=CARTESIAN_POINT ( 'NONE',  ( -105.3755690713226727, -15.38646221621807619, 15.38646221621768362 ) ) ;
#3402=CARTESIAN_POINT ( 'NONE',  ( -208.1127848780264742, -10.60833733270725787, -67.17687982763172272 ) ) ;
#3404=CARTESIAN_POINT ( 'NONE',  ( -114.7820862557368997, 22.12833180681263556, -0.4894207860022879442 ) ) ;
#3405=CARTESIAN_POINT ( 'NONE',  ( -86.86493150571057242, 8.366608963945132871, -19.60045294883092382 ) ) ;
#3406=CARTESIAN_POINT ( 'NONE',  ( -208.1127848780264742, -10.60833733270725787, -67.17687982763172272 ) ) ;
#3407=CARTESIAN_POINT ( 'NONE',  ( -162.0762913951020892, -1.198031840315659124, -57.76657433523998009 ) ) ;
#3408=CARTESIAN_POINT ( 'NONE',  ( -213.1075012329537230, -18.58567234101102272, -37.98287015391260013 ) ) ;
#3409=CARTESIAN_POINT ( 'NONE',  ( -192.9588430854689989, 10.23066800230756712, -10.23066800230735396 ) ) ;
#3411=CARTESIAN_POINT ( 'NONE',  ( 107.5473083967439720, 23.99138244111466989, 0.000000000000000000 ) ) ;
#3412=CARTESIAN_POINT ( 'NONE',  ( 0.2972598230770103767, -40.00000000000021316, 54.33493731733921805 ) ) ;
#3414=CARTESIAN_POINT ( 'NONE',  ( -213.1075012329537230, 53.71589010951910836, 2.449293598294708485E-15 ) ) ;
#3416=CARTESIAN_POINT ( 'NONE',  ( -86.96347745069644475, 12.89780903124410472, -43.67073346367977393 ) ) ;
#3417=CARTESIAN_POINT ( 'NONE',  ( 89.37937299509916045, 21.71466159691463815, 8.994507335784314606 ) ) ;
#3418=CARTESIAN_POINT ( 'NONE',  ( 90.68848423392005031, 8.814708751053737856, 21.28058941705803164 ) ) ;
#3419=CARTESIAN_POINT ( 'NONE',  ( -70.30307074936186496, -22.52851052426727207, -10.20829450353408596 ) ) ;
#3421=CARTESIAN_POINT ( 'NONE',  ( -195.5009199109952363, -44.52807166370936187, 18.44413118942235386 ) ) ;
#3423=CARTESIAN_POINT ( 'NONE',  ( 27.26078259667537296, -17.35591035708258545, 41.90087417143249837 ) ) ;
#3429=CARTESIAN_POINT ( 'NONE',  ( 200.0000000000000000, 40.00000000000012790, -19.99999999999996092 ) ) ;
#3430=CARTESIAN_POINT ( 'NONE',  ( -82.24286369198219404, -2.516305986770045688, 20.07657290678962170 ) ) ;
#3431=CARTESIAN_POINT ( 'NONE',  ( -200.0000000000001421, -14.17215463606902404, -49.28189405767602693 ) ) ;
#3432=CARTESIAN_POINT ( 'NONE',  ( 14.38125909742181285, -15.17850393972633505, 40.00000000000002132 ) ) ;
#3436=EDGE_CURVE ( 'NONE', #23332, #16255, #7824, .T. ) ;
#3437=CARTESIAN_POINT ( 'NONE',  ( -192.9588430854689989, -14.46834944099973086, 0.000000000000000000 ) ) ;
#3438=CARTESIAN_POINT ( 'NONE',  ( -259.2033419157646676, -30.48217210827743884, -40.00000000000002132 ) ) ;
#3440=CARTESIAN_POINT ( 'NONE',  ( 192.4448373802100889, -20.00000000003938538, 0.000000000000000000 ) ) ;
#3441=CARTESIAN_POINT ( 'NONE',  ( 199.9999999999999432, -1.727494763561684666E-13, 20.00000000000010303 ) ) ;
#3445=CARTESIAN_POINT ( 'NONE',  ( 132.4329763957084936, -29.78197873630821491, -12.33609950688606105 ) ) ;
#3447=CARTESIAN_POINT ( 'NONE',  ( 98.29820294267355507, 10.58389073156783233, -16.98253775143902544 ) ) ;
#3448=CARTESIAN_POINT ( 'NONE',  ( -2.557884977113219716, 43.43882039326797440, -23.77085849411954044 ) ) ;
#3449=CARTESIAN_POINT ( 'NONE',  ( -280.0000000000000568, 19.99999999999996092, 40.00000000000002132 ) ) ;
#3453=ORIENTED_EDGE ( 'NONE', *, *, #11657, .F. ) ;
#3454=CARTESIAN_POINT ( 'NONE',  ( -162.0762913951020892, -1.198031840385783919, 1.198031840385741731 ) ) ;
#3456=ORIENTED_EDGE ( 'NONE', *, *, #21627, .T. ) ;
#3457=CARTESIAN_POINT ( 'NONE',  ( -103.9474983244994490, 8.027156558344955783, -20.15710290851550113 ) ) ;
#3460=CIRCLE ( 'NONE', #18320, 69.99999999999994316 ) ;
#3461=CARTESIAN_POINT ( 'NONE',  ( 169.9999999999999432, 22.62041470344884075, 9.369682556672378482 ) ) ;
#3462=CARTESIAN_POINT ( 'NONE',  ( -56.48582580120559982, 50.09629031063966664, -6.472252184284094767 ) ) ;
#3464=( BOUNDED_CURVE ( )  B_SPLINE_CURVE ( 3, ( #22414, #8556, #16672, #20411 ),
 .UNSPECIFIED., .F., .F. ) 
 B_SPLINE_CURVE_WITH_KNOTS ( ( 4, 4 ),
 ( 0.007854122480096750389, 0.01576650722528986220 ),
 .UNSPECIFIED. ) 
 CURVE ( )  GEOMETRIC_REPRESENTATION_ITEM ( )  RATIONAL_B_SPLINE_CURVE ( ( 0.9999999999999497069, 0.8893928793063790028, 0.7971366613349945007, 0.7232313460858209586 ) ) 
 REPRESENTATION_ITEM ( '' )  );
#3465=CARTESIAN_POINT ( 'NONE',  ( -91.56559293963834989, 6.234561990864368500E-14, -22.67402823373191723 ) ) ;
#3468=CARTESIAN_POINT ( 'NONE',  ( -65.65555754753384576, 11.16466304451119207, -24.04429191298344293 ) ) ;
#3469=CARTESIAN_POINT ( 'NONE',  ( -162.0762913951020892, -1.202636532414034422E-14, -1.694272876828323948 ) ) ;
#3470=CARTESIAN_POINT ( 'NONE',  ( -162.0762913951020892, -39.99999999999961631, -41.69427287692722928 ) ) ;
#3471=CARTESIAN_POINT ( 'NONE',  ( -200.0000000000000853, -46.19968414209463958, -18.59955921182009320 ) ) ;
#3472=CARTESIAN_POINT ( 'NONE',  ( 130.8568914410475088, -4.207082182989324792, -52.36146031193423056 ) ) ;
#3473=CARTESIAN_POINT ( 'NONE',  ( -199.9999999999999716, 16.85576820966628375, -47.13392792188996339 ) ) ;
#3474=EDGE_CURVE ( 'NONE', #16387, #11522, #2624, .T. ) ;
#3475=CARTESIAN_POINT ( 'NONE',  ( 14.38125909742183062, -67.30136555898262429, 10.73282306405838682 ) ) ;
#3476=CARTESIAN_POINT ( 'NONE',  ( 98.29820294267314296, 18.47759065023127079, 7.653668647304074923 ) ) ;
#3479=CARTESIAN_POINT ( 'NONE',  ( -192.9588430854689989, -8.596193650988133061E-14, 14.46834944099969533 ) ) ;
#3480=CARTESIAN_POINT ( 'NONE',  ( 136.1360204305621551, -24.77266263493126885, 31.79587985999256006 ) ) ;
#3482=CARTESIAN_POINT ( 'NONE',  ( 146.6084372240433709, -32.08495691632075619, 24.48358557860298035 ) ) ;
#3483=CARTESIAN_POINT ( 'NONE',  ( -151.4802930569721582, -11.09498731348586809, -33.96623840869666111 ) ) ;
#3484=CARTESIAN_POINT ( 'NONE',  ( -99.21568817060989431, 16.03295912088691821, 16.03295912088721309 ) ) ;
#3485=ORIENTED_EDGE ( 'NONE', *, *, #16965, .T. ) ;
#3486=CARTESIAN_POINT ( 'NONE',  ( -192.9588430854689989, 38.51493924976983152, -38.51493924976893624 ) ) ;
#3487=CARTESIAN_POINT ( 'NONE',  ( -397.9898987322331436, 69.99999999999990052, 0.000000000000000000 ) ) ;
#3489=CARTESIAN_POINT ( 'NONE',  ( -82.23726319249651340, -1.560758868889668476E-13, 20.19517362732914734 ) ) ;
#3490=EDGE_LOOP ( 'NONE', ( #23899, #8227, #21798, #19049, #6930, #1071, #22614, #7062, #14089, #10565, #17173, #6596, #1301, #5112, #2291, #13494 ) ) ;
#3491=CARTESIAN_POINT ( 'NONE',  ( 130.8568914410475372, -3.326198072800416995E-13, 34.05028731879788495 ) ) ;
#3492=CARTESIAN_POINT ( 'NONE',  ( -1.255560987024274322, -23.98612781107772918, 43.73013506549201423 ) ) ;
#3493=CARTESIAN_POINT ( 'NONE',  ( -65.65550967573656749, 11.16467289560276122, 24.04430752631849799 ) ) ;
#3494=EDGE_LOOP ( 'NONE', ( #17738, #5415, #9928, #20149, #22246, #12129, #8634 ) ) ;
#3496=CARTESIAN_POINT ( 'NONE',  ( 14.38125909742180752, 55.17850393971008316, -40.00000000000002132 ) ) ;
#3497=CARTESIAN_POINT ( 'NONE',  ( -280.0000000000000568, -14.14213562373078226, -42.42640687119295251 ) ) ;
#3498=CARTESIAN_POINT ( 'NONE',  ( -280.0000000000000568, 39.99999999999990763, 20.00000000000015987 ) ) ;
#3499=CARTESIAN_POINT ( 'NONE',  ( -114.7826396787322665, -15.64922767586156915, -15.64922767586183383 ) ) ;
#3501=DIRECTION ( 'NONE',  ( 1.000000000000000000, 1.836970198721030181E-16, 0.000000000000000000 ) ) ;
#3502=CARTESIAN_POINT ( 'NONE',  ( 136.1360204305621551, 39.99999999999968026, 35.03383547441337953 ) ) ;
#3503=CARTESIAN_POINT ( 'NONE',  ( 192.4448373802101173, -40.00000000000005684, 19.99999999996046185 ) ) ;
#3505=CARTESIAN_POINT ( 'NONE',  ( 91.82158438592156813, 40.00000000000009948, -17.20528682183286051 ) ) ;
#3506=CARTESIAN_POINT ( 'NONE',  ( -190.0000000000001705, 69.99999999999994316, 0.000000000000000000 ) ) ;
#3507=CARTESIAN_POINT ( 'NONE',  ( -105.3755690713226727, -15.38646221621807619, 15.38646221621768362 ) ) ;
#3508=CARTESIAN_POINT ( 'NONE',  ( -192.9588430854690273, -10.23066800231931239, -66.79921049724377724 ) ) ;
#3509=CARTESIAN_POINT ( 'NONE',  ( 136.1360204305621266, -24.77266263493151044, 24.77266263493093135 ) ) ;
#3510=CARTESIAN_POINT ( 'NONE',  ( -259.2033419157646676, -1.473088368616265084E-13, 9.517827891722632216 ) ) ;
#3512=CARTESIAN_POINT ( 'NONE',  ( 4.995406935893293543, -15.24977328854832592, 0.000000000000000000 ) ) ;
#3513=CARTESIAN_POINT ( 'NONE',  ( -192.9588430854690273, -54.46834944101725284, -40.00000000000002132 ) ) ;
#3514=CARTESIAN_POINT ( 'NONE',  ( 57.59792236341147031, 1.722363176415065089, -1.722363176415036445 ) ) ;
#3515=CARTESIAN_POINT ( 'NONE',  ( 19.06497207195981503, -14.19242893257840166, 0.000000000000000000 ) ) ;
#3516=CARTESIAN_POINT ( 'NONE',  ( 7.307793593482452721, -44.91153572052488840, -24.85783611765727485 ) ) ;
#3517=CARTESIAN_POINT ( 'NONE',  ( -259.2033419157646676, 39.99999999999987921, 9.517827891723049660 ) ) ;
#3518=CARTESIAN_POINT ( 'NONE',  ( -100.7734535825088358, 12.25131212657480440, 12.25131212657487012 ) ) ;
#3519=CARTESIAN_POINT ( 'NONE',  ( -162.0762913951020892, 41.69427287682832173, 2.449293598294708485E-15 ) ) ;
#3521=CARTESIAN_POINT ( 'NONE',  ( 23.40652632867992367, -42.84715492600945197, 23.33303889678550647 ) ) ;
#3523=CARTESIAN_POINT ( 'NONE',  ( 192.4448373802100889, 14.14213562370310662, 14.14213562370312438 ) ) ;
#3524=CARTESIAN_POINT ( 'NONE',  ( 14.38125909742181818, -1.924622159709266762E-13, 55.17850393972636880 ) ) ;
#3525=CARTESIAN_POINT ( 'NONE',  ( -135.8532207217289738, -6.472252184284280396, 6.472252184284099208 ) ) ;
#3526=CARTESIAN_POINT ( 'NONE',  ( -192.9588430854690273, 14.46834944099966336, -40.00000000000002132 ) ) ;
#3529=CARTESIAN_POINT ( 'NONE',  ( -87.02115643441359794, 5.416235655370554625, -20.76466217920002677 ) ) ;
#3530=CARTESIAN_POINT ( 'NONE',  ( -56.48582580120559271, -6.472252184284276844, 6.472252184284108978 ) ) ;
#3531=CARTESIAN_POINT ( 'NONE',  ( -162.0762913951020892, -29.48230308784744125, -29.48230308784792442 ) ) ;
#3533=CARTESIAN_POINT ( 'NONE',  ( -77.55640685876512919, -22.13135000837101884, -1.398618882111774653 ) ) ;
#3534=CARTESIAN_POINT ( 'NONE',  ( -86.90968602919654984, 19.36074508458825605, -9.002619558036901282 ) ) ;
#3535=CARTESIAN_POINT ( 'NONE',  ( 151.7948205124835681, 51.78348778862544322, -4.785054706298002891 ) ) ;
#3536=CARTESIAN_POINT ( 'NONE',  ( 146.6084372240433709, 52.76785682606523409, -3.800685668858194255 ) ) ;
#3537=CARTESIAN_POINT ( 'NONE',  ( -192.9588430854690273, 10.23066800229588758, -66.79921049721882298 ) ) ;
#3538=CARTESIAN_POINT ( 'NONE',  ( 146.6084372240433709, -24.48358557860284179, -32.08495691632087699 ) ) ;
#3539=FACE_OUTER_BOUND ( 'NONE', #4304, .T. ) ;
#3540=CARTESIAN_POINT ( 'NONE',  ( 91.82158438592158234, -12.16597498397761967, -12.16597498397768007 ) ) ;
#3542=CARTESIAN_POINT ( 'NONE',  ( -135.8532207217289738, -40.00000000000001421, -9.153146818113709671 ) ) ;
#3543=CARTESIAN_POINT ( 'NONE',  ( -30.26275506840323359, -1.198031551616339341, 57.76657404653985139 ) ) ;
#3544=CARTESIAN_POINT ( 'NONE',  ( -91.56559293963836410, 16.03295912088692177, 16.03295912088721664 ) ) ;
#3545=CARTESIAN_POINT ( 'NONE',  ( -280.0000000000000568, 19.99999999999995737, 40.00000000000002132 ) ) ;
#3547=CARTESIAN_POINT ( 'NONE',  ( -192.9588430854689989, 10.23066800230742679, 10.23066800230749607 ) ) ;
#3550=CARTESIAN_POINT ( 'NONE',  ( 57.59792236341147031, -2.435789363418150444, 0.000000000000000000 ) ) ;
#3552=CARTESIAN_POINT ( 'NONE',  ( -189.2667466962258231, -43.39859272266359369, 17.97628569363223505 ) ) ;
#3554=CARTESIAN_POINT ( 'NONE',  ( 98.29820294267315717, -7.653668647304114891, 18.47759065023121039 ) ) ;
#3555=CARTESIAN_POINT ( 'NONE',  ( 23.10188454848542605, 13.81611343686443405, -46.91040837924335705 ) ) ;
#3558=CARTESIAN_POINT ( 'NONE',  ( 136.1360204305621551, 40.00000000000002842, 4.966164525587208445 ) ) ;
#3559=CARTESIAN_POINT ( 'NONE',  ( -82.23726319249655603, -1.556969561919214781E-13, 20.19517362732914734 ) ) ;
#3560=CARTESIAN_POINT ( 'NONE',  ( -200.0000000000000000, -20.93268228684324939, -45.36622447512537093 ) ) ;
#3561=CARTESIAN_POINT ( 'NONE',  ( -280.0000000000000568, -20.00000000000007105, 40.00000000000002132 ) ) ;
#3562=CARTESIAN_POINT ( 'NONE',  ( -184.9730489280194945, 13.59277546670732661, -45.83721239347746490 ) ) ;
#3565=CARTESIAN_POINT ( 'NONE',  ( 57.59792236341147031, 2.435789363418171760, 0.000000000000000000 ) ) ;
#3566=CARTESIAN_POINT ( 'NONE',  ( 19.06497207195980792, 14.19242893257840876, 0.000000000000000000 ) ) ;
#3567=CARTESIAN_POINT ( 'NONE',  ( 19.06497207195982924, -39.99999999999945288, -54.19242893257885640 ) ) ;
#3568=CARTESIAN_POINT ( 'NONE',  ( 0.2972598230769957217, 1.502051041545559470E-13, -14.33493731733933352 ) ) ;
#3570=CARTESIAN_POINT ( 'NONE',  ( -213.1075012329537230, 18.58567234101174037, -37.98287015391222354 ) ) ;
#3572=DIRECTION ( 'NONE',  ( 0.01051738792034368278, 0.3995761383040613568, 0.9166396752537755432 ) ) ;
#3573=CARTESIAN_POINT ( 'NONE',  ( 4.995406935893293543, -15.24977328854832592, 0.000000000000000000 ) ) ;
#3575=CARTESIAN_POINT ( 'NONE',  ( -198.0012400611977057, 49.19397081476455469, -14.15884001207452592 ) ) ;
#3577=VERTEX_POINT ( 'NONE', #13331 ) ;
#3580=CARTESIAN_POINT ( 'NONE',  ( 22.79879570922434695, -43.16776802602853280, -17.88067497375694970 ) ) ;
#3582=CARTESIAN_POINT ( 'NONE',  ( -105.3755690713226585, 18.24025645688350750, -40.00000000000002132 ) ) ;
#3586=DIRECTION ( 'NONE',  ( 0.000000000000000000, -0.3656393565213487129, 0.9307566067252244224 ) ) ;
#3587=CARTESIAN_POINT ( 'NONE',  ( -280.0000000000000000, 14.14213562373088351, 14.14213562373098654 ) ) ;
#3589=CARTESIAN_POINT ( 'NONE',  ( -259.2033419157646676, -1.438356298054549103E-14, -9.517827891722632216 ) ) ;
#3594=CARTESIAN_POINT ( 'NONE',  ( -100.7734535825088500, -39.99999999999986500, -17.32597176626853397 ) ) ;
#3595=CARTESIAN_POINT ( 'NONE',  ( -199.9999999999999432, -44.86773131993655994, -24.32899771311787518 ) ) ;
#3596=B_SPLINE_CURVE_WITH_KNOTS ( 'NONE', 3,
 ( #3257, #25875, #9248, #26016, #7619, #11753, #23605, #15734 ),
 .UNSPECIFIED., .F., .F.,
 ( 4, 2, 2, 4 ),
 ( 0.008473926332009199328, 0.01052499632800952059, 0.01257606632400984359, 0.01667820631601048265 ),
 .UNSPECIFIED. ) ;
#3597=CARTESIAN_POINT ( 'NONE',  ( -162.0762913951021176, -29.48230308784755493, -27.08623940707632372 ) ) ;
#3598=CARTESIAN_POINT ( 'NONE',  ( -208.1127848780265026, -15.00245453012673202, 0.000000000000000000 ) ) ;
#3599=CARTESIAN_POINT ( 'NONE',  ( -259.2033419157646676, -21.55415060305854524, 21.55415060305827524 ) ) ;
#3600=DIRECTION ( 'NONE',  ( -0.01051738777840956381, -0.9166396752739809362, -0.3995761382614453905 ) ) ;
#3601=CARTESIAN_POINT ( 'NONE',  ( -3.763361371728476623, -47.08953757622906267, 13.84281709279670380 ) ) ;
#3602=CARTESIAN_POINT ( 'NONE',  ( -280.0000000000000568, 39.99999999999976552, 20.00000000000043343 ) ) ;
#3603=CARTESIAN_POINT ( 'NONE',  ( -162.0762913951020892, -3.568845385355699554E-14, 1.694272876828323948 ) ) ;
#3604=CARTESIAN_POINT ( 'NONE',  ( 146.6084372240433709, -24.48358557860329299, 32.08495691632052882 ) ) ;
#3605=CARTESIAN_POINT ( 'NONE',  ( 0.2972598230769976091, -10.13633138497465147, -10.13633138497482733 ) ) ;
#3606=CARTESIAN_POINT ( 'NONE',  ( -189.1288815661887099, -23.62384257861826597, -43.24061771117260378 ) ) ;
#3607=CARTESIAN_POINT ( 'NONE',  ( -91.56559293963836410, -12.25131212657462321, -44.31723036834905827 ) ) ;
#3608=ORIENTED_EDGE ( 'NONE', *, *, #2296, .T. ) ;
#3609=CARTESIAN_POINT ( 'NONE',  ( -162.0762913951020892, 1.198031840456041497, -57.76657433537918251 ) ) ;
#3610=CARTESIAN_POINT ( 'NONE',  ( -238.4067589809705794, -0.9644942799826263791, -40.00000000000002132 ) ) ;
#3612=CARTESIAN_POINT ( 'NONE',  ( -4.039451493210489907, 13.82811171175507603, -46.99046209229789639 ) ) ;
#3613=CARTESIAN_POINT ( 'NONE',  ( -86.96347745069644475, -15.38646221621738164, -41.18208027870615240 ) ) ;
#3617=CARTESIAN_POINT ( 'NONE',  ( 151.7948205124836250, -3.202120068677277203E-13, 33.23291073765553705 ) ) ;
#3619=EDGE_CURVE ( 'NONE', #15141, #22947, #10886, .T. ) ;
#3620=CARTESIAN_POINT ( 'NONE',  ( -17.28139728211933956, 20.85871090886837109, 39.07633224434955821 ) ) ;
#3621=ORIENTED_EDGE ( 'NONE', *, *, #5241, .F. ) ;
#3622=ORIENTED_EDGE ( 'NONE', *, *, #11647, .T. ) ;
#3623=CARTESIAN_POINT ( 'NONE',  ( 130.8568914410475372, 5.949712681206715814, 2.449293598294708485E-15 ) ) ;
#3624=CARTESIAN_POINT ( 'NONE',  ( 14.38125909742181285, -10.73282306404727393, 10.73282306404716380 ) ) ;
#3625=CARTESIAN_POINT ( 'NONE',  ( -30.26275506840324425, 39.99999999999987210, 41.69427246844643520 ) ) ;
#3627=EDGE_CURVE ( 'NONE', #10094, #6927, #8937, .T. ) ;
#3628=CARTESIAN_POINT ( 'NONE',  ( -86.86493150571118349, -19.60045294882770506, 8.366608963953762412 ) ) ;
#3631=CARTESIAN_POINT ( 'NONE',  ( -56.48582580120559271, -1.062504017861011783E-13, 9.153146818113587102 ) ) ;
#3633=CIRCLE ( 'NONE', #4066, 14.99999999999999822 ) ;
#3634=CIRCLE ( 'NONE', #22755, 14.99999999999999822 ) ;
#3636=CARTESIAN_POINT ( 'NONE',  ( -4.112199523540028601, -13.82298295336114791, -46.96527782736897905 ) ) ;
#3637=CARTESIAN_POINT ( 'NONE',  ( 200.0000000000000000, 42.42640687119310172, -14.14213562373052646 ) ) ;
#3639=CARTESIAN_POINT ( 'NONE',  ( 130.8568914410475088, -4.207082182989324792, -52.36146031193423056 ) ) ;
#3640=CARTESIAN_POINT ( 'NONE',  ( -135.8532207217289738, -40.00000000000014211, 9.153146818113153671 ) ) ;
#3642=CARTESIAN_POINT ( 'NONE',  ( 130.8568914410475372, 34.05028731879791337, 0.000000000000000000 ) ) ;
#3643=CARTESIAN_POINT ( 'NONE',  ( -198.0356074513804572, -55.37879056874826489, 40.00000000000002132 ) ) ;
#3645=CARTESIAN_POINT ( 'NONE',  ( 151.7948205124835681, 51.78348778862537927, 4.785054706298732086 ) ) ;
#3647=CARTESIAN_POINT ( 'NONE',  ( -135.8532207217289454, -30.84685318188648750, -40.00000000000002132 ) ) ;
#3649=CARTESIAN_POINT ( 'NONE',  ( 57.59792236341147031, -1.493297263419786540E-14, 2.435789363418160658 ) ) ;
#3650=CARTESIAN_POINT ( 'NONE',  ( -213.1075012329537230, 37.98287015391228749, 37.98287015391245802 ) ) ;
#3651=CARTESIAN_POINT ( 'NONE',  ( -192.9588430854690273, 54.46834944098218756, -40.00000000000002132 ) ) ;
#3652=ORIENTED_EDGE ( 'NONE', *, *, #13762, .T. ) ;
#3655=CARTESIAN_POINT ( 'NONE',  ( -200.0000000000000853, -24.82633483071228753, -44.86878812508721381 ) ) ;
#3656=CARTESIAN_POINT ( 'NONE',  ( -30.26275506840325136, 29.48230279907798135, -27.08623969584585112 ) ) ;
#3657=CARTESIAN_POINT ( 'NONE',  ( -208.1127848780265026, -2.327190355601776466E-13, 55.00245453012672670 ) ) ;
#3658=CARTESIAN_POINT ( 'NONE',  ( -208.1127848780265026, 10.60833733269551615, -10.60833733269529766 ) ) ;
#3659=CARTESIAN_POINT ( 'NONE',  ( 136.1360204305621266, -3.419521671106983309E-13, 35.03383547441296741 ) ) ;
#3660=CARTESIAN_POINT ( 'NONE',  ( -91.56559293963834989, -22.67402823373193499, 0.000000000000000000 ) ) ;
#3664=CARTESIAN_POINT ( 'NONE',  ( -192.9588430854689989, 38.51493924976983152, -38.51493924976893624 ) ) ;
#3665=CARTESIAN_POINT ( 'NONE',  ( -86.96347745069643054, 15.38646221621821297, -41.18208027870583265 ) ) ;
#3666=CARTESIAN_POINT ( 'NONE',  ( 130.8568914410475372, 24.07718906447243867, -24.07718906447216156 ) ) ;
#3668=CARTESIAN_POINT ( 'NONE',  ( 163.1118516004056573, 47.56205970284970164, -9.006482792073828847 ) ) ;
#3670=CARTESIAN_POINT ( 'NONE',  ( 57.59792236341147031, 30.00663442387720181, -26.56190807104661289 ) ) ;
#3671=CARTESIAN_POINT ( 'NONE',  ( 14.38125909742181285, -17.55144818341421598, -39.01709431150935359 ) ) ;
#3672=CARTESIAN_POINT ( 'NONE',  ( 130.8568914410475088, -52.36146031193413108, -4.207082182990267150 ) ) ;
#3676=CARTESIAN_POINT ( 'NONE',  ( 130.8568914410475372, 1.429239637432775288E-13, -34.05028731879788495 ) ) ;
#3677=CARTESIAN_POINT ( 'NONE',  ( -56.48582580120559982, 34.75652343174597547, 21.81201906317791384 ) ) ;
#3679=CARTESIAN_POINT ( 'NONE',  ( -86.96347745069644475, -21.75974354311652093, 40.00000000000002132 ) ) ;
#3681=CARTESIAN_POINT ( 'NONE',  ( 19.06497207195980792, 66.60410523465817789, 10.03556273973446800 ) ) ;
#3683=CIRCLE ( 'NONE', #8352, 15.00000000000000178 ) ;
#3685=CARTESIAN_POINT ( 'NONE',  ( -213.1075012329537230, 13.71589010951907994, 0.000000000000000000 ) ) ;
#3687=CARTESIAN_POINT ( 'NONE',  ( -190.0144222803064338, -43.47820992357731029, 23.79986276082939156 ) ) ;
#3690=CARTESIAN_POINT ( 'NONE',  ( -3.434479974377895761, -17.93814274724460844, 43.30650750418254802 ) ) ;
#3692=CARTESIAN_POINT ( 'NONE',  ( 23.84827734669535459, 13.76599369847180121, -46.63681169410599381 ) ) ;
#3695=DIRECTION ( 'NONE',  ( 1.000000000000000000, 0.000000000000000000, 0.000000000000000000 ) ) ;
#3696=CIRCLE ( 'NONE', #4514, 15.00000000000000355 ) ;
#3697=CARTESIAN_POINT ( 'NONE',  ( -208.1127848780264742, 10.60833733268383483, -67.17687982760675425 ) ) ;
#3698=CARTESIAN_POINT ( 'NONE',  ( 0.2972598230769983307, -14.33493731733933352, 40.00000000000002132 ) ) ;
#3701=CARTESIAN_POINT ( 'NONE',  ( 4.995406935893293543, -15.24977328854832592, 0.000000000000000000 ) ) ;
#3702=B_SPLINE_CURVE_WITH_KNOTS ( 'NONE', 3,
 ( #7612, #19999, #5377, #23722, #13604, #1785, #25613, #7358 ),
 .UNSPECIFIED., .F., .F.,
 ( 4, 2, 2, 4 ),
 ( 0.008396858476685838471, 0.01250098582283842678, 0.01455304949591472267, 0.01660511316899102030 ),
 .UNSPECIFIED. ) ;
#3704=CARTESIAN_POINT ( 'NONE',  ( 130.8568914410475088, 34.05028731879790627, -40.00000000000002132 ) ) ;
#3705=CARTESIAN_POINT ( 'NONE',  ( -198.0356074513804572, 15.37879056873066830, 40.00000000000002132 ) ) ;
#3707=CARTESIAN_POINT ( 'NONE',  ( 163.1118516004056573, -39.99999999999986500, -12.73709011382517353 ) ) ;
#3708=CARTESIAN_POINT ( 'NONE',  ( 130.8568914410475372, -3.326198072800416995E-13, 34.05028731879788495 ) ) ;
#3709=CARTESIAN_POINT ( 'NONE',  ( 146.6084372240433993, 24.48358557860307272, 24.48358557860347418 ) ) ;
#3711=ORIENTED_EDGE ( 'NONE', *, *, #21113, .T. ) ;
#3712=CARTESIAN_POINT ( 'NONE',  ( -28.75808802781983076, 35.61482992978302775, -18.59445401971593270 ) ) ;
#3713=CARTESIAN_POINT ( 'NONE',  ( 151.7948205124836250, 33.23291073765556547, 0.000000000000000000 ) ) ;
#3714=CARTESIAN_POINT ( 'NONE',  ( -193.0908541284702551, 48.38978395451683667, -14.03723495791108533 ) ) ;
#3716=ORIENTED_EDGE ( 'NONE', *, *, #5638, .F. ) ;
#3718=CARTESIAN_POINT ( 'NONE',  ( -259.2033419157646676, -21.55415060305824326, -35.01439189186556433 ) ) ;
#3719=CARTESIAN_POINT ( 'NONE',  ( 37.37129771728702821, -41.71823991396121301, -12.75330473327949576 ) ) ;
#3720=ORIENTED_EDGE ( 'NONE', *, *, #1194, .T. ) ;
#3721=CARTESIAN_POINT ( 'NONE',  ( 14.38125909742180752, 55.17850393971008316, -40.00000000000002132 ) ) ;
#3726=CARTESIAN_POINT ( 'NONE',  ( -208.1127848780265026, 38.89260858015724409, 38.89260858015741462 ) ) ;
#3727=CARTESIAN_POINT ( 'NONE',  ( -188.8753834511964840, -43.29882472894603751, -17.93496043754511859 ) ) ;
#3728=CARTESIAN_POINT ( 'NONE',  ( 19.06497207195981147, -4.605042221739098431E-14, 14.19242893257840521 ) ) ;
#3729=CARTESIAN_POINT ( 'NONE',  ( 184.8905102610680444, -20.92133201514440799, 0.000000000000000000 ) ) ;
#3732=CARTESIAN_POINT ( 'NONE',  ( -162.0762913951021176, -40.00000000000005684, 1.694272876828184504 ) ) ;
#3733=CARTESIAN_POINT ( 'NONE',  ( -100.7734535825088358, -2.560096224687585342E-13, 22.67402823373191723 ) ) ;
#3734=CARTESIAN_POINT ( 'NONE',  ( -114.6297772182897319, -11.19545617568720886, 18.93772329700642842 ) ) ;
#3735=CARTESIAN_POINT ( 'NONE',  ( -100.7734535825088358, -12.25131212657493052, 12.25131212657478130 ) ) ;
#3736=CARTESIAN_POINT ( 'NONE',  ( 0.2972598230769983307, -14.33493731733933352, -40.00000000000002132 ) ) ;
#3737=CARTESIAN_POINT ( 'NONE',  ( -91.56559293963834989, -40.53558337403669753, -16.03295912088728770 ) ) ;
#3740=CARTESIAN_POINT ( 'NONE',  ( -238.4067589809705794, 39.99999999999999289, -0.9644942799821634161 ) ) ;
#3741=CARTESIAN_POINT ( 'NONE',  ( -91.56559293963834989, 6.234561990864368500E-14, -22.67402823373191723 ) ) ;
#3742=CARTESIAN_POINT ( 'NONE',  ( 0.2972598230769959993, 38.42060263243659080, 38.42060263243672580 ) ) ;
#3743=CARTESIAN_POINT ( 'NONE',  ( -114.7816107152219729, 16.24027016579831795, 15.05025810000610420 ) ) ;
#3744=CARTESIAN_POINT ( 'NONE',  ( -188.6013942375869590, -13.84412886956378586, -47.09843442133011138 ) ) ;
#3747=CARTESIAN_POINT ( 'NONE',  ( -100.7734535825088500, -44.31723036834885932, -12.25131212657538171 ) ) ;
#3748=CARTESIAN_POINT ( 'NONE',  ( 170.2234770963711128, 17.36149277827004411, -17.36149277826983095 ) ) ;
#3749=CARTESIAN_POINT ( 'NONE',  ( 151.7948205124836250, 33.23291073765556547, 0.000000000000000000 ) ) ;
#3750=LINE ( 'NONE', #24103, #17009 ) ;
#3751=CARTESIAN_POINT ( 'NONE',  ( 146.6084372240433709, -52.76785682606510619, -3.800685668859292043 ) ) ;
#3752=CARTESIAN_POINT ( 'NONE',  ( -200.5022929845069939, -18.58571294254629436, -44.86988025226661847 ) ) ;
#3753=CARTESIAN_POINT ( 'NONE',  ( -93.12335834970892279, 22.67402823373189946, -0.000000000000000000 ) ) ;
#3756=CARTESIAN_POINT ( 'NONE',  ( -4.039451493210483690, -23.44932283416618191, -43.00522595894033628 ) ) ;
#3757=CARTESIAN_POINT ( 'NONE',  ( -4.260882601034492900, 23.40615483283669818, 42.93997571557765269 ) ) ;
#3758=ORIENTED_EDGE ( 'NONE', *, *, #13522, .T. ) ;
#3760=CARTESIAN_POINT ( 'NONE',  ( -30.26275506840324070, 1.198031551616013601, 1.198031551616023371 ) ) ;
#3762=CARTESIAN_POINT ( 'NONE',  ( -110.0368417077424539, -7.441767003010021142, -18.74474319002755252 ) ) ;
#3763=CARTESIAN_POINT ( 'NONE',  ( -89.91498783729113597, -20.43892340019855780, -8.087768383230207192 ) ) ;
#3765=ADVANCED_FACE ( 'NONE', ( #14118 ), #5143, .T. ) ;
#3767=CARTESIAN_POINT ( 'NONE',  ( 91.82158438592158234, -1.633484621919921769E-13, 17.20528682183300262 ) ) ;
#3769=CARTESIAN_POINT ( 'NONE',  ( -82.24286375075958233, -20.07657133907689939, -2.516278881350180630 ) ) ;
#3773=CARTESIAN_POINT ( 'NONE',  ( -1.087763065866631962, -13.97201973055225466, -47.95583523904139156 ) ) ;
#3775=CARTESIAN_POINT ( 'NONE',  ( 199.9999999999999432, -14.14213562373073607, -14.14213562373102206 ) ) ;
#3776=CARTESIAN_POINT ( 'NONE',  ( -105.4741150117398263, -19.77569912953930498, 7.943527260776862775 ) ) ;
#3777=CARTESIAN_POINT ( 'NONE',  ( -213.1075012329537230, -66.26714140138676612, 9.698598906462487790 ) ) ;
#3778=CARTESIAN_POINT ( 'NONE',  ( -100.7734535825088500, -40.00000000000027711, 22.67402823373149801 ) ) ;
#3779=CARTESIAN_POINT ( 'NONE',  ( -100.7734535825088500, 16.03295912088691821, 16.03295912088721309 ) ) ;
#3780=CARTESIAN_POINT ( 'NONE',  ( 57.59792236341148453, -37.56421063658185489, 40.00000000000002132 ) ) ;
#3783=CARTESIAN_POINT ( 'NONE',  ( -280.0000000000000000, 14.14213562373098299, -14.14213562373088706 ) ) ;
#3784=CARTESIAN_POINT ( 'NONE',  ( 170.2234770963711128, -15.44714144992812699, -40.00000000000002132 ) ) ;
#3785=CARTESIAN_POINT ( 'NONE',  ( -105.2136831797469654, 16.29138911077802021, 14.02836134671350266 ) ) ;
#3786=CARTESIAN_POINT ( 'NONE',  ( 199.9999999999999432, -1.727494763561684666E-13, 20.00000000000010303 ) ) ;
#3787=CARTESIAN_POINT ( 'NONE',  ( -105.3755690713226585, 12.89780903124410472, -43.67073346367977393 ) ) ;
#3788=CARTESIAN_POINT ( 'NONE',  ( -238.4067589809705794, 0.9644942799825385604, -40.00000000000002132 ) ) ;
#3790=ORIENTED_EDGE ( 'NONE', *, *, #7999, .T. ) ;
#3791=CARTESIAN_POINT ( 'NONE',  ( 22.82148508083520966, -43.16138278736967493, 17.87803012130510183 ) ) ;
#3793=SPHERICAL_SURFACE ( 'NONE', #11934, 15.00000000000000000 ) ;
#3794=CARTESIAN_POINT ( 'NONE',  ( -238.4067589809705794, 57.25054294077225592, 0.6820004458485544596 ) ) ;
#3795=CARTESIAN_POINT ( 'NONE',  ( -198.0356074513804572, -40.00000000000025580, 55.37879056871310013 ) ) ;
#3796=CARTESIAN_POINT ( 'NONE',  ( -56.48582580120559271, -6.472252184284276844, 6.472252184284108978 ) ) ;
#3798=CARTESIAN_POINT ( 'NONE',  ( 146.6084372240433709, 5.374981219217002781, -40.00000000000002132 ) ) ;
#3799=EDGE_CURVE ( 'NONE', #8569, #2955, #7293, .T. ) ;
#3804=CARTESIAN_POINT ( 'NONE',  ( -30.26275506840323715, 29.48230279907829754, -29.48230279907758344 ) ) ;
#3805=CARTESIAN_POINT ( 'NONE',  ( 192.4448373802100889, -14.14213562370293431, -14.14213562370322030 ) ) ;
#3806=CARTESIAN_POINT ( 'NONE',  ( -105.2468259004641595, 21.22367899003718961, -3.281783220163879911 ) ) ;
#3807=CARTESIAN_POINT ( 'NONE',  ( -77.58512834295702021, 17.50146741020782315, -13.57440574225726770 ) ) ;
#3808=CARTESIAN_POINT ( 'NONE',  ( 91.82158438592156813, -16.11829626348459144, 40.45024623143943643 ) ) ;
#3809=CARTESIAN_POINT ( 'NONE',  ( 163.1118516004056573, -9.006482792069506971, -9.006482792069697041 ) ) ;
#3810=CARTESIAN_POINT ( 'NONE',  ( -4.039451493210489019, 13.82811171175440812, 46.99046209229809534 ) ) ;
#3811=CARTESIAN_POINT ( 'NONE',  ( -208.1127848780264742, -17.67593391476605547, -38.89260858015755673 ) ) ;
#3817=CARTESIAN_POINT ( 'NONE',  ( -213.1075012329537230, -40.00000000000025580, 53.71589010953650956 ) ) ;
#3818=CARTESIAN_POINT ( 'NONE',  ( -238.4067589809705794, -0.6820004457913680929, 0.6820004457913170226 ) ) ;
#3819=CARTESIAN_POINT ( 'NONE',  ( 130.8568914410475372, 24.07718906447210472, 24.07718906447249907 ) ) ;
#3820=CARTESIAN_POINT ( 'NONE',  ( 19.06497207195980792, 54.19242893257844429, 40.00000000000002132 ) ) ;
#3821=ORIENTED_EDGE ( 'NONE', *, *, #7653, .T. ) ;
#3822=CARTESIAN_POINT ( 'NONE',  ( 163.1118516004056573, -19.27778845538761132, -19.27778845538770724 ) ) ;
#3823=B_SPLINE_CURVE_WITH_KNOTS ( 'NONE', 3,
 ( #22877, #4654, #25655, #11276, #1181, #9154, #23144, #5047 ),
 .UNSPECIFIED., .F., .F.,
 ( 4, 2, 2, 4 ),
 ( 0.008471746898050105251, 0.01057975003289800958, 0.01268775316774591218, 0.01690375943744171564 ),
 .UNSPECIFIED. ) ;
#3825=CARTESIAN_POINT ( 'NONE',  ( 83.01683444506757326, 9.947410331246418380, 24.01517293248988594 ) ) ;
#3827=CARTESIAN_POINT ( 'NONE',  ( -197.6434631108370752, -44.74794079766468258, 18.53520396667546066 ) ) ;
#3830=CARTESIAN_POINT ( 'NONE',  ( 13.28449813595630680, -24.75673736219087928, 44.77439867188066813 ) ) ;
#3831=CARTESIAN_POINT ( 'NONE',  ( 17.49521241101495406, 18.35049639060493121, -44.30201726252816741 ) ) ;
#3833=CARTESIAN_POINT ( 'NONE',  ( 147.2817042152899205, -29.82799917201331752, 12.35516179550115545 ) ) ;
#3834=DIRECTION ( 'NONE',  ( 0.000000000000000000, 1.000000000000000000, 0.000000000000000000 ) ) ;
#3835=CARTESIAN_POINT ( 'NONE',  ( 170.2234770963711128, 39.20704971665372796, 17.36149277827039583 ) ) ;
#3836=CARTESIAN_POINT ( 'NONE',  ( 91.82158438592159655, -22.79471317813468545, -2.449293598294708485E-15 ) ) ;
#3838=CARTESIAN_POINT ( 'NONE',  ( 200.0000000000000000, 3.673940397442060756E-14, 0.000000000000000000 ) ) ;
#3839=CARTESIAN_POINT ( 'NONE',  ( 98.29820294268675696, -5.307337294603860833, -19.44947291833535274 ) ) ;
#3840=CARTESIAN_POINT ( 'NONE',  ( 4.995406935893293543, -15.24977328854832592, 0.000000000000000000 ) ) ;
#3841=CARTESIAN_POINT ( 'NONE',  ( -213.1075012329537230, 13.71589010951907994, 0.000000000000000000 ) ) ;
#3842=CARTESIAN_POINT ( 'NONE',  ( 192.4448373802101173, 40.00000000000026290, -19.99999999996018474 ) ) ;
#3843=CARTESIAN_POINT ( 'NONE',  ( 163.1118516004056573, 9.006482792069629539, 9.006482792069634868 ) ) ;
#3844=CARTESIAN_POINT ( 'NONE',  ( -259.2033419157646676, -1.473088368616265084E-13, 9.517827891722632216 ) ) ;
#3845=CARTESIAN_POINT ( 'NONE',  ( -100.7734535825088500, 16.03295912088691821, 16.03295912088721309 ) ) ;
#3846=ORIENTED_EDGE ( 'NONE', *, *, #26147, .F. ) ;
#3847=CARTESIAN_POINT ( 'NONE',  ( -86.86493150571116928, 19.77569912839177846, -7.943527260495974573 ) ) ;
#3850=CARTESIAN_POINT ( 'NONE',  ( -189.2428547182110776, 47.31876910929169355, -13.87687415872436070 ) ) ;
#3853=ORIENTED_EDGE ( 'NONE', *, *, #3071, .T. ) ;
#3854=CARTESIAN_POINT ( 'NONE',  ( 200.0000000000000000, -14.14213562373062949, -42.42640687119301646 ) ) ;
#3855=CARTESIAN_POINT ( 'NONE',  ( 22.72611120194082446, -43.18769924474469946, -17.88893075486395645 ) ) ;
#3857=CARTESIAN_POINT ( 'NONE',  ( -100.7734535825088500, 17.32597176626809699, -40.00000000000002132 ) ) ;
#3858=CARTESIAN_POINT ( 'NONE',  ( -89.91498783728933120, -20.43892340021436738, 8.087768383194113397 ) ) ;
#3861=CARTESIAN_POINT ( 'NONE',  ( -83.21262154144251610, -13.72187187061454949, -33.12752917118435647 ) ) ;
#3863=CARTESIAN_POINT ( 'NONE',  ( -280.0000000000000568, 14.14213562373097943, -42.42640687119285303 ) ) ;
#3864=CARTESIAN_POINT ( 'NONE',  ( -183.1091233172472812, -41.47045062399658377, -22.43565125812520122 ) ) ;
#3865=CARTESIAN_POINT ( 'NONE',  ( 146.6084372240433709, -39.99999999999987921, -34.62501878078319351 ) ) ;
#3867=CARTESIAN_POINT ( 'NONE',  ( -100.7734535825088500, 17.32597176626808988, 40.00000000000002132 ) ) ;
#3871=CARTESIAN_POINT ( 'NONE',  ( 146.6084372240433709, -39.99999999999987921, -34.62501878078319351 ) ) ;
#3872=CARTESIAN_POINT ( 'NONE',  ( 136.1360204305621551, -39.99999999999994316, -4.966164525587488221 ) ) ;
#3873=CARTESIAN_POINT ( 'NONE',  ( -110.0563856373150315, -9.155970533462395977, 17.99047586674176458 ) ) ;
#3874=CARTESIAN_POINT ( 'NONE',  ( -105.3755690713226727, -12.89780903124413847, 12.89780903124398037 ) ) ;
#3875=CARTESIAN_POINT ( 'NONE',  ( 4.995406935893293543, -15.24977328854832592, 0.000000000000000000 ) ) ;
#3877=CARTESIAN_POINT ( 'NONE',  ( -30.26275506840322294, -57.76657404653985139, 1.198031551615709844 ) ) ;
#3881=CARTESIAN_POINT ( 'NONE',  ( -198.0356074513804572, 1.247057299367198800E-13, -15.37879056873070560 ) ) ;
#3882=CARTESIAN_POINT ( 'NONE',  ( -208.1127848780264742, -40.00000000000011369, 15.00245453012655439 ) ) ;
#3883=CARTESIAN_POINT ( 'NONE',  ( -105.3755690713226585, 12.89780903124410472, -43.67073346367977393 ) ) ;
#3884=CARTESIAN_POINT ( 'NONE',  ( 192.4448373802100889, 14.14213562375873678, 14.14213562375894817 ) ) ;
#3885=CARTESIAN_POINT ( 'NONE',  ( -188.6013942376020793, -23.51434495930271851, -43.09289976588667770 ) ) ;
#3887=CARTESIAN_POINT ( 'NONE',  ( -198.0356074513804572, -10.87444709759729911, 10.87444709759714812 ) ) ;
#3889=CARTESIAN_POINT ( 'NONE',  ( -135.8532207217289738, -6.472252184284280396, 6.472252184284099208 ) ) ;
#3891=CARTESIAN_POINT ( 'NONE',  ( 163.1118516004056573, 47.56205970284957374, 9.006482792074494981 ) ) ;
#3894=CARTESIAN_POINT ( 'NONE',  ( 163.1118516004056573, -19.27778845539181063, -37.29075403953176959 ) ) ;
#3895=B_SPLINE_CURVE_WITH_KNOTS ( 'NONE', 3,
 ( #8163, #26143, #20544, #12286, #18540, #18136, #8423, #8024, #24673, #20414 ),
 .UNSPECIFIED., .F., .F.,
 ( 4, 2, 2, 2, 4 ),
 ( 0.7921542097164072649, 0.8508620842112317728, 0.8814014469398914198, 0.9119408096685510667, 0.9406682828396428775 ),
 .UNSPECIFIED. ) ;
#3896=CARTESIAN_POINT ( 'NONE',  ( 35.93739780878637902, -38.99308239425781863, 20.78453051019726772 ) ) ;
#3901=CARTESIAN_POINT ( 'NONE',  ( 1.925538622596562277, 24.44644315487925113, 44.35335385591492496 ) ) ;
#3905=FACE_OUTER_BOUND ( 'NONE', #15425, .T. ) ;
#3907=CARTESIAN_POINT ( 'NONE',  ( -114.7544846451821030, -2.764907549246811591, -21.97700197333382377 ) ) ;
#3908=CARTESIAN_POINT ( 'NONE',  ( -109.0492076899303555, -25.45044590702468668, -25.45044590702569565 ) ) ;
#3910=CARTESIAN_POINT ( 'NONE',  ( 14.38125909742181108, 1.616281842095393922E-13, -15.17850393972633682 ) ) ;
#3912=CARTESIAN_POINT ( 'NONE',  ( -77.58456329405633767, -21.97699521662486077, -2.764787398945805386 ) ) ;
#3916=CARTESIAN_POINT ( 'NONE',  ( -142.4595961066947041, 29.46485439465666900, 12.20474230359199908 ) ) ;
#3917=CARTESIAN_POINT ( 'NONE',  ( -3.675706741948236100, -17.91131112508005074, -43.24173023805411731 ) ) ;
#3918=CARTESIAN_POINT ( 'NONE',  ( 200.0000000000000000, 14.14213562373142352, -42.42640687119268961 ) ) ;
#3919=CARTESIAN_POINT ( 'NONE',  ( -110.0574659385135305, 6.253952508993774195, -19.22572883246642306 ) ) ;
#3920=CARTESIAN_POINT ( 'NONE',  ( -105.3755690713226727, -12.89780903124413847, 12.89780903124398037 ) ) ;
#3921=CARTESIAN_POINT ( 'NONE',  ( 4.995406935893290878, 1.606505379428369110E-13, -15.24977328854832592 ) ) ;
#3922=CARTESIAN_POINT ( 'NONE',  ( 199.9999999999999432, 20.00000000000013856, 0.000000000000000000 ) ) ;
#3924=CARTESIAN_POINT ( 'NONE',  ( 170.2234770963711128, -15.44714144992813409, 40.00000000000002132 ) ) ;
#3926=CARTESIAN_POINT ( 'NONE',  ( 170.2234770963711128, -15.44714144992812876, -2.449293598294708485E-15 ) ) ;
#3927=CARTESIAN_POINT ( 'NONE',  ( -114.7581397844644187, 13.68781109932255546, 17.42046360869897725 ) ) ;
#3928=CARTESIAN_POINT ( 'NONE',  ( 136.1360204305621551, 40.00000000000009948, -4.966164525586641787 ) ) ;
#3929=CARTESIAN_POINT ( 'NONE',  ( 184.8905102610680444, 41.77492675556005253, -14.79361573936377461 ) ) ;
#3930=CARTESIAN_POINT ( 'NONE',  ( -135.8532207217289738, -9.153146818113595984, 0.000000000000000000 ) ) ;
#3931=VERTEX_POINT ( 'NONE', #11667 ) ;
#3932=ADVANCED_FACE ( 'NONE', ( #11290 ), #20441, .T. ) ;
#3933=CARTESIAN_POINT ( 'NONE',  ( -259.2033419157646676, -9.517827891722680178, 0.000000000000000000 ) ) ;
#3935=CARTESIAN_POINT ( 'NONE',  ( -65.65510974524491417, -9.107311025939104354, 24.89665924127723784 ) ) ;
#3936=CARTESIAN_POINT ( 'NONE',  ( 184.8905102610680444, 41.77492675556005253, -14.79361573936377461 ) ) ;
#3937=CARTESIAN_POINT ( 'NONE',  ( -280.0000000000000568, -40.00000000000014211, 19.99999999999987210 ) ) ;
#3938=CARTESIAN_POINT ( 'NONE',  ( 14.38125909742180220, 39.01709431150892016, 17.55144818341517166 ) ) ;
#3939=CARTESIAN_POINT ( 'NONE',  ( 4.995406935893288214, 15.24977328854832770, 0.000000000000000000 ) ) ;
#3943=CARTESIAN_POINT ( 'NONE',  ( -192.9588430854690273, 66.79921049724377724, -10.23066800231904239 ) ) ;
#3944=CARTESIAN_POINT ( 'NONE',  ( 170.2234770963711128, -39.20704971665404059, 17.36149277826957160 ) ) ;
#3945=CARTESIAN_POINT ( 'NONE',  ( -105.4536606934774738, 19.90286765811677228, 7.687677726850456139 ) ) ;
#3946=CARTESIAN_POINT ( 'NONE',  ( -238.4067589809705794, -3.369206980223063916E-14, -0.9644942799825824142 ) ) ;
#3947=CARTESIAN_POINT ( 'NONE',  ( -208.1127848780264742, -38.89260858015753541, 17.67593391476614784 ) ) ;
#3948=CARTESIAN_POINT ( 'NONE',  ( -105.3755690713226727, -15.38646221621807619, 15.38646221621768362 ) ) ;
#3949=CARTESIAN_POINT ( 'NONE',  ( -198.0356074513804572, -17.40982414986427429, -39.15871834505933435 ) ) ;
#3950=CARTESIAN_POINT ( 'NONE',  ( 170.2234770963711128, -10.92277846919171935, -45.64576402573189995 ) ) ;
#3953=CARTESIAN_POINT ( 'NONE',  ( 184.8905102610680444, 1.070102760522089011E-13, -20.92133201514444352 ) ) ;
#3954=CARTESIAN_POINT ( 'NONE',  ( -135.8532207217289738, 6.472252184284096543, 6.472252184284234211 ) ) ;
#3955=CARTESIAN_POINT ( 'NONE',  ( 11.38508063394172609, 44.88728980639542243, -24.83994849155190821 ) ) ;
#3956=CARTESIAN_POINT ( 'NONE',  ( 163.1118516004056573, 12.73709011382478273, 2.449293598294708485E-15 ) ) ;
#3958=CARTESIAN_POINT ( 'NONE',  ( -280.0000000000000000, -20.00000000000006750, 0.000000000000000000 ) ) ;
#3959=EDGE_CURVE ( 'NONE', #14912, #15079, #21981, .T. ) ;
#3960=CARTESIAN_POINT ( 'NONE',  ( 25.86856017011190900, 41.48891248390243902, 17.18527023894284156 ) ) ;
#3962=CARTESIAN_POINT ( 'NONE',  ( 170.2234770963711128, -24.55285855007183926, 0.000000000000000000 ) ) ;
#3965=CARTESIAN_POINT ( 'NONE',  ( -188.6889827002315769, -43.11787295909560669, 23.53286111060863561 ) ) ;
#3967=CARTESIAN_POINT ( 'NONE',  ( -0.6848998193154250957, -13.98809697771007343, 48.06291537634446343 ) ) ;
#3970=CARTESIAN_POINT ( 'NONE',  ( 25.88393124175084026, 13.61573025394702974, -45.90075965688677684 ) ) ;
#3973=CARTESIAN_POINT ( 'NONE',  ( -151.7004448981651024, -13.46262099556660097, 32.50164219284836520 ) ) ;
#3974=CARTESIAN_POINT ( 'NONE',  ( -208.1127848780265026, 38.89260858015777700, -38.89260858015687461 ) ) ;
#3975=CARTESIAN_POINT ( 'NONE',  ( 170.2234770963711128, 24.55285855007190676, 40.00000000000002132 ) ) ;
#3976=CARTESIAN_POINT ( 'NONE',  ( -192.9370379451515873, 24.26711011076366376, -44.11033005022372322 ) ) ;
#3977=CARTESIAN_POINT ( 'NONE',  ( -86.96347745069644475, -15.38646221621807442, 15.38646221621768184 ) ) ;
#3978=CARTESIAN_POINT ( 'NONE',  ( 98.29820294267474878, -15.06873823043769534, -13.21553301703162298 ) ) ;
#3979=CARTESIAN_POINT ( 'NONE',  ( 146.6084372240433993, 34.62501878078308692, 0.000000000000000000 ) ) ;
#3980=CARTESIAN_POINT ( 'NONE',  ( 14.38125909742180752, 55.17850393972636880, 2.449293598294708485E-15 ) ) ;
#3981=CARTESIAN_POINT ( 'NONE',  ( -91.56559293963834989, -39.99999999999985789, -17.32597176626853042 ) ) ;
#3982=CARTESIAN_POINT ( 'NONE',  ( -208.1127848780265026, 38.89260858015724409, 38.89260858015741462 ) ) ;
#3984=CARTESIAN_POINT ( 'NONE',  ( -259.2033419157646676, 35.01439189186559275, -21.55415060305807984 ) ) ;
#3986=CARTESIAN_POINT ( 'NONE',  ( 163.1118516004056573, -47.56205970284957374, 9.006482792074162802 ) ) ;
#3991=CARTESIAN_POINT ( 'NONE',  ( 170.2234770963711128, -39.20704971665379190, -17.36149277827012938 ) ) ;
#3992=CARTESIAN_POINT ( 'NONE',  ( 36.88256715603331060, -39.10885149551745599, -16.19941669847073840 ) ) ;
#3993=ORIENTED_EDGE ( 'NONE', *, *, #4040, .F. ) ;
#3994=CARTESIAN_POINT ( 'NONE',  ( 200.0000000000000000, -20.00000000000006750, -40.00000000000002132 ) ) ;
#3995=CARTESIAN_POINT ( 'NONE',  ( -88.37877758188346888, -20.15391234948233290, 8.026456973548603102 ) ) ;
#3998=DIRECTION ( 'NONE',  ( 0.9352143323240051931, 0.3271292299060145070, 0.1355013636716006220 ) ) ;
#3999=CARTESIAN_POINT ( 'NONE',  ( -135.8532207217289738, 21.81201906317777883, -34.75652343174605363 ) ) ;
#4000=CARTESIAN_POINT ( 'NONE',  ( -188.3392995398611163, -47.00482667599626296, -13.83024151208815233 ) ) ;
#4001=CARTESIAN_POINT ( 'NONE',  ( -162.0762913951021176, -40.00000000000019895, 41.69427287672974813 ) ) ;
#4002=CARTESIAN_POINT ( 'NONE',  ( -198.0356074513804572, 15.37879056873066830, 40.00000000000002132 ) ) ;
#4005=CARTESIAN_POINT ( 'NONE',  ( 136.1360204305621551, -39.99999999999987921, -35.03383547441310242 ) ) ;
#4006=CARTESIAN_POINT ( 'NONE',  ( -238.4067589809705794, -1.892706720741712928E-13, 40.96449427998260973 ) ) ;
#4007=CARTESIAN_POINT ( 'NONE',  ( 130.8568914410475088, -40.00000000000036238, 34.05028731879746573 ) ) ;
#4008=CARTESIAN_POINT ( 'NONE',  ( 130.8568914410475088, 40.00000000000002842, 5.949712681206834830 ) ) ;
#4010=CARTESIAN_POINT ( 'NONE',  ( -86.96347745069643054, -41.18208027870589660, -15.38646221621809040 ) ) ;
#4011=CARTESIAN_POINT ( 'NONE',  ( -280.0000000000000568, 19.99999999999996092, -40.00000000000002132 ) ) ;
#4012=CARTESIAN_POINT ( 'NONE',  ( -192.9588430854690273, -66.79921049724377724, 10.23066800231950069 ) ) ;
#4013=CARTESIAN_POINT ( 'NONE',  ( -99.29480781227071873, -8.934325994365618584, 20.48155342677138790 ) ) ;
#4015=CARTESIAN_POINT ( 'NONE',  ( -208.1127848780265026, 1.189126717069624012E-13, -15.00245453012669472 ) ) ;
#4016=CARTESIAN_POINT ( 'NONE',  ( 4.995406935893305089, -40.00000000000021316, 55.24977328853194791 ) ) ;
#4017=CARTESIAN_POINT ( 'NONE',  ( -213.1075012329537230, 66.26714140136188291, 9.698598906438215650 ) ) ;
#4018=CARTESIAN_POINT ( 'NONE',  ( -114.5325442475739663, 19.70118921568331416, 9.696479999167626929 ) ) ;
#4019=CARTESIAN_POINT ( 'NONE',  ( -192.6563370915134783, -18.27409561805844618, -44.11756948122080502 ) ) ;
#4022=CARTESIAN_POINT ( 'NONE',  ( -86.96347745069644475, -15.38646221621807442, 15.38646221621768184 ) ) ;
#4024=CARTESIAN_POINT ( 'NONE',  ( 192.4448373802100889, 20.00000000003945644, 0.000000000000000000 ) ) ;
#4025=( BOUNDED_SURFACE ( )  B_SPLINE_SURFACE ( 3, 2, ( 
 ( #12270, #3762, #22262 ),
 ( #6026, #17980, #24387 ),
 ( #18518, #12138, #20396 ),
 ( #24653, #20523, #3907 ),
 ( #24252, #2170, #18118 ),
 ( #8403, #12005, #4039 ) ),
 .UNSPECIFIED., .F., .F., .F. ) 
 B_SPLINE_SURFACE_WITH_KNOTS ( ( 4, 2, 4 ),
 ( 3, 3 ),
 ( 0.04143191525983294654, 0.04845780415094015636, 0.05548369304204737312 ),
 ( 0.000000000000000000, 1.000000000000000000 ),
 .UNSPECIFIED. ) 
 GEOMETRIC_REPRESENTATION_ITEM ( )  RATIONAL_B_SPLINE_SURFACE ( (
 ( 1.000000000000000000, 0.9541700777564462443, 1.000000000000000000),
 ( 1.000000000000000000, 0.9520117619553596366, 1.000000000000000000),
 ( 1.000000000000000000, 0.9503155880217531992, 1.000000000000000000),
 ( 1.000000000000000000, 0.9480088211921217090, 1.000000000000000000),
 ( 1.000000000000000000, 0.9474362549813150070, 1.000000000000000000),
 ( 1.000000000000000000, 0.9474350312570024579, 1.000000000000000000) ) ) 
 REPRESENTATION_ITEM ( '' )  SURFACE ( )  );
#4027=CARTESIAN_POINT ( 'NONE',  ( 4.995406935893297984, 10.78321810390233892, -67.35176059882522281 ) ) ;
#4029=CARTESIAN_POINT ( 'NONE',  ( -86.95450735007487708, 6.704150134086016344, 20.33657406937396672 ) ) ;
#4033=CARTESIAN_POINT ( 'NONE',  ( -17.28139728210405579, 12.88180358344996179, 42.38047544431644553 ) ) ;
#4035=VERTEX_POINT ( 'NONE', #19900 ) ;
#4037=CARTESIAN_POINT ( 'NONE',  ( -30.26275506840324070, 1.694272468446254232, 0.000000000000000000 ) ) ;
#4039=CARTESIAN_POINT ( 'NONE',  ( -114.7826396787322665, 2.131776515495824860E-13, -22.13135001986800532 ) ) ;
#4040=EDGE_CURVE ( 'NONE', #1902, #24441, #21639, .T. ) ;
#4041=CARTESIAN_POINT ( 'NONE',  ( -105.4741150117391157, -7.943527260750152585, -19.77569912955105025 ) ) ;
#4042=CARTESIAN_POINT ( 'NONE',  ( 170.2234770963711128, -2.259079968736224833E-13, 24.55285855007187124 ) ) ;
#4044=CARTESIAN_POINT ( 'NONE',  ( -82.23726319257784212, -20.19517362734544008, -1.261455835848799056 ) ) ;
#4045=DIRECTION ( 'NONE',  ( 0.2259624731720088209, 0.000000000000000000, -0.9741360072997964359 ) ) ;
#4047=DIRECTION ( 'NONE',  ( 0.9698969544100567441, 0.2249791742613287404, 0.09318942523048100168 ) ) ;
#4048=CARTESIAN_POINT ( 'NONE',  ( 3.468680970036517319, -24.60338114561098166, -44.56630890487775787 ) ) ;
#4049=CARTESIAN_POINT ( 'NONE',  ( -30.26275506840322649, -29.48230279907769358, -29.48230279907820162 ) ) ;
#4050=CARTESIAN_POINT ( 'NONE',  ( -114.5516905196692932, 6.814306831805573950, -20.88874846747904357 ) ) ;
#4051=CARTESIAN_POINT ( 'NONE',  ( -259.2033419157646676, -21.55415060305854524, 21.55415060305827524 ) ) ;
#4053=CARTESIAN_POINT ( 'NONE',  ( -30.26275506840324070, -1.198031551616016266, -1.198031551616031587 ) ) ;
#4054=CARTESIAN_POINT ( 'NONE',  ( -100.7734535825088500, -17.32597176626813251, 40.00000000000002132 ) ) ;
#4056=CARTESIAN_POINT ( 'NONE',  ( 184.8905102610680444, -19.07866798485555293, -2.449293598294708485E-15 ) ) ;
#4057=CARTESIAN_POINT ( 'NONE',  ( -105.2926326438279006, 11.51852324731283161, 18.07795834784788624 ) ) ;
#4058=CARTESIAN_POINT ( 'NONE',  ( 130.8568914410475088, 40.00000000000011369, -5.949712681206269949 ) ) ;
#4059=CARTESIAN_POINT ( 'NONE',  ( 163.1118516004056573, 9.006482792074356425, -47.56205970284957374 ) ) ;
#4060=CARTESIAN_POINT ( 'NONE',  ( 130.8568914410475372, -34.05028731879786363, 0.000000000000000000 ) ) ;
#4061=ORIENTED_EDGE ( 'NONE', *, *, #25592, .T. ) ;
#4062=ORIENTED_EDGE ( 'NONE', *, *, #16483, .T. ) ;
#4063=CARTESIAN_POINT ( 'NONE',  ( 151.7948205124836534, -33.23291073765550863, 40.00000000000002132 ) ) ;
#4066=AXIS2_PLACEMENT_3D ( 'NONE', #15847, #12007, #4432 ) ;
#4067=CARTESIAN_POINT ( 'NONE',  ( -213.1075012329537230, -40.00000000000025580, 53.71589010953650956 ) ) ;
#4069=CARTESIAN_POINT ( 'NONE',  ( -135.8532207217289738, 50.09629031063956006, 6.472252184284782217 ) ) ;
#4070=DIRECTION ( 'NONE',  ( -0.01051738777841060291, -0.9307051272558614086, -0.3656191333258823617 ) ) ;
#4075=CARTESIAN_POINT ( 'NONE',  ( 184.8905102610680444, 13.49065550809826952, -13.49065550809790359 ) ) ;
#4076=AXIS2_PLACEMENT_3D ( 'NONE', #23567, #13452, #5342 ) ;
#4077=CARTESIAN_POINT ( 'NONE',  ( -280.0000000000000568, -14.14213562373137556, 42.42640687119276066 ) ) ;
#4079=CARTESIAN_POINT ( 'NONE',  ( -56.48582580120559271, -1.062504017861011783E-13, 9.153146818113587102 ) ) ;
#4080=CARTESIAN_POINT ( 'NONE',  ( 130.8568914410475372, -4.207082182992785135, -4.207082182992884611 ) ) ;
#4081=CARTESIAN_POINT ( 'NONE',  ( 91.82158438592158234, -12.16597498397778843, 12.16597498397750954 ) ) ;
#4082=CARTESIAN_POINT ( 'NONE',  ( -91.56559293963834989, -16.03295912088706388, -16.03295912088710651 ) ) ;
#4083=CARTESIAN_POINT ( 'NONE',  ( 136.1360204305621266, 24.77266263493138965, -24.77266263493110188 ) ) ;
#4086=CARTESIAN_POINT ( 'NONE',  ( 130.8568914410475088, 40.00000000000002842, 5.949712681206834830 ) ) ;
#4087=VECTOR ( 'NONE', #5755, 1000.000000000000114 ) ;
#4090=CARTESIAN_POINT ( 'NONE',  ( 23.37583784646129104, 46.80752016581939046, -13.80085822091003500 ) ) ;
#4091=CARTESIAN_POINT ( 'NONE',  ( 19.06497207195980792, 54.19242893257843718, 2.449293598294708485E-15 ) ) ;
#4094=CARTESIAN_POINT ( 'NONE',  ( -16.78454218905211093, -39.63790004368954811, 16.41855578202928356 ) ) ;
#4095=CARTESIAN_POINT ( 'NONE',  ( -86.96347745069644475, -21.75974354311651737, 0.000000000000000000 ) ) ;
#4097=CARTESIAN_POINT ( 'NONE',  ( -3.069599232962576085, 23.65302469262847751, -43.28003856805327842 ) ) ;
#4099=CARTESIAN_POINT ( 'NONE',  ( -2.164901439689549179, -13.92557459411189313, 47.64638340556978591 ) ) ;
#4100=CARTESIAN_POINT ( 'NONE',  ( 22.70429368897870859, 17.89136451867761579, -43.19357487035025400 ) ) ;
#4102=VECTOR ( 'NONE', #24243, 1000.000000000000000 ) ;
#4103=CARTESIAN_POINT ( 'NONE',  ( 23.37394308801977871, -46.80823611210205115, 13.80096434448272724 ) ) ;
#4104=CARTESIAN_POINT ( 'NONE',  ( 151.0853911467767432, -29.06993079631231325, 12.04115959307964090 ) ) ;
#4105=CARTESIAN_POINT ( 'NONE',  ( 163.1118516004056573, 1.251511021549353291E-13, -27.26290988616872824 ) ) ;
#4107=CARTESIAN_POINT ( 'NONE',  ( -192.9588430854689989, 38.51493924976983152, -38.51493924976893624 ) ) ;
#4108=CARTESIAN_POINT ( 'NONE',  ( -99.21568817060988010, -22.67402823373193499, 0.000000000000000000 ) ) ;
#4109=CARTESIAN_POINT ( 'NONE',  ( -188.8532066752251808, 17.93248812771325262, -43.29285604501834683 ) ) ;
#4110=CARTESIAN_POINT ( 'NONE',  ( -105.3755690713226585, 12.89780903124349720, 43.67073346367994446 ) ) ;
#4111=CARTESIAN_POINT ( 'NONE',  ( 199.9999999999999432, 20.00000000000013856, 0.000000000000000000 ) ) ;
#4112=CARTESIAN_POINT ( 'NONE',  ( 170.2234770963711128, -15.44714144992812699, -40.00000000000002132 ) ) ;
#4113=CARTESIAN_POINT ( 'NONE',  ( -213.1075012329537230, 53.71589010951910836, 2.449293598294708485E-15 ) ) ;
#4115=CARTESIAN_POINT ( 'NONE',  ( 151.7948205124836250, 1.012150473917908975E-13, -6.767089262349031742 ) ) ;
#4116=CARTESIAN_POINT ( 'NONE',  ( -56.48582580120559982, 50.09629031063966664, -6.472252184284094767 ) ) ;
#4118=CARTESIAN_POINT ( 'NONE',  ( -105.4732637872223080, 19.68494377761377123, -8.153770687239582315 ) ) ;
#4119=CARTESIAN_POINT ( 'NONE',  ( -86.96347745069645896, 43.67073346367988762, -12.89780903124366418 ) ) ;
#4121=ADVANCED_FACE ( 'NONE', ( #3539 ), #10569, .T. ) ;
#4123=CARTESIAN_POINT ( 'NONE',  ( -91.56559293963834989, -44.31723036834903695, 12.25131212657476709 ) ) ;
#4124=CARTESIAN_POINT ( 'NONE',  ( -77.55640685876518603, 15.64922766773203122, 15.64922766773211471 ) ) ;
#4126=ORIENTED_EDGE ( 'NONE', *, *, #14927, .T. ) ;
#4128=CARTESIAN_POINT ( 'NONE',  ( -198.0356074513804572, -39.15871834505905724, -17.40982414986491733 ) ) ;
#4129=CARTESIAN_POINT ( 'NONE',  ( 45.01779936579357866, -38.89115870262487107, -12.15764947739186930 ) ) ;
#4131=CARTESIAN_POINT ( 'NONE',  ( -135.8532207217289738, -9.153146818113595984, 0.000000000000000000 ) ) ;
#4132=B_SPLINE_CURVE_WITH_KNOTS ( 'NONE', 3,
 ( #4408, #25162, #8917, #18629, #2811, #412 ),
 .UNSPECIFIED., .F., .F.,
 ( 4, 2, 4 ),
 ( -5.999999999678665604E-08, 0.03937727993095216372, 0.07875461986190432362 ),
 .UNSPECIFIED. ) ;
#4133=CARTESIAN_POINT ( 'NONE',  ( -93.01741312767373415, -20.82169463879412419, 8.169811846252175158 ) ) ;
#4136=( BOUNDED_SURFACE ( )  B_SPLINE_SURFACE ( 3, 2, ( 
 ( #23644, #3046, #21272 ),
 ( #11153, #25402, #5422 ),
 ( #21524, #19268, #21400 ),
 ( #17267, #7401, #21147 ),
 ( #19398, #9283, #6896 ),
 ( #13525, #3173, #23272 ),
 ( #2790, #15395, #1050 ),
 ( #5292, #4915, #23520 ),
 ( #19015, #10903, #23398 ),
 ( #13027, #1302, #5174 ),
 ( #7279, #7021, #25273 ),
 ( #13278, #17391, #17138 ),
 ( #9034, #25530, #2921 ),
 ( #11029, #13399, #19139 ),
 ( #3300, #923, #11394 ),
 ( #9411, #17517, #19777 ),
 ( #25917, #7533, #17910 ),
 ( #13655, #16182, #19648 ),
 ( #21649, #5814, #21779 ),
 ( #11795, #7660, #19914 ),
 ( #17640, #9934, #18040 ),
 ( #26194, #6083, #10070 ),
 ( #12064, #3552, #3965 ),
 ( #25783, #7790, #16048 ),
 ( #20181, #15641, #22190 ),
 ( #5948, #24318, #3687 ),
 ( #22054, #13919, #1965 ),
 ( #18175, #8065, #1698 ),
 ( #23769, #24173, #15772 ),
 ( #5547, #14056, #26323 ),
 ( #11653, #3421, #9803 ),
 ( #26053, #3827, #11523 ),
 ( #11929, #20054, #15906 ),
 ( #1565, #1433, #1833 ) ),
 .UNSPECIFIED., .F., .F., .F. ) 
 B_SPLINE_SURFACE_WITH_KNOTS ( ( 4, 2, 2, 2, 2, 2, 2, 2, 2, 2, 2, 2, 2, 2, 2, 2, 4 ),
 ( 3, 3 ),
 ( 0.005135432767689945138, 0.02907015807668583696, 0.05300488338568172531, 0.07693960869467761365, 0.08292329002192658227, 0.08441921035373882443, 0.08446595786410796003, 0.08448933161929252089, 0.08451270537447708175, 0.08460620039521535296, 0.08479319043669189537, 0.08516717051964495244, 0.08591513068555106658, 0.08890697134917555089, 0.09189881201280003520, 0.09489065267642451951, 0.1008743340036735020 ),
 ( 0.000000000000000000, 1.000000000000000000 ),
 .UNSPECIFIED. ) 
 GEOMETRIC_REPRESENTATION_ITEM ( )  RATIONAL_B_SPLINE_SURFACE ( (
 ( 1.000000000000000000, 0.9997813423552077694, 1.000000000000000000),
 ( 1.000000000000000000, 0.9991063898506412633, 1.000000000000000000),
 ( 1.000000000000000000, 0.9968824705949630438, 1.000000000000000000),
 ( 1.000000000000000000, 0.9891556793369802314, 1.000000000000000000),
 ( 1.000000000000000000, 0.9836552277517739418, 1.000000000000000000),
 ( 1.000000000000000000, 0.9690805015308342485, 1.000000000000000000),
 ( 1.000000000000000000, 0.9600094330338765358, 1.000000000000000000),
 ( 1.000000000000000000, 0.9461485276688212931, 1.000000000000000000),
 ( 1.000000000000000000, 0.9432497373317600964, 1.000000000000000000),
 ( 1.000000000000000000, 0.9394620364518223576, 1.000000000000000000),
 ( 1.000000000000000000, 0.9386962831138082608, 1.000000000000000000),
 ( 1.000000000000000000, 0.9378980481303071937, 1.000000000000000000),
 ( 1.000000000000000000, 0.9378738510928912309, 1.000000000000000000),
 ( 1.000000000000000000, 0.9378375433852945697, 1.000000000000000000),
 ( 1.000000000000000000, 0.9378253334781214701, 1.000000000000000000),
 ( 1.000000000000000000, 0.9378014123365954191, 1.000000000000000000),
 ( 1.000000000000000000, 0.9377894572438932874, 1.000000000000000000),
 ( 1.000000000000000000, 0.9377297092068097584, 1.000000000000000000),
 ( 1.000000000000000000, 0.9376819985415333347, 1.000000000000000000),
 ( 1.000000000000000000, 0.9375391312191839743, 1.000000000000000000),
 ( 1.000000000000000000, 0.9374442392362084542, 1.000000000000000000),
 ( 1.000000000000000000, 0.9371606329891914999, 1.000000000000000000),
 ( 1.000000000000000000, 0.9369729884417196120, 1.000000000000000000),
 ( 1.000000000000000000, 0.9364144211479191737, 1.000000000000000000),
 ( 1.000000000000000000, 0.9360478649890143776, 1.000000000000000000),
 ( 1.000000000000000000, 0.9342453465010664981, 1.000000000000000000),
 ( 1.000000000000000000, 0.9329002455189063792, 1.000000000000000000),
 ( 1.000000000000000000, 0.9304321598240474778, 1.000000000000000000),
 ( 1.000000000000000000, 0.9293115443288696431, 1.000000000000000000),
 ( 1.000000000000000000, 0.9273348408774876317, 1.000000000000000000),
 ( 1.000000000000000000, 0.9264755133097204443, 1.000000000000000000),
 ( 1.000000000000000000, 0.9243017816400511677, 1.000000000000000000),
 ( 1.000000000000000000, 0.9233922826849433330, 1.000000000000000000),
 ( 1.000000000000000000, 0.9230541040371987860, 1.000000000000000000) ) ) 
 REPRESENTATION_ITEM ( '' )  SURFACE ( )  );
#4138=CARTESIAN_POINT ( 'NONE',  ( -259.2033419157646676, -6.730120644403570829, -6.730120644403545960 ) ) ;
#4139=CARTESIAN_POINT ( 'NONE',  ( -188.9266751785330314, -43.31221945728822220, -17.94050871568865091 ) ) ;
#4141=CARTESIAN_POINT ( 'NONE',  ( 151.7948205124836534, -39.99999999999987921, -33.23291073765567916 ) ) ;
#4142=CARTESIAN_POINT ( 'NONE',  ( 136.1360204305621266, -35.03383547441293899, 0.000000000000000000 ) ) ;
#4145=CARTESIAN_POINT ( 'NONE',  ( -56.48582580120558561, -40.00000000000000000, -9.153146818113723882 ) ) ;
#4146=CARTESIAN_POINT ( 'NONE',  ( 19.06497207195981858, -1.881589693694111225E-13, 54.19242893257843008 ) ) ;
#4147=CARTESIAN_POINT ( 'NONE',  ( -135.8532207217289738, 7.002209520526292428E-15, -9.153146818113572891 ) ) ;
#4148=CARTESIAN_POINT ( 'NONE',  ( -192.9588430854689989, -14.46834944099973086, 0.000000000000000000 ) ) ;
#4149=CARTESIAN_POINT ( 'NONE',  ( -86.96347745069644475, -12.89780903124413491, 12.89780903124398037 ) ) ;
#4150=CARTESIAN_POINT ( 'NONE',  ( -100.7734535825088500, 22.67402823373189946, -40.00000000000002132 ) ) ;
#4151=CARTESIAN_POINT ( 'NONE',  ( 151.7948205124836534, 23.49921654116009506, 33.06932595376371609 ) ) ;
#4154=CARTESIAN_POINT ( 'NONE',  ( -100.7734535825088500, 39.99999999999976552, 22.67402823373233645 ) ) ;
#4155=CARTESIAN_POINT ( 'NONE',  ( -198.0356074513804572, 39.99999999999979394, 55.37879056874835726 ) ) ;
#4156=CARTESIAN_POINT ( 'NONE',  ( 136.1360204305621551, 31.79587985999267374, -24.77266263493117293 ) ) ;
#4157=CARTESIAN_POINT ( 'NONE',  ( 14.38125909742181285, -10.73282306404712472, -10.73282306404731301 ) ) ;
#4158=CARTESIAN_POINT ( 'NONE',  ( -188.4265466358326080, -23.47687925214715321, -43.04237830660283493 ) ) ;
#4160=ORIENTED_EDGE ( 'NONE', *, *, #8905, .F. ) ;
#4161=CARTESIAN_POINT ( 'NONE',  ( 151.7948205124836250, -23.49921654116371883, 23.49921654116317526 ) ) ;
#4162=B_SPLINE_CURVE_WITH_KNOTS ( 'NONE', 3,
 ( #19957, #13569, #15688, #16093, #21695, #15959, #3471, #1477, #9715, #5595, #21826, #1877, #3595, #11975 ),
 .UNSPECIFIED., .F., .F.,
 ( 4, 2, 2, 2, 2, 2, 4 ),
 ( 2.647940464546886252E-17, 0.002941681445497028834, 0.004412522168245528939, 0.005883362890994029044, 0.008825044336491017979, 0.01029588505923952069, 0.01176672578198802166 ),
 .UNSPECIFIED. ) ;
#4163=DIRECTION ( 'NONE',  ( -0.3301743741188450376, 0.000000000000000000, -0.9439199556504932476 ) ) ;
#4164=CARTESIAN_POINT ( 'NONE',  ( -198.0356074513804572, -15.37879056873074290, -40.00000000000002132 ) ) ;
#4165=CARTESIAN_POINT ( 'NONE',  ( -87.11017345524855671, 17.07168028895587852, 13.10675206033511131 ) ) ;
#4166=CARTESIAN_POINT ( 'NONE',  ( 0.2972598230769990524, -18.14793986248671231, -38.42060263243687501 ) ) ;
#4167=EDGE_LOOP ( 'NONE', ( #4648, #20084, #12084, #10262, #3453 ) ) ;
#4170=CARTESIAN_POINT ( 'NONE',  ( 1.564570055219380196, -24.39611894128483627, 44.28524390194910865 ) ) ;
#4171=CARTESIAN_POINT ( 'NONE',  ( -2.004660104981413227, 18.09067139728989559, 43.67474423981169451 ) ) ;
#4174=CARTESIAN_POINT ( 'NONE',  ( -100.7734535825088358, -22.67402823373193499, 0.000000000000000000 ) ) ;
#4176=CARTESIAN_POINT ( 'NONE',  ( -77.78698626355769363, -9.956330463956303944, -19.58753875850657167 ) ) ;
#4177=DIRECTION ( 'NONE',  ( 0.000000000000000000, -0.9166903767142837722, -0.3995982397851930989 ) ) ;
#4178=CARTESIAN_POINT ( 'NONE',  ( 3.854700064722245578, 44.60002223906914054, -24.62824689551992563 ) ) ;
#4179=CARTESIAN_POINT ( 'NONE',  ( -91.56559293963836410, 40.00000000000019185, -17.32597176626768487 ) ) ;
#4184=CARTESIAN_POINT ( 'NONE',  ( -121.8281105898911818, 8.694016233166976804, 23.07023229731760239 ) ) ;
#4185=CARTESIAN_POINT ( 'NONE',  ( -3.406542234095930155, -17.94112998239644341, -43.31371932780105283 ) ) ;
#4186=CARTESIAN_POINT ( 'NONE',  ( -100.7734535825088500, -40.53558337403692491, 16.03295912088671571 ) ) ;
#4187=( BOUNDED_SURFACE ( )  B_SPLINE_SURFACE ( 3, 3, ( 
 ( #11115, #20970, #19100, #22839, #12710, #347, #8451, #18972, #6982, #12578, #10584, #8590, #25874, #23728, #1395, #1009, #5509, #25743, #3515, #5383, #1525, #13611, #7618, #13359, #5636, #19229, #7492, #23604, #9112, #13488 ),
 ( #21609, #5257, #9247, #9496, #11360, #9632, #17223, #15477, #7365, #19477, #25619, #3256, #1263, #11235, #19353, #3383, #17601, #11481, #7116, #19609, #7238, #25362, #15733, #23859, #1142, #15227, #17353, #25489, #23358, #15603 ),
 ( #21869, #21739, #11615, #5135, #19737, #17477, #17733, #13743, #3647, #13240, #21365, #3133, #15359, #23483, #21481, #9367, #20280, #7752, #24135, #14016, #24275, #7889, #13880, #1922, #16142, #22013, #3784, #6171, #2059, #10165 ),
 ( #23992, #14150, #18268, #2191, #181, #20415, #52, #22546, #6045, #11752, #10028, #19873, #18138, #5772, #8164, #10299, #26145, #9764, #26286, #11886, #15863, #20007, #16009, #22282, #8025, #12158, #3926, #4056, #16276, #18000 ),
 ( #8288, #20144, #24405, #9896, #6298, #18406, #1792, #16415, #5907, #14281, #22145, #12024, #24543, #14416, #22418, #4194, #12287, #1655, #17865, #26015, #8831, #12827, #12417, #16940, #10830, #14945, #16809, #12956, #25075, #10967 ),
 ( #4327, #18945, #8698, #20545, #24947, #10423, #22940, #20814, #18811, #2586, #23079, #21075, #4452, #6695, #14548, #4851, #12547, #20679, #18541, #726, #6826, #19075, #24808, #2860, #856, #323, #8424, #2315, #14808, #6430 ),
 ( #4720, #591, #4587, #8563, #8965, #16544, #10559, #24674, #10701, #22678, #458, #2448, #17074, #25208, #6956, #15073, #18672, #16677, #6560, #14675, #22811, #12684, #20947, #2725, #11088, #17452, #7591, #11584, #5230, #5355 ) ),
 .UNSPECIFIED., .T., .F., .F. ) 
 B_SPLINE_SURFACE_WITH_KNOTS ( ( 4, 3, 4 ),
 ( 4, 2, 2, 2, 2, 2, 2, 2, 2, 2, 2, 2, 2, 2, 4 ),
 ( 0.000000000000000000, 0.5000000000000000000, 1.000000000000000000 ),
 ( 0.000000000000000000, 0.1357259735107005372, 0.1651108541090157700, 0.1944957347073310028, 0.3598804999793158710, 0.3867117631979620773, 0.4135430264166082281, 0.5789277916885930964, 0.6062785021374117456, 0.6336292125862302838, 0.8508620842112317728, 0.8814014469398914198, 0.9119408096685510667, 0.9559704048342755334, 1.000000000000000000 ),
 .UNSPECIFIED. ) 
 GEOMETRIC_REPRESENTATION_ITEM ( )  RATIONAL_B_SPLINE_SURFACE ( (
 ( 1.000000000000000000, 1.000000000000000000, 1.000000000000000000, 1.000000000000000000, 1.000000000000000000, 1.000000000000000000, 1.000000000000000000, 1.000000000000000000, 1.000000000000000000, 1.000000000000000000, 1.000000000000000000, 1.000000000000000000, 1.000000000000000000, 1.000000000000000000, 1.000000000000000000, 1.000000000000000000, 1.000000000000000000, 1.000000000000000000, 1.000000000000000000, 1.000000000000000000, 1.000000000000000000, 1.000000000000000000, 1.000000000000000000, 1.000000000000000000, 1.000000000000000000, 1.000000000000000000, 1.000000000000000000, 1.000000000000000000, 1.000000000000000000, 1.000000000000000000),
 ( 0.3333333333333333703, 0.3333333333333333703, 0.3333333333333333703, 0.3333333333333333703, 0.3333333333333333703, 0.3333333333333333703, 0.3333333333333333703, 0.3333333333333333703, 0.3333333333333333703, 0.3333333333333333703, 0.3333333333333333703, 0.3333333333333333703, 0.3333333333333333703, 0.3333333333333333703, 0.3333333333333333703, 0.3333333333333333703, 0.3333333333333333703, 0.3333333333333333703, 0.3333333333333333703, 0.3333333333333333703, 0.3333333333333333703, 0.3333333333333333703, 0.3333333333333333703, 0.3333333333333333703, 0.3333333333333333703, 0.3333333333333333703, 0.3333333333333333703, 0.3333333333333333703, 0.3333333333333333703, 0.3333333333333333703),
 ( 0.3333333333333333703, 0.3333333333333333703, 0.3333333333333333703, 0.3333333333333333703, 0.3333333333333333703, 0.3333333333333333703, 0.3333333333333333703, 0.3333333333333333703, 0.3333333333333333703, 0.3333333333333333703, 0.3333333333333333703, 0.3333333333333333703, 0.3333333333333333703, 0.3333333333333333703, 0.3333333333333333703, 0.3333333333333333703, 0.3333333333333333703, 0.3333333333333333703, 0.3333333333333333703, 0.3333333333333333703, 0.3333333333333333703, 0.3333333333333333703, 0.3333333333333333703, 0.3333333333333333703, 0.3333333333333333703, 0.3333333333333333703, 0.3333333333333333703, 0.3333333333333333703, 0.3333333333333333703, 0.3333333333333333703),
 ( 1.000000000000000000, 1.000000000000000000, 1.000000000000000000, 1.000000000000000000, 1.000000000000000000, 1.000000000000000000, 1.000000000000000000, 1.000000000000000000, 1.000000000000000000, 1.000000000000000000, 1.000000000000000000, 1.000000000000000000, 1.000000000000000000, 1.000000000000000000, 1.000000000000000000, 1.000000000000000000, 1.000000000000000000, 1.000000000000000000, 1.000000000000000000, 1.000000000000000000, 1.000000000000000000, 1.000000000000000000, 1.000000000000000000, 1.000000000000000000, 1.000000000000000000, 1.000000000000000000, 1.000000000000000000, 1.000000000000000000, 1.000000000000000000, 1.000000000000000000),
 ( 0.3333333333333333703, 0.3333333333333333703, 0.3333333333333333703, 0.3333333333333333703, 0.3333333333333333703, 0.3333333333333333703, 0.3333333333333333703, 0.3333333333333333703, 0.3333333333333333703, 0.3333333333333333703, 0.3333333333333333703, 0.3333333333333333703, 0.3333333333333333703, 0.3333333333333333703, 0.3333333333333333703, 0.3333333333333333703, 0.3333333333333333703, 0.3333333333333333703, 0.3333333333333333703, 0.3333333333333333703, 0.3333333333333333703, 0.3333333333333333703, 0.3333333333333333703, 0.3333333333333333703, 0.3333333333333333703, 0.3333333333333333703, 0.3333333333333333703, 0.3333333333333333703, 0.3333333333333333703, 0.3333333333333333703),
 ( 0.3333333333333333703, 0.3333333333333333703, 0.3333333333333333703, 0.3333333333333333703, 0.3333333333333333703, 0.3333333333333333703, 0.3333333333333333703, 0.3333333333333333703, 0.3333333333333333703, 0.3333333333333333703, 0.3333333333333333703, 0.3333333333333333703, 0.3333333333333333703, 0.3333333333333333703, 0.3333333333333333703, 0.3333333333333333703, 0.3333333333333333703, 0.3333333333333333703, 0.3333333333333333703, 0.3333333333333333703, 0.3333333333333333703, 0.3333333333333333703, 0.3333333333333333703, 0.3333333333333333703, 0.3333333333333333703, 0.3333333333333333703, 0.3333333333333333703, 0.3333333333333333703, 0.3333333333333333703, 0.3333333333333333703),
 ( 1.000000000000000000, 1.000000000000000000, 1.000000000000000000, 1.000000000000000000, 1.000000000000000000, 1.000000000000000000, 1.000000000000000000, 1.000000000000000000, 1.000000000000000000, 1.000000000000000000, 1.000000000000000000, 1.000000000000000000, 1.000000000000000000, 1.000000000000000000, 1.000000000000000000, 1.000000000000000000, 1.000000000000000000, 1.000000000000000000, 1.000000000000000000, 1.000000000000000000, 1.000000000000000000, 1.000000000000000000, 1.000000000000000000, 1.000000000000000000, 1.000000000000000000, 1.000000000000000000, 1.000000000000000000, 1.000000000000000000, 1.000000000000000000, 1.000000000000000000) ) ) 
 REPRESENTATION_ITEM ( '' )  SURFACE ( )  );
#4188=CARTESIAN_POINT ( 'NONE',  ( -200.0000000000000000, 22.85346793133691889, 44.96258949770047764 ) ) ;
#4189=CARTESIAN_POINT ( 'NONE',  ( 57.59792236341148453, -54.84617931850877426, -1.722363176415331099 ) ) ;
#4190=CARTESIAN_POINT ( 'NONE',  ( -77.80650228860213247, 20.78729124363272973, 7.074397727529034618 ) ) ;
#4191=CARTESIAN_POINT ( 'NONE',  ( 151.7948205124836250, 23.49921654116328540, 23.49921654116366554 ) ) ;
#4192=CARTESIAN_POINT ( 'NONE',  ( 146.6084372240433709, -5.374981219216948602, 40.00000000000002132 ) ) ;
#4193=CARTESIAN_POINT ( 'NONE',  ( 163.1118516004056573, 19.27778845538780317, -19.27778845538757224 ) ) ;
#4194=CARTESIAN_POINT ( 'NONE',  ( 0.2972598230770129857, -54.33493731733938148, 40.00000000000002132 ) ) ;
#4195=CARTESIAN_POINT ( 'NONE',  ( -105.4741150117367283, 19.77569912955882359, -7.943527260733686646 ) ) ;
#4196=CARTESIAN_POINT ( 'NONE',  ( -162.0762913951021176, 40.00000000000001421, -1.694272876827905394 ) ) ;
#4197=CARTESIAN_POINT ( 'NONE',  ( 192.4448373802101173, 42.42640687116508502, -14.14213562375874567 ) ) ;
#4198=CARTESIAN_POINT ( 'NONE',  ( -100.7734535825088500, -22.67402823373193499, -40.00000000000002132 ) ) ;
#4201=CARTESIAN_POINT ( 'NONE',  ( 130.8568914410475372, -34.05028731879786363, 0.000000000000000000 ) ) ;
#4202=CARTESIAN_POINT ( 'NONE',  ( -99.29480781227057662, -8.165122821357709171, -20.80016781325170783 ) ) ;
#4203=CARTESIAN_POINT ( 'NONE',  ( 0.2972598230769883387, 39.99999999999997158, 14.33493731733947563 ) ) ;
#4204=CARTESIAN_POINT ( 'NONE',  ( -91.56559293963834989, 40.53558337403654832, 16.03295912088756481 ) ) ;
#4205=CARTESIAN_POINT ( 'NONE',  ( 151.7948205124836250, -33.23291073765550863, 0.000000000000000000 ) ) ;
#4207=CARTESIAN_POINT ( 'NONE',  ( -126.6834156231674342, 9.107266674873963908, -24.89646324320098714 ) ) ;
#4210=ADVANCED_FACE ( 'NONE', ( #9895, #16414 ), #22677, .F. ) ;
#4212=CARTESIAN_POINT ( 'NONE',  ( 19.06497207195981147, 38.31983398719673772, -38.31983398719579981 ) ) ;
#4213=CARTESIAN_POINT ( 'NONE',  ( -238.4067589809705794, -57.25054294077233408, -0.6820004458489551391 ) ) ;
#4215=CARTESIAN_POINT ( 'NONE',  ( -259.2033419157646676, 40.00000000000029843, -30.48217210827696988 ) ) ;
#4216=CARTESIAN_POINT ( 'NONE',  ( -135.8532207217289738, -50.09629031063973770, 6.472252184283735943 ) ) ;
#4217=CARTESIAN_POINT ( 'NONE',  ( 199.9999999999999432, -14.14213562373115884, 14.14213562373085153 ) ) ;
#4218=CARTESIAN_POINT ( 'NONE',  ( -105.3755690713226585, -43.67073346367983788, 12.89780903124397149 ) ) ;
#4220=CARTESIAN_POINT ( 'NONE',  ( -192.9588430854690273, -38.51493924976932703, -18.05360324515463688 ) ) ;
#4225=CARTESIAN_POINT ( 'NONE',  ( -280.0000000000000568, 39.99999999999990763, 20.00000000000015987 ) ) ;
#4227=CARTESIAN_POINT ( 'NONE',  ( 22.82148508083511729, 43.16138278736985967, -17.87803012130492775 ) ) ;
#4228=CARTESIAN_POINT ( 'NONE',  ( -208.1127848780264742, 15.00245453012665742, -40.00000000000002132 ) ) ;
#4229=CARTESIAN_POINT ( 'NONE',  ( -56.48582580120559271, -9.153146818113595984, 0.000000000000000000 ) ) ;
#4230=CARTESIAN_POINT ( 'NONE',  ( -3.675706741949858802, -43.24173023805415994, 17.91131112508043088 ) ) ;
#4231=B_SPLINE_CURVE_WITH_KNOTS ( 'NONE', 3,
 ( #15197, #19693, #1481, #23444, #17692, #15692, #9082, #21197, #23817, #11080, #977, #19194 ),
 .UNSPECIFIED., .F., .F.,
 ( 4, 2, 2, 2, 2, 4 ),
 ( 1.471635563490154540E-15, 0.004698945756008183518, 0.007048418634011560137, 0.009397891512014935889, 0.01409683726802164749, 0.01879578302402835910 ),
 .UNSPECIFIED. ) ;
#4232=CARTESIAN_POINT ( 'NONE',  ( -100.7734535825088358, 17.32597176626809343, 2.449293598294708485E-15 ) ) ;
#4235=CARTESIAN_POINT ( 'NONE',  ( 0.2972598230769990524, -18.14793986248724522, 38.42060263243662632 ) ) ;
#4236=CARTESIAN_POINT ( 'NONE',  ( -7.297127544296671431, -13.59739983758519699, 45.86058602276306573 ) ) ;
#4237=B_SPLINE_CURVE_WITH_KNOTS ( 'NONE', 3,
 ( #18504, #6795, #424, #14906, #6397, #20914 ),
 .UNSPECIFIED., .F., .F.,
 ( 4, 2, 4 ),
 ( 2.417129106265379096E-15, 0.03937685942888179830, 0.07875371885776118186 ),
 .UNSPECIFIED. ) ;
#4238=CARTESIAN_POINT ( 'NONE',  ( -3.473570583883086371, 17.93385599103773487, -43.29615835920785116 ) ) ;
#4240=CARTESIAN_POINT ( 'NONE',  ( -105.4741150117382773, -19.77569912955116749, -7.943527260750395946 ) ) ;
#4242=CARTESIAN_POINT ( 'NONE',  ( -174.2682069747356479, -16.26528465553954206, 39.26787081107618604 ) ) ;
#4243=CARTESIAN_POINT ( 'NONE',  ( 91.82158438592158234, 16.11829626346161604, -16.11829626346121103 ) ) ;
#4244=CARTESIAN_POINT ( 'NONE',  ( -91.56559293963836410, 22.67402823373189946, -0.000000000000000000 ) ) ;
#4245=CARTESIAN_POINT ( 'NONE',  ( -188.4265466358252752, 23.47687925214783533, -43.04237830660004249 ) ) ;
#4246=DIRECTION ( 'NONE',  ( -1.000000000000000000, -1.836970198721030181E-16, -0.000000000000000000 ) ) ;
#4247=CARTESIAN_POINT ( 'NONE',  ( -259.2033419157646676, 21.55415060305790931, 35.01439189186571355 ) ) ;
#4248=CARTESIAN_POINT ( 'NONE',  ( 200.0000000000000000, -19.99999999999988631, -40.00000000000002132 ) ) ;
#4249=CARTESIAN_POINT ( 'NONE',  ( -105.3755690713226585, 18.24025645688350750, -40.00000000000002132 ) ) ;
#4250=CARTESIAN_POINT ( 'NONE',  ( -213.1075012329537230, 1.045191102001431893E-13, -13.71589010951911902 ) ) ;
#4251=CARTESIAN_POINT ( 'NONE',  ( 163.1118516004056573, -19.27778845539233998, 37.29075403953149959 ) ) ;
#4253=CARTESIAN_POINT ( 'NONE',  ( 0.2972598230770048811, -10.13633138497415942, -66.70487387989865624 ) ) ;
#4254=ORIENTED_EDGE ( 'NONE', *, *, #17937, .F. ) ;
#4255=CARTESIAN_POINT ( 'NONE',  ( 14.38125909742181285, -17.55144818341476309, 39.01709431150910490 ) ) ;
#4256=CARTESIAN_POINT ( 'NONE',  ( -190.1935349183500534, -13.92226178597258723, -47.62328764229022227 ) ) ;
#4258=CARTESIAN_POINT ( 'NONE',  ( 0.2972598230770027716, -38.42060263243656237, -18.14793986248737667 ) ) ;
#4259=CARTESIAN_POINT ( 'NONE',  ( 2.332272417551007226, -48.72342300852339037, -14.08759251167714943 ) ) ;
#4260=ORIENTED_EDGE ( 'NONE', *, *, #704, .F. ) ;
#4261=CARTESIAN_POINT ( 'NONE',  ( -88.39148973765023243, -20.15708830332361856, 8.027153355909467436 ) ) ;
#4267=DIRECTION ( 'NONE',  ( 0.000000000000000000, 1.000000000000000000, 0.000000000000000000 ) ) ;
#4268=CARTESIAN_POINT ( 'NONE',  ( 170.2234770963711128, -17.36149277826985937, -17.36149277826995174 ) ) ;
#4269=CARTESIAN_POINT ( 'NONE',  ( -173.7925586253313668, -41.93433064649144626, -12.78856870755330633 ) ) ;
#4270=CARTESIAN_POINT ( 'NONE',  ( 91.82158438592159655, -40.00000000000008527, 22.79471317813456110 ) ) ;
#4271=CARTESIAN_POINT ( 'NONE',  ( 146.6084372240433709, -34.62501878078303008, 40.00000000000002132 ) ) ;
#4274=EDGE_CURVE ( 'NONE', #20612, #16255, #3895, .T. ) ;
#4275=CARTESIAN_POINT ( 'NONE',  ( -238.4067589809705794, -40.00000000000021316, 40.96449427990166470 ) ) ;
#4276=CARTESIAN_POINT ( 'NONE',  ( -135.8532207217289738, -40.00000000000014921, 30.84685318188631697 ) ) ;
#4277=CARTESIAN_POINT ( 'NONE',  ( -198.0356074513804572, 39.99999999999992895, 15.37879056873084771 ) ) ;
#4278=CARTESIAN_POINT ( 'NONE',  ( -208.1127848780264742, -15.00245453012673202, -40.00000000000002132 ) ) ;
#4279=CARTESIAN_POINT ( 'NONE',  ( -162.0762913951020892, -57.76657433524000851, 1.198031840315820329 ) ) ;
#4280=CARTESIAN_POINT ( 'NONE',  ( 0.2972598230770130412, -54.33493731733936016, -2.449293598294708485E-15 ) ) ;
#4281=CARTESIAN_POINT ( 'NONE',  ( 136.1360204305621551, 24.77266263493108411, 31.79587985999273769 ) ) ;
#4282=CARTESIAN_POINT ( 'NONE',  ( 128.5824617753800680, -11.99766463964393637, -28.96492468983277035 ) ) ;
#4285=CARTESIAN_POINT ( 'NONE',  ( 91.82158438592156813, 39.99999999999986500, 17.20528682183341473 ) ) ;
#4286=CARTESIAN_POINT ( 'NONE',  ( -238.4067589809705794, -1.892706720741712928E-13, 40.96449427998260973 ) ) ;
#4287=CARTESIAN_POINT ( 'NONE',  ( -135.8532207217289738, 21.81201906317777883, -34.75652343174605363 ) ) ;
#4290=CARTESIAN_POINT ( 'NONE',  ( -91.56559293963834989, -40.53558337403669753, -16.03295912088728770 ) ) ;
#4291=EDGE_LOOP ( 'NONE', ( #12196, #25344, #12029, #20080 ) ) ;
#4292=CARTESIAN_POINT ( 'NONE',  ( 4.995406935893294431, -17.50105314357144337, -39.06748935135212264 ) ) ;
#4293=CARTESIAN_POINT ( 'NONE',  ( 98.29820294270297154, 18.47759065022021474, -7.653668647299666894 ) ) ;
#4294=CARTESIAN_POINT ( 'NONE',  ( -238.4067589809705794, -40.96449427990185654, -40.00000000000002132 ) ) ;
#4297=CARTESIAN_POINT ( 'NONE',  ( -198.9233928135198539, -14.16707757975730608, -49.24835219440220158 ) ) ;
#4299=( BOUNDED_SURFACE ( )  B_SPLINE_SURFACE ( 3, 2, ( 
 ( #22878, #12758, #16881 ),
 ( #25013, #2662, #18343 ),
 ( #8898, #794, #17008 ),
 ( #25146, #6897, #15014 ),
 ( #4793, #19016, #12895 ),
 ( #21009, #2791, #10904 ) ),
 .UNSPECIFIED., .F., .F., .F. ) 
 B_SPLINE_SURFACE_WITH_KNOTS ( ( 4, 2, 4 ),
 ( 3, 3 ),
 ( 0.04143177204414218162, 0.04845749460459651548, 0.05548321716505084933 ),
 ( 0.000000000000000000, 1.000000000000000000 ),
 .UNSPECIFIED. ) 
 GEOMETRIC_REPRESENTATION_ITEM ( )  RATIONAL_B_SPLINE_SURFACE ( (
 ( 1.000000000000000000, 0.9541700777564562364, 1.000000000000000000),
 ( 1.000000000000000000, 0.9520119497953954957, 1.000000000000000000),
 ( 1.000000000000000000, 0.9503149742541672218, 1.000000000000000000),
 ( 1.000000000000000000, 0.9480088400359243384, 1.000000000000000000),
 ( 1.000000000000000000, 0.9474362536298478465, 1.000000000000000000),
 ( 1.000000000000000000, 0.9474350312570024579, 1.000000000000000000) ) ) 
 REPRESENTATION_ITEM ( '' )  SURFACE ( )  );
#4300=ORIENTED_EDGE ( 'NONE', *, *, #18004, .T. ) ;
#4303=CARTESIAN_POINT ( 'NONE',  ( 22.31419732600696904, 17.93420418956782214, 43.29699898481114673 ) ) ;
#4304=EDGE_LOOP ( 'NONE', ( #18143, #20206, #24312, #4993, #6022, #2413, #20180, #22349, #2826 ) ) ;
#4306=ORIENTED_EDGE ( 'NONE', *, *, #13609, .T. ) ;
#4307=CARTESIAN_POINT ( 'NONE',  ( -91.56559293963834989, -22.67402823373193499, 0.000000000000000000 ) ) ;
#4309=FACE_OUTER_BOUND ( 'NONE', #6498, .T. ) ;
#4310=ADVANCED_FACE ( 'NONE', ( #180 ), #6990, .T. ) ;
#4311=EDGE_CURVE ( 'NONE', #17229, #17458, #401, .T. ) ;
#4312=CARTESIAN_POINT ( 'NONE',  ( -96.94475454968227268, -8.190683501865384741, -20.92018922312004037 ) ) ;
#4313=CARTESIAN_POINT ( 'NONE',  ( 0.2972598230769956662, 40.00000000000058975, -54.33493731733894094 ) ) ;
#4314=CARTESIAN_POINT ( 'NONE',  ( 199.9999999999999432, -1.727494763561684666E-13, 20.00000000000010303 ) ) ;
#4318=CARTESIAN_POINT ( 'NONE',  ( -191.2489946134182901, 18.16428294930770093, 43.85245824700565720 ) ) ;
#4319=CARTESIAN_POINT ( 'NONE',  ( 136.1360204305621266, -3.511608612530630058, -3.511608612530719764 ) ) ;
#4320=CARTESIAN_POINT ( 'NONE',  ( -102.4068193528145088, 20.17396017424893984, -8.735227608997000459 ) ) ;
#4321=CARTESIAN_POINT ( 'NONE',  ( -30.26275506840325136, 27.08623969584573388, 29.48230279907808793 ) ) ;
#4322=CARTESIAN_POINT ( 'NONE',  ( -77.59261320673972762, 2.779275804817392448, 21.93453874213112087 ) ) ;
#4323=CARTESIAN_POINT ( 'NONE',  ( 146.6084372240433709, 52.76785682606523409, -3.800685668858194255 ) ) ;
#4324=CARTESIAN_POINT ( 'NONE',  ( -280.0000000000000000, 19.99999999999996092, -0.000000000000000000 ) ) ;
#4325=CARTESIAN_POINT ( 'NONE',  ( -135.8532207217289738, -6.472252184284280396, 6.472252184284099208 ) ) ;
#4326=CIRCLE ( 'NONE', #20006, 15.00000000000000178 ) ;
#4327=CARTESIAN_POINT ( 'NONE',  ( -280.0000000000000568, 19.99999999999996092, 40.00000000000002132 ) ) ;
#4328=CARTESIAN_POINT ( 'NONE',  ( -93.02511667906875914, 20.82219708225684940, -8.169918093965478079 ) ) ;
#4329=CARTESIAN_POINT ( 'NONE',  ( 130.8568914410475088, 39.99999999999969447, 34.05028731879830417 ) ) ;
#4330=CARTESIAN_POINT ( 'NONE',  ( -280.0000000000000000, -14.14213562373098831, -14.14213562373098654 ) ) ;
#4331=CARTESIAN_POINT ( 'NONE',  ( 14.38125909742180752, 15.17850393972634038, 0.000000000000000000 ) ) ;
#4334=CARTESIAN_POINT ( 'NONE',  ( 192.4448373802100889, -20.00000000003938538, 0.000000000000000000 ) ) ;
#4335=CARTESIAN_POINT ( 'NONE',  ( -100.0753760173602700, -8.149786832858715968, -20.72827493166402135 ) ) ;
#4336=CARTESIAN_POINT ( 'NONE',  ( 200.0000000000000000, 42.42640687119267540, 14.14213562373153543 ) ) ;
#4338=( BOUNDED_CURVE ( )  B_SPLINE_CURVE ( 3, ( #1130, #6839, #12968, #15085, #14821, #14959, #10980 ),
 .UNSPECIFIED., .F., .F. ) 
 B_SPLINE_CURVE_WITH_KNOTS ( ( 4, 3, 4 ),
 ( 0.0006517261993840123800, 0.02240322356231545103, 0.03884882555987133335 ),
 .UNSPECIFIED. ) 
 CURVE ( )  GEOMETRIC_REPRESENTATION_ITEM ( )  RATIONAL_B_SPLINE_CURVE ( ( 0.5249926329037828410, 0.5828554938567718224, 0.7411912828888442828, 1.000000000000000000, 0.8043231192735467161, 0.6660804010233453143, 0.5852718452493959056 ) ) 
 REPRESENTATION_ITEM ( '' )  );
#4342=CARTESIAN_POINT ( 'NONE',  ( -213.1075012329537230, -18.58567234101102272, -37.98287015391260013 ) ) ;
#4343=CARTESIAN_POINT ( 'NONE',  ( -135.8532207217289738, -21.81201906317806305, 34.75652343174590442 ) ) ;
#4344=CARTESIAN_POINT ( 'NONE',  ( -105.4113873279013660, 20.16970153814047961, 7.043304828828932607 ) ) ;
#4345=CARTESIAN_POINT ( 'NONE',  ( 91.82158438592156813, 40.00000000000027711, -22.79471317813428044 ) ) ;
#4346=CARTESIAN_POINT ( 'NONE',  ( 4.995406935893297984, -39.06748935135205869, 17.50105314357158193 ) ) ;
#4348=CARTESIAN_POINT ( 'NONE',  ( -138.9613193425346651, -13.65853114850577121, -27.95779829453082499 ) ) ;
#4349=CARTESIAN_POINT ( 'NONE',  ( -91.56559293963834989, -40.53558337403669753, -16.03295912088728770 ) ) ;
#4352=CARTESIAN_POINT ( 'NONE',  ( -259.2033419157646676, -1.564921101325656229E-13, 30.48217210827739621 ) ) ;
#4355=CARTESIAN_POINT ( 'NONE',  ( 25.05785482530196617, 42.53113694082225038, -17.61697374401517990 ) ) ;
#4356=CARTESIAN_POINT ( 'NONE',  ( 130.8568914410475088, 5.949712681206719367, -40.00000000000002132 ) ) ;
#4357=CARTESIAN_POINT ( 'NONE',  ( 163.1118516004056573, 27.26290988616875310, 0.000000000000000000 ) ) ;
#4358=CARTESIAN_POINT ( 'NONE',  ( 18.89824403360313454, -24.18164459663342214, -43.99464769172848122 ) ) ;
#4359=B_SPLINE_CURVE_WITH_KNOTS ( 'NONE', 3,
 ( #24552, #22427, #20288, #4335, #4202, #10174, #8034, #2067, #12295, #18278, #2324, #63 ),
 .UNSPECIFIED., .F., .F.,
 ( 4, 2, 2, 2, 2, 4 ),
 ( 1.695971460814453879E-15, 0.004698945756008356123, 0.007048418634011665955, 0.009397891512014975787, 0.01409683726802159545, 0.01879578302402821338 ),
 .UNSPECIFIED. ) ;
#4360=CARTESIAN_POINT ( 'NONE',  ( -3.977426076247516207, -43.16039317622677629, 17.87762021094849274 ) ) ;
#4361=CARTESIAN_POINT ( 'NONE',  ( -91.56559293963834989, 17.32597176626808988, 40.00000000000002132 ) ) ;
#4362=VERTEX_POINT ( 'NONE', #4681 ) ;
#4363=CARTESIAN_POINT ( 'NONE',  ( 22.89172254855150257, 23.44749030158443048, -43.00256445985473164 ) ) ;
#4364=CARTESIAN_POINT ( 'NONE',  ( 91.82158438592158234, -12.16597498397761967, -12.16597498397768007 ) ) ;
#4367=CARTESIAN_POINT ( 'NONE',  ( 3.869409319519631296, 24.63759630012732060, -44.61273074174879838 ) ) ;
#4369=CARTESIAN_POINT ( 'NONE',  ( -135.8532207217289738, -1.208299557080134822E-13, 9.153146818113572891 ) ) ;
#4371=CARTESIAN_POINT ( 'NONE',  ( -188.9524938556157281, -13.86227398172938230, 47.22059665006405282 ) ) ;
#4372=CARTESIAN_POINT ( 'NONE',  ( 170.2234770963711128, -17.36149277826940462, -39.20704971665412586 ) ) ;
#4373=CARTESIAN_POINT ( 'NONE',  ( -105.2274517607667974, 13.17594969605270627, -17.01575307708425200 ) ) ;
#4374=CARTESIAN_POINT ( 'NONE',  ( -188.4702232936790836, 23.48628015403081193, -43.05505437950374414 ) ) ;
#4375=CARTESIAN_POINT ( 'NONE',  ( -91.56559293963834989, 12.25131212657428748, 44.31723036834913643 ) ) ;
#4376=CARTESIAN_POINT ( 'NONE',  ( 57.59792236341147031, 26.56190807104652052, 30.00663442387728708 ) ) ;
#4377=CARTESIAN_POINT ( 'NONE',  ( 4.995406935893307754, -55.24977328853207581, -40.00000000000002132 ) ) ;
#4378=CARTESIAN_POINT ( 'NONE',  ( 170.2234770963711128, 15.44714144992818738, 40.00000000000002132 ) ) ;
#4379=CARTESIAN_POINT ( 'NONE',  ( 14.38125909742181108, 1.616281842095393922E-13, -15.17850393972633682 ) ) ;
#4380=CARTESIAN_POINT ( 'NONE',  ( -135.8532207217289738, 21.81201906317767936, 21.81201906317778239 ) ) ;
#4381=CARTESIAN_POINT ( 'NONE',  ( -86.86493150571118349, 19.60045294882759137, -8.366608963953964917 ) ) ;
#4382=CARTESIAN_POINT ( 'NONE',  ( 136.1360204305621551, 24.77266263493153176, -31.79587985999237887 ) ) ;
#4383=CARTESIAN_POINT ( 'NONE',  ( 0.2972598230769976091, -10.13633138497479180, 10.13633138497468522 ) ) ;
#4386=CARTESIAN_POINT ( 'NONE',  ( -100.7734535825088358, -16.03295912088706743, -16.03295912088710296 ) ) ;
#4387=CARTESIAN_POINT ( 'NONE',  ( -89.91498783734833466, 8.733585468302273114, 20.17141720476648814 ) ) ;
#4388=CARTESIAN_POINT ( 'NONE',  ( -91.56559293963834989, 16.03295912088683650, 40.53558337403684675 ) ) ;
#4389=CARTESIAN_POINT ( 'NONE',  ( -4.022465846214378971, -46.99661175925217549, -13.82902411340760196 ) ) ;
#4391=CARTESIAN_POINT ( 'NONE',  ( -105.4741150117369273, 8.366608964608960974, -19.60045294982168329 ) ) ;
#4392=CARTESIAN_POINT ( 'NONE',  ( -77.55640685876515761, -15.64922766773197260, -15.64922766773223550 ) ) ;
#4395=CARTESIAN_POINT ( 'NONE',  ( -114.7823189589618380, -22.12960287296361273, -1.412059986351657637 ) ) ;
#4396=CARTESIAN_POINT ( 'NONE',  ( -192.1964066538670863, -43.96877160662432260, -24.16259023441631371 ) ) ;
#4397=CARTESIAN_POINT ( 'NONE',  ( 0.2972598230770103767, -40.00000000000021316, 54.33493731733921805 ) ) ;
#4398=CARTESIAN_POINT ( 'NONE',  ( 130.8568914410475372, 5.949712681206715814, 2.449293598294708485E-15 ) ) ;
#4401=CARTESIAN_POINT ( 'NONE',  ( -259.2033419157646676, -1.564921101325656229E-13, 30.48217210827739621 ) ) ;
#4402=CARTESIAN_POINT ( 'NONE',  ( -105.3755690713226585, 40.00000000000007816, -21.75974354311636461 ) ) ;
#4403=CARTESIAN_POINT ( 'NONE',  ( -4.039451493210490796, 46.99046209229823745, -13.82811171175438147 ) ) ;
#4404=CARTESIAN_POINT ( 'NONE',  ( -198.0356074513804572, -15.37879056873074290, 0.000000000000000000 ) ) ;
#4405=CARTESIAN_POINT ( 'NONE',  ( -198.0356074513804572, -55.37879056874826489, 40.00000000000002132 ) ) ;
#4406=CARTESIAN_POINT ( 'NONE',  ( -192.9588430854690273, 18.05360324515418924, 38.51493924976949756 ) ) ;
#4407=CARTESIAN_POINT ( 'NONE',  ( -91.56559293963834989, -2.543181659092656077E-13, 22.67402823373191723 ) ) ;
#4408=CARTESIAN_POINT ( 'NONE',  ( -188.2995950289364657, -23.44932284466040784, 43.00522595870950937 ) ) ;
#4409=CARTESIAN_POINT ( 'NONE',  ( -259.2033419157646676, 2.741182173978444749E-13, -30.48217210827739621 ) ) ;
#4410=CARTESIAN_POINT ( 'NONE',  ( 91.82158438592158234, -6.516925787240506436E-14, 22.79471317813470321 ) ) ;
#4411=CARTESIAN_POINT ( 'NONE',  ( 170.2234770963711128, -17.36149277826985937, -17.36149277826995174 ) ) ;
#4414=CARTESIAN_POINT ( 'NONE',  ( -238.4067589809705794, -57.25054294065807881, 0.6820004457338858517 ) ) ;
#4415=ORIENTED_EDGE ( 'NONE', *, *, #8905, .T. ) ;
#4416=CARTESIAN_POINT ( 'NONE',  ( -8.720657192080711440, 41.62108041047287799, -22.53512351407914593 ) ) ;
#4417=CARTESIAN_POINT ( 'NONE',  ( -4.039451493210483690, -23.44932283416618191, -43.00522595894033628 ) ) ;
#4418=CARTESIAN_POINT ( 'NONE',  ( -192.9588430854690273, -54.46834944101725284, -40.00000000000002132 ) ) ;
#4419=CARTESIAN_POINT ( 'NONE',  ( -87.13361725327072804, -21.49321519333430786, -1.371494219583687668 ) ) ;
#4420=CARTESIAN_POINT ( 'NONE',  ( -162.0762913951020892, 1.694272876828294194, 0.000000000000000000 ) ) ;
#4422=ORIENTED_EDGE ( 'NONE', *, *, #2584, .T. ) ;
#4425=CARTESIAN_POINT ( 'NONE',  ( 125.5832160019860169, 11.61997419108396734, -28.05309928653990781 ) ) ;
#4426=CARTESIAN_POINT ( 'NONE',  ( 22.66553228237577855, 17.89571368754772607, 43.20407469282439905 ) ) ;
#4428=VERTEX_POINT ( 'NONE', #16642 ) ;
#4429=CARTESIAN_POINT ( 'NONE',  ( -56.48582580120559982, -34.75652343174615311, 21.81201906317766870 ) ) ;
#4432=DIRECTION ( 'NONE',  ( 0.000000000000000000, 0.9166903767332116315, -0.3995982397417718879 ) ) ;
#4433=CARTESIAN_POINT ( 'NONE',  ( 170.2234770963711128, 10.92277846919201068, 10.92277846919202133 ) ) ;
#4434=CARTESIAN_POINT ( 'NONE',  ( -199.9999999999999432, -24.32899771311792136, 44.86773131993664521 ) ) ;
#4436=CARTESIAN_POINT ( 'NONE',  ( 200.0000000000000000, 39.99999999999985079, 20.00000000000052225 ) ) ;
#4437=CARTESIAN_POINT ( 'NONE',  ( 170.2234770963711128, 39.99999999999980105, 24.55285855007229401 ) ) ;
#4441=CARTESIAN_POINT ( 'NONE',  ( -187.3036811847890419, 23.25512365539898596, 42.71162014090150905 ) ) ;
#4442=CARTESIAN_POINT ( 'NONE',  ( 57.59792236341147031, 1.722363176415040886, 1.722363176415060426 ) ) ;
#4444=CARTESIAN_POINT ( 'NONE',  ( -200.0000000000000568, 21.40989205436302711, 45.24754806068986568 ) ) ;
#4445=CARTESIAN_POINT ( 'NONE',  ( -238.4067589809705794, -0.6820004458488042598, 57.25054294077229855 ) ) ;
#4447=CARTESIAN_POINT ( 'NONE',  ( -100.7734535825088500, 44.31723036834907958, -12.25131212657445801 ) ) ;
#4449=CARTESIAN_POINT ( 'NONE',  ( 4.995406935893293543, -15.24977328854832592, 0.000000000000000000 ) ) ;
#4450=ADVANCED_FACE ( 'NONE', ( #6524 ), #15995, .T. ) ;
#4451=CARTESIAN_POINT ( 'NONE',  ( -162.0762913951021176, 29.48230308784730980, 27.08623940707652622 ) ) ;
#4452=CARTESIAN_POINT ( 'NONE',  ( -86.96347745069645896, 21.75974354311648895, 40.00000000000002132 ) ) ;
#4454=CARTESIAN_POINT ( 'NONE',  ( 163.1118516004056573, 39.99999999999976552, 27.26290988616914746 ) ) ;
#4455=ADVANCED_FACE ( 'NONE', ( #8709 ), #5983, .T. ) ;
#4461=CARTESIAN_POINT ( 'NONE',  ( 163.1118516004056573, -27.26290988616869626, 40.00000000000002132 ) ) ;
#4463=CARTESIAN_POINT ( 'NONE',  ( 4.995406935893290878, 39.06748935135239265, -39.06748935135144762 ) ) ;
#4465=CARTESIAN_POINT ( 'NONE',  ( -198.0012279374157629, -44.79720170867064155, -24.77357825033872629 ) ) ;
#4469=CARTESIAN_POINT ( 'NONE',  ( 14.38125909742181285, -17.55144818341421598, -39.01709431150935359 ) ) ;
#4471=CARTESIAN_POINT ( 'NONE',  ( -86.96347745069645896, 40.00000000000019895, -18.24025645688310249 ) ) ;
#4472=CARTESIAN_POINT ( 'NONE',  ( 14.38125909742181285, -10.73282306404712472, -10.73282306404731301 ) ) ;
#4473=CARTESIAN_POINT ( 'NONE',  ( 151.7948205124836250, 33.23291073765556547, 0.000000000000000000 ) ) ;
#4474=CARTESIAN_POINT ( 'NONE',  ( -163.5815439473252866, -18.59457101086894681, -35.61501074501018849 ) ) ;
#4475=CARTESIAN_POINT ( 'NONE',  ( -208.1127848780264742, -38.89260858015728672, -17.67593391476669851 ) ) ;
#4478=CARTESIAN_POINT ( 'NONE',  ( 151.7948205124836534, -40.00000000000001421, 6.767089262348889633 ) ) ;
#4481=CARTESIAN_POINT ( 'NONE',  ( 22.66553228237832585, 43.20407469282481827, -17.89571368754818081 ) ) ;
#4482=CARTESIAN_POINT ( 'NONE',  ( -280.0000000000000568, 19.99999999999996447, -40.00000000000002132 ) ) ;
#4483=CARTESIAN_POINT ( 'NONE',  ( -213.1075012329537230, -13.71589010951915810, 0.000000000000000000 ) ) ;
#4484=CARTESIAN_POINT ( 'NONE',  ( -213.1075012329537230, 53.71589010953660193, 40.00000000000002132 ) ) ;
#4485=B_SPLINE_CURVE_WITH_KNOTS ( 'NONE', 3,
 ( #23479, #11477, #1391, #11356, #7488, #19472 ),
 .UNSPECIFIED., .F., .F.,
 ( 4, 2, 4 ),
 ( -0.0001324603514699870008, 0.04003639359265966785, 0.08020524753678931473 ),
 .UNSPECIFIED. ) ;
#4486=CARTESIAN_POINT ( 'NONE',  ( -4.339409867971073531, -43.06267456183169173, 17.83714383556879923 ) ) ;
#4487=CARTESIAN_POINT ( 'NONE',  ( -100.7734535825088500, 17.32597176626808988, 40.00000000000002132 ) ) ;
#4488=EDGE_LOOP ( 'NONE', ( #15103, #19715, #16978, #18514 ) ) ;
#4489=CARTESIAN_POINT ( 'NONE',  ( -199.9999999999999147, 46.69454133506851434, 26.45173932753578683 ) ) ;
#4491=CARTESIAN_POINT ( 'NONE',  ( -4.076660308449226555, -13.82548859978938260, 46.97758120990467035 ) ) ;
#4492=CARTESIAN_POINT ( 'NONE',  ( 6.984886629811533076, 24.81009931999678031, -44.84679502273271368 ) ) ;
#4494=CARTESIAN_POINT ( 'NONE',  ( 136.1360204305621266, -24.77266263493151044, 24.77266263493093135 ) ) ;
#4497=CARTESIAN_POINT ( 'NONE',  ( -188.8842637254074646, -17.93596642850445733, 43.30125340596327987 ) ) ;
#4498=CARTESIAN_POINT ( 'NONE',  ( 170.2234770963711128, -40.00000000000024158, 24.55285855007145202 ) ) ;
#4499=CARTESIAN_POINT ( 'NONE',  ( 130.8568914410475088, -24.07718906446864793, -32.49135343045505664 ) ) ;
#4500=CARTESIAN_POINT ( 'NONE',  ( 130.8568914410475372, 34.05028731879791337, 0.000000000000000000 ) ) ;
#4504=CARTESIAN_POINT ( 'NONE',  ( 184.8905102610680444, 41.77492675555983936, 14.79361573936436081 ) ) ;
#4505=CARTESIAN_POINT ( 'NONE',  ( 170.2234770963711128, 10.92277846919147066, 45.64576402573197811 ) ) ;
#4506=CARTESIAN_POINT ( 'NONE',  ( 163.1118516004056573, -12.73709011382472234, -2.449293598294708485E-15 ) ) ;
#4507=CARTESIAN_POINT ( 'NONE',  ( 163.1118516004056573, 12.73709011382477918, 40.00000000000002132 ) ) ;
#4508=CARTESIAN_POINT ( 'NONE',  ( 184.8905102610680444, -40.00000000000021316, 20.92133201514402430 ) ) ;
#4509=CARTESIAN_POINT ( 'NONE',  ( -208.1127848780265026, 10.60833733269537049, 10.60833733269544510 ) ) ;
#4511=CARTESIAN_POINT ( 'NONE',  ( 57.59792236341148453, 1.722363176415528940, -54.84617931850878136 ) ) ;
#4512=CARTESIAN_POINT ( 'NONE',  ( -114.4364955367327354, 8.064892380842190178, 20.29001642038852182 ) ) ;
#4514=AXIS2_PLACEMENT_3D ( 'NONE', #15403, #23528, #7161 ) ;
#4515=CARTESIAN_POINT ( 'NONE',  ( -86.96347745069644475, -15.38646221621786125, -15.38646221621789856 ) ) ;
#4517=CARTESIAN_POINT ( 'NONE',  ( 170.0000000000000000, -2.301191124287261779E-13, 24.95097643317000546 ) ) ;
#4521=CARTESIAN_POINT ( 'NONE',  ( -86.96347745069643054, 15.38646221621763210, 41.18208027870604582 ) ) ;
#4522=CARTESIAN_POINT ( 'NONE',  ( -3.966425590329097250, -43.02666064534183477, -23.46521855348083463 ) ) ;
#4524=CARTESIAN_POINT ( 'NONE',  ( -86.96347745069644475, -21.75974354311651737, 0.000000000000000000 ) ) ;
#4525=CARTESIAN_POINT ( 'NONE',  ( -77.78738185796684945, -9.951839775390311615, -19.58912165101554592 ) ) ;
#4530=CARTESIAN_POINT ( 'NONE',  ( 184.8905102610680444, 19.07866798485561333, 40.00000000000002132 ) ) ;
#4534=CARTESIAN_POINT ( 'NONE',  ( 4.995406935893312195, -67.35176059882525124, -10.78321810390210445 ) ) ;
#4535=CARTESIAN_POINT ( 'NONE',  ( -259.2033419157646676, 39.99999999999987210, 30.48217210827754542 ) ) ;
#4536=CARTESIAN_POINT ( 'NONE',  ( 14.38125909742180930, 39.99999999999982947, 55.17850393971022527 ) ) ;
#4537=CARTESIAN_POINT ( 'NONE',  ( 151.7948205124836250, 1.439163438361279259E-13, -33.23291073765553705 ) ) ;
#4538=CARTESIAN_POINT ( 'NONE',  ( 91.82158438592158234, 17.20528682183301683, 0.000000000000000000 ) ) ;
#4539=CARTESIAN_POINT ( 'NONE',  ( 199.9999999999999432, 14.14213562373113398, -14.14213562373094923 ) ) ;
#4540=CARTESIAN_POINT ( 'NONE',  ( -86.96347745069643054, -18.24025645688353947, -40.00000000000002132 ) ) ;
#4542=CARTESIAN_POINT ( 'NONE',  ( -198.0356074513804288, -39.15871834505936278, 39.15871834505892224 ) ) ;
#4543=CARTESIAN_POINT ( 'NONE',  ( 140.2235668266255857, -12.60094438999819744, -30.42137084504307509 ) ) ;
#4544=CARTESIAN_POINT ( 'NONE',  ( -110.0960685945713777, 12.40690815813350412, -15.98210693810259286 ) ) ;
#4545=CARTESIAN_POINT ( 'NONE',  ( 200.0000000000000000, 39.99999999999985079, 20.00000000000052225 ) ) ;
#4546=CARTESIAN_POINT ( 'NONE',  ( 4.995406935893298872, -1.944352046434030652E-13, 55.24977328854835434 ) ) ;
#4547=CARTESIAN_POINT ( 'NONE',  ( 151.7948205124836534, 4.785054706298574878, -51.78348778862537927 ) ) ;
#4548=AXIS2_PLACEMENT_3D ( 'NONE', #15192, #10954, #9203 ) ;
#4550=CARTESIAN_POINT ( 'NONE',  ( -188.2995950289364941, -46.99046209955426434, -13.82811170417247126 ) ) ;
#4551=CARTESIAN_POINT ( 'NONE',  ( 14.38125909742181818, -39.01709431150904095, -17.55144818341490165 ) ) ;
#4552=ORIENTED_EDGE ( 'NONE', *, *, #1929, .T. ) ;
#4553=CARTESIAN_POINT ( 'NONE',  ( -190.1935349183499113, 23.83022391594541745, -43.51927535257637913 ) ) ;
#4555=CARTESIAN_POINT ( 'NONE',  ( 184.8905102610680444, 20.92133201514447194, -40.00000000000002132 ) ) ;
#4556=EDGE_CURVE ( 'NONE', #6926, #11522, #21720, .T. ) ;
#4557=DIRECTION ( 'NONE',  ( -0.01051738777841065495, 0.3656191333258888565, -0.9307051272558590771 ) ) ;
#4558=CARTESIAN_POINT ( 'NONE',  ( -100.7734535825088358, -16.03295912088728770, 16.03295912088687913 ) ) ;
#4559=ORIENTED_EDGE ( 'NONE', *, *, #25346, .T. ) ;
#4560=VERTEX_POINT ( 'NONE', #17432 ) ;
#4562=CARTESIAN_POINT ( 'NONE',  ( 121.8740240556053038, 11.10671848392283145, -26.81399039734612089 ) ) ;
#4563=CARTESIAN_POINT ( 'NONE',  ( 23.38399212876430155, 23.33762193384666261, 42.85408588822703280 ) ) ;
#4566=CARTESIAN_POINT ( 'NONE',  ( -198.0356074513804572, -17.40982414986482141, 39.15871834505909987 ) ) ;
#4568=CARTESIAN_POINT ( 'NONE',  ( -110.0904723790771271, 3.161343376072184075, 19.95170499002183107 ) ) ;
#4569=CARTESIAN_POINT ( 'NONE',  ( -56.48582580120559982, -6.472252184284282173, 50.09629031063965243 ) ) ;
#4570=CARTESIAN_POINT ( 'NONE',  ( 4.995406935893289102, 10.78321810388998081, 10.78321810389001811 ) ) ;
#4572=CARTESIAN_POINT ( 'NONE',  ( -190.0000000000001705, 1.836970198721007106E-15, 0.000000000000000000 ) ) ;
#4573=CARTESIAN_POINT ( 'NONE',  ( -135.8532207217289738, 40.00000000000031974, -30.84685318188603986 ) ) ;
#4574=CARTESIAN_POINT ( 'NONE',  ( -56.48582580120559271, -1.062504017861011783E-13, 9.153146818113587102 ) ) ;
#4575=CARTESIAN_POINT ( 'NONE',  ( -77.55640685876512919, -9.396736996787174904E-14, 22.13135000837103661 ) ) ;
#4578=CARTESIAN_POINT ( 'NONE',  ( -183.1090696430332514, 13.45963186436838477, 45.18841929383249578 ) ) ;
#4579=CARTESIAN_POINT ( 'NONE',  ( 14.38125909742181818, -39.01709431150928253, 17.55144818341435808 ) ) ;
#4581=CARTESIAN_POINT ( 'NONE',  ( 14.38125909742181996, -10.73282306403606157, 67.30136555895948902 ) ) ;
#4583=CARTESIAN_POINT ( 'NONE',  ( -30.26275506840325136, 27.08623969584614244, -29.48230279907770779 ) ) ;
#4585=CARTESIAN_POINT ( 'NONE',  ( 136.1360204305621266, 35.03383547441298163, 40.00000000000002132 ) ) ;
#4586=CARTESIAN_POINT ( 'NONE',  ( -105.3755690713226585, 12.89780903124349720, 43.67073346367994446 ) ) ;
#4587=CARTESIAN_POINT ( 'NONE',  ( -238.4067589809705794, -0.9644942799826262680, 0.000000000000000000 ) ) ;
#4590=CARTESIAN_POINT ( 'NONE',  ( 151.7948205124836534, -39.99999999999992184, -6.767089262349454515 ) ) ;
#4593=EDGE_LOOP ( 'NONE', ( #5480, #4756, #26123, #10064, #24035 ) ) ;
#4595=CARTESIAN_POINT ( 'NONE',  ( 91.82158438592158234, 22.79471317813471742, 40.00000000000002132 ) ) ;
#4598=CARTESIAN_POINT ( 'NONE',  ( 136.1360204305621266, 3.511608612530757068, -3.511608612530642937 ) ) ;
#4599=CARTESIAN_POINT ( 'NONE',  ( -105.2053629887268187, -21.49364769383058160, 0.6703845944188828732 ) ) ;
#4601=CARTESIAN_POINT ( 'NONE',  ( -77.55640685876511498, -22.13135000837103661, -4.964495286674871776E-15 ) ) ;
#4602=DIRECTION ( 'NONE',  ( 1.000000000000000000, 1.836970198721030181E-16, 0.000000000000000000 ) ) ;
#4606=CARTESIAN_POINT ( 'NONE',  ( 91.82158438592158234, -12.16597498399995203, -44.40256751092347542 ) ) ;
#4607=CARTESIAN_POINT ( 'NONE',  ( -208.1127848780265026, -10.60833733269537227, -10.60833733269551793 ) ) ;
#4609=CARTESIAN_POINT ( 'NONE',  ( 184.8905102610680444, 39.99999999999983658, 20.92133201514485563 ) ) ;
#4610=CARTESIAN_POINT ( 'NONE',  ( 146.6084372240433993, 24.48358557860307272, 24.48358557860347418 ) ) ;
#4612=CARTESIAN_POINT ( 'NONE',  ( 192.4448373802100889, -14.14213562375876698, -14.14213562375885047 ) ) ;
#4613=CARTESIAN_POINT ( 'NONE',  ( 14.38125909742183062, -67.30136555898262429, 10.73282306405838682 ) ) ;
#4616=CARTESIAN_POINT ( 'NONE',  ( -192.9588430854690273, 39.99999999999980105, 54.46834944098235809 ) ) ;
#4617=CARTESIAN_POINT ( 'NONE',  ( 22.80622392652934494, 43.16567765897924147, -17.87980911537434636 ) ) ;
#4618=CARTESIAN_POINT ( 'NONE',  ( 199.9999999999999432, -20.00000000000006750, 0.000000000000000000 ) ) ;
#4619=CARTESIAN_POINT ( 'NONE',  ( -100.7734535825088500, -16.03295912088716335, 40.53558337403673306 ) ) ;
#4620=CARTESIAN_POINT ( 'NONE',  ( -198.0356074513804572, 55.37879056871320671, 40.00000000000002132 ) ) ;
#4621=CARTESIAN_POINT ( 'NONE',  ( -40.07203023069898506, -34.25109662817532552, 11.15662918590587260 ) ) ;
#4622=CARTESIAN_POINT ( 'NONE',  ( 130.8568914410475088, -34.05028731879786363, 40.00000000000002132 ) ) ;
#4623=ORIENTED_EDGE ( 'NONE', *, *, #14927, .F. ) ;
#4624=CARTESIAN_POINT ( 'NONE',  ( 85.88462004915263037, -10.32535765023374807, -22.72792989731669167 ) ) ;
#4625=CARTESIAN_POINT ( 'NONE',  ( -198.0356074513804572, -17.40982414986482141, 39.15871834505909987 ) ) ;
#4626=CARTESIAN_POINT ( 'NONE',  ( -8.255580677127136724, -22.62611236876437815, 41.75907689859029404 ) ) ;
#4627=CARTESIAN_POINT ( 'NONE',  ( 8.556015491740193823, 14.17785852676870917, -49.31947911770388515 ) ) ;
#4629=CARTESIAN_POINT ( 'NONE',  ( 184.8905102610680444, -14.79361573936399665, 14.79361573936367158 ) ) ;
#4630=EDGE_CURVE ( 'NONE', #25529, #20449, #14665, .T. ) ;
#4633=CARTESIAN_POINT ( 'NONE',  ( -188.2957210513883979, -13.82790368522451452, 46.98905903629621150 ) ) ;
#4635=CARTESIAN_POINT ( 'NONE',  ( -135.8532207217289738, 6.472252184284096543, 6.472252184284234211 ) ) ;
#4636=CARTESIAN_POINT ( 'NONE',  ( -259.2033419157646676, -6.730120644403663199, 6.730120644403451813 ) ) ;
#4637=CARTESIAN_POINT ( 'NONE',  ( -86.96347745069644475, 15.38646221621772092, 15.38646221621800336 ) ) ;
#4638=CARTESIAN_POINT ( 'NONE',  ( -86.96347745069644475, 15.38646221621772092, 15.38646221621800336 ) ) ;
#4639=CARTESIAN_POINT ( 'NONE',  ( 199.9999999999999432, 14.14213562373110911, -14.14213562373072364 ) ) ;
#4640=CARTESIAN_POINT ( 'NONE',  ( -135.8532207217289738, -6.472252184284280396, 6.472252184284099208 ) ) ;
#4641=CARTESIAN_POINT ( 'NONE',  ( 151.7948205124836250, -6.767089262349004208, -2.449293598294708485E-15 ) ) ;
#4642=CARTESIAN_POINT ( 'NONE',  ( -91.56559293963834989, -22.67402823373193499, -40.00000000000002132 ) ) ;
#4643=CARTESIAN_POINT ( 'NONE',  ( -192.9588430854689989, 1.161019517985663313E-13, -14.46834944099969533 ) ) ;
#4644=CARTESIAN_POINT ( 'NONE',  ( -56.48582580120559982, 21.81201906317778594, -34.75652343174606074 ) ) ;
#4645=CARTESIAN_POINT ( 'NONE',  ( -89.91498783732122035, 20.17141720496151436, -8.733585467785427880 ) ) ;
#4646=CARTESIAN_POINT ( 'NONE',  ( 170.2234770963711128, -10.92277846919187034, -10.92277846919209594 ) ) ;
#4648=ORIENTED_EDGE ( 'NONE', *, *, #7991, .F. ) ;
#4649=CARTESIAN_POINT ( 'NONE',  ( 146.6084372240433709, -24.48358557860329299, 32.08495691632052882 ) ) ;
#4650=CARTESIAN_POINT ( 'NONE',  ( -89.91498783732303934, 8.087768383598069377, 20.43892340003915820 ) ) ;
#4651=CARTESIAN_POINT ( 'NONE',  ( -86.96347745069644475, -12.89780903124413491, 12.89780903124398037 ) ) ;
#4652=CARTESIAN_POINT ( 'NONE',  ( 8.556015491675912799, -44.89939803569713916, -24.84887822172902361 ) ) ;
#4653=ORIENTED_EDGE ( 'NONE', *, *, #2327, .F. ) ;
#4654=CARTESIAN_POINT ( 'NONE',  ( -105.2054292635175443, 15.69192375045724930, 14.70407267694731956 ) ) ;
#4655=CARTESIAN_POINT ( 'NONE',  ( -82.28158521660047597, -9.172166285104129457, -18.01696758243814855 ) ) ;
#4659=CARTESIAN_POINT ( 'NONE',  ( -208.1127848780265026, 55.00245453012668406, 2.449293598294708485E-15 ) ) ;
#4662=B_SPLINE_CURVE_WITH_KNOTS ( 'NONE', 3,
 ( #1352, #3468, #21564, #21692, #25695, #25573 ),
 .UNSPECIFIED., .F., .F.,
 ( 4, 2, 4 ),
 ( 0.000000000000000000, 0.03937794852163882531, 0.07875589704327765062 ),
 .UNSPECIFIED. ) ;
#4663=CARTESIAN_POINT ( 'NONE',  ( 19.06497207195981858, -38.31983398719641087, 18.24870850772724040 ) ) ;
#4664=CARTESIAN_POINT ( 'NONE',  ( 130.8568914410475372, 8.154165912415230659E-16, 5.949712681206690945 ) ) ;
#4665=CARTESIAN_POINT ( 'NONE',  ( 151.7948205124836534, 40.00000000000017053, -33.23291073765538783 ) ) ;
#4667=CARTESIAN_POINT ( 'NONE',  ( 192.4448373802101173, -19.99999999996056843, -40.00000000000002132 ) ) ;
#4668=CARTESIAN_POINT ( 'NONE',  ( 21.80824205441264141, -13.88338701302259715, -47.36272483143062573 ) ) ;
#4669=CARTESIAN_POINT ( 'NONE',  ( -105.3755690713226727, 15.38646221621793231, -15.38646221621779020 ) ) ;
#4670=CARTESIAN_POINT ( 'NONE',  ( -208.1127848780264742, -55.00245453012676222, -2.449293598294708485E-15 ) ) ;
#4671=CARTESIAN_POINT ( 'NONE',  ( 163.1118516004056573, -9.006482792069636645, 9.006482792069567367 ) ) ;
#4672=CARTESIAN_POINT ( 'NONE',  ( 141.7948666911894975, -12.58737617328892888, -30.38861427224631839 ) ) ;
#4673=CARTESIAN_POINT ( 'NONE',  ( -114.6097568999588390, 10.88341597703020547, -19.09891331897681255 ) ) ;
#4674=CARTESIAN_POINT ( 'NONE',  ( 151.7948205124836534, 39.99999999999970157, 33.23291073765595627 ) ) ;
#4675=CARTESIAN_POINT ( 'NONE',  ( -135.8532207217289738, 39.99999999999989342, 30.84685318188660474 ) ) ;
#4678=CARTESIAN_POINT ( 'NONE',  ( 19.06497207195981858, -38.31983398719616218, -18.24870850772777331 ) ) ;
#4680=CARTESIAN_POINT ( 'NONE',  ( 170.2234770963711128, 17.36149277826980253, 17.36149277827007253 ) ) ;
#4681=CARTESIAN_POINT ( 'NONE',  ( 98.29820294267312875, 7.653668647304333383, -18.47759065023115355 ) ) ;
#4682=CARTESIAN_POINT ( 'NONE',  ( 125.5832160019861305, 28.05309928654008900, -11.61997419108379859 ) ) ;
#4683=CARTESIAN_POINT ( 'NONE',  ( 192.4448373802101173, 20.00000000003945644, -40.00000000000002132 ) ) ;
#4685=CARTESIAN_POINT ( 'NONE',  ( -105.2054292635176580, 14.23233549213511573, 16.16366093526940517 ) ) ;
#4686=CARTESIAN_POINT ( 'NONE',  ( 200.0000000000000000, -42.42640687119272513, -14.14213562373140753 ) ) ;
#4689=CARTESIAN_POINT ( 'NONE',  ( -105.4741150117369273, 8.366608964608960974, -19.60045294982168329 ) ) ;
#4690=CARTESIAN_POINT ( 'NONE',  ( -102.4294859495706049, 8.407280617849425042, -20.29697089045613012 ) ) ;
#4691=ADVANCED_FACE ( 'NONE', ( #17815 ), #23941, .T. ) ;
#4692=CARTESIAN_POINT ( 'NONE',  ( 22.78333232258906094, 17.88247728649375645, 43.17211919388270758 ) ) ;
#4695=CARTESIAN_POINT ( 'NONE',  ( 14.38125909742181285, -17.55144818341476309, 39.01709431150910490 ) ) ;
#4697=CARTESIAN_POINT ( 'NONE',  ( -114.6659165473969040, -4.804252803496178892, 21.50057250525394181 ) ) ;
#4698=CARTESIAN_POINT ( 'NONE',  ( 146.6084372240433709, -24.48358557860329299, 32.08495691632052882 ) ) ;
#4699=CARTESIAN_POINT ( 'NONE',  ( 184.8905102610680444, -14.79361573936379415, -14.79361573936387941 ) ) ;
#4700=CARTESIAN_POINT ( 'NONE',  ( 151.7948205124836534, 40.00000000000002842, 6.767089262349174739 ) ) ;
#4701=CARTESIAN_POINT ( 'NONE',  ( -199.9999999999999716, -18.14835560307974660, 46.41341197396111795 ) ) ;
#4703=CARTESIAN_POINT ( 'NONE',  ( -88.37877758191619648, -8.575405934157467769, -19.92653024494341807 ) ) ;
#4705=ADVANCED_FACE ( 'NONE', ( #17949 ), #22095, .F. ) ;
#4706=CARTESIAN_POINT ( 'NONE',  ( -86.96347745069644475, 1.775309070576523494E-13, -18.24025645688352881 ) ) ;
#4707=CARTESIAN_POINT ( 'NONE',  ( -86.96347745069644475, -2.438961472018186339E-13, 21.75974354311649961 ) ) ;
#4709=CARTESIAN_POINT ( 'NONE',  ( -87.13361725327072804, -21.49321519333431141, -3.542586001259484843E-15 ) ) ;
#4711=CARTESIAN_POINT ( 'NONE',  ( -188.9524464571000522, 23.58788642769107469, 43.19209889639545707 ) ) ;
#4712=CARTESIAN_POINT ( 'NONE',  ( 184.8905102610680444, -41.77492675556007384, 14.79361573936348684 ) ) ;
#4713=CARTESIAN_POINT ( 'NONE',  ( -94.58366989427474891, 9.000605044545403999, 20.58370269626844618 ) ) ;
#4714=CARTESIAN_POINT ( 'NONE',  ( -198.0356074513804572, -10.87444709760996986, 67.44298959253333692 ) ) ;
#4716=CARTESIAN_POINT ( 'NONE',  ( 200.0000000000000000, 42.42640687119310172, -14.14213562373052646 ) ) ;
#4718=DIRECTION ( 'NONE',  ( -7.401486830834374307E-15, 0.9307566067077635008, -0.3656393565657962141 ) ) ;
#4719=CARTESIAN_POINT ( 'NONE',  ( -208.1127848780264742, 38.89260858015707356, 17.67593391476696141 ) ) ;
#4720=CARTESIAN_POINT ( 'NONE',  ( -280.0000000000000000, 19.99999999999996092, -0.000000000000000000 ) ) ;
#4721=DIRECTION ( 'NONE',  ( 0.9698969544411717436, -0.09318942518908124306, 0.2249791741443379622 ) ) ;
#4722=ORIENTED_EDGE ( 'NONE', *, *, #11245, .F. ) ;
#4723=CARTESIAN_POINT ( 'NONE',  ( 163.1118516004056573, -39.99999999999986500, -12.73709011382517353 ) ) ;
#4726=VERTEX_POINT ( 'NONE', #5855 ) ;
#4727=VERTEX_POINT ( 'NONE', #13442 ) ;
#4728=CARTESIAN_POINT ( 'NONE',  ( 91.82158438592158234, 22.79471317813472098, 2.449293598294708485E-15 ) ) ;
#4729=CARTESIAN_POINT ( 'NONE',  ( -102.4309680866828671, -20.43798635329655866, -8.087567261865729051 ) ) ;
#4730=CARTESIAN_POINT ( 'NONE',  ( -114.6097568999414733, -21.20070836099096923, -5.809233881233475394 ) ) ;
#4732=CARTESIAN_POINT ( 'NONE',  ( 91.82158438592159655, -39.99999999999994316, -17.20528682183314118 ) ) ;
#4736=CIRCLE ( 'NONE', #5992, 15.00000000000000533 ) ;
#4737=CARTESIAN_POINT ( 'NONE',  ( 130.8568914410475088, -24.07718906446864793, -32.49135343045505664 ) ) ;
#4738=CARTESIAN_POINT ( 'NONE',  ( -162.0762913951020892, -1.198031840385767266, -1.198031840385758384 ) ) ;
#4740=SPHERICAL_SURFACE ( 'NONE', #23344, 15.00000000000000000 ) ;
#4741=CARTESIAN_POINT ( 'NONE',  ( 136.1360204305621266, -3.419521671106983309E-13, 35.03383547441296741 ) ) ;
#4742=CARTESIAN_POINT ( 'NONE',  ( 192.4448373802100889, 14.14213562375873678, 14.14213562375894817 ) ) ;
#4743=CARTESIAN_POINT ( 'NONE',  ( 21.99343714674520811, 13.87412077874984462, 47.30053030063388064 ) ) ;
#4744=CARTESIAN_POINT ( 'NONE',  ( 184.8905102610680444, -14.79361573936389540, 41.77492675555996016 ) ) ;
#4745=CARTESIAN_POINT ( 'NONE',  ( 151.7948205124836250, -4.785054706301671068, 4.785054706301645311 ) ) ;
#4748=CARTESIAN_POINT ( 'NONE',  ( 0.2972598230769883387, 39.99999999999997158, 14.33493731733947563 ) ) ;
#4750=CARTESIAN_POINT ( 'NONE',  ( -86.96347745069644475, -43.67073346367983788, 12.89780903124397149 ) ) ;
#4751=CARTESIAN_POINT ( 'NONE',  ( 163.1118516004056573, -27.26290988616869626, 40.00000000000002132 ) ) ;
#4753=CARTESIAN_POINT ( 'NONE',  ( 8.209392600955618846, -49.31072049266142443, 14.17653494425346672 ) ) ;
#4754=CIRCLE ( 'NONE', #11964, 14.99999999999999822 ) ;
#4755=CARTESIAN_POINT ( 'NONE',  ( -135.8532207217289738, 30.84685318188643421, 40.00000000000002132 ) ) ;
#4756=ORIENTED_EDGE ( 'NONE', *, *, #8977, .T. ) ;
#4758=AXIS2_PLACEMENT_3D ( 'NONE', #21726, #24121, #17720 ) ;
#4759=CARTESIAN_POINT ( 'NONE',  ( -91.56559293963834989, -16.03295912088706388, -16.03295912088710651 ) ) ;
#4760=CARTESIAN_POINT ( 'NONE',  ( -6.754359963543765666, -17.56548336386596532, 42.40682816667121102 ) ) ;
#4762=CARTESIAN_POINT ( 'NONE',  ( 4.155455573169746231, 18.49472242011614398, -44.65020969900606218 ) ) ;
#4764=CARTESIAN_POINT ( 'NONE',  ( 151.7948205124836534, 4.785054706297857230, 51.78348778862544322 ) ) ;
#4765=CARTESIAN_POINT ( 'NONE',  ( -86.95450734974414786, -20.33657406931063605, 6.704150134019479346 ) ) ;
#4767=CARTESIAN_POINT ( 'NONE',  ( -191.2490444017190327, -18.16428715637485780, 43.85246840377622846 ) ) ;
#4768=CARTESIAN_POINT ( 'NONE',  ( -213.1075012329537230, 18.58567234101174037, -37.98287015391222354 ) ) ;
#4769=CARTESIAN_POINT ( 'NONE',  ( 14.38125909742180752, 17.55144818341448953, 39.01709431150923280 ) ) ;
#4770=CARTESIAN_POINT ( 'NONE',  ( -56.48582580120559982, -6.472252184283581400, -50.09629031063973059 ) ) ;
#4771=CARTESIAN_POINT ( 'NONE',  ( -238.4067589809705794, -0.6820004457913585449, -0.6820004457913265705 ) ) ;
#4773=CARTESIAN_POINT ( 'NONE',  ( -280.0000000000000000, 14.14213562373078581, 14.14213562373108424 ) ) ;
#4774=CARTESIAN_POINT ( 'NONE',  ( -198.0356074513804572, 39.15871834505956173, -39.15871834505865223 ) ) ;
#4775=CARTESIAN_POINT ( 'NONE',  ( -192.9588430854690273, 66.79921049724377724, -10.23066800231904239 ) ) ;
#4776=CARTESIAN_POINT ( 'NONE',  ( 184.8905102610680444, 20.92133201514447194, 40.00000000000002132 ) ) ;
#4777=CARTESIAN_POINT ( 'NONE',  ( 151.7948205124836534, -33.23291073765550863, -40.00000000000002132 ) ) ;
#4778=CARTESIAN_POINT ( 'NONE',  ( 184.8905102610680444, 41.77492675556005253, -14.79361573936377461 ) ) ;
#4781=CARTESIAN_POINT ( 'NONE',  ( 200.0000000000000000, -42.42640687119290988, 14.14213562373064903 ) ) ;
#4783=CARTESIAN_POINT ( 'NONE',  ( -121.8281105901294978, 23.07023229646648943, -8.694016235322095554 ) ) ;
#4785=CARTESIAN_POINT ( 'NONE',  ( -30.26275506840324070, 1.198031551615912571, 57.76657404653985139 ) ) ;
#4786=CARTESIAN_POINT ( 'NONE',  ( -102.4068193528165835, -20.44188272012828023, -8.088405365068805253 ) ) ;
#4787=CARTESIAN_POINT ( 'NONE',  ( -280.0000000000000568, 14.14213562373067745, 42.42640687119295251 ) ) ;
#4788=CARTESIAN_POINT ( 'NONE',  ( 9.345847406389310663, -44.90706793518258877, -24.85453859512280417 ) ) ;
#4792=CARTESIAN_POINT ( 'NONE',  ( -30.26275506840324070, 1.694272468446254232, 0.000000000000000000 ) ) ;
#4793=CARTESIAN_POINT ( 'NONE',  ( -114.7826396786174001, -14.66973228884550373, -16.62872306281069257 ) ) ;
#4797=CARTESIAN_POINT ( 'NONE',  ( -213.1075012329537230, 53.71589010950162191, -40.00000000000002132 ) ) ;
#4798=CARTESIAN_POINT ( 'NONE',  ( -108.4672927838138605, 19.20738496773866544, 7.955959351357155818 ) ) ;
#4800=CARTESIAN_POINT ( 'NONE',  ( -208.1127848780264742, -67.17687982760682530, -10.60833733268364298 ) ) ;
#4801=CARTESIAN_POINT ( 'NONE',  ( -86.96347745069644475, -8.210974027862429531E-14, 18.24025645688352881 ) ) ;
#4802=CARTESIAN_POINT ( 'NONE',  ( 136.1360204305621551, 40.00000000000002842, 4.966164525587208445 ) ) ;
#4804=CARTESIAN_POINT ( 'NONE',  ( 192.4448373802101173, 20.00000000003945644, -40.00000000000002132 ) ) ;
#4805=CARTESIAN_POINT ( 'NONE',  ( 22.13784119383913662, -17.95298715833818193, -43.34234508276890807 ) ) ;
#4807=CARTESIAN_POINT ( 'NONE',  ( 192.4448373802100889, -19.99999999996057198, -2.449293598294708485E-15 ) ) ;
#4808=CARTESIAN_POINT ( 'NONE',  ( 19.06497207195981147, -10.03556273973439517, 10.03556273973429214 ) ) ;
#4809=CARTESIAN_POINT ( 'NONE',  ( -100.7734535825088358, -2.560096224687585342E-13, 22.67402823373191723 ) ) ;
#4810=CARTESIAN_POINT ( 'NONE',  ( -105.3846709044788810, 19.12138504417525198, -9.637707283830140526 ) ) ;
#4811=CARTESIAN_POINT ( 'NONE',  ( -198.0356074513804572, 5.461327841961909642E-13, -55.37879056873073580 ) ) ;
#4812=CARTESIAN_POINT ( 'NONE',  ( 151.7948205124836250, -23.49921654116339553, -23.49921654116350211 ) ) ;
#4815=CARTESIAN_POINT ( 'NONE',  ( 0.2972598230770153171, -66.70487387989861361, 10.13633138497438324 ) ) ;
#4816=ORIENTED_EDGE ( 'NONE', *, *, #5570, .F. ) ;
#4817=CARTESIAN_POINT ( 'NONE',  ( -77.78673448795173329, 6.807559357124845612, -20.89197888679335691 ) ) ;
#4818=CARTESIAN_POINT ( 'NONE',  ( -16.78454218927527108, 39.63790004360789965, -16.41855578212769728 ) ) ;
#4819=DIRECTION ( 'NONE',  ( 0.9352143323239582307, 0.1355013636775663222, -0.3271292299036774320 ) ) ;
#4820=CARTESIAN_POINT ( 'NONE',  ( 0.2972598230770129857, -54.33493731733936016, -40.00000000000002132 ) ) ;
#4821=CARTESIAN_POINT ( 'NONE',  ( -114.6382724355127607, 18.98542650371850016, -11.21026131167359807 ) ) ;
#4822=CARTESIAN_POINT ( 'NONE',  ( -86.96347745069644475, -15.38646221621807442, 15.38646221621768184 ) ) ;
#4823=ORIENTED_EDGE ( 'NONE', *, *, #8977, .F. ) ;
#4825=CARTESIAN_POINT ( 'NONE',  ( 23.37394308801976450, 46.80823611210215063, -13.80096434448263309 ) ) ;
#4828=CARTESIAN_POINT ( 'NONE',  ( -259.2033419157646676, -35.01439189186554302, 21.55415060305832498 ) ) ;
#4830=CARTESIAN_POINT ( 'NONE',  ( -105.3841230195786096, -19.11845054111881481, -9.645493323979394518 ) ) ;
#4831=CARTESIAN_POINT ( 'NONE',  ( -162.0762913951021176, -27.08623940707624911, 29.48230308784761888 ) ) ;
#4832=CARTESIAN_POINT ( 'NONE',  ( 151.7948205124836250, -23.49921654116339553, -23.49921654116350211 ) ) ;
#4833=CARTESIAN_POINT ( 'NONE',  ( -135.8532207217289738, 39.99999999999989342, 30.84685318188660474 ) ) ;
#4835=CARTESIAN_POINT ( 'NONE',  ( -199.9999999999999432, 14.17215463606929227, 49.28189405767592746 ) ) ;
#4836=CARTESIAN_POINT ( 'NONE',  ( 136.1360204305621551, -40.00000000000036238, 35.03383547441254109 ) ) ;
#4837=CARTESIAN_POINT ( 'NONE',  ( 184.8905102610680444, -1.851754852062639767E-13, 20.92133201514444352 ) ) ;
#4838=CARTESIAN_POINT ( 'NONE',  ( -82.23726319249648498, 14.28014421912408061, 14.28014421912424226 ) ) ;
#4841=CARTESIAN_POINT ( 'NONE',  ( -188.2956751479549098, 23.44846780264100872, 43.00407324591984093 ) ) ;
#4842=CARTESIAN_POINT ( 'NONE',  ( 19.06497207195981147, -10.03556273973425483, -10.03556273973443247 ) ) ;
#4844=CARTESIAN_POINT ( 'NONE',  ( -100.7734535825088500, 44.31723036834890905, 12.25131212657507795 ) ) ;
#4845=CARTESIAN_POINT ( 'NONE',  ( -87.01506749147795006, -18.46228859040754955, 10.84947533659219943 ) ) ;
#4846=CARTESIAN_POINT ( 'NONE',  ( 57.59792236341147031, 30.00663442387720181, -26.56190807104661289 ) ) ;
#4848=CARTESIAN_POINT ( 'NONE',  ( -192.9588430854690273, -14.46834944099973264, 40.00000000000002132 ) ) ;
#4849=B_SPLINE_CURVE_WITH_KNOTS ( 'NONE', 3,
 ( #24970, #6717, #12978, #14968, #2471, #16964, #20705, #10723, #8991, #10452, #2338, #24697, #12707, #8586, #6453, #12439, #23103, #15094, #24830, #2610, #4743, #16698, #6583, #10851, #18833, #14831 ),
 .UNSPECIFIED., .F., .F.,
 ( 4, 2, 1, 2, 2, 2, 2, 2, 2, 2, 2, 1, 2, 4 ),
 ( -5.999999999144898528E-08, 0.0004354487530732512827, 0.0008709575061464940775, 0.001741975012292979559, 0.003484010024585944883, 0.006968080049171870329, 0.01045215007375779707, 0.01393622009834372295, 0.02090436014751557645, 0.02438843017210149886, 0.02613046518439446353, 0.02700148269054095107, 0.02743699144361419484, 0.02787250019668744208 ),
 .UNSPECIFIED. ) ;
#4850=CARTESIAN_POINT ( 'NONE',  ( 163.1118516004056573, 9.006482792073693844, 47.56205970284970164 ) ) ;
#4851=CARTESIAN_POINT ( 'NONE',  ( 0.2972598230769983307, -14.33493731733933352, 40.00000000000002132 ) ) ;
#4853=EDGE_LOOP ( 'NONE', ( #4992, #22520, #1464, #4722 ) ) ;
#4854=CARTESIAN_POINT ( 'NONE',  ( 14.38125909742182529, -39.99999999999944578, -55.17850393971050238 ) ) ;
#4858=ORIENTED_EDGE ( 'NONE', *, *, #15559, .T. ) ;
#4860=CARTESIAN_POINT ( 'NONE',  ( 0.2972598230769930572, 54.33493731733936016, 2.449293598294708485E-15 ) ) ;
#4864=CARTESIAN_POINT ( 'NONE',  ( -110.0737093975827747, -19.58505513374902662, 5.042781230409048021 ) ) ;
#4865=DIRECTION ( 'NONE',  ( -0.2259624730540135129, 0.000000000000000000, -0.9741360073271668751 ) ) ;
#4866=CARTESIAN_POINT ( 'NONE',  ( -192.9588430854690273, -40.00000000000011369, 14.46834944099955855 ) ) ;
#4869=CARTESIAN_POINT ( 'NONE',  ( -30.26275506840324070, -27.08623969584554558, -29.48230279907826912 ) ) ;
#4870=CARTESIAN_POINT ( 'NONE',  ( -192.9588430854689989, -10.23066800230742501, -10.23066800230756712 ) ) ;
#4871=CARTESIAN_POINT ( 'NONE',  ( -114.6380801921741011, -18.98799529646051454, -11.20622827607009597 ) ) ;
#4872=CARTESIAN_POINT ( 'NONE',  ( 4.995406935893306866, -39.99999999999944578, -55.24977328856505920 ) ) ;
#4873=CARTESIAN_POINT ( 'NONE',  ( -97.72675010090193837, -8.185591577777461936, 20.89622088363365648 ) ) ;
#4876=CARTESIAN_POINT ( 'NONE',  ( -162.0762913951020607, -1.198031840455708430, 57.76657433537920383 ) ) ;
#4879=CARTESIAN_POINT ( 'NONE',  ( 200.0000000000000000, 40.00000000000012790, -19.99999999999996092 ) ) ;
#4881=CARTESIAN_POINT ( 'NONE',  ( 57.59792236341147031, -1.722363176415123043, 54.84617931850879557 ) ) ;
#4882=CARTESIAN_POINT ( 'NONE',  ( -208.1127848780264742, 15.00245453012665742, 40.00000000000002132 ) ) ;
#4883=EDGE_LOOP ( 'NONE', ( #14685, #25180, #18872, #7123 ) ) ;
#4884=CARTESIAN_POINT ( 'NONE',  ( 20.69615274311347974, -43.59383154590178577, 23.88537831998399241 ) ) ;
#4885=CARTESIAN_POINT ( 'NONE',  ( -56.48582580120559982, -9.153146818113595984, -40.00000000000002132 ) ) ;
#4886=CARTESIAN_POINT ( 'NONE',  ( 170.0000000000000284, -24.95097643316995928, -3.062538285713102937 ) ) ;
#4887=CARTESIAN_POINT ( 'NONE',  ( -213.1075012329537230, 37.98287015391228749, 37.98287015391245802 ) ) ;
#4888=CARTESIAN_POINT ( 'NONE',  ( 19.06497207195981858, -40.00000000000007105, 14.19242893257826665 ) ) ;
#4889=CARTESIAN_POINT ( 'NONE',  ( -77.59213678343638776, 21.93717451302018517, 2.696620339532176835 ) ) ;
#4890=CARTESIAN_POINT ( 'NONE',  ( 14.32711937312299355, -14.14294248749784089, -49.08922911798412514 ) ) ;
#4892=B_SPLINE_CURVE_WITH_KNOTS ( 'NONE', 3,
 ( #17968, #11993, #10266, #15975, #9998, #24511 ),
 .UNSPECIFIED., .F., .F.,
 ( 4, 2, 4 ),
 ( -0.0001324603514674868305, 0.04003846212280023908, 0.08020938459706797308 ),
 .UNSPECIFIED. ) ;
#4893=CARTESIAN_POINT ( 'NONE',  ( -280.0000000000000568, 14.14213562373038968, 42.42640687119305198 ) ) ;
#4896=CARTESIAN_POINT ( 'NONE',  ( -188.4265466358232572, -23.47687925214823323, 43.04237830659958064 ) ) ;
#4897=CARTESIAN_POINT ( 'NONE',  ( -30.26275506840324070, 1.218738420030236455E-14, -1.694272468446259783 ) ) ;
#4898=CARTESIAN_POINT ( 'NONE',  ( -86.96347745069644475, 15.38646221621793586, -15.38646221621778842 ) ) ;
#4899=CARTESIAN_POINT ( 'NONE',  ( -213.1075012329537230, -18.58567234101102272, -37.98287015391260013 ) ) ;
#4900=CARTESIAN_POINT ( 'NONE',  ( -200.0000000000000000, 6.162975822039154730E-30, 0.000000000000000000 ) ) ;
#4901=CARTESIAN_POINT ( 'NONE',  ( -30.26275506840325136, 27.08623969584614244, -29.48230279907770779 ) ) ;
#4902=CARTESIAN_POINT ( 'NONE',  ( -198.0356074513804572, 67.44298959250878056, -10.87444709758402261 ) ) ;
#4903=CARTESIAN_POINT ( 'NONE',  ( -259.2033419157646676, -6.730120644402966867, -49.83842185052038332 ) ) ;
#4904=CARTESIAN_POINT ( 'NONE',  ( 184.8905102610680444, 19.07866798485562398, -40.00000000000002132 ) ) ;
#4905=CARTESIAN_POINT ( 'NONE',  ( 19.06497207195979726, 38.31983398719629719, -18.24870850772750686 ) ) ;
#4907=CARTESIAN_POINT ( 'NONE',  ( 14.38125909742181818, -39.01709431150928253, 17.55144818341435808 ) ) ;
#4908=CARTESIAN_POINT ( 'NONE',  ( -188.2870673237559060, 46.98612534495561022, -13.82722856953786206 ) ) ;
#4910=CARTESIAN_POINT ( 'NONE',  ( -280.0000000000000000, 14.14213562373088351, 14.14213562373098654 ) ) ;
#4911=CARTESIAN_POINT ( 'NONE',  ( -96.93773665438899911, -20.92028269119435180, -8.190703376740806618 ) ) ;
#4912=CARTESIAN_POINT ( 'NONE',  ( 4.995406935893301537, -10.78321810390187530, 67.35176059882529387 ) ) ;
#4915=CARTESIAN_POINT ( 'NONE',  ( -183.6284948307073819, -41.87131864454406127, 17.34366805704014780 ) ) ;
#4917=CARTESIAN_POINT ( 'NONE',  ( 0.4226707250629899715, 14.03458789212690938, -48.37218667320253473 ) ) ;
#4919=CARTESIAN_POINT ( 'NONE',  ( 184.8905102610680444, 19.07866798485562043, 2.449293598294708485E-15 ) ) ;
#4920=CARTESIAN_POINT ( 'NONE',  ( 35.93739820626764470, 38.99308227184688036, -20.78453043603687433 ) ) ;
#4924=CARTESIAN_POINT ( 'NONE',  ( 192.4448373802101173, -14.14213562370342281, 42.42640687122062104 ) ) ;
#4925=CARTESIAN_POINT ( 'NONE',  ( -30.26275506840323359, -40.00000000000017053, 41.69427246844613677 ) ) ;
#4926=CARTESIAN_POINT ( 'NONE',  ( -56.48582580120559982, 39.99999999999990763, 30.84685318188658698 ) ) ;
#4927=DIRECTION ( 'NONE',  ( -1.000000000000000000, -1.836970198721030181E-16, -0.000000000000000000 ) ) ;
#4928=CARTESIAN_POINT ( 'NONE',  ( 200.0000000000000000, 20.00000000000013856, -40.00000000000002132 ) ) ;
#4929=CARTESIAN_POINT ( 'NONE',  ( 23.26364522860123785, -23.36474233297011338, -42.89098160628034151 ) ) ;
#4931=EDGE_CURVE ( 'NONE', #16948, #15141, #22345, .T. ) ;
#4932=CARTESIAN_POINT ( 'NONE',  ( -192.9588430854690273, -14.46834944099973264, 40.00000000000002132 ) ) ;
#4933=EDGE_CURVE ( 'NONE', #4362, #18547, #12126, .T. ) ;
#4935=CARTESIAN_POINT ( 'NONE',  ( 91.82158438592158234, 12.16597498397773869, -12.16597498397759303 ) ) ;
#4938=CARTESIAN_POINT ( 'NONE',  ( -105.3755690713226585, 39.99999999999977263, 21.75974354311691883 ) ) ;
#4939=CARTESIAN_POINT ( 'NONE',  ( -105.2053629887423796, 15.67233752942116176, -14.72427054405869917 ) ) ;
#4940=CARTESIAN_POINT ( 'NONE',  ( -105.3755690713226585, -40.00000000000027711, 21.75974354311608749 ) ) ;
#4942=CARTESIAN_POINT ( 'NONE',  ( -65.65550967573157948, -24.04430752632008961, 11.16467289560384835 ) ) ;
#4944=CARTESIAN_POINT ( 'NONE',  ( -30.26275506840325136, 27.08623969584573388, 29.48230279907808793 ) ) ;
#4945=EDGE_LOOP ( 'NONE', ( #23397, #466, #21424, #17582, #15581, #26118 ) ) ;
#4946=CARTESIAN_POINT ( 'NONE',  ( 57.59792236341147031, 1.722363176415040886, 1.722363176415060426 ) ) ;
#4947=CARTESIAN_POINT ( 'NONE',  ( -199.9999999999998010, 24.82633483071100500, -44.86878812508844305 ) ) ;
#4948=CARTESIAN_POINT ( 'NONE',  ( 164.1122551457365262, 24.38379312608506666, -10.10009781492404635 ) ) ;
#4949=CARTESIAN_POINT ( 'NONE',  ( 151.7948205124836250, -6.767089262349004208, -2.449293598294708485E-15 ) ) ;
#4951=CARTESIAN_POINT ( 'NONE',  ( -114.7826396787321954, 1.398624481943209208, -22.13135001986790940 ) ) ;
#4953=ORIENTED_EDGE ( 'NONE', *, *, #21445, .F. ) ;
#4954=AXIS2_PLACEMENT_3D ( 'NONE', #21453, #21333, #23575 ) ;
#4956=CARTESIAN_POINT ( 'NONE',  ( -93.01741312767317993, 8.169811846188826721, -20.82169463882216576 ) ) ;
#4960=CARTESIAN_POINT ( 'NONE',  ( -114.5444905533463356, -6.798574478255778430, 20.85462941671082859 ) ) ;
#4962=CARTESIAN_POINT ( 'NONE',  ( -135.8532207217289738, -34.75652343174615311, 21.81201906317767936 ) ) ;
#4963=CARTESIAN_POINT ( 'NONE',  ( -105.4415978763232147, 19.97871834610316455, 7.511821620885758222 ) ) ;
#4964=CARTESIAN_POINT ( 'NONE',  ( -280.0000000000000568, 40.00000000000004263, -19.99999999999987210 ) ) ;
#4967=CARTESIAN_POINT ( 'NONE',  ( -198.0356074513804572, -39.99999999999948130, -55.37879056874863437 ) ) ;
#4968=CARTESIAN_POINT ( 'NONE',  ( -208.1127848780265026, 5.403397259664334602E-13, -55.00245453012672670 ) ) ;
#4969=CARTESIAN_POINT ( 'NONE',  ( -114.6375327213470143, -18.99176668987167105, 11.19832436705239687 ) ) ;
#4974=CARTESIAN_POINT ( 'NONE',  ( -192.9588430854689989, -10.23066800230756890, 10.23066800230742501 ) ) ;
#4975=CARTESIAN_POINT ( 'NONE',  ( 130.8568914410475372, 24.07718906447210472, 24.07718906447249907 ) ) ;
#4976=CARTESIAN_POINT ( 'NONE',  ( -188.2995950289364941, -46.99046209955528042, 13.82811170417144453 ) ) ;
#4977=CARTESIAN_POINT ( 'NONE',  ( -30.26275506840324070, -1.198031551616032919, 1.198031551616014712 ) ) ;
#4978=CARTESIAN_POINT ( 'NONE',  ( -86.86493150571111244, -8.366608963953618527, 19.60045294882771572 ) ) ;
#4979=CARTESIAN_POINT ( 'NONE',  ( 163.1118516004056573, -9.006482792069506971, -9.006482792069697041 ) ) ;
#4980=CARTESIAN_POINT ( 'NONE',  ( -184.9730489281237737, -13.59277546675971671, -45.83721239347640619 ) ) ;
#4983=CARTESIAN_POINT ( 'NONE',  ( 130.8568914410475088, 4.207082182989012153, 52.36146031193425188 ) ) ;
#4984=CARTESIAN_POINT ( 'NONE',  ( -199.9999999999999432, 43.68705981750494516, 18.09577267661451927 ) ) ;
#4988=CARTESIAN_POINT ( 'NONE',  ( 146.6084372240433993, 8.568076647504290689E-14, -5.374981219216972583 ) ) ;
#4990=CARTESIAN_POINT ( 'NONE',  ( 199.9999999999999432, -20.00000000000006750, 0.000000000000000000 ) ) ;
#4992=ORIENTED_EDGE ( 'NONE', *, *, #22984, .T. ) ;
#4993=ORIENTED_EDGE ( 'NONE', *, *, #14820, .T. ) ;
#4994=CARTESIAN_POINT ( 'NONE',  ( 146.6084372240433993, 5.374981219216999229, 2.449293598294708485E-15 ) ) ;
#4998=CARTESIAN_POINT ( 'NONE',  ( -91.56559293963834989, -39.99999999999995737, -22.67402823373205933 ) ) ;
#5001=CARTESIAN_POINT ( 'NONE',  ( 0.2972598230769938343, 10.13633138497486286, -10.13633138497461594 ) ) ;
#5002=CARTESIAN_POINT ( 'NONE',  ( 91.82158438592156813, -16.11829626348459144, 40.45024623143943643 ) ) ;
#5003=CARTESIAN_POINT ( 'NONE',  ( -114.7544849857915636, -17.49519532552859857, -13.58498122706649447 ) ) ;
#5004=CARTESIAN_POINT ( 'NONE',  ( 14.38125909742181818, 5.830552384690105017E-13, -55.17850393972636880 ) ) ;
#5005=CARTESIAN_POINT ( 'NONE',  ( -162.0762913951020892, -1.198031840385767266, -1.198031840385758384 ) ) ;
#5006=CARTESIAN_POINT ( 'NONE',  ( 91.82158438592156813, 17.20528682183302038, -40.00000000000002132 ) ) ;
#5007=CARTESIAN_POINT ( 'NONE',  ( -100.7734535825088358, -12.25131212657493052, 12.25131212657478130 ) ) ;
#5010=CARTESIAN_POINT ( 'NONE',  ( 136.1360204305621266, 1.473277640373554421E-13, -35.03383547441296741 ) ) ;
#5011=CARTESIAN_POINT ( 'NONE',  ( 146.6084372240433993, -34.62501878078303008, 0.000000000000000000 ) ) ;
#5012=CARTESIAN_POINT ( 'NONE',  ( 184.8905102610680444, -14.79361573936379415, -14.79361573936387941 ) ) ;
#5013=CARTESIAN_POINT ( 'NONE',  ( 14.38125909742180752, 15.17850393972634038, 0.000000000000000000 ) ) ;
#5015=CARTESIAN_POINT ( 'NONE',  ( 21.80824205438601382, -47.36272483143281420, 13.88338701303066713 ) ) ;
#5016=CARTESIAN_POINT ( 'NONE',  ( -30.26275506840324425, 1.694272468446254232, -40.00000000000002132 ) ) ;
#5019=CARTESIAN_POINT ( 'NONE',  ( 192.4448373802101173, -14.14213562375886291, 42.42640687116498555 ) ) ;
#5021=CARTESIAN_POINT ( 'NONE',  ( -87.13238242893044116, 21.48515709343678282, 0.8941846428760004128 ) ) ;
#5024=CARTESIAN_POINT ( 'NONE',  ( 14.38125909742180220, 39.01709431150892016, 17.55144818341517166 ) ) ;
#5027=CARTESIAN_POINT ( 'NONE',  ( -280.0000000000000000, 14.14213562373098299, -14.14213562373088706 ) ) ;
#5028=CARTESIAN_POINT ( 'NONE',  ( 151.7948205124836250, 23.49921654116328540, 23.49921654116366554 ) ) ;
#5030=CARTESIAN_POINT ( 'NONE',  ( -135.8532207217289738, 6.472252184284186249, -6.472252184284142729 ) ) ;
#5032=DIRECTION ( 'NONE',  ( 0.000000000000000000, 1.000000000000000000, 0.000000000000000000 ) ) ;
#5033=CARTESIAN_POINT ( 'NONE',  ( 151.7948205124836250, 23.49921654116328540, 23.49921654116366554 ) ) ;
#5034=CARTESIAN_POINT ( 'NONE',  ( 130.8568914410475088, 32.49135343045448820, 24.07718906446946860 ) ) ;
#5035=CARTESIAN_POINT ( 'NONE',  ( 4.995406935893286438, 67.35176059880245703, -10.78321810387767066 ) ) ;
#5036=CARTESIAN_POINT ( 'NONE',  ( 4.995406935893288214, 15.24977328854832770, -40.00000000000002132 ) ) ;
#5037=CARTESIAN_POINT ( 'NONE',  ( -135.8532207217289738, -6.472252184284190690, -6.472252184284188914 ) ) ;
#5038=( BOUNDED_CURVE ( )  B_SPLINE_CURVE ( 3, ( #25463, #15579, #13215, #15206 ),
 .UNSPECIFIED., .F., .F. ) 
 B_SPLINE_CURVE_WITH_KNOTS ( ( 4, 4 ),
 ( 0.01388163287021914639, 0.02359082919309998458 ),
 .UNSPECIFIED. ) 
 CURVE ( )  GEOMETRIC_REPRESENTATION_ITEM ( )  RATIONAL_B_SPLINE_CURVE ( ( 1.000000000000000000, 0.8672072324488988571, 0.7608653435686189015, 0.6809743333591601333 ) ) 
 REPRESENTATION_ITEM ( '' )  );
#5039=CARTESIAN_POINT ( 'NONE',  ( -208.1127848780265026, -9.061048840815752106E-14, 15.00245453012669472 ) ) ;
#5040=CARTESIAN_POINT ( 'NONE',  ( -86.96347745069643054, -41.18208027870611687, 15.38646221621750954 ) ) ;
#5041=CARTESIAN_POINT ( 'NONE',  ( -188.2652133075324343, 42.99509596150244306, -23.44262061655331308 ) ) ;
#5042=ORIENTED_EDGE ( 'NONE', *, *, #15894, .T. ) ;
#5043=CARTESIAN_POINT ( 'NONE',  ( -30.26275506840323715, 29.48230279907789253, 29.48230279907799556 ) ) ;
#5045=CARTESIAN_POINT ( 'NONE',  ( -24.53392603776244485, -36.88304647107583634, -19.42583462365220015 ) ) ;
#5047=CARTESIAN_POINT ( 'NONE',  ( -105.4894168351564048, 19.67999904371083275, 8.151722511394638104 ) ) ;
#5049=CARTESIAN_POINT ( 'NONE',  ( 83.11963132830025813, -9.001241435568109850, 24.42551322431495819 ) ) ;
#5051=CARTESIAN_POINT ( 'NONE',  ( -208.1127848780265026, 15.00245453012665564, 0.000000000000000000 ) ) ;
#5054=CARTESIAN_POINT ( 'NONE',  ( 192.4448373802101173, -42.42640687116510634, 14.14213562375845257 ) ) ;
#5055=CARTESIAN_POINT ( 'NONE',  ( -208.1127848780264742, 39.99999999999992895, 15.00245453012683683 ) ) ;
#5057=CARTESIAN_POINT ( 'NONE',  ( 3.854699808470055444, 48.95177852071795854, -14.12217777258769047 ) ) ;
#5058=CARTESIAN_POINT ( 'NONE',  ( 57.59792236341148453, -37.56421063658185489, -40.00000000000002132 ) ) ;
#5059=CARTESIAN_POINT ( 'NONE',  ( 23.58679727197007736, -23.29637218065869675, -42.79169916605220436 ) ) ;
#5061=CARTESIAN_POINT ( 'NONE',  ( 14.38125909742181285, -15.17850393972633505, 40.00000000000002132 ) ) ;
#5062=CARTESIAN_POINT ( 'NONE',  ( 163.1118516004056573, 19.27778845538780317, -19.27778845538757224 ) ) ;
#5063=CARTESIAN_POINT ( 'NONE',  ( 163.1118516004056573, -2.556006622855449647E-13, 27.26290988616872824 ) ) ;
#5064=CARTESIAN_POINT ( 'NONE',  ( -105.3901353554191900, 9.627478968577326768, -19.08722479148772067 ) ) ;
#5065=CARTESIAN_POINT ( 'NONE',  ( 170.2234770963711128, -39.99999999999982947, -15.44714144992858529 ) ) ;
#5067=CARTESIAN_POINT ( 'NONE',  ( -77.90255099906772784, 20.04994828523968664, -8.644468104261312291 ) ) ;
#5069=CARTESIAN_POINT ( 'NONE',  ( -198.0356074513804572, 17.40982414986446969, 39.15871834505921356 ) ) ;
#5072=CARTESIAN_POINT ( 'NONE',  ( -3.977426076247482900, 43.16039317622643523, -17.87762021094837195 ) ) ;
#5073=B_SPLINE_CURVE_WITH_KNOTS ( 'NONE', 3,
 ( #12279, #25865, #6035, #3916, #15724, #12015, #5627, #18126, #15999, #14005, #6162, #10156, #16131, #17988, #20135, #9753, #8153, #7741, #1913, #7609, #18259, #23982 ),
 .UNSPECIFIED., .F., .F.,
 ( 4, 2, 2, 2, 2, 2, 2, 2, 2, 2, 4 ),
 ( 0.005049353704792979534, 0.02738431423455156208, 0.04971927476431014375, 0.07205423529406872196, 0.07763797542650840988, 0.08042984549272826078, 0.08182578052583817929, 0.08322171555894809780, 0.08880545569138770245, 0.09159732575760753948, 0.09438919582382739037 ),
 .UNSPECIFIED. ) ;
#5074=CARTESIAN_POINT ( 'NONE',  ( 130.8568914410475088, 34.05028731879790627, 40.00000000000002132 ) ) ;
#5076=CARTESIAN_POINT ( 'NONE',  ( -175.9234132810913991, -42.70618379831009293, 12.95567001217066760 ) ) ;
#5077=CARTESIAN_POINT ( 'NONE',  ( -109.1264249741455785, -33.12752917269520481, -13.72187187123273233 ) ) ;
#5081=CARTESIAN_POINT ( 'NONE',  ( 4.995406935893293543, -10.78321810389005364, 10.78321810388994173 ) ) ;
#5082=CARTESIAN_POINT ( 'NONE',  ( 35.93765801236255442, -38.99300236445704115, -20.78447758918573385 ) ) ;
#5083=ORIENTED_EDGE ( 'NONE', *, *, #306, .F. ) ;
#5087=ADVANCED_FACE ( 'NONE', ( #9882 ), #24163, .T. ) ;
#5088=CARTESIAN_POINT ( 'NONE',  ( 146.6084372240433709, -52.76785682606516303, 3.800685668858563737 ) ) ;
#5089=CARTESIAN_POINT ( 'NONE',  ( -208.1127848780265026, 10.60833733269537049, 10.60833733269544510 ) ) ;
#5090=CARTESIAN_POINT ( 'NONE',  ( 136.1360204305621551, 40.00000000000017053, -35.03383547441281820 ) ) ;
#5091=DIRECTION ( 'NONE',  ( 0.000000000000000000, 1.000000000000000000, 0.000000000000000000 ) ) ;
#5093=CARTESIAN_POINT ( 'NONE',  ( -192.9588430854690273, -39.99999999999991473, -14.46834944100011633 ) ) ;
#5094=CARTESIAN_POINT ( 'NONE',  ( -192.9588430854689989, 5.375290060580374156E-13, -54.46834944099972375 ) ) ;
#5095=CARTESIAN_POINT ( 'NONE',  ( -82.23726319253047734, 14.74589317219750662, 13.81439526601152679 ) ) ;
#5096=CARTESIAN_POINT ( 'NONE',  ( -30.26275506840324070, -29.48230279907780016, -27.08623969584605362 ) ) ;
#5097=CARTESIAN_POINT ( 'NONE',  ( -200.0000000000000284, 23.83302776610025475, -44.89135967046703257 ) ) ;
#5101=DIRECTION ( 'NONE',  ( 0.000000000000000000, 0.9307566067254452458, -0.3656393565207865515 ) ) ;
#5102=CARTESIAN_POINT ( 'NONE',  ( 200.0000000000000000, 42.42640687119290988, 14.14213562373111976 ) ) ;
#5103=CARTESIAN_POINT ( 'NONE',  ( -77.67315633213154058, -18.60060890639466180, 11.80559230995901387 ) ) ;
#5104=CARTESIAN_POINT ( 'NONE',  ( -162.0762913951021176, -29.48230308784793152, 27.08623940707591515 ) ) ;
#5107=EDGE_LOOP ( 'NONE', ( #3352, #6536, #18275, #8400 ) ) ;
#5108=CARTESIAN_POINT ( 'NONE',  ( 14.38125909742180397, 67.30136555898270956, -10.73282306405792319 ) ) ;
#5111=CARTESIAN_POINT ( 'NONE',  ( -105.2054292635175585, -2.444554031225951202E-13, 21.49321519473985020 ) ) ;
#5112=ORIENTED_EDGE ( 'NONE', *, *, #697, .F. ) ;
#5113=CARTESIAN_POINT ( 'NONE',  ( 151.7948205124836534, -40.00000000000034817, 33.23291073765511072 ) ) ;
#5115=CARTESIAN_POINT ( 'NONE',  ( -4.039451493210496125, 23.44932283416649454, 43.00522595894017286 ) ) ;
#5116=ORIENTED_EDGE ( 'NONE', *, *, #11656, .T. ) ;
#5118=CARTESIAN_POINT ( 'NONE',  ( -208.1127848780264742, 55.00245453010919050, -40.00000000000002132 ) ) ;
#5120=ADVANCED_FACE ( 'NONE', ( #10609 ), #21450, .T. ) ;
#5122=CARTESIAN_POINT ( 'NONE',  ( -100.0968563617265943, -20.41799937594479530, -8.893120081421919565 ) ) ;
#5125=CARTESIAN_POINT ( 'NONE',  ( 57.59792236341148453, -40.00000000000000000, -2.435789363418300546 ) ) ;
#5127=CARTESIAN_POINT ( 'NONE',  ( -87.02160542365453466, 10.86122935277673918, 18.50851042352477194 ) ) ;
#5128=CARTESIAN_POINT ( 'NONE',  ( -62.79433447039818361, -11.74096317475005691, -24.94280497470819569 ) ) ;
#5129=CARTESIAN_POINT ( 'NONE',  ( 91.82158438592158234, 12.16597498397756993, 12.16597498397776356 ) ) ;
#5130=CARTESIAN_POINT ( 'NONE',  ( -77.55640685876517182, -16.63820247459988622, -14.66025286086431478 ) ) ;
#5131=CARTESIAN_POINT ( 'NONE',  ( -105.3755690713226585, -39.99999999999985079, -18.24025645688394448 ) ) ;
#5133=CARTESIAN_POINT ( 'NONE',  ( -56.48582580120559982, 9.153146818113574668, -40.00000000000002132 ) ) ;
#5134=CARTESIAN_POINT ( 'NONE',  ( 14.38125909742182529, -39.01709431150933938, 39.01709431150894147 ) ) ;
#5135=CARTESIAN_POINT ( 'NONE',  ( -213.1075012329537230, -53.71589010953668719, -40.00000000000002132 ) ) ;
#5137=CARTESIAN_POINT ( 'NONE',  ( -100.7734535825088500, 40.00000000000008527, -22.67402823373177512 ) ) ;
#5138=CARTESIAN_POINT ( 'NONE',  ( -238.4067589809705794, 0.9644942799825386714, 0.000000000000000000 ) ) ;
#5139=CARTESIAN_POINT ( 'NONE',  ( 146.6084372240433993, 3.800685668858676980, 3.800685668858667210 ) ) ;
#5140=CARTESIAN_POINT ( 'NONE',  ( -105.3755690713226585, 18.24025645688350750, -40.00000000000002132 ) ) ;
#5142=CARTESIAN_POINT ( 'NONE',  ( 5.823571940226716315, -44.77584346942416715, 24.75780943188591010 ) ) ;
#5143=( BOUNDED_SURFACE ( )  B_SPLINE_SURFACE ( 3, 3, ( 
 ( #12120, #23824, #7719, #9861, #12254, #3887, #1622, #5870, #7986, #14243, #24236, #24095, #22110, #20245, #2025, #17831, #6009, #9729, #15970, #16243, #25844, #17700, #13713, #19971, #15829, #21838, #9595, #10127, #7588, #13839 ),
 ( #22245, #5734, #23959, #16104, #18228, #15, #8126, #17963, #6135, #22383, #15700, #3607, #11717, #19836, #25978, #10261, #24769, #4551, #4678, #18903, #554, #8387, #12648, #24506, #2412, #24634, #6266, #16640, #6392, #12379 ),
 ( #20773, #14508, #4414, #20908, #14379, #2543, #22512, #16903, #10661, #18770, #22639, #4290, #20507, #16509, #16766, #4815, #8791, #6788, #12508, #20376, #150, #2279, #16372, #418, #10388, #18371, #10793, #18499, #2686, #280 ),
 ( #8522, #8254, #22900, #25035, #20636, #10521, #18635, #6522, #12781, #14900, #14633, #22770, #23040, #2151, #8658, #24900, #6655, #682, #14770, #13644, #17032, #9793, #21770, #11643, #7051, #25167, #13050, #947, #9661, #24024 ),
 ( #10926, #15762, #15035, #11172, #25424, #23293, #25907, #1689, #8922, #12917, #7524, #19287, #816, #1556, #3543, #21296, #23757, #19765, #5538, #11785, #15168, #19905, #26044, #1070, #2817, #6918, #23891, #17765, #7648, #21034 ),
 ( #11051, #19037, #17896, #9179, #17290, #5069, #15632, #23165, #13175, #5667, #13773, #3070, #21900, #3677, #4944, #7781, #15897, #21168, #19162, #2941, #9055, #17160, #25294, #1822, #18030, #16037, #26180, #9924, #7920, #5803 ),
 ( #13910, #22045, #3818, #11921, #20043, #10650, #17151, #12636, #25026, #4669, #12908, #23156, #1062, #15281, #6779, #14891, #9046, #8781, #672, #2933, #10917, #25158, #21159, #18893, #13166, #10781, #23031, #8648, #9168, #4539 ) ),
 .UNSPECIFIED., .T., .F., .F. ) 
 B_SPLINE_SURFACE_WITH_KNOTS ( ( 4, 3, 4 ),
 ( 4, 2, 2, 2, 2, 2, 2, 2, 2, 2, 2, 2, 2, 2, 4 ),
 ( 0.000000000000000000, 0.5000000000000000000, 1.000000000000000000 ),
 ( 0.000000000000000000, 0.1357259735107005372, 0.1651108541090157700, 0.1944957347073310028, 0.3598804999793158710, 0.3867117631979620773, 0.4135430264166082281, 0.5789277916885930964, 0.6062785021374117456, 0.6336292125862302838, 0.8508620842112317728, 0.8814014469398914198, 0.9119408096685510667, 0.9559704048342755334, 1.000000000000000000 ),
 .UNSPECIFIED. ) 
 GEOMETRIC_REPRESENTATION_ITEM ( )  RATIONAL_B_SPLINE_SURFACE ( (
 ( 1.000000000000000000, 1.000000000000000000, 1.000000000000000000, 1.000000000000000000, 1.000000000000000000, 1.000000000000000000, 1.000000000000000000, 1.000000000000000000, 1.000000000000000000, 1.000000000000000000, 1.000000000000000000, 1.000000000000000000, 1.000000000000000000, 1.000000000000000000, 1.000000000000000000, 1.000000000000000000, 1.000000000000000000, 1.000000000000000000, 1.000000000000000000, 1.000000000000000000, 1.000000000000000000, 1.000000000000000000, 1.000000000000000000, 1.000000000000000000, 1.000000000000000000, 1.000000000000000000, 1.000000000000000000, 1.000000000000000000, 1.000000000000000000, 1.000000000000000000),
 ( 0.3333333333333333703, 0.3333333333333333703, 0.3333333333333333703, 0.3333333333333333703, 0.3333333333333333703, 0.3333333333333333703, 0.3333333333333333703, 0.3333333333333333703, 0.3333333333333333703, 0.3333333333333333703, 0.3333333333333333703, 0.3333333333333333703, 0.3333333333333333703, 0.3333333333333333703, 0.3333333333333333703, 0.3333333333333333703, 0.3333333333333333703, 0.3333333333333333703, 0.3333333333333333703, 0.3333333333333333703, 0.3333333333333333703, 0.3333333333333333703, 0.3333333333333333703, 0.3333333333333333703, 0.3333333333333333703, 0.3333333333333333703, 0.3333333333333333703, 0.3333333333333333703, 0.3333333333333333703, 0.3333333333333333703),
 ( 0.3333333333333333703, 0.3333333333333333703, 0.3333333333333333703, 0.3333333333333333703, 0.3333333333333333703, 0.3333333333333333703, 0.3333333333333333703, 0.3333333333333333703, 0.3333333333333333703, 0.3333333333333333703, 0.3333333333333333703, 0.3333333333333333703, 0.3333333333333333703, 0.3333333333333333703, 0.3333333333333333703, 0.3333333333333333703, 0.3333333333333333703, 0.3333333333333333703, 0.3333333333333333703, 0.3333333333333333703, 0.3333333333333333703, 0.3333333333333333703, 0.3333333333333333703, 0.3333333333333333703, 0.3333333333333333703, 0.3333333333333333703, 0.3333333333333333703, 0.3333333333333333703, 0.3333333333333333703, 0.3333333333333333703),
 ( 1.000000000000000000, 1.000000000000000000, 1.000000000000000000, 1.000000000000000000, 1.000000000000000000, 1.000000000000000000, 1.000000000000000000, 1.000000000000000000, 1.000000000000000000, 1.000000000000000000, 1.000000000000000000, 1.000000000000000000, 1.000000000000000000, 1.000000000000000000, 1.000000000000000000, 1.000000000000000000, 1.000000000000000000, 1.000000000000000000, 1.000000000000000000, 1.000000000000000000, 1.000000000000000000, 1.000000000000000000, 1.000000000000000000, 1.000000000000000000, 1.000000000000000000, 1.000000000000000000, 1.000000000000000000, 1.000000000000000000, 1.000000000000000000, 1.000000000000000000),
 ( 0.3333333333333333703, 0.3333333333333333703, 0.3333333333333333703, 0.3333333333333333703, 0.3333333333333333703, 0.3333333333333333703, 0.3333333333333333703, 0.3333333333333333703, 0.3333333333333333703, 0.3333333333333333703, 0.3333333333333333703, 0.3333333333333333703, 0.3333333333333333703, 0.3333333333333333703, 0.3333333333333333703, 0.3333333333333333703, 0.3333333333333333703, 0.3333333333333333703, 0.3333333333333333703, 0.3333333333333333703, 0.3333333333333333703, 0.3333333333333333703, 0.3333333333333333703, 0.3333333333333333703, 0.3333333333333333703, 0.3333333333333333703, 0.3333333333333333703, 0.3333333333333333703, 0.3333333333333333703, 0.3333333333333333703),
 ( 0.3333333333333333703, 0.3333333333333333703, 0.3333333333333333703, 0.3333333333333333703, 0.3333333333333333703, 0.3333333333333333703, 0.3333333333333333703, 0.3333333333333333703, 0.3333333333333333703, 0.3333333333333333703, 0.3333333333333333703, 0.3333333333333333703, 0.3333333333333333703, 0.3333333333333333703, 0.3333333333333333703, 0.3333333333333333703, 0.3333333333333333703, 0.3333333333333333703, 0.3333333333333333703, 0.3333333333333333703, 0.3333333333333333703, 0.3333333333333333703, 0.3333333333333333703, 0.3333333333333333703, 0.3333333333333333703, 0.3333333333333333703, 0.3333333333333333703, 0.3333333333333333703, 0.3333333333333333703, 0.3333333333333333703),
 ( 1.000000000000000000, 1.000000000000000000, 1.000000000000000000, 1.000000000000000000, 1.000000000000000000, 1.000000000000000000, 1.000000000000000000, 1.000000000000000000, 1.000000000000000000, 1.000000000000000000, 1.000000000000000000, 1.000000000000000000, 1.000000000000000000, 1.000000000000000000, 1.000000000000000000, 1.000000000000000000, 1.000000000000000000, 1.000000000000000000, 1.000000000000000000, 1.000000000000000000, 1.000000000000000000, 1.000000000000000000, 1.000000000000000000, 1.000000000000000000, 1.000000000000000000, 1.000000000000000000, 1.000000000000000000, 1.000000000000000000, 1.000000000000000000, 1.000000000000000000) ) ) 
 REPRESENTATION_ITEM ( '' )  SURFACE ( )  );
#5144=CARTESIAN_POINT ( 'NONE',  ( -87.12803293485012546, -14.20621343981222928, 16.13817828097420204 ) ) ;
#5145=CARTESIAN_POINT ( 'NONE',  ( 57.59792236341147031, -1.722363176415123043, 54.84617931850879557 ) ) ;
#5146=CARTESIAN_POINT ( 'NONE',  ( -198.0356074513804572, -40.00000000000011369, 15.37879056873056527 ) ) ;
#5147=FACE_OUTER_BOUND ( 'NONE', #10997, .T. ) ;
#5149=CARTESIAN_POINT ( 'NONE',  ( 8.517493190815727644, -14.17913040910352329, -49.32792454093244316 ) ) ;
#5152=CARTESIAN_POINT ( 'NONE',  ( 170.0000000000000284, -22.62041470344884431, 9.369682556672202622 ) ) ;
#5153=CARTESIAN_POINT ( 'NONE',  ( 19.06497207195979726, 38.31983398719604139, 18.24870850772803976 ) ) ;
#5154=CARTESIAN_POINT ( 'NONE',  ( -213.1075012329537230, -9.698598906462304825, -66.26714140138675191 ) ) ;
#5155=CARTESIAN_POINT ( 'NONE',  ( 192.4448373802101173, 42.42640687122070631, 14.14213562370331623 ) ) ;
#5156=CARTESIAN_POINT ( 'NONE',  ( 192.4448373802100889, -14.14213562375896061, 14.14213562375865330 ) ) ;
#5157=CARTESIAN_POINT ( 'NONE',  ( -162.0762913951021176, 27.08623940707639477, -29.48230308784743059 ) ) ;
#5158=CARTESIAN_POINT ( 'NONE',  ( -213.1075012329537230, -9.698598906462304825, -66.26714140138675191 ) ) ;
#5159=CARTESIAN_POINT ( 'NONE',  ( 200.0000000000000000, -14.14213562373046784, -42.42640687119298804 ) ) ;
#5160=CARTESIAN_POINT ( 'NONE',  ( 0.2972598230769959993, 38.42060263243713081, -38.42060263243619289 ) ) ;
#5161=CARTESIAN_POINT ( 'NONE',  ( 0.2972598230769930017, 14.33493731733933352, -40.00000000000002132 ) ) ;
#5164=CARTESIAN_POINT ( 'NONE',  ( -100.7734535825088500, -12.25131212657524316, 44.31723036834888774 ) ) ;
#5166=CARTESIAN_POINT ( 'NONE',  ( -188.2506440019725176, 46.97351617221541176, -13.82466072834929705 ) ) ;
#5168=CARTESIAN_POINT ( 'NONE',  ( 146.6084372240433709, 32.08495691632064961, -24.48358557860320417 ) ) ;
#5170=CARTESIAN_POINT ( 'NONE',  ( -88.39148973765153983, -20.15708830332398804, -8.027153355909376842 ) ) ;
#5171=CARTESIAN_POINT ( 'NONE',  ( 19.94008347562303030, 24.01421467034686330, 43.76810615267632443 ) ) ;
#5172=CARTESIAN_POINT ( 'NONE',  ( -3.564770973659422193, -43.27160733161171891, -17.92368662243730171 ) ) ;
#5174=CARTESIAN_POINT ( 'NONE',  ( -187.3036811847832723, -42.71162014090015191, 23.25512365538946469 ) ) ;
#5175=ADVANCED_FACE ( 'NONE', ( #20701 ), #562, .T. ) ;
#5177=CARTESIAN_POINT ( 'NONE',  ( 23.32574057153296110, -13.80366151303459077, 46.82643129194502762 ) ) ;
#5178=CARTESIAN_POINT ( 'NONE',  ( 48.46027422360368320, 35.02097763790654739, -18.19770396007656643 ) ) ;
#5181=CARTESIAN_POINT ( 'NONE',  ( 128.5824617753800680, -28.96492468983284496, 11.99766463964388663 ) ) ;
#5182=CARTESIAN_POINT ( 'NONE',  ( -100.7734535825088358, 6.065416334915073333E-14, -22.67402823373191723 ) ) ;
#5183=CARTESIAN_POINT ( 'NONE',  ( 91.82158438592158234, 7.693928927950222250E-14, -17.20528682183300262 ) ) ;
#5184=( BOUNDED_SURFACE ( )  B_SPLINE_SURFACE ( 3, 2, ( 
 ( #12598, #10606, #11502 ),
 ( #19626, #21756, #23877 ),
 ( #3529, #19248, #7133 ),
 ( #15749, #19752, #9263 ),
 ( #25381, #5272, #5653 ),
 ( #13377, #1159, #11630 ),
 ( #7381, #1411, #17370 ),
 ( #15492, #11133, #5524 ),
 ( #15246, #9512, #23377 ),
 ( #23622, #1029, #5402 ),
 ( #21624, #19495, #17494 ),
 ( #9128, #25508, #17617 ),
 ( #25635, #3276, #9387 ),
 ( #25762, #7257, #15375 ),
 ( #17752, #19372, #13759 ),
 ( #1542, #13631, #11374 ) ),
 .UNSPECIFIED., .F., .F., .F. ) 
 B_SPLINE_SURFACE_WITH_KNOTS ( ( 4, 2, 2, 2, 2, 2, 2, 4 ),
 ( 3, 3 ),
 ( 0.04143342415447111293, 0.04844559399083352147, 0.05195167890901472574, 0.05545776382719592307, 0.06246993366355832467, 0.06422297612264893374, 0.06597601858173952893, 0.06948210349992073320 ),
 ( 0.000000000000000000, 1.000000000000000000 ),
 .UNSPECIFIED. ) 
 GEOMETRIC_REPRESENTATION_ITEM ( )  RATIONAL_B_SPLINE_SURFACE ( (
 ( 1.000000000000000000, 0.9541700779530459808, 1.000000000000000000),
 ( 1.000000000000000000, 0.9520168980288470362, 1.000000000000000000),
 ( 1.000000000000000000, 0.9503263051615414847, 1.000000000000000000),
 ( 1.000000000000000000, 0.9485964699089932672, 1.000000000000000000),
 ( 1.000000000000000000, 0.9481599523395594087, 1.000000000000000000),
 ( 1.000000000000000000, 0.9475783919172264813, 1.000000000000000000),
 ( 1.000000000000000000, 0.9474332805893206366, 1.000000000000000000),
 ( 1.000000000000000000, 0.9474385816627715062, 1.000000000000000000),
 ( 1.000000000000000000, 0.9480200071115888472, 1.000000000000000000),
 ( 1.000000000000000000, 0.9494436219492867757, 1.000000000000000000),
 ( 1.000000000000000000, 0.9497633688930613438, 1.000000000000000000),
 ( 1.000000000000000000, 0.9504729676350489598, 1.000000000000000000),
 ( 1.000000000000000000, 0.9508638236297636270, 1.000000000000000000),
 ( 1.000000000000000000, 0.9521268919818258736, 1.000000000000000000),
 ( 1.000000000000000000, 0.9530924015899429058, 1.000000000000000000),
 ( 1.000000000000000000, 0.9541700779530460919, 1.000000000000000000) ) ) 
 REPRESENTATION_ITEM ( '' )  SURFACE ( )  );
#5186=CARTESIAN_POINT ( 'NONE',  ( -91.56559293963834989, -17.32597176626812896, -2.449293598294708485E-15 ) ) ;
#5187=CARTESIAN_POINT ( 'NONE',  ( 25.05785482536186137, -17.61697374403291505, -42.53113694077947571 ) ) ;
#5188=CARTESIAN_POINT ( 'NONE',  ( 170.0000000000000000, 30.00000000000007105, 0.000000000000000000 ) ) ;
#5189=CARTESIAN_POINT ( 'NONE',  ( -208.1127848780265026, -15.00245453012673202, 0.000000000000000000 ) ) ;
#5190=CARTESIAN_POINT ( 'NONE',  ( 136.1360204305621266, 24.77266263493138965, -24.77266263493110188 ) ) ;
#5191=CARTESIAN_POINT ( 'NONE',  ( 151.7948205124836534, 39.99999999999970157, 33.23291073765595627 ) ) ;
#5192=CARTESIAN_POINT ( 'NONE',  ( -100.7734535825088500, -39.99999999999986500, -17.32597176626853397 ) ) ;
#5196=CARTESIAN_POINT ( 'NONE',  ( 11.28112952480928755, 44.87390167243371053, -18.58737866929334359 ) ) ;
#5197=CARTESIAN_POINT ( 'NONE',  ( 146.6084372240433709, -5.374981219216948602, 40.00000000000002132 ) ) ;
#5199=CARTESIAN_POINT ( 'NONE',  ( -194.7885354600941525, 44.44047100927782878, -18.40784581029470957 ) ) ;
#5201=EDGE_LOOP ( 'NONE', ( #20211, #11684, #5915, #4160 ) ) ;
#5203=CARTESIAN_POINT ( 'NONE',  ( 136.1360204305621266, 24.77266263493138965, -24.77266263493110188 ) ) ;
#5206=VERTEX_POINT ( 'NONE', #8690 ) ;
#5208=CARTESIAN_POINT ( 'NONE',  ( -114.4364955367327070, 8.644468109209567430, -20.04994829327642947 ) ) ;
#5209=CARTESIAN_POINT ( 'NONE',  ( 170.2234770963711128, 10.92277846919201068, 10.92277846919202133 ) ) ;
#5210=CARTESIAN_POINT ( 'NONE',  ( -114.4364955367319965, -20.29001642039104070, -8.064892380835031460 ) ) ;
#5211=CARTESIAN_POINT ( 'NONE',  ( -56.48582580120559271, 2.158176344243877536E-14, -9.153146818113587102 ) ) ;
#5214=CARTESIAN_POINT ( 'NONE',  ( 0.2972598230770103767, -39.99999999999945288, -54.33493731733979359 ) ) ;
#5215=CARTESIAN_POINT ( 'NONE',  ( 19.06497207195981858, 5.735870351258996432E-13, -54.19242893257843008 ) ) ;
#5216=CARTESIAN_POINT ( 'NONE',  ( -77.71409353909379547, 19.10608670630663397, 10.98878756468862861 ) ) ;
#5217=CARTESIAN_POINT ( 'NONE',  ( -192.9588430854690273, -66.79921049724377724, 10.23066800231950069 ) ) ;
#5218=CARTESIAN_POINT ( 'NONE',  ( 19.06497207195981147, -4.605042221739098431E-14, 14.19242893257840521 ) ) ;
#5219=CARTESIAN_POINT ( 'NONE',  ( -56.48582580120559271, 6.472252184284211118, -6.472252184284153387 ) ) ;
#5220=CARTESIAN_POINT ( 'NONE',  ( 133.2080217031554810, 29.90338805389109211, 12.38638889282741573 ) ) ;
#5223=CARTESIAN_POINT ( 'NONE',  ( -82.23729782350187634, -15.18297044030989440, 13.37626936638599950 ) ) ;
#5224=CARTESIAN_POINT ( 'NONE',  ( -30.26275506840323715, 29.48230279907789253, 29.48230279907799556 ) ) ;
#5225=CARTESIAN_POINT ( 'NONE',  ( 0.2972598230770027716, -38.42060263243681817, 18.14793986248684377 ) ) ;
#5226=CARTESIAN_POINT ( 'NONE',  ( -114.4364955367321102, -8.064892380842767494, -20.29001642038801734 ) ) ;
#5227=CARTESIAN_POINT ( 'NONE',  ( -93.12335834970892279, 16.03295912088692177, 16.03295912088721664 ) ) ;
#5228=ORIENTED_EDGE ( 'NONE', *, *, #21220, .F. ) ;
#5229=CARTESIAN_POINT ( 'NONE',  ( 146.6084372240433709, 32.08495691632030145, 24.48358557860365181 ) ) ;
#5230=CARTESIAN_POINT ( 'NONE',  ( 192.4448373802100889, 20.00000000003945644, 0.000000000000000000 ) ) ;
#5231=DIRECTION ( 'NONE',  ( 1.000000000000000000, 1.836970198721030181E-16, 0.000000000000000000 ) ) ;
#5232=VERTEX_POINT ( 'NONE', #7203 ) ;
#5233=DIRECTION ( 'NONE',  ( 0.9352143323240564854, -0.1355013636652032116, 0.3271292299085176158 ) ) ;
#5235=CARTESIAN_POINT ( 'NONE',  ( -200.0000000000001421, -14.17215463606902404, -49.28189405767602693 ) ) ;
#5236=ORIENTED_EDGE ( 'NONE', *, *, #11202, .T. ) ;
#5238=CARTESIAN_POINT ( 'NONE',  ( 136.1360204305621266, 24.77266263493138965, -24.77266263493110188 ) ) ;
#5239=CARTESIAN_POINT ( 'NONE',  ( -105.3755690713226585, 40.00000000000007816, -21.75974354311636461 ) ) ;
#5240=CARTESIAN_POINT ( 'NONE',  ( -97.73860346104240193, -20.89580782304671658, -8.185503821051291595 ) ) ;
#5241=EDGE_CURVE ( 'NONE', #9554, #24441, #12998, .T. ) ;
#5243=CARTESIAN_POINT ( 'NONE',  ( -135.8532207217289738, -40.00000000000001421, -9.153146818113709671 ) ) ;
#5245=EDGE_CURVE ( 'NONE', #11726, #6963, #15001, .T. ) ;
#5246=CARTESIAN_POINT ( 'NONE',  ( -77.55640685878515228, 14.66973228108125582, 16.62872305437120701 ) ) ;
#5247=CARTESIAN_POINT ( 'NONE',  ( -6.342283169552904276, -23.00001740814894546, -42.32555349774978737 ) ) ;
#5248=CARTESIAN_POINT ( 'NONE',  ( -198.0356074513804572, -10.87444709758429262, -67.44298959250878056 ) ) ;
#5249=LINE ( 'NONE', #11745, #15248 ) ;
#5250=CARTESIAN_POINT ( 'NONE',  ( -213.1075012329537230, -39.99999999999948841, -53.71589010950208376 ) ) ;
#5252=CARTESIAN_POINT ( 'NONE',  ( 200.0000000000000000, 20.00000000000013856, 40.00000000000002132 ) ) ;
#5253=CARTESIAN_POINT ( 'NONE',  ( -162.0762913951020892, -41.69427287672991866, -40.00000000000002132 ) ) ;
#5256=CARTESIAN_POINT ( 'NONE',  ( 57.59792236341148453, 1.722363176414758668, 54.84617931850880268 ) ) ;
#5257=CARTESIAN_POINT ( 'NONE',  ( -259.2033419157646676, 9.517827891722582478, -40.00000000000002132 ) ) ;
#5258=CARTESIAN_POINT ( 'NONE',  ( -114.4008516218694496, 20.18474087537135730, 8.248277354728019262 ) ) ;
#5259=CARTESIAN_POINT ( 'NONE',  ( 4.995406935893283773, 39.99999999999997158, 15.24977328854846803 ) ) ;
#5260=CARTESIAN_POINT ( 'NONE',  ( -114.6170081391615838, 21.23870042814614933, 5.725526104550264783 ) ) ;
#5261=CARTESIAN_POINT ( 'NONE',  ( 151.7948205124836534, -23.49921654116027980, 33.06932595376354556 ) ) ;
#5262=CARTESIAN_POINT ( 'NONE',  ( -135.8532207217289738, 30.84685318188643777, -40.00000000000002132 ) ) ;
#5264=CARTESIAN_POINT ( 'NONE',  ( 22.66553228237864204, -43.20407469282417168, 17.89571368754787528 ) ) ;
#5265=CARTESIAN_POINT ( 'NONE',  ( -105.2502153031277601, 17.39736479739449138, -12.58638139385909760 ) ) ;
#5266=CARTESIAN_POINT ( 'NONE',  ( -100.7734535825088358, 12.25131212657480440, 12.25131212657487012 ) ) ;
#5267=CARTESIAN_POINT ( 'NONE',  ( 14.38125909742181108, -5.035366881890652543E-14, 15.17850393972633682 ) ) ;
#5268=CARTESIAN_POINT ( 'NONE',  ( -77.65265458751275673, 21.61050232527882287, -4.374419871749616107 ) ) ;
#5269=CARTESIAN_POINT ( 'NONE',  ( 1.564252679174726213, -14.06374044400928724, -48.56509332159251358 ) ) ;
#5271=CARTESIAN_POINT ( 'NONE',  ( -87.13361725323537144, -21.49321519332493580, -1.359587258213210248 ) ) ;
#5272=CARTESIAN_POINT ( 'NONE',  ( -82.24432634617156168, 2.528896859437274269, -20.04338201863724578 ) ) ;
#5273=CARTESIAN_POINT ( 'NONE',  ( -259.2033419157646676, -6.730120644403663199, 6.730120644403451813 ) ) ;
#5274=CARTESIAN_POINT ( 'NONE',  ( -198.0356074513804572, -10.87444709758429262, -67.44298959250878056 ) ) ;
#5275=CARTESIAN_POINT ( 'NONE',  ( -56.48582580120559982, 34.75652343174597547, 21.81201906317791384 ) ) ;
#5276=CARTESIAN_POINT ( 'NONE',  ( 199.9999999999999432, -14.14213562373115884, 14.14213562373085153 ) ) ;
#5277=CARTESIAN_POINT ( 'NONE',  ( -135.8532207217289738, 6.472252184284583265, -50.09629031063960980 ) ) ;
#5278=CARTESIAN_POINT ( 'NONE',  ( 184.8905102610680444, 14.79361573936424890, -41.77492675555986068 ) ) ;
#5279=CARTESIAN_POINT ( 'NONE',  ( 57.59792236341147031, -1.722363176414363206, -54.84617931850881689 ) ) ;
#5280=CARTESIAN_POINT ( 'NONE',  ( 4.995406935893290878, 39.06748935135239265, -39.06748935135144762 ) ) ;
#5281=CARTESIAN_POINT ( 'NONE',  ( -105.2054292635175585, -15.19799821370250825, 15.19799821370211923 ) ) ;
#5282=CARTESIAN_POINT ( 'NONE',  ( 130.8568914410475372, -24.07718906447222551, -24.07718906447233209 ) ) ;
#5284=CARTESIAN_POINT ( 'NONE',  ( 170.2234770963711128, -10.92277846919235529, 45.64576402573175073 ) ) ;
#5285=CARTESIAN_POINT ( 'NONE',  ( -192.9588430854690273, 54.46834944101718889, 40.00000000000002132 ) ) ;
#5287=CARTESIAN_POINT ( 'NONE',  ( -135.8532207217289738, 21.81201906317777883, -34.75652343174605363 ) ) ;
#5288=CARTESIAN_POINT ( 'NONE',  ( -82.24286360236595783, -15.97561011111183049, -12.41695498259727692 ) ) ;
#5289=CARTESIAN_POINT ( 'NONE',  ( 25.62979979009272924, 22.88075396655783322, 42.16299361905724652 ) ) ;
#5290=CARTESIAN_POINT ( 'NONE',  ( -8.255580677151938218, -41.75907689858397731, -22.62611236873543774 ) ) ;
#5292=CARTESIAN_POINT ( 'NONE',  ( -183.1090696431200229, -45.18841929385192202, 13.45963186438693704 ) ) ;
#5294=CARTESIAN_POINT ( 'NONE',  ( 37.37129771735379080, -20.48130208310442413, 38.51719860173601262 ) ) ;
#5298=CARTESIAN_POINT ( 'NONE',  ( -91.56559293963836410, 40.00000000000008527, -22.67402823373177867 ) ) ;
#5299=CARTESIAN_POINT ( 'NONE',  ( -82.26522640325165980, -5.034412314778461628, 19.58751121911369708 ) ) ;
#5301=CARTESIAN_POINT ( 'NONE',  ( 146.6084372240433709, -5.374981219216948602, 40.00000000000002132 ) ) ;
#5302=CARTESIAN_POINT ( 'NONE',  ( 36.66494225458649225, -16.22659705900232652, -39.17447069114147951 ) ) ;
#5304=CARTESIAN_POINT ( 'NONE',  ( 57.59792236341147031, 2.435789363418170872, 40.00000000000002132 ) ) ;
#5305=CARTESIAN_POINT ( 'NONE',  ( 14.38125909742181285, -10.73282306404727393, 10.73282306404716380 ) ) ;
#5306=CARTESIAN_POINT ( 'NONE',  ( -238.4067589809705794, 40.00000000000040501, -40.96449427990138759 ) ) ;
#5307=CARTESIAN_POINT ( 'NONE',  ( -30.26275506840323359, -39.99999999999959499, -41.69427246844670520 ) ) ;
#5308=EDGE_CURVE ( 'NONE', #12893, #2033, #4231, .T. ) ;
#5309=CARTESIAN_POINT ( 'NONE',  ( 104.1674819957097355, -20.61915445364400412, -8.540733419364878287 ) ) ;
#5310=ORIENTED_EDGE ( 'NONE', *, *, #22980, .F. ) ;
#5312=CARTESIAN_POINT ( 'NONE',  ( -4.082462733454346626, 46.97557262069204853, -13.82507958736555231 ) ) ;
#5313=CARTESIAN_POINT ( 'NONE',  ( -198.0356074513804572, -55.37879056874826489, 40.00000000000002132 ) ) ;
#5315=CARTESIAN_POINT ( 'NONE',  ( -197.4154352060510575, 44.73190714601614815, -24.72550168627246592 ) ) ;
#5319=ORIENTED_EDGE ( 'NONE', *, *, #16953, .F. ) ;
#5321=CARTESIAN_POINT ( 'NONE',  ( 154.0339099654740949, 11.67508747798894753, -28.18615453125283210 ) ) ;
#5322=CARTESIAN_POINT ( 'NONE',  ( 107.5473083967345076, 1.035215841339324533E-13, -23.99138244111055585 ) ) ;
#5323=ORIENTED_EDGE ( 'NONE', *, *, #14014, .T. ) ;
#5327=CARTESIAN_POINT ( 'NONE',  ( -189.2428547182112766, 13.87687415872436603, 47.31876910929162960 ) ) ;
#5329=CARTESIAN_POINT ( 'NONE',  ( -259.2033419157646676, 21.55415060305830366, 21.55415060305842800 ) ) ;
#5330=CARTESIAN_POINT ( 'NONE',  ( 23.37394308801978937, 23.33966569535129310, -42.85717664514559999 ) ) ;
#5331=CARTESIAN_POINT ( 'NONE',  ( -259.2033419157646676, -1.438356298054549103E-14, -9.517827891722632216 ) ) ;
#5332=CARTESIAN_POINT ( 'NONE',  ( -199.9999999999999716, -48.92947633520100226, 14.52307781036571299 ) ) ;
#5334=B_SPLINE_CURVE_WITH_KNOTS ( 'NONE', 3,
 ( #15033, #11415, #13543, #25165, #4942, #15534 ),
 .UNSPECIFIED., .F., .F.,
 ( 4, 2, 4 ),
 ( -5.998621905481146787E-08, 0.03937827992695891455, 0.07875661984013687666 ),
 .UNSPECIFIED. ) ;
#5336=CARTESIAN_POINT ( 'NONE',  ( 14.38125909742181818, -39.99999999999986500, -15.17850393972675604 ) ) ;
#5337=CARTESIAN_POINT ( 'NONE',  ( 199.9999999999999432, 2.486775779033024914E-13, -19.99999999999992539 ) ) ;
#5338=CARTESIAN_POINT ( 'NONE',  ( -82.24528527568789116, 16.01766212874386142, 12.29859689796261435 ) ) ;
#5339=CARTESIAN_POINT ( 'NONE',  ( 0.2972598230770027716, -38.42060263243656237, -18.14793986248737667 ) ) ;
#5340=CARTESIAN_POINT ( 'NONE',  ( 4.995406935893290878, -5.232665749138292703E-14, 15.24977328854832592 ) ) ;
#5341=CARTESIAN_POINT ( 'NONE',  ( 170.2234770963711128, 17.36149277827004411, -17.36149277826983095 ) ) ;
#5342=DIRECTION ( 'NONE',  ( 0.000000000000000000, 0.3656393565198218232, -0.9307566067258242759 ) ) ;
#5345=CARTESIAN_POINT ( 'NONE',  ( -198.0356074513804572, -10.87444709759729911, 10.87444709759714812 ) ) ;
#5346=CARTESIAN_POINT ( 'NONE',  ( -77.84351360267456243, 20.59686641853765110, -7.423967632478677636 ) ) ;
#5347=CARTESIAN_POINT ( 'NONE',  ( 151.7948205124836534, -51.78348778862535795, 4.785054706298367044 ) ) ;
#5350=CARTESIAN_POINT ( 'NONE',  ( -213.1075012329537230, -66.26714140136188291, -9.698598906438677503 ) ) ;
#5354=CARTESIAN_POINT ( 'NONE',  ( 170.2234770963711128, 39.20704971665372796, 17.36149277827039583 ) ) ;
#5355=CARTESIAN_POINT ( 'NONE',  ( 199.9999999999999432, 20.00000000000013856, 0.000000000000000000 ) ) ;
#5356=CARTESIAN_POINT ( 'NONE',  ( 170.0000000000001421, 9.369682556672135121, 22.62041470344889760 ) ) ;
#5358=CARTESIAN_POINT ( 'NONE',  ( 130.8568914410475088, -40.00000000000036238, 34.05028731879746573 ) ) ;
#5360=CARTESIAN_POINT ( 'NONE',  ( -70.33906596057607885, 9.443630424063320206, 22.79894064192813730 ) ) ;
#5364=AXIS2_PLACEMENT_3D ( 'NONE', #7596, #5233, #17709 ) ;
#5365=CARTESIAN_POINT ( 'NONE',  ( -105.3755690713226585, -12.89780903124383471, -43.67073346367985920 ) ) ;
#5366=CARTESIAN_POINT ( 'NONE',  ( 130.8568914410475372, 8.154165912415230659E-16, 5.949712681206690945 ) ) ;
#5370=CARTESIAN_POINT ( 'NONE',  ( 19.06497207195982924, -40.00000000000021316, 54.19242893257830218 ) ) ;
#5372=CARTESIAN_POINT ( 'NONE',  ( 57.59792236341147031, 1.908507979671054758E-14, -2.435789363418160658 ) ) ;
#5375=CARTESIAN_POINT ( 'NONE',  ( -16.78454218927544517, -16.41855578218329725, -39.63790004357984031 ) ) ;
#5376=CARTESIAN_POINT ( 'NONE',  ( -91.56559293963836410, 44.31723036834908669, -12.25131212657445801 ) ) ;
#5377=CARTESIAN_POINT ( 'NONE',  ( -87.11162894489338271, -17.01505826597962923, 13.17695786910780242 ) ) ;
#5378=CARTESIAN_POINT ( 'NONE',  ( -162.0762913951020892, -39.99999999999961631, -41.69427287692722928 ) ) ;
#5380=CARTESIAN_POINT ( 'NONE',  ( 163.1118516004056573, -12.73709011382472589, 40.00000000000002132 ) ) ;
#5381=CARTESIAN_POINT ( 'NONE',  ( -192.9588430854690273, -14.46834944099973264, -40.00000000000002132 ) ) ;
#5382=CARTESIAN_POINT ( 'NONE',  ( -91.56559293963836410, 44.31723036834890905, 12.25131212657507795 ) ) ;
#5383=CARTESIAN_POINT ( 'NONE',  ( 57.59792236341147031, 2.435789363418171760, 0.000000000000000000 ) ) ;
#5384=CARTESIAN_POINT ( 'NONE',  ( 14.33519843538174143, -44.71104701565631956, -24.71012982060716467 ) ) ;
#5386=CARTESIAN_POINT ( 'NONE',  ( -114.7498586125400948, 21.95311410698565879, -2.658373467578531546 ) ) ;
#5387=CARTESIAN_POINT ( 'NONE',  ( 163.1118516004056573, -19.27778845539233998, 37.29075403953149959 ) ) ;
#5388=CARTESIAN_POINT ( 'NONE',  ( -162.0762913951020892, 41.69427287692678163, -40.00000000000002132 ) ) ;
#5391=CARTESIAN_POINT ( 'NONE',  ( 23.58679727197032605, -46.73132340479989466, 13.78527791282015080 ) ) ;
#5392=CARTESIAN_POINT ( 'NONE',  ( -200.0000000000000000, -30.70179486994625861, -44.88127304973837539 ) ) ;
#5395=CARTESIAN_POINT ( 'NONE',  ( 192.4448373802101173, -42.42640687122073473, 14.14213562370301780 ) ) ;
#5396=CARTESIAN_POINT ( 'NONE',  ( 130.8568914410475372, 1.429239637432775288E-13, -34.05028731879788495 ) ) ;
#5397=CARTESIAN_POINT ( 'NONE',  ( -77.72102721667458525, 21.24333237935468688, 5.844331514166557717 ) ) ;
#5401=CARTESIAN_POINT ( 'NONE',  ( -87.02161082285356031, -20.76757691164967667, -5.407310480324148294 ) ) ;
#5402=CARTESIAN_POINT ( 'NONE',  ( -77.65695844554115013, -4.467916498578468065, -21.58737861310262929 ) ) ;
#5403=CARTESIAN_POINT ( 'NONE',  ( 4.995406935893289102, 10.78321810389013002, -10.78321810388986712 ) ) ;
#5404=CARTESIAN_POINT ( 'NONE',  ( 163.1118516004056573, 47.56205970284970164, -9.006482792073828847 ) ) ;
#5405=CARTESIAN_POINT ( 'NONE',  ( -105.2058579006776569, 21.49041530794428567, -0.4803593358688896808 ) ) ;
#5406=CARTESIAN_POINT ( 'NONE',  ( -105.3755690713226585, 15.38646221621820764, -41.18208027870583265 ) ) ;
#5407=CARTESIAN_POINT ( 'NONE',  ( -280.0000000000000000, -14.14213562373088706, -14.14213562373108424 ) ) ;
#5408=CARTESIAN_POINT ( 'NONE',  ( 192.4448373802101173, -42.42640687122053578, -14.14213562370360577 ) ) ;
#5409=CARTESIAN_POINT ( 'NONE',  ( 136.1360204305621266, 3.511608612530757068, -3.511608612530642937 ) ) ;
#5410=CARTESIAN_POINT ( 'NONE',  ( 57.59792236341147031, -2.435789363418150444, 0.000000000000000000 ) ) ;
#5411=DIRECTION ( 'NONE',  ( -1.000000000000000000, -1.836970198721030181E-16, -0.000000000000000000 ) ) ;
#5412=CARTESIAN_POINT ( 'NONE',  ( -280.0000000000000568, -40.00000000000014211, 19.99999999999987210 ) ) ;
#5414=CARTESIAN_POINT ( 'NONE',  ( 192.4448373802101173, 19.99999999996063949, 40.00000000000002132 ) ) ;
#5415=ORIENTED_EDGE ( 'NONE', *, *, #1674, .F. ) ;
#5416=CARTESIAN_POINT ( 'NONE',  ( -30.26275506840325136, 29.48230279907798135, -27.08623969584585112 ) ) ;
#5418=CARTESIAN_POINT ( 'NONE',  ( 8.833560042532678125, 43.71578035519811323, 18.10766911284586200 ) ) ;
#5419=CARTESIAN_POINT ( 'NONE',  ( 90.68848816916745648, 9.291443204245480203, 21.08311784283745638 ) ) ;
#5420=CARTESIAN_POINT ( 'NONE',  ( -5.379830816903176327, -46.52611083736033493, -13.73345071524792438 ) ) ;
#5422=CARTESIAN_POINT ( 'NONE',  ( -121.8281105900276202, -22.46071553383595187, 10.16551987041848548 ) ) ;
#5424=CARTESIAN_POINT ( 'NONE',  ( 90.71510531252879161, -8.810647084079668900, 21.27078368671903164 ) ) ;
#5428=B_SPLINE_CURVE_WITH_KNOTS ( 'NONE', 3,
 ( #4403, #6643, #6906, #18890, #14757, #2930, #12768, #22887, #11039, #11532, #5057, #15278, #9295, #11664, #11405, #9165, #13410, #3309, #5433, #21534, #19527, #7038, #1443, #1311, #25793, #19407 ),
 .UNSPECIFIED., .F., .F.,
 ( 4, 2, 1, 2, 2, 2, 2, 2, 2, 2, 2, 1, 2, 4 ),
 ( -5.999999997206916261E-08, 0.0004354487530732705815, 0.0008709575061465131595, 0.001741975012292999074, 0.003484010024585964399, 0.006968080049171889410, 0.01045215007375781442, 0.01393622009834374030, 0.02090436014751559726, 0.02438843017210152314, 0.02613046518439449475, 0.02700148269054097883, 0.02743699144361421913, 0.02787250019668745596 ),
 .UNSPECIFIED. ) ;
#5429=B_SPLINE_CURVE_WITH_KNOTS ( 'NONE', 3,
 ( #26105, #26246, #16099, #14238, #11845, #17826, #22240, #24090, #25973, #11981 ),
 .UNSPECIFIED., .F., .F.,
 ( 4, 2, 2, 2, 4 ),
 ( 0.7921542097165071850, 0.8508620842112317728, 0.8814014469398914198, 0.9119408096685510667, 0.9406682828395843687 ),
 .UNSPECIFIED. ) ;
#5430=CARTESIAN_POINT ( 'NONE',  ( 121.8740240556052470, -26.81399039734623102, 11.10671848392256855 ) ) ;
#5431=CARTESIAN_POINT ( 'NONE',  ( 192.4448373802101173, 40.00000000000012790, -20.00000000003928236 ) ) ;
#5432=CARTESIAN_POINT ( 'NONE',  ( -86.96347745069644475, 5.999880687339585546E-14, -21.75974354311649961 ) ) ;
#5433=CARTESIAN_POINT ( 'NONE',  ( 20.59573805978977035, 47.74081960064699359, -13.93986955483940626 ) ) ;
#5434=CARTESIAN_POINT ( 'NONE',  ( -56.48582580120559982, 9.153146818113574668, 40.00000000000002132 ) ) ;
#5435=CARTESIAN_POINT ( 'NONE',  ( 90.68848423385740887, -8.814708749674085908, -21.28058941768224699 ) ) ;
#5437=CARTESIAN_POINT ( 'NONE',  ( -259.2033419157646676, 9.517827891722582478, 40.00000000000002132 ) ) ;
#5438=CARTESIAN_POINT ( 'NONE',  ( 151.7948205124835681, 33.23291073765556547, -40.00000000000002132 ) ) ;
#5439=CARTESIAN_POINT ( 'NONE',  ( 130.8568914410475372, -34.05028731879786363, 0.000000000000000000 ) ) ;
#5440=CARTESIAN_POINT ( 'NONE',  ( -105.3755690713226585, 40.00000000000019185, -18.24025645688310249 ) ) ;
#5441=CARTESIAN_POINT ( 'NONE',  ( 151.7948205124836534, -39.99999999999992184, -6.767089262349454515 ) ) ;
#5442=CARTESIAN_POINT ( 'NONE',  ( 158.3376637473630240, -26.51176758098464958, -10.98153369452720796 ) ) ;
#5444=CARTESIAN_POINT ( 'NONE',  ( -53.37769371643640426, -29.42719939405413854, 10.11111068829016801 ) ) ;
#5445=CARTESIAN_POINT ( 'NONE',  ( -1.087763065869005397, 47.95583523902985235, -13.97201973056374946 ) ) ;
#5446=CARTESIAN_POINT ( 'NONE',  ( 192.4448373802100889, -19.99999999996057198, -2.449293598294708485E-15 ) ) ;
#5448=CARTESIAN_POINT ( 'NONE',  ( -105.4732637872235728, -8.153770687239582315, 19.68494377761378544 ) ) ;
#5450=VERTEX_POINT ( 'NONE', #8119 ) ;
#5453=CARTESIAN_POINT ( 'NONE',  ( 140.2235668266255857, 12.60094438999845678, -30.42137084504298272 ) ) ;
#5458=CARTESIAN_POINT ( 'NONE',  ( -192.9588430854690273, 66.79921049721887982, 10.23066800229522677 ) ) ;
#5460=CARTESIAN_POINT ( 'NONE',  ( 184.8905102610680444, 1.070102760522089011E-13, -20.92133201514444352 ) ) ;
#5463=CARTESIAN_POINT ( 'NONE',  ( 98.29820294273055481, 14.14213562373424971, 14.14213562373465116 ) ) ;
#5464=CARTESIAN_POINT ( 'NONE',  ( 98.29820294267423719, -14.14213562374330024, 14.14213562372619926 ) ) ;
#5465=CARTESIAN_POINT ( 'NONE',  ( -198.0356074513804572, -39.99999999999948130, -55.37879056874863437 ) ) ;
#5466=CARTESIAN_POINT ( 'NONE',  ( -105.4741150117390447, -8.366608964578304608, 19.60045294983322961 ) ) ;
#5467=CARTESIAN_POINT ( 'NONE',  ( -86.96347745069644475, 15.38646221621793586, -15.38646221621778842 ) ) ;
#5468=CARTESIAN_POINT ( 'NONE',  ( 0.2972598230769957217, -4.999556039334937811E-14, 14.33493731733933352 ) ) ;
#5469=CARTESIAN_POINT ( 'NONE',  ( -114.4364955367336449, 20.04994829326807348, -8.644468109231272734 ) ) ;
#5470=CARTESIAN_POINT ( 'NONE',  ( 159.7744820660626317, 25.95909830917683792, 10.75261058663758540 ) ) ;
#5472=B_SPLINE_CURVE_WITH_KNOTS ( 'NONE', 3,
 ( #13441, #3336, #11436, #1347, #9449, #25693 ),
 .UNSPECIFIED., .F., .F.,
 ( 4, 2, 4 ),
 ( 0.0002283715791020996064, 0.004317053718188323432, 0.008405735857274547473 ),
 .UNSPECIFIED. ) ;
#5474=CARTESIAN_POINT ( 'NONE',  ( -192.9588430854689989, -10.23066800230756890, 10.23066800230742501 ) ) ;
#5475=CARTESIAN_POINT ( 'NONE',  ( 170.2234770963711128, -39.99999999999991473, -24.55285855007201334 ) ) ;
#5476=CARTESIAN_POINT ( 'NONE',  ( 130.8568914410475088, -24.07718906446910623, 32.49135343045471558 ) ) ;
#5477=CARTESIAN_POINT ( 'NONE',  ( 184.8905102610680444, -13.49065550809791603, -13.49065550809818781 ) ) ;
#5478=CARTESIAN_POINT ( 'NONE',  ( -144.0562696877137796, -14.68019673979266848, -29.54283206235778536 ) ) ;
#5479=CARTESIAN_POINT ( 'NONE',  ( 14.32711916788072770, 24.71075626504586609, 44.71189734681512107 ) ) ;
#5480=ORIENTED_EDGE ( 'NONE', *, *, #1775, .F. ) ;
#5481=CARTESIAN_POINT ( 'NONE',  ( 200.0000000000000000, 42.42640687119267540, 14.14213562373153543 ) ) ;
#5485=CARTESIAN_POINT ( 'NONE',  ( -105.3755690713226727, -2.472783935621397949E-13, 21.75974354311649961 ) ) ;
#5490=CARTESIAN_POINT ( 'NONE',  ( 4.995406935893289102, 55.24977328856464709, -40.00000000000002132 ) ) ;
#5491=CARTESIAN_POINT ( 'NONE',  ( -86.96347745069644475, 15.38646221621793586, -15.38646221621778842 ) ) ;
#5492=CARTESIAN_POINT ( 'NONE',  ( -162.0762913951020892, 39.99999999999985079, 41.69427287692695216 ) ) ;
#5493=CARTESIAN_POINT ( 'NONE',  ( 98.29820294267312875, 7.653668647304333383, -18.47759065023115355 ) ) ;
#5497=CARTESIAN_POINT ( 'NONE',  ( -213.1075012329537230, -40.00000000000025580, 53.71589010953650956 ) ) ;
#5499=CARTESIAN_POINT ( 'NONE',  ( 0.2972598230769883387, 39.99999999999997158, 14.33493731733947563 ) ) ;
#5501=FACE_OUTER_BOUND ( 'NONE', #1270, .T. ) ;
#5502=CARTESIAN_POINT ( 'NONE',  ( -100.7734535825088500, 16.03295912088740494, -40.53558337403661938 ) ) ;
#5504=CARTESIAN_POINT ( 'NONE',  ( -213.1075012329537230, -39.99999999999991473, -13.71589010951953647 ) ) ;
#5506=CARTESIAN_POINT ( 'NONE',  ( -91.56559293963836410, 22.67402823373189946, -0.000000000000000000 ) ) ;
#5507=CARTESIAN_POINT ( 'NONE',  ( -208.1127848780264742, -15.00245453012673202, -40.00000000000002132 ) ) ;
#5508=CARTESIAN_POINT ( 'NONE',  ( 14.38125909742181285, -10.73282306404727393, 10.73282306404716380 ) ) ;
#5509=CARTESIAN_POINT ( 'NONE',  ( 4.995406935893293543, -15.24977328854832592, 0.000000000000000000 ) ) ;
#5511=CARTESIAN_POINT ( 'NONE',  ( 136.1360204305621266, -3.419521671106983309E-13, 35.03383547441296741 ) ) ;
#5512=CARTESIAN_POINT ( 'NONE',  ( -30.26275506840325136, 57.76657404653985139, 1.198031551616126178 ) ) ;
#5513=CARTESIAN_POINT ( 'NONE',  ( 163.1118516004056573, 12.73709011382478273, 2.449293598294708485E-15 ) ) ;
#5515=CIRCLE ( 'NONE', #7624, 15.00000000000000178 ) ;
#5516=CARTESIAN_POINT ( 'NONE',  ( 90.68848816917943623, -21.08311784259292665, 9.291443204823380597 ) ) ;
#5517=CARTESIAN_POINT ( 'NONE',  ( -199.9999999999999432, -42.45148791632019680, -35.57044988732180002 ) ) ;
#5518=CARTESIAN_POINT ( 'NONE',  ( 91.82158438592158234, 44.40256751092336884, -12.16597498400043342 ) ) ;
#5519=CARTESIAN_POINT ( 'NONE',  ( -91.56559293963834989, -7.976292724337646577E-14, 17.32597176626811120 ) ) ;
#5520=CARTESIAN_POINT ( 'NONE',  ( -30.26275506840324070, 1.198031551616030033, -1.198031551616006496 ) ) ;
#5521=CARTESIAN_POINT ( 'NONE',  ( -30.26275506840324425, 1.694272468446254232, -40.00000000000002132 ) ) ;
#5524=CARTESIAN_POINT ( 'NONE',  ( -77.55658273862232477, -1.402866402507712218, -22.13039188814530789 ) ) ;
#5525=CARTESIAN_POINT ( 'NONE',  ( 57.59792236341147031, -1.722363176415055985, 1.722363176415024677 ) ) ;
#5526=CARTESIAN_POINT ( 'NONE',  ( 130.8568914410475088, 24.07718906446937623, -32.49135343045455215 ) ) ;
#5528=FACE_OUTER_BOUND ( 'NONE', #14582, .T. ) ;
#5529=CARTESIAN_POINT ( 'NONE',  ( 19.06497207195981147, 1.521599808664285085E-13, -14.19242893257840521 ) ) ;
#5530=CARTESIAN_POINT ( 'NONE',  ( 4.995406935893300648, -10.78321810387790514, -67.35176059880241439 ) ) ;
#5531=CARTESIAN_POINT ( 'NONE',  ( -280.0000000000000568, 14.14213562373127431, -42.42640687119274645 ) ) ;
#5532=CARTESIAN_POINT ( 'NONE',  ( 19.06497207195981858, 10.03556273973516078, -66.60410523465806421 ) ) ;
#5533=CARTESIAN_POINT ( 'NONE',  ( 19.06497207195980792, 10.03556273973447155, -10.03556273973422286 ) ) ;
#5537=CARTESIAN_POINT ( 'NONE',  ( 151.7948205124836534, -39.99999999999987921, -33.23291073765567916 ) ) ;
#5538=CARTESIAN_POINT ( 'NONE',  ( 19.06497207195981858, -10.03556273973469715, 66.60410523465813526 ) ) ;
#5540=CARTESIAN_POINT ( 'NONE',  ( -86.96347745069644475, 18.24025645688350750, 40.00000000000002132 ) ) ;
#5542=CARTESIAN_POINT ( 'NONE',  ( -213.1075012329537230, 9.698598906450410340, 9.698598906450483170 ) ) ;
#5543=CARTESIAN_POINT ( 'NONE',  ( -70.70793901134142345, 22.66153234904986746, 9.386714043133100205 ) ) ;
#5544=CARTESIAN_POINT ( 'NONE',  ( 23.58679727196918918, 23.29637218066034521, 42.79169916605225410 ) ) ;
#5545=CARTESIAN_POINT ( 'NONE',  ( -280.0000000000000568, -20.00000000000006750, 40.00000000000002132 ) ) ;
#5547=CARTESIAN_POINT ( 'NONE',  ( -194.4222775680590871, -48.65439176089972051, 14.07715774765395267 ) ) ;
#5549=CARTESIAN_POINT ( 'NONE',  ( 23.36927571439213480, -13.80130822340191443, 46.80992244775416111 ) ) ;
#5550=CARTESIAN_POINT ( 'NONE',  ( 20.16956056503097372, 13.95858718339115434, -47.86583268168163130 ) ) ;
#5553=CARTESIAN_POINT ( 'NONE',  ( -93.02511667906934179, -20.50052124204830406, -8.946512270084891583 ) ) ;
#5554=CARTESIAN_POINT ( 'NONE',  ( -162.0762913951020892, -3.568845385355699554E-14, 1.694272876828323948 ) ) ;
#5555=CARTESIAN_POINT ( 'NONE',  ( 151.7948205124836250, 1.439163438361279259E-13, -33.23291073765553705 ) ) ;
#5558=CARTESIAN_POINT ( 'NONE',  ( -238.4067589809705794, -40.96449428006345528, 40.00000000000002132 ) ) ;
#5560=CARTESIAN_POINT ( 'NONE',  ( 83.06440094991440048, -9.006081069352781299, -24.44702070095364377 ) ) ;
#5563=CARTESIAN_POINT ( 'NONE',  ( 192.4448373802100889, 20.00000000003945644, 0.000000000000000000 ) ) ;
#5564=CARTESIAN_POINT ( 'NONE',  ( -86.96347745069645896, 21.75974354311648895, -0.000000000000000000 ) ) ;
#5566=CARTESIAN_POINT ( 'NONE',  ( -100.7734535825088358, -22.67402823373193499, 0.000000000000000000 ) ) ;
#5567=CARTESIAN_POINT ( 'NONE',  ( -208.1127848780265026, 5.403397259664334602E-13, -55.00245453012672670 ) ) ;
#5568=CARTESIAN_POINT ( 'NONE',  ( 163.1118516004056573, -2.556006622855449647E-13, 27.26290988616872824 ) ) ;
#5569=CARTESIAN_POINT ( 'NONE',  ( -238.4067589809705794, -0.6820004457913585449, -0.6820004457913265705 ) ) ;
#5570=EDGE_CURVE ( 'NONE', #22478, #19077, #3683, .T. ) ;
#5572=ORIENTED_EDGE ( 'NONE', *, *, #17908, .F. ) ;
#5575=CARTESIAN_POINT ( 'NONE',  ( -188.2995950289364089, 46.99046209955525200, -13.82811170417133617 ) ) ;
#5578=CARTESIAN_POINT ( 'NONE',  ( -89.92902785008901390, -20.17328762787336061, 8.734793929541309510 ) ) ;
#5579=CARTESIAN_POINT ( 'NONE',  ( 22.01478053668312640, -47.29427690643675675, -13.87318432394964773 ) ) ;
#5580=VERTEX_POINT ( 'NONE', #11841 ) ;
#5581=CARTESIAN_POINT ( 'NONE',  ( 4.995406935893288214, 15.24977328854832770, -40.00000000000002132 ) ) ;
#5583=ORIENTED_EDGE ( 'NONE', *, *, #9954, .F. ) ;
#5587=CARTESIAN_POINT ( 'NONE',  ( -91.56559293963834989, 12.25131212657480440, 12.25131212657486834 ) ) ;
#5589=CARTESIAN_POINT ( 'NONE',  ( 19.06497207195981147, -4.605042221739098431E-14, 14.19242893257840521 ) ) ;
#5592=CARTESIAN_POINT ( 'NONE',  ( -259.2033419157646676, -1.438356298054549103E-14, -9.517827891722632216 ) ) ;
#5593=CARTESIAN_POINT ( 'NONE',  ( -30.26275506840324070, 1.218738420030236455E-14, -1.694272468446259783 ) ) ;
#5594=CARTESIAN_POINT ( 'NONE',  ( 151.7948205124836534, -39.99999999999992184, -6.767089262349454515 ) ) ;
#5595=CARTESIAN_POINT ( 'NONE',  ( -200.0000000000000000, -45.06067021511792348, -22.35311919176578499 ) ) ;
#5596=CARTESIAN_POINT ( 'NONE',  ( -100.7734535825088500, 16.03295912088713848, -16.03295912088698927 ) ) ;
#5597=DIRECTION ( 'NONE',  ( -0.01051738777841000790, -0.3995761382614314572, 0.9166396752739868203 ) ) ;
#5598=CARTESIAN_POINT ( 'NONE',  ( 184.8905102610680444, -41.77492675555986779, -14.79361573936407304 ) ) ;
#5601=CARTESIAN_POINT ( 'NONE',  ( 192.4448373802100889, -1.741373372144848397E-13, 20.00000000003942091 ) ) ;
#5602=CARTESIAN_POINT ( 'NONE',  ( 151.7948205124836534, -39.99999999999987921, -33.23291073765567916 ) ) ;
#5603=CARTESIAN_POINT ( 'NONE',  ( -208.1127848780265026, 38.89260858015724409, 38.89260858015741462 ) ) ;
#5605=CARTESIAN_POINT ( 'NONE',  ( -280.0000000000000000, 14.14213562373078581, 14.14213562373108424 ) ) ;
#5606=CARTESIAN_POINT ( 'NONE',  ( -194.7884774423998238, -18.40784251728203458, -44.44046305925559892 ) ) ;
#5607=CARTESIAN_POINT ( 'NONE',  ( 146.6084372240433993, -3.357462877844280890E-13, 34.62501878078305850 ) ) ;
#5608=ORIENTED_EDGE ( 'NONE', *, *, #21741, .F. ) ;
#5609=CARTESIAN_POINT ( 'NONE',  ( 130.8568914410475088, 32.49135343045448820, 24.07718906446946860 ) ) ;
#5610=CARTESIAN_POINT ( 'NONE',  ( -208.1127848780265026, -15.00245453012673202, 0.000000000000000000 ) ) ;
#5612=CARTESIAN_POINT ( 'NONE',  ( -56.48582580120559982, -6.472252184283581400, -50.09629031063973059 ) ) ;
#5613=CARTESIAN_POINT ( 'NONE',  ( -86.86493150570900923, 7.943527260525790723, 19.77569912837828880 ) ) ;
#5614=ORIENTED_EDGE ( 'NONE', *, *, #16291, .F. ) ;
#5617=CARTESIAN_POINT ( 'NONE',  ( -0.5869797817581398069, 18.21245090265434996, 43.96874597320426403 ) ) ;
#5618=EDGE_LOOP ( 'NONE', ( #9317, #7959, #10627, #13945 ) ) ;
#5619=ORIENTED_EDGE ( 'NONE', *, *, #5245, .T. ) ;
#5620=CARTESIAN_POINT ( 'NONE',  ( 57.59792236341147031, 37.56421063658187620, 2.449293598294708485E-15 ) ) ;
#5621=CARTESIAN_POINT ( 'NONE',  ( -259.2033419157646676, 6.730120644403521979, -6.730120644403498886 ) ) ;
#5622=CARTESIAN_POINT ( 'NONE',  ( -91.56559293963836410, 39.99999999999994316, 17.32597176626825330 ) ) ;
#5625=CARTESIAN_POINT ( 'NONE',  ( 4.995406935893283773, 40.00000000000017764, -15.24977328854790848 ) ) ;
#5627=CARTESIAN_POINT ( 'NONE',  ( -170.8329924482306410, 37.82183460435096123, 15.66631684693926907 ) ) ;
#5628=CARTESIAN_POINT ( 'NONE',  ( 2.303792037523120673, -18.40682559463839496, -44.43800799080462127 ) ) ;
#5629=CARTESIAN_POINT ( 'NONE',  ( -30.26275506840323359, -1.198031551615522439, -57.76657404653986561 ) ) ;
#5630=CARTESIAN_POINT ( 'NONE',  ( -77.59261320674056606, -21.93453874212654853, 2.779275804850804388 ) ) ;
#5632=CARTESIAN_POINT ( 'NONE',  ( -105.3895334812064988, -20.30817960290562141, -6.678845697774401735 ) ) ;
#5633=CARTESIAN_POINT ( 'NONE',  ( 91.82158438592159655, -22.79471317813468900, 40.00000000000002132 ) ) ;
#5634=CARTESIAN_POINT ( 'NONE',  ( 136.1360204305621266, -4.966164525587039691, -2.449293598294708485E-15 ) ) ;
#5635=CARTESIAN_POINT ( 'NONE',  ( 91.82158438592158234, 12.16597498397773869, -12.16597498397759303 ) ) ;
#5636=CARTESIAN_POINT ( 'NONE',  ( 151.7948205124836250, 33.23291073765556547, 0.000000000000000000 ) ) ;
#5637=CARTESIAN_POINT ( 'NONE',  ( -105.5018627849130723, 19.74131065641399729, 7.980562150497299001 ) ) ;
#5638=EDGE_CURVE ( 'NONE', #24441, #2026, #20384, .T. ) ;
#5639=CARTESIAN_POINT ( 'NONE',  ( 163.1118516004056573, -2.556006622855449647E-13, 27.26290988616872824 ) ) ;
#5640=CARTESIAN_POINT ( 'NONE',  ( -213.1075012329537230, 66.26714140136188291, 9.698598906438215650 ) ) ;
#5641=CARTESIAN_POINT ( 'NONE',  ( -100.7734535825088358, 17.32597176626809343, 2.449293598294708485E-15 ) ) ;
#5643=CARTESIAN_POINT ( 'NONE',  ( 98.29820294267354086, -18.47759065023110736, 7.653668647303992323 ) ) ;
#5644=FACE_OUTER_BOUND ( 'NONE', #2789, .T. ) ;
#5645=CARTESIAN_POINT ( 'NONE',  ( 136.1360204305621551, 3.511608612530801032, -53.05693388239316022 ) ) ;
#5646=CARTESIAN_POINT ( 'NONE',  ( 151.7948205124836250, 1.807796684091926154E-15, 6.767089262349031742 ) ) ;
#5647=CARTESIAN_POINT ( 'NONE',  ( -198.0356074513804572, 10.87444709759730088, -10.87444709759707173 ) ) ;
#5649=EDGE_CURVE ( 'NONE', #19014, #6051, #9567, .T. ) ;
#5650=CARTESIAN_POINT ( 'NONE',  ( 4.995406935893288214, 15.24977328854832770, -40.00000000000002132 ) ) ;
#5653=CARTESIAN_POINT ( 'NONE',  ( -77.59243545043536017, 2.773626963377854526, -21.93550214427983391 ) ) ;
#5654=B_SPLINE_CURVE_WITH_KNOTS ( 'NONE', 3,
 ( #14116, #4018, #2149, #148, #7717, #2023, #3743, #15827, #24093, #11848, #12118, #20243, #19969, #10125, #1750, #5868 ),
 .UNSPECIFIED., .F., .F.,
 ( 4, 2, 2, 2, 2, 2, 2, 4 ),
 ( 1.329418552447366687E-15, 0.004250215530321975466, 0.006375323295482298799, 0.008500431060642620398, 0.01275064659096327400, 0.01381320047354344174, 0.01487575435612360948, 0.01700086212128394322 ),
 .UNSPECIFIED. ) ;
#5655=CARTESIAN_POINT ( 'NONE',  ( 170.2234770963711128, -17.36149277827010096, 17.36149277826970660 ) ) ;
#5656=CARTESIAN_POINT ( 'NONE',  ( 0.2972598230770100991, -38.42060263243632079, -38.42060263243699580 ) ) ;
#5657=CARTESIAN_POINT ( 'NONE',  ( -114.7505577291900352, 21.95690638031361530, -2.633416689372234831 ) ) ;
#5658=CARTESIAN_POINT ( 'NONE',  ( -213.1075012329537230, 1.045191102001431893E-13, -13.71589010951911902 ) ) ;
#5659=CARTESIAN_POINT ( 'NONE',  ( -238.4067589809705794, -28.96627169325303797, -28.96627169325349627 ) ) ;
#5660=CARTESIAN_POINT ( 'NONE',  ( 14.38125909742182529, -39.01709431150879936, -39.01709431150948859 ) ) ;
#5661=CARTESIAN_POINT ( 'NONE',  ( -30.26275506840324070, 1.198031551616724366, -57.76657404653984429 ) ) ;
#5662=CARTESIAN_POINT ( 'NONE',  ( -86.96347745069644475, -43.67073346367964604, -12.89780903124457545 ) ) ;
#5666=CARTESIAN_POINT ( 'NONE',  ( 163.1118516004056573, 1.251511021549353291E-13, -27.26290988616872824 ) ) ;
#5667=CARTESIAN_POINT ( 'NONE',  ( -105.3755690713226585, 43.67073346367970288, 12.89780903124427702 ) ) ;
#5669=CARTESIAN_POINT ( 'NONE',  ( -162.0762913951021176, 1.694272876828294194, 40.00000000000002132 ) ) ;
#5671=CARTESIAN_POINT ( 'NONE',  ( -198.0356074513804572, 39.15871834505912119, -17.40982414986464377 ) ) ;
#5672=FACE_OUTER_BOUND ( 'NONE', #12887, .T. ) ;
#5674=CARTESIAN_POINT ( 'NONE',  ( 19.06497207195980792, 14.19242893257840876, 0.000000000000000000 ) ) ;
#5676=CARTESIAN_POINT ( 'NONE',  ( -3.971463587461111722, 23.46415232638922888, -43.02522237042865072 ) ) ;
#5678=CARTESIAN_POINT ( 'NONE',  ( -3.379936260373897383, -17.94397654175175560, 43.32059152999903517 ) ) ;
#5680=CARTESIAN_POINT ( 'NONE',  ( 20.91285618074644503, 23.84652503048867089, -43.54130497317085968 ) ) ;
#5683=CARTESIAN_POINT ( 'NONE',  ( 136.1360204305621266, 1.473277640373554421E-13, -35.03383547441296741 ) ) ;
#5685=CARTESIAN_POINT ( 'NONE',  ( -91.56559293963834989, 40.53558337403654832, 16.03295912088756481 ) ) ;
#5686=CARTESIAN_POINT ( 'NONE',  ( 136.1360204305621266, -4.966164525587039691, -2.449293598294708485E-15 ) ) ;
#5687=CARTESIAN_POINT ( 'NONE',  ( 59.93546481446576024, -13.19882033562139512, -31.86477106152662131 ) ) ;
#5689=CARTESIAN_POINT ( 'NONE',  ( -198.0356074513804572, 10.87444709759730088, -10.87444709759707173 ) ) ;
#5690=CARTESIAN_POINT ( 'NONE',  ( -30.26275506840324070, -1.694272468446265112, 0.000000000000000000 ) ) ;
#5691=CARTESIAN_POINT ( 'NONE',  ( 184.8905102610680444, -20.92133201514440799, 40.00000000000002132 ) ) ;
#5692=CARTESIAN_POINT ( 'NONE',  ( -280.0000000000000568, -39.99999999999987210, -20.00000000000043343 ) ) ;
#5693=CARTESIAN_POINT ( 'NONE',  ( 98.29820294267351244, -10.58389073158543958, 16.98253775142841704 ) ) ;
#5694=CARTESIAN_POINT ( 'NONE',  ( -259.2033419157646676, 6.730120644403426944, 6.730120644403592145 ) ) ;
#5696=CARTESIAN_POINT ( 'NONE',  ( 98.29820294267170766, 13.21553301702797789, -15.06873823044322869 ) ) ;
#5697=CARTESIAN_POINT ( 'NONE',  ( -105.3755690713226869, 21.75974354311648540, -0.000000000000000000 ) ) ;
#5698=CARTESIAN_POINT ( 'NONE',  ( -103.9650464695103551, -8.298274100672328402, 20.03380587528770462 ) ) ;
#5700=ORIENTED_EDGE ( 'NONE', *, *, #12057, .T. ) ;
#5701=ORIENTED_EDGE ( 'NONE', *, *, #25271, .T. ) ;
#5702=CARTESIAN_POINT ( 'NONE',  ( -280.0000000000000568, -14.14213562373078226, -42.42640687119295251 ) ) ;
#5703=CARTESIAN_POINT ( 'NONE',  ( 22.50777602749823814, -43.24633676485594691, -17.91321921096134417 ) ) ;
#5705=CARTESIAN_POINT ( 'NONE',  ( 57.59792236341147031, -2.435789363418150000, -40.00000000000002132 ) ) ;
#5706=B_SPLINE_CURVE_WITH_KNOTS ( 'NONE', 3,
 ( #12677, #2851, #14801, #17189, #18804, #7084, #25068, #3099, #19066, #23195, #15198, #4976 ),
 .UNSPECIFIED., .F., .F.,
 ( 4, 2, 2, 2, 2, 4 ),
 ( 5.597004042492164534E-17, 0.005971690550335823772, 0.008957535825503749535, 0.01045045846308766992, 0.01119691978187959194, 0.01194338110067151397 ),
 .UNSPECIFIED. ) ;
#5708=EDGE_CURVE ( 'NONE', #14842, #19288, #16554, .T. ) ;
#5709=ORIENTED_EDGE ( 'NONE', *, *, #8830, .F. ) ;
#5711=DIRECTION ( 'NONE',  ( -0.3301743741156225598, 0.000000000000000000, -0.9439199556516204570 ) ) ;
#5712=CARTESIAN_POINT ( 'NONE',  ( 91.82158438592158234, 16.11829626346139577, 16.11829626346143840 ) ) ;
#5713=ADVANCED_FACE ( 'NONE', ( #22892 ), #6837, .T. ) ;
#5714=SPHERICAL_SURFACE ( 'NONE', #9315, 15.00000000000000000 ) ;
#5715=CARTESIAN_POINT ( 'NONE',  ( -30.26275506840324070, -1.147469862568086380E-14, 1.694272468446259783 ) ) ;
#5716=CARTESIAN_POINT ( 'NONE',  ( 91.82158438592158234, -17.20528682183298486, 0.000000000000000000 ) ) ;
#5722=CARTESIAN_POINT ( 'NONE',  ( 163.1118516004056573, -40.00000000000027711, 27.26290988616830546 ) ) ;
#5723=CARTESIAN_POINT ( 'NONE',  ( -110.0471271032161553, -8.580892274476465076, 18.26740471935241672 ) ) ;
#5724=CARTESIAN_POINT ( 'NONE',  ( -135.8532207217289738, -21.81201906317788186, 21.81201906317762962 ) ) ;
#5725=CARTESIAN_POINT ( 'NONE',  ( -56.48582580120559982, 9.153146818113574668, -40.00000000000002132 ) ) ;
#5726=CARTESIAN_POINT ( 'NONE',  ( -198.0356074513804572, -39.15871834505905724, -17.40982414986491733 ) ) ;
#5728=CARTESIAN_POINT ( 'NONE',  ( -77.90255099906772784, 20.04994828523968664, -8.644468104261312291 ) ) ;
#5730=CARTESIAN_POINT ( 'NONE',  ( -56.48582580120559271, 2.158176344243877536E-14, -9.153146818113587102 ) ) ;
#5731=CARTESIAN_POINT ( 'NONE',  ( 19.06497207195980792, 66.60410523465817789, 10.03556273973446800 ) ) ;
#5732=CARTESIAN_POINT ( 'NONE',  ( -105.3755690713226727, 15.38646221621771737, 15.38646221621800514 ) ) ;
#5733=CARTESIAN_POINT ( 'NONE',  ( -188.2957210513761197, -13.82790368522227986, -46.98905903629284353 ) ) ;
#5734=CARTESIAN_POINT ( 'NONE',  ( -259.2033419157646676, -21.55415060305824326, -35.01439189186556433 ) ) ;
#5735=ORIENTED_EDGE ( 'NONE', *, *, #26147, .T. ) ;
#5736=CARTESIAN_POINT ( 'NONE',  ( 136.1360204305621266, -24.77266263493151044, 24.77266263493093135 ) ) ;
#5737=CARTESIAN_POINT ( 'NONE',  ( -208.1127848780265026, -10.60833733269551971, 10.60833733269537049 ) ) ;
#5739=DIRECTION ( 'NONE',  ( 0.3301743741186746739, 0.9439199556505528665, 0.000000000000000000 ) ) ;
#5740=CARTESIAN_POINT ( 'NONE',  ( 170.2234770963711128, -45.64576402573167258, -10.92277846919254891 ) ) ;
#5741=CARTESIAN_POINT ( 'NONE',  ( 73.43374839995014725, -26.88865971588853299, 12.96823619005398420 ) ) ;
#5742=AXIS2_PLACEMENT_3D ( 'NONE', #3908, #24654, #8404 ) ;
#5743=ORIENTED_EDGE ( 'NONE', *, *, #23766, .T. ) ;
#5745=CARTESIAN_POINT ( 'NONE',  ( 23.09861257792919176, -23.40165480222906069, 42.94075326233394918 ) ) ;
#5746=CARTESIAN_POINT ( 'NONE',  ( -4.201409602820223910, 23.41774994521163222, 42.95750343186378473 ) ) ;
#5750=CARTESIAN_POINT ( 'NONE',  ( -208.1127848780264742, 15.00245453012665742, -40.00000000000002132 ) ) ;
#5751=CARTESIAN_POINT ( 'NONE',  ( -162.0762913951020892, -1.198031840385783919, 1.198031840385741731 ) ) ;
#5752=CARTESIAN_POINT ( 'NONE',  ( 19.06497207195979726, 39.99999999999997158, 14.19242893257854554 ) ) ;
#5755=DIRECTION ( 'NONE',  ( 0.7071067811865441310, -0.7071067811865507924, 8.659560562354974766E-17 ) ) ;
#5756=FACE_OUTER_BOUND ( 'NONE', #10224, .T. ) ;
#5759=CIRCLE ( 'NONE', #1104, 15.00000000000000533 ) ;
#5761=CARTESIAN_POINT ( 'NONE',  ( -144.0562564038984021, 10.50946916234533468, 31.27039870030377244 ) ) ;
#5762=CARTESIAN_POINT ( 'NONE',  ( -4.260882601031005912, -13.81249720866826358, -46.91379881627400295 ) ) ;
#5763=CARTESIAN_POINT ( 'NONE',  ( -91.56559293963834989, -12.25131212657475466, -12.25131212657495361 ) ) ;
#5765=CARTESIAN_POINT ( 'NONE',  ( 0.2972598230770027716, -38.42060263243656237, -18.14793986248737667 ) ) ;
#5766=CARTESIAN_POINT ( 'NONE',  ( -105.3755690713226727, -2.472783935621397949E-13, 21.75974354311649961 ) ) ;
#5768=CARTESIAN_POINT ( 'NONE',  ( -208.1127848780265026, -10.60833733269537227, -10.60833733269551793 ) ) ;
#5769=CARTESIAN_POINT ( 'NONE',  ( -162.0762913951020607, -41.69427287682838568, -2.449293598294708485E-15 ) ) ;
#5771=CARTESIAN_POINT ( 'NONE',  ( -259.2033419157646676, 35.01439189186528722, 21.55415060305857011 ) ) ;
#5772=CARTESIAN_POINT ( 'NONE',  ( -56.48582580120557850, -30.84685318188645198, -2.449293598294708485E-15 ) ) ;
#5773=CARTESIAN_POINT ( 'NONE',  ( -110.0968994563038450, 12.50898707784705088, 15.90535099103004768 ) ) ;
#5775=CARTESIAN_POINT ( 'NONE',  ( 4.995406935893290878, 1.606505379428369110E-13, -15.24977328854832592 ) ) ;
#5776=CARTESIAN_POINT ( 'NONE',  ( 136.1360204305621551, 3.511608612530801032, -53.05693388239316022 ) ) ;
#5777=CARTESIAN_POINT ( 'NONE',  ( 192.4448373802101173, -20.00000000003938538, -40.00000000000002132 ) ) ;
#5778=ORIENTED_EDGE ( 'NONE', *, *, #8487, .T. ) ;
#5779=CARTESIAN_POINT ( 'NONE',  ( 23.42154907652890472, -42.84253412640328662, 23.32998349128528304 ) ) ;
#5781=CARTESIAN_POINT ( 'NONE',  ( 133.2080217031554810, 12.38638889282702671, 29.90338805389126264 ) ) ;
#5782=CARTESIAN_POINT ( 'NONE',  ( 14.38125909742180220, 39.01709431150916885, -17.55144818341463164 ) ) ;
#5783=CARTESIAN_POINT ( 'NONE',  ( 200.0000000000000000, -39.99999999999991473, -20.00000000000024514 ) ) ;
#5784=CARTESIAN_POINT ( 'NONE',  ( -162.0762913951020892, 1.198031840385732849, -1.198031840385733515 ) ) ;
#5785=CARTESIAN_POINT ( 'NONE',  ( -135.8532207217289738, -9.153146818113595984, 0.000000000000000000 ) ) ;
#5786=CARTESIAN_POINT ( 'NONE',  ( 151.7948205124836534, 6.767089262349062828, -40.00000000000002132 ) ) ;
#5787=CARTESIAN_POINT ( 'NONE',  ( 170.0000000000000000, 24.95097643317004099, -3.062538285713088282 ) ) ;
#5790=CARTESIAN_POINT ( 'NONE',  ( -100.7734535825088358, 12.25131212657497848, -12.25131212657469604 ) ) ;
#5791=CARTESIAN_POINT ( 'NONE',  ( -86.96347745069645896, -12.89780903124443689, 43.67073346367968156 ) ) ;
#5792=CARTESIAN_POINT ( 'NONE',  ( -105.2302824411781330, 21.33128297465077594, -2.585500233827331851 ) ) ;
#5793=CARTESIAN_POINT ( 'NONE',  ( -87.10570614286989155, 13.14378919785584010, -16.99508527299807170 ) ) ;
#5794=CARTESIAN_POINT ( 'NONE',  ( 200.0000000000000000, 14.14213562373142352, -42.42640687119268961 ) ) ;
#5795=CIRCLE ( 'NONE', #20687, 60.00000000000000000 ) ;
#5796=CARTESIAN_POINT ( 'NONE',  ( 199.9999999999999432, -14.14213562373073607, -14.14213562373102206 ) ) ;
#5797=CARTESIAN_POINT ( 'NONE',  ( -86.86493150571111244, 8.366608963953098055, -19.60045294882791467 ) ) ;
#5798=CARTESIAN_POINT ( 'NONE',  ( -135.8532207217289738, -6.472252184284280396, 6.472252184284099208 ) ) ;
#5799=CARTESIAN_POINT ( 'NONE',  ( 130.8568914410475372, -34.05028731879786363, 0.000000000000000000 ) ) ;
#5802=CARTESIAN_POINT ( 'NONE',  ( 163.1118516004056573, -39.99999999999990052, -27.26290988616886679 ) ) ;
#5803=CARTESIAN_POINT ( 'NONE',  ( 200.0000000000000000, 42.42640687119290988, 14.14213562373111976 ) ) ;
#5805=CARTESIAN_POINT ( 'NONE',  ( 200.0000000000000000, 19.99999999999995737, 40.00000000000002132 ) ) ;
#5807=EDGE_CURVE ( 'NONE', #2026, #12388, #20258, .T. ) ;
#5808=CARTESIAN_POINT ( 'NONE',  ( 1.564253033640332413, -24.39614062124443450, -44.28527310957341712 ) ) ;
#5810=CARTESIAN_POINT ( 'NONE',  ( 12.71631587212106140, 43.65709841108841260, 18.08336225573125944 ) ) ;
#5811=CARTESIAN_POINT ( 'NONE',  ( 27.55177309534125385, 22.48880744263714959, 41.56868263113059925 ) ) ;
#5812=CARTESIAN_POINT ( 'NONE',  ( 4.995406935893288214, 15.24977328854832770, 0.000000000000000000 ) ) ;
#5814=CARTESIAN_POINT ( 'NONE',  ( -188.9478457324744056, -43.31767415847494362, 17.94276812689867029 ) ) ;
#5815=B_SPLINE_CURVE_WITH_KNOTS ( 'NONE', 3,
 ( #11782, #3411, #9658, #1170, #23632, #19762, #13770, #17892, #23887, #1553 ),
 .UNSPECIFIED., .F., .F.,
 ( 4, 2, 2, 2, 4 ),
 ( 0.7921542097164249174, 0.8508620842112317728, 0.8814014469398914198, 0.9119408096685510667, 0.9406682828395580565 ),
 .UNSPECIFIED. ) ;
#5817=CARTESIAN_POINT ( 'NONE',  ( 8.556015491684524576, -14.17785852676789560, 49.31947911770178195 ) ) ;
#5818=ADVANCED_FACE ( 'NONE', ( #2070 ), #17015, .T. ) ;
#5820=CARTESIAN_POINT ( 'NONE',  ( 23.35928221536259386, 13.80178577956188768, -46.81377789283278190 ) ) ;
#5823=CARTESIAN_POINT ( 'NONE',  ( -183.6285492669661323, -17.34367427885804247, 41.87133366546909485 ) ) ;
#5824=CIRCLE ( 'NONE', #15112, 15.00000000000000000 ) ;
#5825=CARTESIAN_POINT ( 'NONE',  ( 130.8568914410475088, 32.49135343045448820, 24.07718906446946860 ) ) ;
#5826=CARTESIAN_POINT ( 'NONE',  ( -100.7734535825088500, -17.32597176626813251, 40.00000000000002132 ) ) ;
#5828=CARTESIAN_POINT ( 'NONE',  ( -280.0000000000000000, -14.14213562373118549, 14.14213562373078936 ) ) ;
#5829=CARTESIAN_POINT ( 'NONE',  ( -30.26275506840324070, -1.694272468446265112, 0.000000000000000000 ) ) ;
#5830=CARTESIAN_POINT ( 'NONE',  ( 192.4448373802100889, 20.00000000003945644, 0.000000000000000000 ) ) ;
#5831=CARTESIAN_POINT ( 'NONE',  ( -86.96347745069644475, -21.75974354311652093, 40.00000000000002132 ) ) ;
#5832=CARTESIAN_POINT ( 'NONE',  ( -192.9588430854689989, 5.375290060580374156E-13, -54.46834944099972375 ) ) ;
#5833=CARTESIAN_POINT ( 'NONE',  ( -198.0356074513804572, 1.247057299367198800E-13, -15.37879056873070560 ) ) ;
#5834=CARTESIAN_POINT ( 'NONE',  ( -86.96347745069644475, 15.38646221621772092, 15.38646221621800336 ) ) ;
#5836=CARTESIAN_POINT ( 'NONE',  ( 200.0000000000000000, 7.347880794884121511E-14, 0.000000000000000000 ) ) ;
#5837=CARTESIAN_POINT ( 'NONE',  ( -91.56559293963836410, 22.67402823373189946, -0.000000000000000000 ) ) ;
#5838=CARTESIAN_POINT ( 'NONE',  ( -192.1166648175281182, 48.16216898722869644, -14.00295691731063030 ) ) ;
#5840=EDGE_LOOP ( 'NONE', ( #10170, #12344, #11680, #5700 ) ) ;
#5841=VERTEX_POINT ( 'NONE', #11238 ) ;
#5842=CARTESIAN_POINT ( 'NONE',  ( -213.1075012329537230, -37.98287015391232302, -18.58567234101164800 ) ) ;
#5843=CARTESIAN_POINT ( 'NONE',  ( 23.39921416754908279, -46.79910576274356515, -13.79910252519598934 ) ) ;
#5844=ORIENTED_EDGE ( 'NONE', *, *, #9776, .F. ) ;
#5845=CARTESIAN_POINT ( 'NONE',  ( 91.82158438592158234, -17.20528682183298486, -40.00000000000002132 ) ) ;
#5846=CARTESIAN_POINT ( 'NONE',  ( 170.0000000000000000, 1.183443619805854272E-13, -24.95097643317000546 ) ) ;
#5847=ORIENTED_EDGE ( 'NONE', *, *, #14110, .T. ) ;
#5849=CARTESIAN_POINT ( 'NONE',  ( -105.2054292635175727, 21.49321519473981823, -0.6786951374309612151 ) ) ;
#5850=CARTESIAN_POINT ( 'NONE',  ( -238.4067589809705794, 0.6820004457912757223, 0.6820004457913219076 ) ) ;
#5851=CARTESIAN_POINT ( 'NONE',  ( -189.5227851116976581, -43.46196956062707528, -18.00253723946215700 ) ) ;
#5852=CARTESIAN_POINT ( 'NONE',  ( -30.26275506840323359, -40.00000000000017053, 41.69427246844613677 ) ) ;
#5853=CARTESIAN_POINT ( 'NONE',  ( -105.3755690713226585, 18.24025645688349684, 40.00000000000002132 ) ) ;
#5855=CARTESIAN_POINT ( 'NONE',  ( -114.4364955367314991, -8.644468109207263495, -20.04994829327655737 ) ) ;
#5856=CARTESIAN_POINT ( 'NONE',  ( 19.06497207195981858, -40.00000000000007105, 14.19242893257826665 ) ) ;
#5857=CARTESIAN_POINT ( 'NONE',  ( -100.7734535825088500, -40.00000000000027711, 22.67402823373149801 ) ) ;
#5859=CARTESIAN_POINT ( 'NONE',  ( -135.8532207217289738, 6.472252184283881604, 50.09629031063969506 ) ) ;
#5860=CARTESIAN_POINT ( 'NONE',  ( 19.06497207195981503, -14.19242893257840166, 0.000000000000000000 ) ) ;
#5861=CARTESIAN_POINT ( 'NONE',  ( 200.0000000000000000, -14.14213562373062949, -42.42640687119301646 ) ) ;
#5865=CARTESIAN_POINT ( 'NONE',  ( -280.0000000000000000, -2.609240458947769655E-13, 20.00000000000001421 ) ) ;
#5866=CARTESIAN_POINT ( 'NONE',  ( 200.0000000000000000, -39.99999999999991473, -20.00000000000024514 ) ) ;
#5867=CARTESIAN_POINT ( 'NONE',  ( 146.6084372240433709, 32.08495691632064961, -24.48358557860320417 ) ) ;
#5868=CARTESIAN_POINT ( 'NONE',  ( -114.4364955367322949, 8.644468109217019247, 20.04994829327305794 ) ) ;
#5869=CARTESIAN_POINT ( 'NONE',  ( -188.3066136396996058, -23.45085387054324144, -43.00728998844858353 ) ) ;
#5870=CARTESIAN_POINT ( 'NONE',  ( -162.0762913951020892, -1.198031840385783919, 1.198031840385741731 ) ) ;
#5872=CARTESIAN_POINT ( 'NONE',  ( 14.38125909742181285, -17.55144818341421598, -39.01709431150935359 ) ) ;
#5874=CARTESIAN_POINT ( 'NONE',  ( 19.06497207195981147, -10.03556273973439517, 10.03556273973429214 ) ) ;
#5876=( BOUNDED_SURFACE ( )  B_SPLINE_SURFACE ( 3, 3, ( 
 ( #16605, #8220, #22609, #5969, #22476, #18467, #10492, #8491, #20076, #24339, #4386, #6103, #4515, #10225, #1853, #113, #14080, #10355, #2380, #14210, #18064, #18333, #12085, #24199, #20207, #22344, #24467, #16338, #20474, #12217 ),
 ( #7951, #14348, #9957, #24738, #2116, #2248, #18194, #14606, #18605, #1985, #6494, #4123, #22735, #20339, #6233, #26215, #16069, #4255, #12345, #12478, #22211, #20604, #384, #24604, #245, #3986, #6357, #8357, #10090, #16478 ),
 ( #26346, #8626, #11024, #16737, #25139, #19134, #16875, #25007, #7148, #6760, #17003, #14872, #2656, #21141, #4785, #3041, #12616, #8892, #787, #12888, #19010, #23007, #21003, #4649, #12752, #6890, #2916, #15006, #521, #23139 ),
 ( #4910, #2785, #917, #20873, #10898, #15264, #13022, #9029, #24869, #17133, #25266, #7016, #15137, #23267, #5043, #6624, #13150, #23393, #21268, #18873, #11149, #19263, #20744, #1044, #10761, #9147, #17262, #18739, #25397, #2513 ),
 ( #10628, #14741, #22872, #653, #8760, #21519, #19643, #17901, #23895, #11271, #11389, #3168, #21643, #19391, #1296, #17386, #11648, #19909, #3681, #7652, #9278, #13273, #1176, #5168, #21395, #23638, #1427, #7396, #25525, #25778 ),
 ( #9405, #15509, #1693, #7274, #15767, #5671, #15390, #23513, #5287, #26048, #21907, #19511, #3416, #13394, #5416, #7528, #17511, #17769, #15636, #13518, #3293, #15901, #7785, #11789, #25650, #9797, #13777, #11518, #25911, #9527 ),
 ( #17635, #19771, #23761, #5542, #13649, #21774, #3547, #1560, #9665, #14181, #16449, #14452, #24168, #10198, #7925, #24574, #5943, #14051, #11924, #20445, #18440, #12450, #18171, #6330, #22579, #3822, #1826, #13914, #88, #16177 ) ),
 .UNSPECIFIED., .T., .F., .F. ) 
 B_SPLINE_SURFACE_WITH_KNOTS ( ( 4, 3, 4 ),
 ( 4, 2, 2, 2, 2, 2, 2, 2, 2, 2, 2, 2, 2, 2, 4 ),
 ( 0.000000000000000000, 0.5000000000000000000, 1.000000000000000000 ),
 ( 0.000000000000000000, 0.1357259735107005372, 0.1651108541090157700, 0.1944957347073310028, 0.3598804999793158710, 0.3867117631979620773, 0.4135430264166082281, 0.5789277916885930964, 0.6062785021374117456, 0.6336292125862302838, 0.8508620842112317728, 0.8814014469398914198, 0.9119408096685510667, 0.9559704048342755334, 1.000000000000000000 ),
 .UNSPECIFIED. ) 
 GEOMETRIC_REPRESENTATION_ITEM ( )  RATIONAL_B_SPLINE_SURFACE ( (
 ( 1.000000000000000000, 1.000000000000000000, 1.000000000000000000, 1.000000000000000000, 1.000000000000000000, 1.000000000000000000, 1.000000000000000000, 1.000000000000000000, 1.000000000000000000, 1.000000000000000000, 1.000000000000000000, 1.000000000000000000, 1.000000000000000000, 1.000000000000000000, 1.000000000000000000, 1.000000000000000000, 1.000000000000000000, 1.000000000000000000, 1.000000000000000000, 1.000000000000000000, 1.000000000000000000, 1.000000000000000000, 1.000000000000000000, 1.000000000000000000, 1.000000000000000000, 1.000000000000000000, 1.000000000000000000, 1.000000000000000000, 1.000000000000000000, 1.000000000000000000),
 ( 0.3333333333333333703, 0.3333333333333333703, 0.3333333333333333703, 0.3333333333333333703, 0.3333333333333333703, 0.3333333333333333703, 0.3333333333333333703, 0.3333333333333333703, 0.3333333333333333703, 0.3333333333333333703, 0.3333333333333333703, 0.3333333333333333703, 0.3333333333333333703, 0.3333333333333333703, 0.3333333333333333703, 0.3333333333333333703, 0.3333333333333333703, 0.3333333333333333703, 0.3333333333333333703, 0.3333333333333333703, 0.3333333333333333703, 0.3333333333333333703, 0.3333333333333333703, 0.3333333333333333703, 0.3333333333333333703, 0.3333333333333333703, 0.3333333333333333703, 0.3333333333333333703, 0.3333333333333333703, 0.3333333333333333703),
 ( 0.3333333333333333703, 0.3333333333333333703, 0.3333333333333333703, 0.3333333333333333703, 0.3333333333333333703, 0.3333333333333333703, 0.3333333333333333703, 0.3333333333333333703, 0.3333333333333333703, 0.3333333333333333703, 0.3333333333333333703, 0.3333333333333333703, 0.3333333333333333703, 0.3333333333333333703, 0.3333333333333333703, 0.3333333333333333703, 0.3333333333333333703, 0.3333333333333333703, 0.3333333333333333703, 0.3333333333333333703, 0.3333333333333333703, 0.3333333333333333703, 0.3333333333333333703, 0.3333333333333333703, 0.3333333333333333703, 0.3333333333333333703, 0.3333333333333333703, 0.3333333333333333703, 0.3333333333333333703, 0.3333333333333333703),
 ( 1.000000000000000000, 1.000000000000000000, 1.000000000000000000, 1.000000000000000000, 1.000000000000000000, 1.000000000000000000, 1.000000000000000000, 1.000000000000000000, 1.000000000000000000, 1.000000000000000000, 1.000000000000000000, 1.000000000000000000, 1.000000000000000000, 1.000000000000000000, 1.000000000000000000, 1.000000000000000000, 1.000000000000000000, 1.000000000000000000, 1.000000000000000000, 1.000000000000000000, 1.000000000000000000, 1.000000000000000000, 1.000000000000000000, 1.000000000000000000, 1.000000000000000000, 1.000000000000000000, 1.000000000000000000, 1.000000000000000000, 1.000000000000000000, 1.000000000000000000),
 ( 0.3333333333333333703, 0.3333333333333333703, 0.3333333333333333703, 0.3333333333333333703, 0.3333333333333333703, 0.3333333333333333703, 0.3333333333333333703, 0.3333333333333333703, 0.3333333333333333703, 0.3333333333333333703, 0.3333333333333333703, 0.3333333333333333703, 0.3333333333333333703, 0.3333333333333333703, 0.3333333333333333703, 0.3333333333333333703, 0.3333333333333333703, 0.3333333333333333703, 0.3333333333333333703, 0.3333333333333333703, 0.3333333333333333703, 0.3333333333333333703, 0.3333333333333333703, 0.3333333333333333703, 0.3333333333333333703, 0.3333333333333333703, 0.3333333333333333703, 0.3333333333333333703, 0.3333333333333333703, 0.3333333333333333703),
 ( 0.3333333333333333703, 0.3333333333333333703, 0.3333333333333333703, 0.3333333333333333703, 0.3333333333333333703, 0.3333333333333333703, 0.3333333333333333703, 0.3333333333333333703, 0.3333333333333333703, 0.3333333333333333703, 0.3333333333333333703, 0.3333333333333333703, 0.3333333333333333703, 0.3333333333333333703, 0.3333333333333333703, 0.3333333333333333703, 0.3333333333333333703, 0.3333333333333333703, 0.3333333333333333703, 0.3333333333333333703, 0.3333333333333333703, 0.3333333333333333703, 0.3333333333333333703, 0.3333333333333333703, 0.3333333333333333703, 0.3333333333333333703, 0.3333333333333333703, 0.3333333333333333703, 0.3333333333333333703, 0.3333333333333333703),
 ( 1.000000000000000000, 1.000000000000000000, 1.000000000000000000, 1.000000000000000000, 1.000000000000000000, 1.000000000000000000, 1.000000000000000000, 1.000000000000000000, 1.000000000000000000, 1.000000000000000000, 1.000000000000000000, 1.000000000000000000, 1.000000000000000000, 1.000000000000000000, 1.000000000000000000, 1.000000000000000000, 1.000000000000000000, 1.000000000000000000, 1.000000000000000000, 1.000000000000000000, 1.000000000000000000, 1.000000000000000000, 1.000000000000000000, 1.000000000000000000, 1.000000000000000000, 1.000000000000000000, 1.000000000000000000, 1.000000000000000000, 1.000000000000000000, 1.000000000000000000) ) ) 
 REPRESENTATION_ITEM ( '' )  SURFACE ( )  );
#5877=DIRECTION ( 'NONE',  ( 1.000000000000000000, 1.836970198721030181E-16, -0.000000000000000000 ) ) ;
#5878=CARTESIAN_POINT ( 'NONE',  ( -198.0356074513804572, 10.87444709761036066, -67.44298959253325165 ) ) ;
#5879=CARTESIAN_POINT ( 'NONE',  ( -87.11136440740810372, 2.379156564867217494, 21.34823163554904824 ) ) ;
#5880=ORIENTED_EDGE ( 'NONE', *, *, #6304, .T. ) ;
#5882=CARTESIAN_POINT ( 'NONE',  ( 23.37394308801977871, -23.33966569535098046, 42.85717664514577763 ) ) ;
#5883=CARTESIAN_POINT ( 'NONE',  ( -4.580761711670050751, 17.81010960708292501, 42.99740816077149930 ) ) ;
#5886=CARTESIAN_POINT ( 'NONE',  ( 0.2972598230769930572, 14.33493731733933352, 0.000000000000000000 ) ) ;
#5891=CARTESIAN_POINT ( 'NONE',  ( -1.821043593238388603, 43.61003463695197269, -23.89737153267502023 ) ) ;
#5892=CARTESIAN_POINT ( 'NONE',  ( -280.0000000000000568, 39.99999999999976552, 20.00000000000043343 ) ) ;
#5893=CARTESIAN_POINT ( 'NONE',  ( 98.29820294267362613, 4.524526698164271110, -19.49240851342956660 ) ) ;
#5897=CARTESIAN_POINT ( 'NONE',  ( -166.7090608782836227, 15.35183551246269928, 37.06260950135659726 ) ) ;
#5898=CARTESIAN_POINT ( 'NONE',  ( 5.823571940223811083, -14.15488761396733608, -49.16771748718979751 ) ) ;
#5899=CARTESIAN_POINT ( 'NONE',  ( -259.2033419157646676, -21.55415060305824326, -21.55415060305857367 ) ) ;
#5902=CARTESIAN_POINT ( 'NONE',  ( 19.06497207195982924, -66.60410523465823474, 10.03556273973400081 ) ) ;
#5903=CARTESIAN_POINT ( 'NONE',  ( -91.56559293963834989, -40.00000000000027711, 22.67402823373149801 ) ) ;
#5904=CARTESIAN_POINT ( 'NONE',  ( 136.1360204305621266, 35.03383547441298873, 0.000000000000000000 ) ) ;
#5905=CARTESIAN_POINT ( 'NONE',  ( -280.0000000000000568, -20.00000000000007105, 40.00000000000002132 ) ) ;
#5906=CARTESIAN_POINT ( 'NONE',  ( 199.9999999999999432, 14.14213562373113398, -14.14213562373094923 ) ) ;
#5907=CARTESIAN_POINT ( 'NONE',  ( -135.8532207217289454, -30.84685318188649106, 40.00000000000002132 ) ) ;
#5908=CARTESIAN_POINT ( 'NONE',  ( -110.0368417077421128, 7.992411109433636973, 18.51665893310612532 ) ) ;
#5909=CARTESIAN_POINT ( 'NONE',  ( 151.7948205124836534, 39.99999999999970157, 33.23291073765595627 ) ) ;
#5911=CARTESIAN_POINT ( 'NONE',  ( 57.59792236341147031, -1.722363176415032004, -1.722363176415048880 ) ) ;
#5913=CARTESIAN_POINT ( 'NONE',  ( -198.0356074513804572, 15.37879056873067007, 0.000000000000000000 ) ) ;
#5914=AXIS2_PLACEMENT_3D ( 'NONE', #24827, #8445, #16564 ) ;
#5915=ORIENTED_EDGE ( 'NONE', *, *, #21658, .F. ) ;
#5916=CARTESIAN_POINT ( 'NONE',  ( -105.3755690713226727, -21.75974354311652093, 0.000000000000000000 ) ) ;
#5919=CARTESIAN_POINT ( 'NONE',  ( -91.56559293963834989, 40.53558337403677569, -16.03295912088699993 ) ) ;
#5920=CARTESIAN_POINT ( 'NONE',  ( -213.1075012329537230, -2.291445344039133686E-13, 53.71589010951915100 ) ) ;
#5921=CARTESIAN_POINT ( 'NONE',  ( -91.56559293963834989, -16.03295912088728414, 16.03295912088688269 ) ) ;
#5922=CARTESIAN_POINT ( 'NONE',  ( -280.0000000000000000, -20.00000000000006750, 0.000000000000000000 ) ) ;
#5923=CARTESIAN_POINT ( 'NONE',  ( -208.1127848780264742, 15.00245453012665742, -40.00000000000002132 ) ) ;
#5928=CARTESIAN_POINT ( 'NONE',  ( 57.59792236341147031, 26.56190807104720975, -26.56190807104655249 ) ) ;
#5929=CARTESIAN_POINT ( 'NONE',  ( 91.82158438592159655, -16.11829626346125011, -16.11829626346154853 ) ) ;
#5930=CARTESIAN_POINT ( 'NONE',  ( 0.2972598230769976091, -10.13633138497479180, 10.13633138497468522 ) ) ;
#5932=CARTESIAN_POINT ( 'NONE',  ( 91.82158438592159655, -44.40256751092341858, 12.16597498400012434 ) ) ;
#5934=CARTESIAN_POINT ( 'NONE',  ( -213.1075012329537230, -18.58567234101102272, -37.98287015391260013 ) ) ;
#5935=CARTESIAN_POINT ( 'NONE',  ( -238.4067589809705794, -28.96627169325313389, -27.60227080167074831 ) ) ;
#5938=CARTESIAN_POINT ( 'NONE',  ( 170.2234770963711128, -39.99999999999991473, -24.55285855007201334 ) ) ;
#5940=CARTESIAN_POINT ( 'NONE',  ( -3.406542234095620625, 43.31371932780143652, -17.94112998239643630 ) ) ;
#5941=CARTESIAN_POINT ( 'NONE',  ( -56.48582580120559271, 30.84685318188643066, 2.449293598294708485E-15 ) ) ;
#5943=CARTESIAN_POINT ( 'NONE',  ( 4.995406935893289102, 10.78321810388998081, 10.78321810389001811 ) ) ;
#5944=CARTESIAN_POINT ( 'NONE',  ( 98.29820294267314296, 18.47759065023127079, 7.653668647304074923 ) ) ;
#5946=CARTESIAN_POINT ( 'NONE',  ( -56.48582580120559271, -9.153146818113595984, 0.000000000000000000 ) ) ;
#5947=ORIENTED_EDGE ( 'NONE', *, *, #11202, .F. ) ;
#5948=CARTESIAN_POINT ( 'NONE',  ( -190.0144222802868228, -47.57278142029906576, 13.91469272131868884 ) ) ;
#5951=CARTESIAN_POINT ( 'NONE',  ( 16.38602454706083122, -24.50452114744929233, 44.43226271088774837 ) ) ;
#5953=CARTESIAN_POINT ( 'NONE',  ( 17.91733029159796686, 14.04577174276132290, -48.44632265253467551 ) ) ;
#5956=CARTESIAN_POINT ( 'NONE',  ( 184.8905102610680444, 1.070102760522089011E-13, -20.92133201514444352 ) ) ;
#5957=CARTESIAN_POINT ( 'NONE',  ( -213.1075012329537230, 37.98287015391280619, -37.98287015391192512 ) ) ;
#5958=CARTESIAN_POINT ( 'NONE',  ( -87.13361725327075646, -1.371494812282539888, 21.49321519333427588 ) ) ;
#5959=CARTESIAN_POINT ( 'NONE',  ( -191.2490444017329878, 18.16428715637510294, -43.85246840377958932 ) ) ;
#5960=CARTESIAN_POINT ( 'NONE',  ( -162.0762913951020892, 1.198031840385732849, -1.198031840385733515 ) ) ;
#5961=CARTESIAN_POINT ( 'NONE',  ( 146.6084372240433993, 34.62501878078308692, 0.000000000000000000 ) ) ;
#5962=CARTESIAN_POINT ( 'NONE',  ( -56.48582580120559982, 9.153146818113574668, -40.00000000000002132 ) ) ;
#5963=CARTESIAN_POINT ( 'NONE',  ( -192.9588430854690273, 14.46834944099966336, 40.00000000000002132 ) ) ;
#5964=CARTESIAN_POINT ( 'NONE',  ( -198.0356074513804572, -39.99999999999948130, -55.37879056874863437 ) ) ;
#5965=CARTESIAN_POINT ( 'NONE',  ( -192.9588430854690273, 66.79921049721887982, 10.23066800229522677 ) ) ;
#5967=CARTESIAN_POINT ( 'NONE',  ( -238.4067589809705794, 27.60227080167080160, -28.96627169325299533 ) ) ;
#5968=ORIENTED_EDGE ( 'NONE', *, *, #56, .T. ) ;
#5969=CARTESIAN_POINT ( 'NONE',  ( -213.1075012329537230, 9.698598906450410340, 9.698598906450483170 ) ) ;
#5972=CARTESIAN_POINT ( 'NONE',  ( -97.73806390046074455, -8.581719943970163911, 20.71810467719253523 ) ) ;
#5975=ORIENTED_EDGE ( 'NONE', *, *, #3142, .T. ) ;
#5976=CARTESIAN_POINT ( 'NONE',  ( 151.7948205124836534, -33.06932595376343897, -23.49921654116042902 ) ) ;
#5977=CARTESIAN_POINT ( 'NONE',  ( 23.84827734669607580, -46.63681169410487115, -13.76599369847224530 ) ) ;
#5979=CARTESIAN_POINT ( 'NONE',  ( 163.1118516004056573, -27.26290988616869626, -40.00000000000002132 ) ) ;
#5980=CARTESIAN_POINT ( 'NONE',  ( -93.01854144619034059, -20.65013722612175329, 8.553566904080200928 ) ) ;
#5983=( BOUNDED_SURFACE ( )  B_SPLINE_SURFACE ( 3, 2, ( 
 ( #6705, #16822, #470 ),
 ( #18821, #10712, #16952 ),
 ( #25088, #4864, #24819 ),
 ( #14427, #20956, #6571 ),
 ( #21089, #6838, #8438 ),
 ( #16687, #14691, #22822 ),
 ( #4599, #18417, #12697 ),
 ( #20825, #10571, #601 ),
 ( #12967, #24959, #22689 ),
 ( #23093, #20691, #14819 ),
 ( #10437, #10841, #14958 ),
 ( #16557, #2872, #16427 ),
 ( #22952, #192, #4730 ),
 ( #8302, #18959, #24554 ),
 ( #6309, #12839, #22558 ),
 ( #739, #12429, #20557 ) ),
 .UNSPECIFIED., .F., .F., .F. ) 
 B_SPLINE_SURFACE_WITH_KNOTS ( ( 4, 2, 2, 2, 2, 2, 2, 4 ),
 ( 3, 3 ),
 ( 0.04143342415519529059, 0.04844520227997907436, 0.05195109134237096277, 0.05545698040476285118, 0.06246875852954662800, 0.06422170306074256874, 0.06597464759193852335, 0.06948053665433040482 ),
 ( 0.000000000000000000, 1.000000000000000000 ),
 .UNSPECIFIED. ) 
 GEOMETRIC_REPRESENTATION_ITEM ( )  RATIONAL_B_SPLINE_SURFACE ( (
 ( 1.000000000000000000, 0.9541700777564864344, 1.000000000000000000),
 ( 1.000000000000000000, 0.9520170179160779567, 1.000000000000000000),
 ( 1.000000000000000000, 0.9503264940267351912, 1.000000000000000000),
 ( 1.000000000000000000, 0.9485966650357424701, 1.000000000000000000),
 ( 1.000000000000000000, 0.9481601953987753850, 1.000000000000000000),
 ( 1.000000000000000000, 0.9475786562871791885, 1.000000000000000000),
 ( 1.000000000000000000, 0.9474333041661833210, 1.000000000000000000),
 ( 1.000000000000000000, 0.9474385324120137009, 1.000000000000000000),
 ( 1.000000000000000000, 0.9480205960577967605, 1.000000000000000000),
 ( 1.000000000000000000, 0.9494433550397415322, 1.000000000000000000),
 ( 1.000000000000000000, 0.9497628485353458716, 1.000000000000000000),
 ( 1.000000000000000000, 0.9504717112743156227, 1.000000000000000000),
 ( 1.000000000000000000, 0.9508623530681812319, 1.000000000000000000),
 ( 1.000000000000000000, 0.9521262215765325942, 1.000000000000000000),
 ( 1.000000000000000000, 0.9530922057186239638, 1.000000000000000000),
 ( 1.000000000000000000, 0.9541700777564561253, 1.000000000000000000) ) ) 
 REPRESENTATION_ITEM ( '' )  SURFACE ( )  );
#5985=CARTESIAN_POINT ( 'NONE',  ( 0.2972598230769886718, 38.42060263243669027, -18.14793986248710667 ) ) ;
#5986=CARTESIAN_POINT ( 'NONE',  ( -188.3611024622163370, -43.02327292322560481, -23.46270902204799569 ) ) ;
#5987=CARTESIAN_POINT ( 'NONE',  ( -162.0762913951021176, -40.00000000000005684, 1.694272876828184504 ) ) ;
#5988=CARTESIAN_POINT ( 'NONE',  ( -198.0356074513804572, 55.37879056871320671, 40.00000000000002132 ) ) ;
#5992=AXIS2_PLACEMENT_3D ( 'NONE', #1911, #14139, #4045 ) ;
#5993=CARTESIAN_POINT ( 'NONE',  ( 146.6084372240433993, 1.478241399363601114E-13, -34.62501878078305850 ) ) ;
#5994=CARTESIAN_POINT ( 'NONE',  ( 200.0000000000000000, -40.00000000000005684, 19.99999999999978328 ) ) ;
#5996=CARTESIAN_POINT ( 'NONE',  ( -91.56559293963834989, -2.543181659092656077E-13, 22.67402823373191723 ) ) ;
#5997=CARTESIAN_POINT ( 'NONE',  ( 14.38125909742180220, 39.99999999999997158, 15.17850393972647716 ) ) ;
#5999=CARTESIAN_POINT ( 'NONE',  ( 4.995406935893310418, -67.35176059880237176, 10.78321810387813429 ) ) ;
#6000=CARTESIAN_POINT ( 'NONE',  ( -105.3755690713226869, 21.75974354311648540, -0.000000000000000000 ) ) ;
#6001=CARTESIAN_POINT ( 'NONE',  ( 19.06497207195981858, -38.31983398719616218, -18.24870850772777331 ) ) ;
#6004=CARTESIAN_POINT ( 'NONE',  ( -91.56559293963836410, 39.99999999999976552, 22.67402823373234000 ) ) ;
#6005=CARTESIAN_POINT ( 'NONE',  ( -91.56559293963834989, -7.976292724337646577E-14, 17.32597176626811120 ) ) ;
#6006=CARTESIAN_POINT ( 'NONE',  ( 0.2972598230769907257, 66.70487387989857098, 10.13633138497486641 ) ) ;
#6007=CARTESIAN_POINT ( 'NONE',  ( 91.82158438592158234, 12.16597498397756993, 12.16597498397776356 ) ) ;
#6008=CARTESIAN_POINT ( 'NONE',  ( -188.3120606736019909, -13.82878088495181323, -46.99497558484008408 ) ) ;
#6009=CARTESIAN_POINT ( 'NONE',  ( 4.995406935893293543, -10.78321810389005364, 10.78321810388994173 ) ) ;
#6011=CARTESIAN_POINT ( 'NONE',  ( -259.2033419157646676, -6.730120644403663199, 6.730120644403451813 ) ) ;
#6012=CARTESIAN_POINT ( 'NONE',  ( 98.29820294267868519, -19.50609486047250840, 5.170639833975480215 ) ) ;
#6013=CARTESIAN_POINT ( 'NONE',  ( 98.29820294267493352, -20.00000000000511235, 5.223721743777709619E-12 ) ) ;
#6014=CARTESIAN_POINT ( 'NONE',  ( -192.9588430854690273, -18.05360324515400094, -38.51493924976961836 ) ) ;
#6016=ORIENTED_EDGE ( 'NONE', *, *, #20204, .F. ) ;
#6020=CARTESIAN_POINT ( 'NONE',  ( -4.439300432585279843, 23.37136716947921755, 42.88738538954466151 ) ) ;
#6022=ORIENTED_EDGE ( 'NONE', *, *, #23619, .T. ) ;
#6024=CARTESIAN_POINT ( 'NONE',  ( 136.1360204305621266, -35.03383547441293899, 0.000000000000000000 ) ) ;
#6026=CARTESIAN_POINT ( 'NONE',  ( -105.3844690779178137, -6.703180366840864046, -20.33701293466475946 ) ) ;
#6027=DIRECTION ( 'NONE',  ( 0.01051738792037367962, -0.3995761383046945725, 0.9166396752534989867 ) ) ;
#6028=CARTESIAN_POINT ( 'NONE',  ( 18.89824403360310967, 43.99464769172853096, -24.18164459663352517 ) ) ;
#6029=CARTESIAN_POINT ( 'NONE',  ( -162.0762913951021176, 40.00000000000001421, -1.694272876827905394 ) ) ;
#6032=AXIS2_PLACEMENT_3D ( 'NONE', #11312, #25567, #3586 ) ;
#6035=CARTESIAN_POINT ( 'NONE',  ( -128.3942957220574215, 24.92786587692849665, 10.32546012722446704 ) ) ;
#6036=CARTESIAN_POINT ( 'NONE',  ( -2.557884977116410941, -13.90734923103991072, -47.52441970260808546 ) ) ;
#6037=CARTESIAN_POINT ( 'NONE',  ( 4.995406935893305977, -39.06748935135157552, -39.06748935135225764 ) ) ;
#6038=( BOUNDED_SURFACE ( )  B_SPLINE_SURFACE ( 3, 3, ( 
 ( #17531, #15283, #21413, #11293, #25544, #1317, #7295, #15409, #3314, #21539, #26067, #13933, #5564, #19793, #5690, #21793, #3840, #1448, #22204, #3565, #1580, #16062, #22068, #3979, #21930, #1845, #19661, #9819, #5830, #24188 ),
 ( #11669, #25934, #13795, #11807, #18057, #20069, #7415, #23915, #21665, #9683, #9548, #11943, #12076, #5962, #9948, #20198, #15530, #1710, #14072, #23658, #7675, #3704, #17789, #15788, #5438, #11537, #26208, #1977, #13539, #19927 ),
 ( #7944, #3438, #17657, #25798, #10083, #18187, #13671, #17923, #7546, #7805, #15658, #23784, #15921, #24054, #18729, #10483, #4377, #24730, #14337, #22864, #106, #6615, #12210, #6486, #22337, #14598, #4112, #12468, #22728, #4248 ),
 ( #6096, #18597, #16469, #14468, #14732, #10616, #16597, #18458, #20595, #10218, #513, #8213, #2371, #8080, #8618, #16729, #24860, #16198, #8479, #22469, #14203, #20332, #24332, #375, #4641, #4506, #6349, #2241, #12607, #20466 ),
 ( #2109, #12743, #20736, #20863, #18325, #16331, #10348, #2647, #24460, #6224, #236, #2505, #8348, #10754, #12338, #24593, #22601, #26338, #25871, #13356, #5633, #18865, #25737, #23601, #8752, #5380, #25000, #11478, #9364, #7361 ),
 ( #16868, #16996, #9493, #15472, #13485, #19473, #25616, #21606, #15600, #25131, #6881, #21736, #15730, #8885, #17730, #3379, #15356, #6753, #7615, #19606, #7489, #12880, #646, #23480, #14865, #1392, #779, #4776, #9627, #5252 ),
 ( #21478, #20996, #17598, #3253, #10890, #13740, #22999, #11357, #2778, #23725, #19002, #5506, #13607, #1260, #23855, #17474, #3512, #11612, #19734, #1521, #21866, #3642, #5904, #19867, #22141, #14278, #10295, #12284, #16006, #3922 ) ),
 .UNSPECIFIED., .T., .F., .T. ) 
 B_SPLINE_SURFACE_WITH_KNOTS ( ( 4, 3, 4 ),
 ( 4, 2, 2, 2, 2, 2, 2, 2, 2, 2, 2, 2, 2, 2, 4 ),
 ( 0.000000000000000000, 0.5000000000000000000, 1.000000000000000000 ),
 ( 0.000000000000000000, 0.1357259735107005372, 0.1651108541090157700, 0.1944957347073310028, 0.3598804999793158710, 0.3867117631979620773, 0.4135430264166082281, 0.5789277916885930964, 0.6062785021374117456, 0.6336292125862302838, 0.8508620842112317728, 0.8814014469398914198, 0.9119408096685510667, 0.9559704048342755334, 1.000000000000000000 ),
 .UNSPECIFIED. ) 
 GEOMETRIC_REPRESENTATION_ITEM ( )  RATIONAL_B_SPLINE_SURFACE ( (
 ( 1.000000000000000000, 1.000000000000000000, 1.000000000000000000, 1.000000000000000000, 1.000000000000000000, 1.000000000000000000, 1.000000000000000000, 1.000000000000000000, 1.000000000000000000, 1.000000000000000000, 1.000000000000000000, 1.000000000000000000, 1.000000000000000000, 1.000000000000000000, 1.000000000000000000, 1.000000000000000000, 1.000000000000000000, 1.000000000000000000, 1.000000000000000000, 1.000000000000000000, 1.000000000000000000, 1.000000000000000000, 1.000000000000000000, 1.000000000000000000, 1.000000000000000000, 1.000000000000000000, 1.000000000000000000, 1.000000000000000000, 1.000000000000000000, 1.000000000000000000),
 ( 0.3333333333333333703, 0.3333333333333333703, 0.3333333333333333703, 0.3333333333333333703, 0.3333333333333333703, 0.3333333333333333703, 0.3333333333333333703, 0.3333333333333333703, 0.3333333333333333703, 0.3333333333333333703, 0.3333333333333333703, 0.3333333333333333703, 0.3333333333333333703, 0.3333333333333333703, 0.3333333333333333703, 0.3333333333333333703, 0.3333333333333333703, 0.3333333333333333703, 0.3333333333333333703, 0.3333333333333333703, 0.3333333333333333703, 0.3333333333333333703, 0.3333333333333333703, 0.3333333333333333703, 0.3333333333333333703, 0.3333333333333333703, 0.3333333333333333703, 0.3333333333333333703, 0.3333333333333333703, 0.3333333333333333703),
 ( 0.3333333333333333703, 0.3333333333333333703, 0.3333333333333333703, 0.3333333333333333703, 0.3333333333333333703, 0.3333333333333333703, 0.3333333333333333703, 0.3333333333333333703, 0.3333333333333333703, 0.3333333333333333703, 0.3333333333333333703, 0.3333333333333333703, 0.3333333333333333703, 0.3333333333333333703, 0.3333333333333333703, 0.3333333333333333703, 0.3333333333333333703, 0.3333333333333333703, 0.3333333333333333703, 0.3333333333333333703, 0.3333333333333333703, 0.3333333333333333703, 0.3333333333333333703, 0.3333333333333333703, 0.3333333333333333703, 0.3333333333333333703, 0.3333333333333333703, 0.3333333333333333703, 0.3333333333333333703, 0.3333333333333333703),
 ( 1.000000000000000000, 1.000000000000000000, 1.000000000000000000, 1.000000000000000000, 1.000000000000000000, 1.000000000000000000, 1.000000000000000000, 1.000000000000000000, 1.000000000000000000, 1.000000000000000000, 1.000000000000000000, 1.000000000000000000, 1.000000000000000000, 1.000000000000000000, 1.000000000000000000, 1.000000000000000000, 1.000000000000000000, 1.000000000000000000, 1.000000000000000000, 1.000000000000000000, 1.000000000000000000, 1.000000000000000000, 1.000000000000000000, 1.000000000000000000, 1.000000000000000000, 1.000000000000000000, 1.000000000000000000, 1.000000000000000000, 1.000000000000000000, 1.000000000000000000),
 ( 0.3333333333333333703, 0.3333333333333333703, 0.3333333333333333703, 0.3333333333333333703, 0.3333333333333333703, 0.3333333333333333703, 0.3333333333333333703, 0.3333333333333333703, 0.3333333333333333703, 0.3333333333333333703, 0.3333333333333333703, 0.3333333333333333703, 0.3333333333333333703, 0.3333333333333333703, 0.3333333333333333703, 0.3333333333333333703, 0.3333333333333333703, 0.3333333333333333703, 0.3333333333333333703, 0.3333333333333333703, 0.3333333333333333703, 0.3333333333333333703, 0.3333333333333333703, 0.3333333333333333703, 0.3333333333333333703, 0.3333333333333333703, 0.3333333333333333703, 0.3333333333333333703, 0.3333333333333333703, 0.3333333333333333703),
 ( 0.3333333333333333703, 0.3333333333333333703, 0.3333333333333333703, 0.3333333333333333703, 0.3333333333333333703, 0.3333333333333333703, 0.3333333333333333703, 0.3333333333333333703, 0.3333333333333333703, 0.3333333333333333703, 0.3333333333333333703, 0.3333333333333333703, 0.3333333333333333703, 0.3333333333333333703, 0.3333333333333333703, 0.3333333333333333703, 0.3333333333333333703, 0.3333333333333333703, 0.3333333333333333703, 0.3333333333333333703, 0.3333333333333333703, 0.3333333333333333703, 0.3333333333333333703, 0.3333333333333333703, 0.3333333333333333703, 0.3333333333333333703, 0.3333333333333333703, 0.3333333333333333703, 0.3333333333333333703, 0.3333333333333333703),
 ( 1.000000000000000000, 1.000000000000000000, 1.000000000000000000, 1.000000000000000000, 1.000000000000000000, 1.000000000000000000, 1.000000000000000000, 1.000000000000000000, 1.000000000000000000, 1.000000000000000000, 1.000000000000000000, 1.000000000000000000, 1.000000000000000000, 1.000000000000000000, 1.000000000000000000, 1.000000000000000000, 1.000000000000000000, 1.000000000000000000, 1.000000000000000000, 1.000000000000000000, 1.000000000000000000, 1.000000000000000000, 1.000000000000000000, 1.000000000000000000, 1.000000000000000000, 1.000000000000000000, 1.000000000000000000, 1.000000000000000000, 1.000000000000000000, 1.000000000000000000) ) ) 
 REPRESENTATION_ITEM ( '' )  SURFACE ( )  );
#6039=CARTESIAN_POINT ( 'NONE',  ( -200.0000000000000568, 19.51623549979305494, 45.81998439131043455 ) ) ;
#6040=CARTESIAN_POINT ( 'NONE',  ( -280.0000000000000568, -42.42640687119285303, -14.14213562373118371 ) ) ;
#6041=CARTESIAN_POINT ( 'NONE',  ( 199.9999999999999432, -1.727494763561684666E-13, 20.00000000000010303 ) ) ;
#6042=CARTESIAN_POINT ( 'NONE',  ( -192.9588430854690273, 18.05360324515473280, -38.51493924976924177 ) ) ;
#6043=CARTESIAN_POINT ( 'NONE',  ( -86.96347745069643054, -18.24025645688353947, 40.00000000000002132 ) ) ;
#6044=CARTESIAN_POINT ( 'NONE',  ( -208.1127848780265026, 10.60833733269551615, -10.60833733269529766 ) ) ;
#6045=CARTESIAN_POINT ( 'NONE',  ( -135.8532207217289738, -30.84685318188647685, -2.449293598294708485E-15 ) ) ;
#6046=CARTESIAN_POINT ( 'NONE',  ( -114.7366410982253910, 17.62971985773716810, 13.31543432720488518 ) ) ;
#6047=CARTESIAN_POINT ( 'NONE',  ( -213.1075012329537230, 5.259461644596141978E-13, -53.71589010951915100 ) ) ;
#6048=CARTESIAN_POINT ( 'NONE',  ( -30.26275506840324070, 1.198031551616013601, 1.198031551616023371 ) ) ;
#6049=CARTESIAN_POINT ( 'NONE',  ( -280.0000000000000568, -20.00000000000006750, -40.00000000000002132 ) ) ;
#6050=VERTEX_POINT ( 'NONE', #7620 ) ;
#6051=VERTEX_POINT ( 'NONE', #15866 ) ;
#6052=CARTESIAN_POINT ( 'NONE',  ( 130.8568914410475088, -34.05028731879786363, 40.00000000000002132 ) ) ;
#6054=EDGE_CURVE ( 'NONE', #1209, #15843, #12725, .T. ) ;
#6055=CARTESIAN_POINT ( 'NONE',  ( -56.48582580120558561, -1.205267837095813407E-13, 30.84685318188644132 ) ) ;
#6056=CARTESIAN_POINT ( 'NONE',  ( -208.1127848780264742, 38.89260858015707356, 17.67593391476696141 ) ) ;
#6057=CARTESIAN_POINT ( 'NONE',  ( 130.8568914410475372, -34.05028731879786363, 0.000000000000000000 ) ) ;
#6061=ADVANCED_FACE ( 'NONE', ( #3259 ), #8708, .T. ) ;
#6062=EDGE_CURVE ( 'NONE', #22617, #1078, #16835, .T. ) ;
#6064=CARTESIAN_POINT ( 'NONE',  ( 163.1118516004056573, 9.006482792069759213, -9.006482792069505194 ) ) ;
#6065=CARTESIAN_POINT ( 'NONE',  ( -192.9588430854690273, -66.79921049721887982, -10.23066800229569040 ) ) ;
#6067=CARTESIAN_POINT ( 'NONE',  ( -91.56559293963834989, -2.543181659092656077E-13, 22.67402823373191723 ) ) ;
#6068=CARTESIAN_POINT ( 'NONE',  ( -238.4067589809705794, -28.96627169325352469, 27.60227080167035041 ) ) ;
#6069=CARTESIAN_POINT ( 'NONE',  ( -135.8532207217289738, -6.472252184284280396, 6.472252184284099208 ) ) ;
#6070=CARTESIAN_POINT ( 'NONE',  ( -100.7734535825088500, -44.31723036834885932, -12.25131212657538171 ) ) ;
#6071=CARTESIAN_POINT ( 'NONE',  ( 163.1118516004056573, 19.27778845538780317, -19.27778845538757224 ) ) ;
#6074=CARTESIAN_POINT ( 'NONE',  ( 151.7948205124836250, 1.807796684091926154E-15, 6.767089262349031742 ) ) ;
#6076=CARTESIAN_POINT ( 'NONE',  ( 23.17367289775338435, 46.88342923877050339, -13.81211338457316806 ) ) ;
#6077=CARTESIAN_POINT ( 'NONE',  ( 57.59792236341147031, 37.56421063658187620, -40.00000000000002132 ) ) ;
#6079=CARTESIAN_POINT ( 'NONE',  ( -162.0762913951020892, 1.694272876828294194, 0.000000000000000000 ) ) ;
#6080=CARTESIAN_POINT ( 'NONE',  ( -40.07203023070061931, -32.10811084140490834, 16.33025453626358825 ) ) ;
#6081=CARTESIAN_POINT ( 'NONE',  ( -238.4067589809705794, 0.9644942799825386714, 0.000000000000000000 ) ) ;
#6083=CARTESIAN_POINT ( 'NONE',  ( -189.1815713358170399, -43.37724571962257158, 17.96744347545579146 ) ) ;
#6085=CARTESIAN_POINT ( 'NONE',  ( 6.202588567996007995, -24.77700748806806175, 44.80189419270405438 ) ) ;
#6086=CARTESIAN_POINT ( 'NONE',  ( 23.25494099740788556, 17.82744980610155849, -43.03927110441497916 ) ) ;
#6090=CARTESIAN_POINT ( 'NONE',  ( -114.4388184736403389, -8.352332320002028965, 20.16431396440694002 ) ) ;
#6091=CARTESIAN_POINT ( 'NONE',  ( 192.4448373802100889, 14.14213562370330379, -14.14213562370292365 ) ) ;
#6092=CARTESIAN_POINT ( 'NONE',  ( 163.1118516004056573, 27.26290988616876021, 40.00000000000002132 ) ) ;
#6093=CARTESIAN_POINT ( 'NONE',  ( -188.2507053403064674, 13.82466505297411885, -46.97353740712659231 ) ) ;
#6094=CARTESIAN_POINT ( 'NONE',  ( -100.7734535825088358, -16.03295912088728770, 16.03295912088687913 ) ) ;
#6095=CARTESIAN_POINT ( 'NONE',  ( -238.4067589809705794, 0.6820004457912851592, -0.6820004457913123597 ) ) ;
#6096=CARTESIAN_POINT ( 'NONE',  ( -280.0000000000000000, -20.00000000000006750, -2.449293598294708485E-15 ) ) ;
#6097=CARTESIAN_POINT ( 'NONE',  ( -100.7734535825088358, 17.32597176626809343, 2.449293598294708485E-15 ) ) ;
#6098=CARTESIAN_POINT ( 'NONE',  ( -56.48582580120557850, -39.99999999999970868, -30.84685318188687120 ) ) ;
#6099=CARTESIAN_POINT ( 'NONE',  ( -105.3755690713226585, 41.18208027870598187, -15.38646221621779731 ) ) ;
#6101=CARTESIAN_POINT ( 'NONE',  ( -105.3755690713226585, 43.67073346367988051, -12.89780903124366418 ) ) ;
#6103=CARTESIAN_POINT ( 'NONE',  ( -91.56559293963834989, -16.03295912088706388, -16.03295912088710651 ) ) ;
#6104=CARTESIAN_POINT ( 'NONE',  ( -188.5332406156510388, -13.84065976281315180, -47.07509730618265564 ) ) ;
#6107=CARTESIAN_POINT ( 'NONE',  ( 192.4448373802100889, 14.14213562375893574, -14.14213562375874922 ) ) ;
#6108=CARTESIAN_POINT ( 'NONE',  ( 60.28378959931642100, -31.18416451518941912, -15.72633063265140407 ) ) ;
#6110=CARTESIAN_POINT ( 'NONE',  ( -91.56559293963834989, 17.32597176626809699, -40.00000000000002132 ) ) ;
#6115=CARTESIAN_POINT ( 'NONE',  ( 192.4448373802100889, -14.14213562375876698, -14.14213562375885047 ) ) ;
#6116=CARTESIAN_POINT ( 'NONE',  ( -188.3392995398489802, -43.01688924973668549, -23.45797413244871166 ) ) ;
#6117=CARTESIAN_POINT ( 'NONE',  ( -198.0356074513804572, -40.00000000000025580, 55.37879056871310013 ) ) ;
#6118=CARTESIAN_POINT ( 'NONE',  ( 136.1360204305621551, -35.03383547441293899, 40.00000000000002132 ) ) ;
#6121=CARTESIAN_POINT ( 'NONE',  ( -91.56559293963834989, -39.99999999999995737, -22.67402823373205933 ) ) ;
#6122=CARTESIAN_POINT ( 'NONE',  ( 163.1118516004056573, -1.695744499706194789E-14, 12.73709011382475254 ) ) ;
#6123=CARTESIAN_POINT ( 'NONE',  ( -238.4067589809705794, 39.99999999999997158, 0.9644942799827220803 ) ) ;
#6124=CARTESIAN_POINT ( 'NONE',  ( -162.0762913951021176, -1.694272876828353702, -40.00000000000002132 ) ) ;
#6125=CARTESIAN_POINT ( 'NONE',  ( 170.2234770963711128, -10.92277846919202666, 10.92277846919193962 ) ) ;
#6126=CARTESIAN_POINT ( 'NONE',  ( 130.8568914410475372, 34.05028731879791337, 0.000000000000000000 ) ) ;
#6127=CARTESIAN_POINT ( 'NONE',  ( 184.8905102610680444, -13.49065550809780412, -43.07788698682583828 ) ) ;
#6128=CARTESIAN_POINT ( 'NONE',  ( -93.02511667906880177, -8.946512270085145602, 20.50052124204815129 ) ) ;
#6130=CARTESIAN_POINT ( 'NONE',  ( -56.48582580120559271, -1.062504017861011783E-13, 9.153146818113587102 ) ) ;
#6131=CARTESIAN_POINT ( 'NONE',  ( 192.4448373802101173, -40.00000000000005684, 19.99999999996046185 ) ) ;
#6132=CARTESIAN_POINT ( 'NONE',  ( 57.59792236341147031, 54.84617931850881689, -1.722363176414946073 ) ) ;
#6133=CARTESIAN_POINT ( 'NONE',  ( -91.56559293963836410, 16.03295912088692177, 16.03295912088721664 ) ) ;
#6134=CARTESIAN_POINT ( 'NONE',  ( -188.2507053402904660, -13.82466505297120740, -46.97353740712224379 ) ) ;
#6135=CARTESIAN_POINT ( 'NONE',  ( -135.8532207217289738, -21.81201906317758343, -34.75652343174620995 ) ) ;
#6137=CARTESIAN_POINT ( 'NONE',  ( -198.0356074513804572, 10.87444709759730088, -10.87444709759707173 ) ) ;
#6139=CARTESIAN_POINT ( 'NONE',  ( -162.0762913951021176, -1.694272876828353702, -40.00000000000002132 ) ) ;
#6141=CARTESIAN_POINT ( 'NONE',  ( 170.2234770963711128, -17.36149277826940462, -39.20704971665412586 ) ) ;
#6143=ORIENTED_EDGE ( 'NONE', *, *, #1201, .T. ) ;
#6145=CARTESIAN_POINT ( 'NONE',  ( 7.307793593482389660, -24.85783611765724999, 44.91153572052495235 ) ) ;
#6147=CARTESIAN_POINT ( 'NONE',  ( -5.866564133101844547, 13.69896896866289815, 46.35727274689033806 ) ) ;
#6150=CARTESIAN_POINT ( 'NONE',  ( 146.6084372240433993, -34.62501878078303008, 0.000000000000000000 ) ) ;
#6154=B_SPLINE_CURVE_WITH_KNOTS ( 'NONE', 3,
 ( #1216, #9704, #21686, #7188, #23554, #13692, #11691, #9571, #5327, #9194, #17678, #15304 ),
 .UNSPECIFIED., .F., .F.,
 ( 4, 2, 2, 2, 2, 4 ),
 ( 2.860979249076398407E-17, 0.005971690550335911375, 0.008957535825503855353, 0.01045045846308778267, 0.01119691978187970643, 0.01194338110067163193 ),
 .UNSPECIFIED. ) ;
#6155=CARTESIAN_POINT ( 'NONE',  ( -105.4741150117390731, -8.366608964594128395, -19.60045294982696973 ) ) ;
#6157=CARTESIAN_POINT ( 'NONE',  ( 146.6084372240433709, 39.99999999999968026, 34.62501878078347772 ) ) ;
#6158=CARTESIAN_POINT ( 'NONE',  ( 98.29820294267348402, 6.423630604792454513, -18.95183585406372373 ) ) ;
#6160=CARTESIAN_POINT ( 'NONE',  ( -188.2995950289364089, 43.00522595870987885, -23.44932284465868477 ) ) ;
#6162=CARTESIAN_POINT ( 'NONE',  ( -185.1929807734386486, 41.48858353734955529, 17.18513398481663756 ) ) ;
#6163=CARTESIAN_POINT ( 'NONE',  ( 16.10036699868241783, -14.09853761975161390, -48.79524671499645905 ) ) ;
#6164=CARTESIAN_POINT ( 'NONE',  ( -280.0000000000000000, -14.14213562373088706, -14.14213562373108424 ) ) ;
#6166=CARTESIAN_POINT ( 'NONE',  ( -100.7734535825088500, -40.53558337403669753, -16.03295912088728770 ) ) ;
#6168=CARTESIAN_POINT ( 'NONE',  ( 130.8568914410475372, 24.07718906447210472, 24.07718906447249907 ) ) ;
#6169=CARTESIAN_POINT ( 'NONE',  ( 170.2234770963711128, -15.44714144992812876, -2.449293598294708485E-15 ) ) ;
#6171=CARTESIAN_POINT ( 'NONE',  ( 184.8905102610680444, -19.07866798485553872, -40.00000000000002132 ) ) ;
#6173=CARTESIAN_POINT ( 'NONE',  ( 146.6084372240433709, 40.00000000000010658, -5.374981219216549810 ) ) ;
#6174=CARTESIAN_POINT ( 'NONE',  ( 200.0000000000000000, 42.42640687119288856, -14.14213562373094746 ) ) ;
#6175=CARTESIAN_POINT ( 'NONE',  ( 170.2234770963711128, -24.55285855007183926, 0.000000000000000000 ) ) ;
#6176=VERTEX_POINT ( 'NONE', #4825 ) ;
#6177=ORIENTED_EDGE ( 'NONE', *, *, #17258, .T. ) ;
#6178=CARTESIAN_POINT ( 'NONE',  ( -56.48582580120559271, -9.153146818113595984, 0.000000000000000000 ) ) ;
#6180=CARTESIAN_POINT ( 'NONE',  ( 200.0000000000000000, 39.99999999999999289, 20.00000000000007105 ) ) ;
#6181=CARTESIAN_POINT ( 'NONE',  ( -208.1127848780264742, 67.17687982763172272, -10.60833733270698254 ) ) ;
#6182=CARTESIAN_POINT ( 'NONE',  ( 151.7948205124836250, -33.23291073765550863, 0.000000000000000000 ) ) ;
#6187=CARTESIAN_POINT ( 'NONE',  ( -259.2033419157646676, 21.55415060305860209, -21.55415060305812602 ) ) ;
#6189=CARTESIAN_POINT ( 'NONE',  ( 163.1118516004056573, -37.29075403953166301, 19.27778845539196695 ) ) ;
#6190=CARTESIAN_POINT ( 'NONE',  ( -110.0414657791425412, 18.85420805687117607, 7.195370614811373855 ) ) ;
#6191=CARTESIAN_POINT ( 'NONE',  ( -91.56559293963836410, 39.99999999999976552, 22.67402823373234000 ) ) ;
#6192=CARTESIAN_POINT ( 'NONE',  ( 192.4448373802101173, -42.42640687116510634, 14.14213562375845257 ) ) ;
#6193=CARTESIAN_POINT ( 'NONE',  ( -100.7734535825088358, -16.03295912088728770, 16.03295912088687913 ) ) ;
#6194=CARTESIAN_POINT ( 'NONE',  ( -135.8532207217289738, -34.75652343174615311, 21.81201906317767936 ) ) ;
#6195=CARTESIAN_POINT ( 'NONE',  ( 199.9999999999999432, 14.14213562373113398, -14.14213562373094923 ) ) ;
#6197=ADVANCED_FACE ( 'NONE', ( #21045 ), #429, .T. ) ;
#6199=CARTESIAN_POINT ( 'NONE',  ( 0.2972598230769956662, 39.99999999999983658, 54.33493731733950938 ) ) ;
#6201=AXIS2_PLACEMENT_3D ( 'NONE', #12823, #10828, #8828 ) ;
#6202=CARTESIAN_POINT ( 'NONE',  ( 17.65190074000982534, 48.50354960736528653, -14.05440436230914614 ) ) ;
#6203=CARTESIAN_POINT ( 'NONE',  ( -280.0000000000000568, -20.00000000000006750, -40.00000000000002132 ) ) ;
#6205=CARTESIAN_POINT ( 'NONE',  ( -86.96347745069644475, -21.75974354311651737, 0.000000000000000000 ) ) ;
#6206=CARTESIAN_POINT ( 'NONE',  ( -3.856733984649761915, -43.19294614843409619, 17.89110409353252962 ) ) ;
#6207=CARTESIAN_POINT ( 'NONE',  ( -213.1075012329537230, 53.71589010953660193, 40.00000000000002132 ) ) ;
#6210=ORIENTED_EDGE ( 'NONE', *, *, #3627, .T. ) ;
#6211=CARTESIAN_POINT ( 'NONE',  ( 18.90082831370066074, 24.18116416851832540, -43.99399836018032062 ) ) ;
#6213=CARTESIAN_POINT ( 'NONE',  ( 9.345847406404407920, -14.17927947630302832, 49.32890504404208798 ) ) ;
#6214=CARTESIAN_POINT ( 'NONE',  ( 6.984886629791395407, 14.16808340396298149, -49.25486234614871961 ) ) ;
#6216=CARTESIAN_POINT ( 'NONE',  ( -213.1075012329537230, 1.045191102001431893E-13, -13.71589010951911902 ) ) ;
#6217=CARTESIAN_POINT ( 'NONE',  ( 141.7948666911895828, -30.38861427224640366, 12.58737617328886316 ) ) ;
#6218=CARTESIAN_POINT ( 'NONE',  ( -121.8281150764609890, -10.16552078725288588, 22.46071699956211276 ) ) ;
#6219=CARTESIAN_POINT ( 'NONE',  ( 163.1118516004056573, 37.29075403953132906, 19.27778845539275565 ) ) ;
#6220=CARTESIAN_POINT ( 'NONE',  ( -208.1127848780265026, -15.00245453012673202, 0.000000000000000000 ) ) ;
#6221=CARTESIAN_POINT ( 'NONE',  ( -189.1288815661742433, 13.87115472124111193, -47.28031329128402405 ) ) ;
#6222=DIRECTION ( 'NONE',  ( 0.000000000000000000, 1.000000000000000000, 0.000000000000000000 ) ) ;
#6223=CARTESIAN_POINT ( 'NONE',  ( -91.56559293963834989, 40.53558337403654832, 16.03295912088756481 ) ) ;
#6224=CARTESIAN_POINT ( 'NONE',  ( -105.3755690713226585, -18.24025645688355013, 40.00000000000002132 ) ) ;
#6226=CARTESIAN_POINT ( 'NONE',  ( 192.4448373802100889, 19.99999999996064304, 2.449293598294708485E-15 ) ) ;
#6227=CARTESIAN_POINT ( 'NONE',  ( 0.2972598230770030492, -39.99999999999987210, -14.33493731733975451 ) ) ;
#6228=CARTESIAN_POINT ( 'NONE',  ( -192.9588430854689989, 38.51493924976929861, 38.51493924976947625 ) ) ;
#6230=CARTESIAN_POINT ( 'NONE',  ( 98.29820294269173075, 19.99999999998819433, -2.308575297063409524E-13 ) ) ;
#6231=CARTESIAN_POINT ( 'NONE',  ( -105.3755690713226585, 15.38646221621820764, -41.18208027870583265 ) ) ;
#6233=CARTESIAN_POINT ( 'NONE',  ( -30.26275506840324070, -27.08623969584595770, 29.48230279907789608 ) ) ;
#6234=CARTESIAN_POINT ( 'NONE',  ( -93.01854144614468112, 8.553566903488155404, 20.65013722641577942 ) ) ;
#6237=CARTESIAN_POINT ( 'NONE',  ( -105.3755690713226585, -41.18208027870589660, -15.38646221621809040 ) ) ;
#6238=CARTESIAN_POINT ( 'NONE',  ( 2.332272417556284339, -44.41409500754987505, -24.49123061635837217 ) ) ;
#6239=EDGE_CURVE ( 'NONE', #25051, #13683, #16823, .T. ) ;
#6241=CARTESIAN_POINT ( 'NONE',  ( 163.1118516004056573, -27.26290988616869626, 0.000000000000000000 ) ) ;
#6246=CARTESIAN_POINT ( 'NONE',  ( 57.59792236341147031, -1.722363176415032004, -1.722363176415048880 ) ) ;
#6247=CARTESIAN_POINT ( 'NONE',  ( -188.8532066752250955, -43.29285604501843210, -17.93248812771291512 ) ) ;
#6248=CARTESIAN_POINT ( 'NONE',  ( 170.2234770963711128, -39.99999999999991473, -24.55285855007201334 ) ) ;
#6249=CARTESIAN_POINT ( 'NONE',  ( 0.2972598230769930017, 14.33493731733933352, 40.00000000000002132 ) ) ;
#6252=CARTESIAN_POINT ( 'NONE',  ( 170.2234770963711128, -39.99999999999991473, -24.55285855007201334 ) ) ;
#6253=CARTESIAN_POINT ( 'NONE',  ( 146.6084372240433709, -40.00000000000001421, 5.374981219216829587 ) ) ;
#6254=CARTESIAN_POINT ( 'NONE',  ( 200.0000000000000000, 39.99999999999999289, 20.00000000000007105 ) ) ;
#6256=CARTESIAN_POINT ( 'NONE',  ( 0.2972598230770100991, -38.42060263243686791, 38.42060263243645579 ) ) ;
#6257=CARTESIAN_POINT ( 'NONE',  ( 170.2234770963711128, 24.55285855007190321, 0.000000000000000000 ) ) ;
#6258=CARTESIAN_POINT ( 'NONE',  ( 91.82158438592159655, 12.16597498400028776, 44.40256751092339016 ) ) ;
#6259=CARTESIAN_POINT ( 'NONE',  ( 126.3230993689412571, -11.72464299830483014, -28.30579214049048531 ) ) ;
#6260=CARTESIAN_POINT ( 'NONE',  ( 7.340276806054861325, -49.28408872342596680, 14.17250878947614545 ) ) ;
#6261=CARTESIAN_POINT ( 'NONE',  ( 192.4448373802101173, 40.00000000000026290, -19.99999999996018474 ) ) ;
#6262=CARTESIAN_POINT ( 'NONE',  ( -259.2033419157646676, -1.564921101325656229E-13, 30.48217210827739621 ) ) ;
#6263=CARTESIAN_POINT ( 'NONE',  ( -280.0000000000000568, 42.42640687119285303, -14.14213562373088351 ) ) ;
#6264=CARTESIAN_POINT ( 'NONE',  ( -163.5815439473247181, -38.33196286486852955, -12.03526835478797175 ) ) ;
#6266=CARTESIAN_POINT ( 'NONE',  ( 170.2234770963711128, -10.92277846919171935, -45.64576402573189995 ) ) ;
#6267=ORIENTED_EDGE ( 'NONE', *, *, #25724, .F. ) ;
#6268=CARTESIAN_POINT ( 'NONE',  ( -198.0356074513804572, -17.40982414986427429, -39.15871834505933435 ) ) ;
#6269=CARTESIAN_POINT ( 'NONE',  ( -87.02160367299343591, -10.86259082821564981, -18.50714494492524054 ) ) ;
#6270=CARTESIAN_POINT ( 'NONE',  ( 192.4448373802101173, -19.99999999996056843, -40.00000000000002132 ) ) ;
#6271=CARTESIAN_POINT ( 'NONE',  ( -86.94486753505690046, 19.19951378115808893, 9.473579212373534730 ) ) ;
#6272=CARTESIAN_POINT ( 'NONE',  ( -4.039451493210483690, -43.00522595894025812, 23.44932283416647323 ) ) ;
#6276=CARTESIAN_POINT ( 'NONE',  ( -65.65550967573733487, -11.16467289560236509, -24.04430752631839496 ) ) ;
#6277=CARTESIAN_POINT ( 'NONE',  ( 17.65190073994290643, 14.05440436231865320, 48.50354960737508492 ) ) ;
#6282=CARTESIAN_POINT ( 'NONE',  ( -196.0240759113458466, -44.60678620512906889, 24.63338926175166321 ) ) ;
#6284=CARTESIAN_POINT ( 'NONE',  ( 130.8568914410475372, 8.880724697947696879E-14, -5.949712681206690945 ) ) ;
#6285=CARTESIAN_POINT ( 'NONE',  ( 136.1360204305621266, -3.419521671106983309E-13, 35.03383547441296741 ) ) ;
#6289=CARTESIAN_POINT ( 'NONE',  ( -190.7345856381787144, 13.94676320010972859, 47.78725959878661200 ) ) ;
#6290=CARTESIAN_POINT ( 'NONE',  ( 23.17367289775331329, -13.81211338457429427, -46.88342923876911073 ) ) ;
#6291=CARTESIAN_POINT ( 'NONE',  ( -86.96347745069644475, -12.89780903124395195, -12.89780903124416511 ) ) ;
#6292=CARTESIAN_POINT ( 'NONE',  ( -103.9474983244999180, 19.92928099173798628, -8.577167319634817488 ) ) ;
#6293=CARTESIAN_POINT ( 'NONE',  ( 170.2234770963711128, -10.92277846919202666, 10.92277846919193962 ) ) ;
#6295=CARTESIAN_POINT ( 'NONE',  ( 163.1118516004056573, 19.27778845538753316, 19.27778845538783870 ) ) ;
#6296=CARTESIAN_POINT ( 'NONE',  ( 146.6084372240433709, 34.62501878078307982, 40.00000000000002132 ) ) ;
#6297=CARTESIAN_POINT ( 'NONE',  ( 184.8905102610680444, 14.79361573936396113, -14.79361573936377461 ) ) ;
#6298=CARTESIAN_POINT ( 'NONE',  ( -208.1127848780264742, -55.00245453010926866, 40.00000000000002132 ) ) ;
#6299=CARTESIAN_POINT ( 'NONE',  ( -105.4741150117383057, 8.366608964593771347, 19.60045294982731789 ) ) ;
#6300=CARTESIAN_POINT ( 'NONE',  ( -280.0000000000000000, 1.605030083646939673E-13, -20.00000000000001421 ) ) ;
#6301=CARTESIAN_POINT ( 'NONE',  ( 19.06497207195979726, 38.31983398719629719, -18.24870850772750686 ) ) ;
#6302=CARTESIAN_POINT ( 'NONE',  ( -192.9588430854689989, 14.46834944099965981, 0.000000000000000000 ) ) ;
#6304=EDGE_CURVE ( 'NONE', #7462, #10709, #25090, .T. ) ;
#6306=CARTESIAN_POINT ( 'NONE',  ( 57.59792236341147031, -2.435789363418150444, 0.000000000000000000 ) ) ;
#6307=CARTESIAN_POINT ( 'NONE',  ( 156.1979191798868669, 11.34289806466567363, 27.38417834433186471 ) ) ;
#6308=CARTESIAN_POINT ( 'NONE',  ( -162.0762913951020892, 29.48230308784799902, -29.48230308784730980 ) ) ;
#6309=CARTESIAN_POINT ( 'NONE',  ( -105.4293522941955814, -20.05597878317656679, -7.324187428710191128 ) ) ;
#6310=CARTESIAN_POINT ( 'NONE',  ( 163.1118516004056573, -27.26290988616869626, 0.000000000000000000 ) ) ;
#6311=CARTESIAN_POINT ( 'NONE',  ( -163.5815475691942993, 18.59457173339185232, 35.61501186087235027 ) ) ;
#6314=CARTESIAN_POINT ( 'NONE',  ( -56.48582580120559982, 50.09629031063956717, 6.472252184284792875 ) ) ;
#6315=CARTESIAN_POINT ( 'NONE',  ( 19.06497207195982568, -38.31983398719592770, -38.31983398719660272 ) ) ;
#6316=CARTESIAN_POINT ( 'NONE',  ( -110.0305084685578976, 18.59638600693097032, 7.798154251660106340 ) ) ;
#6317=CARTESIAN_POINT ( 'NONE',  ( 14.38125909742180220, 40.00000000000017764, -15.17850393972591760 ) ) ;
#6318=CARTESIAN_POINT ( 'NONE',  ( -30.26275506840324070, -29.48230279907817675, 27.08623969584564151 ) ) ;
#6319=CARTESIAN_POINT ( 'NONE',  ( 170.2234770963711128, -17.36149277827010096, 17.36149277826970660 ) ) ;
#6320=CARTESIAN_POINT ( 'NONE',  ( 170.2234770963711128, -17.36149277826985937, -17.36149277826995174 ) ) ;
#6321=CARTESIAN_POINT ( 'NONE',  ( -30.26275506840324070, -29.48230279907780016, -27.08623969584605362 ) ) ;
#6325=CARTESIAN_POINT ( 'NONE',  ( 146.6084372240433993, 5.715592784339989804E-15, 5.374981219216972583 ) ) ;
#6327=CARTESIAN_POINT ( 'NONE',  ( 23.58679727196860298, 46.73132340480132996, -13.78527791281944737 ) ) ;
#6328=CARTESIAN_POINT ( 'NONE',  ( -192.9588430854690273, 54.46834944098218756, -40.00000000000002132 ) ) ;
#6329=CARTESIAN_POINT ( 'NONE',  ( -280.0000000000000000, -14.14213562373098831, -14.14213562373098654 ) ) ;
#6330=CARTESIAN_POINT ( 'NONE',  ( 146.6084372240433993, -24.48358557860319706, -24.48358557860330720 ) ) ;
#6331=CARTESIAN_POINT ( 'NONE',  ( -4.027137536849500599, -46.99492183298355030, 13.82877337592804956 ) ) ;
#6332=CARTESIAN_POINT ( 'NONE',  ( -192.9588430854690273, 54.46834944101718889, 40.00000000000002132 ) ) ;
#6333=EDGE_LOOP ( 'NONE', ( #11996, #19300, #863, #22353, #19983 ) ) ;
#6334=CARTESIAN_POINT ( 'NONE',  ( -2.652172544013607247, 23.73409167602034131, -43.38951316025613636 ) ) ;
#6335=CARTESIAN_POINT ( 'NONE',  ( 130.8568914410475372, -24.07718906447222551, -24.07718906447233209 ) ) ;
#6337=CARTESIAN_POINT ( 'NONE',  ( -4.061681315507500223, 23.44498947467636185, -42.99867639910915074 ) ) ;
#6340=B_SPLINE_CURVE_WITH_KNOTS ( 'NONE', 3,
 ( #14878, #18746, #20348, #8767, #527, #8632 ),
 .UNSPECIFIED., .F., .F.,
 ( 4, 2, 4 ),
 ( 0.3689590070116580689, 0.3867117631979620773, 0.4044645193949217288 ),
 .UNSPECIFIED. ) ;
#6342=CARTESIAN_POINT ( 'NONE',  ( -188.8948648269077637, -17.93710299892617854, 43.30399732969031135 ) ) ;
#6344=CARTESIAN_POINT ( 'NONE',  ( 192.4448373802101173, -42.42640687122053578, -14.14213562370360577 ) ) ;
#6345=CARTESIAN_POINT ( 'NONE',  ( -93.12335834970889437, -22.67402823373193499, 0.000000000000000000 ) ) ;
#6346=CARTESIAN_POINT ( 'NONE',  ( -195.5008451366929307, 18.44412755962871131, -44.52806290063609396 ) ) ;
#6347=CARTESIAN_POINT ( 'NONE',  ( -192.9588430854690273, 38.51493924976913519, 18.05360324515490333 ) ) ;
#6348=CARTESIAN_POINT ( 'NONE',  ( -30.26275506840325136, 29.48230279907760121, 27.08623969584625613 ) ) ;
#6349=CARTESIAN_POINT ( 'NONE',  ( 170.2234770963711128, -15.44714144992812876, -2.449293598294708485E-15 ) ) ;
#6350=CARTESIAN_POINT ( 'NONE',  ( 146.6084372240433709, 5.374981219216996564, 40.00000000000002132 ) ) ;
#6351=CARTESIAN_POINT ( 'NONE',  ( -198.0356074513804572, 1.247057299367198800E-13, -15.37879056873070560 ) ) ;
#6352=CARTESIAN_POINT ( 'NONE',  ( 192.4448373802100889, 14.14213562370310662, 14.14213562370312438 ) ) ;
#6353=CARTESIAN_POINT ( 'NONE',  ( -93.01741312761465963, 20.82169463873246684, -8.169811846372676101 ) ) ;
#6354=CARTESIAN_POINT ( 'NONE',  ( -208.1127848780264742, -38.89260858015704514, -38.89260858015768463 ) ) ;
#6355=CARTESIAN_POINT ( 'NONE',  ( 91.82158438592156813, 40.45024623143950038, 16.11829626348447420 ) ) ;
#6356=ORIENTED_EDGE ( 'NONE', *, *, #14380, .F. ) ;
#6357=CARTESIAN_POINT ( 'NONE',  ( 170.2234770963711128, -45.64576402573183600, 10.92277846919191653 ) ) ;
#6358=B_SPLINE_CURVE_WITH_KNOTS ( 'NONE', 3,
 ( #19455, #13586, #15455, #19584, #1115, #17333, #1374, #25467, #3492, #9605, #4170, #8264, #6145, #10137, #9739, #14256, #8137, #12264, #14127, #10273, #22394, #23969, #26, #5745, #22255, #16253, #5882 ),
 .UNSPECIFIED., .F., .F.,
 ( 4, 2, 1, 1, 2, 2, 2, 2, 2, 2, 2, 2, 1, 2, 4 ),
 ( -5.999999999696028456E-08, 0.0002171475752860094221, 0.0004343551505720157774, 0.0008687703011440240427, 0.001737600602288037104, 0.003475261204576063443, 0.006950582409152111785, 0.01390122481830420934, 0.02085186722745630342, 0.02432718843203235046, 0.02606484903432037745, 0.02693367933546438747, 0.02736809448603639422, 0.02758530206132240106, 0.02780250963660840791 ),
 .UNSPECIFIED. ) ;
#6359=CARTESIAN_POINT ( 'NONE',  ( -93.01741312761399172, 8.946232117102187686, 20.50009083249028663 ) ) ;
#6360=CARTESIAN_POINT ( 'NONE',  ( 91.82158438592159655, -16.11829626346147393, 16.11829626346132116 ) ) ;
#6361=CARTESIAN_POINT ( 'NONE',  ( -3.786831587084357853, -43.07879808621907358, -23.50387725151980689 ) ) ;
#6364=CARTESIAN_POINT ( 'NONE',  ( -199.9999999999999432, -44.88127304973825460, 30.70179486994645401 ) ) ;
#6365=CIRCLE ( 'NONE', #22104, 15.00000000000000000 ) ;
#6368=CARTESIAN_POINT ( 'NONE',  ( 4.990270234119173587, 14.15117691407241196, -49.14367003637708819 ) ) ;
#6369=CARTESIAN_POINT ( 'NONE',  ( -185.5190930961063316, -42.39056500339492572, -17.55874694107016154 ) ) ;
#6371=CARTESIAN_POINT ( 'NONE',  ( -208.1127848780264742, -40.00000000000025580, 55.00245453014408525 ) ) ;
#6372=CARTESIAN_POINT ( 'NONE',  ( 151.7948205124836534, 6.767089262349056611, 40.00000000000002132 ) ) ;
#6376=CARTESIAN_POINT ( 'NONE',  ( -280.0000000000000568, -40.00000000000014211, 19.99999999999987210 ) ) ;
#6377=CARTESIAN_POINT ( 'NONE',  ( -162.0762913951021176, 39.99999999999998579, 1.694272876828463614 ) ) ;
#6378=CARTESIAN_POINT ( 'NONE',  ( -93.12335834970892279, 16.03295912088714203, -16.03295912088699282 ) ) ;
#6381=CARTESIAN_POINT ( 'NONE',  ( 57.59792236341148453, -37.56421063658185489, -40.00000000000002132 ) ) ;
#6383=CARTESIAN_POINT ( 'NONE',  ( 146.6084372240433993, -3.800685668858652999, 3.800685668858636568 ) ) ;
#6384=CARTESIAN_POINT ( 'NONE',  ( -56.48582580120559271, -1.062504017861011783E-13, 9.153146818113587102 ) ) ;
#6387=CARTESIAN_POINT ( 'NONE',  ( 184.8905102610680444, 39.99999999999983658, 20.92133201514485563 ) ) ;
#6388=CARTESIAN_POINT ( 'NONE',  ( -213.1075012329537230, -2.291445344039133686E-13, 53.71589010951915100 ) ) ;
#6391=CARTESIAN_POINT ( 'NONE',  ( -114.7469200037860162, -17.46524160228793576, 13.55861222482207396 ) ) ;
#6392=CARTESIAN_POINT ( 'NONE',  ( 192.4448373802101173, -14.14213562370283128, -42.42640687122081999 ) ) ;
#6394=CARTESIAN_POINT ( 'NONE',  ( -77.90255099906769942, 20.29001641120658306, -8.064892378658445438 ) ) ;
#6395=CARTESIAN_POINT ( 'NONE',  ( 144.1620285550791607, 30.21661402164566823, -12.51613133675856382 ) ) ;
#6396=CARTESIAN_POINT ( 'NONE',  ( 91.82158438592159655, -22.79471317813468545, -2.449293598294708485E-15 ) ) ;
#6397=CARTESIAN_POINT ( 'NONE',  ( -175.9235632129417866, -39.35891845656527721, 21.03681927447506794 ) ) ;
#6398=CARTESIAN_POINT ( 'NONE',  ( -213.1075012329537230, 13.71589010951907994, 0.000000000000000000 ) ) ;
#6400=ORIENTED_EDGE ( 'NONE', *, *, #24197, .F. ) ;
#6401=ORIENTED_EDGE ( 'NONE', *, *, #20013, .F. ) ;
#6403=CARTESIAN_POINT ( 'NONE',  ( -89.91646883266056989, 8.407637968211338020, -20.29783361036653133 ) ) ;
#6404=CARTESIAN_POINT ( 'NONE',  ( 22.17571259162627939, 23.59965736304510742, 43.20787961118917764 ) ) ;
#6406=VERTEX_POINT ( 'NONE', #11682 ) ;
#6407=CARTESIAN_POINT ( 'NONE',  ( 192.4448373802101173, -42.42640687122073473, 14.14213562370301780 ) ) ;
#6409=CARTESIAN_POINT ( 'NONE',  ( -110.0368417077423118, 7.441767003019926108, 18.74474319002354505 ) ) ;
#6410=CARTESIAN_POINT ( 'NONE',  ( 57.59792236341147031, -1.722363176415032004, -1.722363176415048880 ) ) ;
#6412=CARTESIAN_POINT ( 'NONE',  ( -86.96347745069644475, 41.18208027870598187, -15.38646221621779731 ) ) ;
#6413=FACE_OUTER_BOUND ( 'NONE', #17007, .T. ) ;
#6414=CARTESIAN_POINT ( 'NONE',  ( -96.94449363885368598, -8.590991631001321238, -20.74048850981448311 ) ) ;
#6415=( BOUNDED_SURFACE ( )  B_SPLINE_SURFACE ( 3, 3, ( 
 ( #2488, #24985, #25115, #14457, #18850, #8604, #24579, #22981, #22587, #8735, #10601, #4759, #6735, #2762, #8465, #12863, #20981, #10470, #10869, #10739, #4364, #6335, #18445, #16583, #24845, #22456, #20722, #16714, #2228, #629 ),
 ( #12455, #220, #20582, #22713, #24716, #4625, #14718, #8333, #6470, #14584, #18985, #6598, #12592, #763, #12726, #4235, #2629, #16854, #12324, #20453, #2356, #16457, #3394, #21374, #1273, #19111, #15237, #3269, #5395, #9506 ),
 ( #7127, #11127, #1021, #23614, #9257, #25500, #15109, #21495, #12994, #11490, #23370, #17109, #17363, #1405, #19489, #25375, #9378, #15369, #6865, #5145, #3143, #9122, #13251, #14981, #7247, #11246, #19363, #23492, #5019, #17611 ),
 ( #23115, #11001, #894, #4887, #13124, #19620, #1153, #9004, #17487, #11369, #5266, #25629, #13369, #7375, #21245, #15486, #17234, #21619, #2893, #13497, #21116, #25241, #6993, #23244, #3019, #19240, #4433, #13889, #3523, #20525 ),
 ( #25755, #2294, #3794, #7761, #20658, #22156, #12032, #14528, #10405, #21749, #12526, #5919, #6412, #19882, #2430, #7503, #14027, #11897, #15613, #20020, #5518, #18010, #15873, #22023, #18522, #10541, #25884, #3936, #1801, #9640 ),
 ( #302, #9904, #16527, #8405, #22661, #1665, #24655, #23737, #21878, #13622, #11624, #7627, #17743, #19745, #3656, #26155, #1535, #5782, #7899, #15740, #23870, #16018, #5645, #24143, #13751, #11763, #9773, #17873, #26024, #24000 ),
 ( #22920, #9071, #2838, #10812, #5089, #18923, #3089, #10948, #836, #18652, #21316, #24924, #13193, #15186, #6807, #13071, #4570, #707, #15054, #17178, #438, #967, #6936, #8543, #4832, #8811, #25313, #4699, #23183, #2707 ) ),
 .UNSPECIFIED., .T., .F., .F. ) 
 B_SPLINE_SURFACE_WITH_KNOTS ( ( 4, 3, 4 ),
 ( 4, 2, 2, 2, 2, 2, 2, 2, 2, 2, 2, 2, 2, 2, 4 ),
 ( 0.000000000000000000, 0.5000000000000000000, 1.000000000000000000 ),
 ( 0.000000000000000000, 0.1357259735107005372, 0.1651108541090157700, 0.1944957347073310028, 0.3598804999793158710, 0.3867117631979620773, 0.4135430264166082281, 0.5789277916885930964, 0.6062785021374117456, 0.6336292125862302838, 0.8508620842112317728, 0.8814014469398914198, 0.9119408096685510667, 0.9559704048342755334, 1.000000000000000000 ),
 .UNSPECIFIED. ) 
 GEOMETRIC_REPRESENTATION_ITEM ( )  RATIONAL_B_SPLINE_SURFACE ( (
 ( 1.000000000000000000, 1.000000000000000000, 1.000000000000000000, 1.000000000000000000, 1.000000000000000000, 1.000000000000000000, 1.000000000000000000, 1.000000000000000000, 1.000000000000000000, 1.000000000000000000, 1.000000000000000000, 1.000000000000000000, 1.000000000000000000, 1.000000000000000000, 1.000000000000000000, 1.000000000000000000, 1.000000000000000000, 1.000000000000000000, 1.000000000000000000, 1.000000000000000000, 1.000000000000000000, 1.000000000000000000, 1.000000000000000000, 1.000000000000000000, 1.000000000000000000, 1.000000000000000000, 1.000000000000000000, 1.000000000000000000, 1.000000000000000000, 1.000000000000000000),
 ( 0.3333333333333333703, 0.3333333333333333703, 0.3333333333333333703, 0.3333333333333333703, 0.3333333333333333703, 0.3333333333333333703, 0.3333333333333333703, 0.3333333333333333703, 0.3333333333333333703, 0.3333333333333333703, 0.3333333333333333703, 0.3333333333333333703, 0.3333333333333333703, 0.3333333333333333703, 0.3333333333333333703, 0.3333333333333333703, 0.3333333333333333703, 0.3333333333333333703, 0.3333333333333333703, 0.3333333333333333703, 0.3333333333333333703, 0.3333333333333333703, 0.3333333333333333703, 0.3333333333333333703, 0.3333333333333333703, 0.3333333333333333703, 0.3333333333333333703, 0.3333333333333333703, 0.3333333333333333703, 0.3333333333333333703),
 ( 0.3333333333333333703, 0.3333333333333333703, 0.3333333333333333703, 0.3333333333333333703, 0.3333333333333333703, 0.3333333333333333703, 0.3333333333333333703, 0.3333333333333333703, 0.3333333333333333703, 0.3333333333333333703, 0.3333333333333333703, 0.3333333333333333703, 0.3333333333333333703, 0.3333333333333333703, 0.3333333333333333703, 0.3333333333333333703, 0.3333333333333333703, 0.3333333333333333703, 0.3333333333333333703, 0.3333333333333333703, 0.3333333333333333703, 0.3333333333333333703, 0.3333333333333333703, 0.3333333333333333703, 0.3333333333333333703, 0.3333333333333333703, 0.3333333333333333703, 0.3333333333333333703, 0.3333333333333333703, 0.3333333333333333703),
 ( 1.000000000000000000, 1.000000000000000000, 1.000000000000000000, 1.000000000000000000, 1.000000000000000000, 1.000000000000000000, 1.000000000000000000, 1.000000000000000000, 1.000000000000000000, 1.000000000000000000, 1.000000000000000000, 1.000000000000000000, 1.000000000000000000, 1.000000000000000000, 1.000000000000000000, 1.000000000000000000, 1.000000000000000000, 1.000000000000000000, 1.000000000000000000, 1.000000000000000000, 1.000000000000000000, 1.000000000000000000, 1.000000000000000000, 1.000000000000000000, 1.000000000000000000, 1.000000000000000000, 1.000000000000000000, 1.000000000000000000, 1.000000000000000000, 1.000000000000000000),
 ( 0.3333333333333333703, 0.3333333333333333703, 0.3333333333333333703, 0.3333333333333333703, 0.3333333333333333703, 0.3333333333333333703, 0.3333333333333333703, 0.3333333333333333703, 0.3333333333333333703, 0.3333333333333333703, 0.3333333333333333703, 0.3333333333333333703, 0.3333333333333333703, 0.3333333333333333703, 0.3333333333333333703, 0.3333333333333333703, 0.3333333333333333703, 0.3333333333333333703, 0.3333333333333333703, 0.3333333333333333703, 0.3333333333333333703, 0.3333333333333333703, 0.3333333333333333703, 0.3333333333333333703, 0.3333333333333333703, 0.3333333333333333703, 0.3333333333333333703, 0.3333333333333333703, 0.3333333333333333703, 0.3333333333333333703),
 ( 0.3333333333333333703, 0.3333333333333333703, 0.3333333333333333703, 0.3333333333333333703, 0.3333333333333333703, 0.3333333333333333703, 0.3333333333333333703, 0.3333333333333333703, 0.3333333333333333703, 0.3333333333333333703, 0.3333333333333333703, 0.3333333333333333703, 0.3333333333333333703, 0.3333333333333333703, 0.3333333333333333703, 0.3333333333333333703, 0.3333333333333333703, 0.3333333333333333703, 0.3333333333333333703, 0.3333333333333333703, 0.3333333333333333703, 0.3333333333333333703, 0.3333333333333333703, 0.3333333333333333703, 0.3333333333333333703, 0.3333333333333333703, 0.3333333333333333703, 0.3333333333333333703, 0.3333333333333333703, 0.3333333333333333703),
 ( 1.000000000000000000, 1.000000000000000000, 1.000000000000000000, 1.000000000000000000, 1.000000000000000000, 1.000000000000000000, 1.000000000000000000, 1.000000000000000000, 1.000000000000000000, 1.000000000000000000, 1.000000000000000000, 1.000000000000000000, 1.000000000000000000, 1.000000000000000000, 1.000000000000000000, 1.000000000000000000, 1.000000000000000000, 1.000000000000000000, 1.000000000000000000, 1.000000000000000000, 1.000000000000000000, 1.000000000000000000, 1.000000000000000000, 1.000000000000000000, 1.000000000000000000, 1.000000000000000000, 1.000000000000000000, 1.000000000000000000, 1.000000000000000000, 1.000000000000000000) ) ) 
 REPRESENTATION_ITEM ( '' )  SURFACE ( )  );
#6416=CARTESIAN_POINT ( 'NONE',  ( 151.7948205124836250, 1.012150473917908975E-13, -6.767089262349031742 ) ) ;
#6417=CARTESIAN_POINT ( 'NONE',  ( -135.8532207217289738, 39.99999999999990763, 9.153146818113990335 ) ) ;
#6421=CARTESIAN_POINT ( 'NONE',  ( -173.7925187078237172, 20.60915802531267715, 38.69492115335059879 ) ) ;
#6422=CARTESIAN_POINT ( 'NONE',  ( -213.1075012329537230, -37.98287015391257881, 18.58567234101111509 ) ) ;
#6424=CARTESIAN_POINT ( 'NONE',  ( -105.3755690713226585, 15.38646221621762678, 41.18208027870604582 ) ) ;
#6426=CARTESIAN_POINT ( 'NONE',  ( 170.2234770963711128, 17.36149277827028925, -39.20704971665377059 ) ) ;
#6428=CARTESIAN_POINT ( 'NONE',  ( -162.0762913951020892, -1.694272876828353702, 0.000000000000000000 ) ) ;
#6429=CARTESIAN_POINT ( 'NONE',  ( -280.0000000000000000, -14.14213562373118549, 14.14213562373078936 ) ) ;
#6430=CARTESIAN_POINT ( 'NONE',  ( 200.0000000000000000, 20.00000000000013856, 40.00000000000002132 ) ) ;
#6431=CARTESIAN_POINT ( 'NONE',  ( -109.1264249741457917, -13.72187187121247831, 33.12752917270314157 ) ) ;
#6432=CARTESIAN_POINT ( 'NONE',  ( -56.48582580120560692, 39.99999999999991473, 9.153146818114004546 ) ) ;
#6434=CARTESIAN_POINT ( 'NONE',  ( 110.0479209278585842, -9.419601331808975075, 22.74092928740035191 ) ) ;
#6438=CARTESIAN_POINT ( 'NONE',  ( -208.1127848780265026, 15.00245453012665564, 0.000000000000000000 ) ) ;
#6439=CARTESIAN_POINT ( 'NONE',  ( 153.3020327024399023, 11.77299484472913527, 28.42252382389429499 ) ) ;
#6441=CARTESIAN_POINT ( 'NONE',  ( -30.26275506840323715, 29.48230279907829754, -29.48230279907758344 ) ) ;
#6442=CARTESIAN_POINT ( 'NONE',  ( 90.68848816921392597, 21.47805809169735269, -8.337973099072662819 ) ) ;
#6444=CARTESIAN_POINT ( 'NONE',  ( -196.0240701931630269, 14.12332411430307921, -48.96019555158512304 ) ) ;
#6447=CARTESIAN_POINT ( 'NONE',  ( -135.8532207217289738, -34.75652343174584757, -21.81201906317816253 ) ) ;
#6448=CARTESIAN_POINT ( 'NONE',  ( 14.38125909742181285, -10.73282306404712472, -10.73282306404731301 ) ) ;
#6449=CARTESIAN_POINT ( 'NONE',  ( -114.7831797584708085, 22.13429202244894256, -0.1329151402176787233 ) ) ;
#6450=CARTESIAN_POINT ( 'NONE',  ( 136.1360204305621551, 39.99999999999968026, 35.03383547441337953 ) ) ;
#6451=CARTESIAN_POINT ( 'NONE',  ( 57.59792236341147031, -26.56190807104712448, 30.00663442387673285 ) ) ;
#6452=EDGE_CURVE ( 'NONE', #8800, #22947, #6694, .T. ) ;
#6453=CARTESIAN_POINT ( 'NONE',  ( 12.01676479903290939, 14.17570730777196530, 49.30523874212529023 ) ) ;
#6454=CARTESIAN_POINT ( 'NONE',  ( -114.4364955367314991, -8.644468109207263495, -20.04994829327655737 ) ) ;
#6455=CARTESIAN_POINT ( 'NONE',  ( -56.48582580120558561, -50.09629031063963112, -6.472252184284449150 ) ) ;
#6458=CARTESIAN_POINT ( 'NONE',  ( -135.8532207217289738, -1.351063376314938213E-13, 30.84685318188645553 ) ) ;
#6461=CARTESIAN_POINT ( 'NONE',  ( 23.35901252181226795, 42.86175755505349372, -23.34306388117427389 ) ) ;
#6462=CARTESIAN_POINT ( 'NONE',  ( 136.1360204305621551, 4.966164525587093870, -40.00000000000002132 ) ) ;
#6463=CARTESIAN_POINT ( 'NONE',  ( -86.96347745069644475, -15.38646221621786125, -15.38646221621789856 ) ) ;
#6464=CARTESIAN_POINT ( 'NONE',  ( -192.9588430854690273, 54.46834944101718889, 40.00000000000002132 ) ) ;
#6465=CARTESIAN_POINT ( 'NONE',  ( -70.33906594828840753, -22.79894061172027264, 9.443630411840176819 ) ) ;
#6466=CARTESIAN_POINT ( 'NONE',  ( 136.1360204305621551, -35.03383547441293899, 40.00000000000002132 ) ) ;
#6467=ADVANCED_FACE ( 'NONE', ( #1334 ), #18946, .T. ) ;
#6469=CARTESIAN_POINT ( 'NONE',  ( -199.9999999999999432, 30.70179486994649309, 44.88127304973814802 ) ) ;
#6470=CARTESIAN_POINT ( 'NONE',  ( -135.8532207217289738, -34.75652343174615311, 21.81201906317767936 ) ) ;
#6471=CARTESIAN_POINT ( 'NONE',  ( -16.87994666116329157, -12.91133298910015270, 42.52193590818846758 ) ) ;
#6472=EDGE_CURVE ( 'NONE', #6051, #15971, #334, .T. ) ;
#6473=CARTESIAN_POINT ( 'NONE',  ( -4.031723327955585745, 13.82865651623174763, -46.99313739789371880 ) ) ;
#6475=CARTESIAN_POINT ( 'NONE',  ( -100.7734535825088358, -16.03295912088728770, 16.03295912088687913 ) ) ;
#6477=CARTESIAN_POINT ( 'NONE',  ( -28.75704569508346964, -35.61514925947763288, -18.59466133783093156 ) ) ;
#6478=CARTESIAN_POINT ( 'NONE',  ( -198.9233928134166831, -24.80620717265403030, 44.84148042516471833 ) ) ;
#6479=CARTESIAN_POINT ( 'NONE',  ( -86.96347745069643054, -40.00000000000026290, 21.75974354311608749 ) ) ;
#6481=CARTESIAN_POINT ( 'NONE',  ( 19.06497207195981858, 10.03556273973516078, -66.60410523465806421 ) ) ;
#6482=CARTESIAN_POINT ( 'NONE',  ( 0.2972598230769983307, -14.33493731733933352, 0.000000000000000000 ) ) ;
#6483=CARTESIAN_POINT ( 'NONE',  ( -188.9266751785346230, 17.94050871568887118, -43.31221945728822931 ) ) ;
#6484=CARTESIAN_POINT ( 'NONE',  ( 57.59792236341147031, 54.84617931850878136, 1.722363176415705910 ) ) ;
#6485=CARTESIAN_POINT ( 'NONE',  ( -192.9588430854690273, 38.51493924976913519, 18.05360324515490333 ) ) ;
#6486=CARTESIAN_POINT ( 'NONE',  ( 146.6084372240433709, -5.374981219216942385, -40.00000000000002132 ) ) ;
#6487=CARTESIAN_POINT ( 'NONE',  ( -100.7734535825088500, 17.32597176626808988, 40.00000000000002132 ) ) ;
#6488=CARTESIAN_POINT ( 'NONE',  ( -213.1075012329537230, -39.99999999999991473, -13.71589010951953647 ) ) ;
#6489=CARTESIAN_POINT ( 'NONE',  ( 19.06497207195981858, 10.03556273973424062, 66.60410523465820631 ) ) ;
#6490=CARTESIAN_POINT ( 'NONE',  ( 98.29820294267327085, -1.310413973320513126, 20.00000000000587264 ) ) ;
#6491=CARTESIAN_POINT ( 'NONE',  ( 57.59792236341148453, -26.56190807104663421, -26.56190807104710672 ) ) ;
#6492=CARTESIAN_POINT ( 'NONE',  ( -114.6382724355124623, 5.497872032160218581, 21.35157561685027972 ) ) ;
#6494=CARTESIAN_POINT ( 'NONE',  ( -100.7734535825088500, -44.31723036834903695, 12.25131212657476709 ) ) ;
#6495=FACE_OUTER_BOUND ( 'NONE', #12453, .T. ) ;
#6496=CARTESIAN_POINT ( 'NONE',  ( 184.8905102610680444, 14.79361573936366092, 41.77492675556006674 ) ) ;
#6497=CARTESIAN_POINT ( 'NONE',  ( -0.6848998192559355713, -48.06291537635265598, -13.98809697771682004 ) ) ;
#6498=EDGE_LOOP ( 'NONE', ( #12422, #4061, #18115, #8361, #2320 ) ) ;
#6501=ORIENTED_EDGE ( 'NONE', *, *, #1020, .F. ) ;
#6504=CARTESIAN_POINT ( 'NONE',  ( -189.1288815661534386, -47.28031329127756521, -13.87115472123938709 ) ) ;
#6505=CARTESIAN_POINT ( 'NONE',  ( -135.8532207217289738, -1.351063376314938213E-13, 30.84685318188645553 ) ) ;
#6506=CARTESIAN_POINT ( 'NONE',  ( -280.0000000000000568, 19.99999999999996447, -40.00000000000002132 ) ) ;
#6509=CARTESIAN_POINT ( 'NONE',  ( 136.1360204305621266, 5.219216885335291329E-15, 4.966164525587064560 ) ) ;
#6510=CARTESIAN_POINT ( 'NONE',  ( 192.4448373802101173, 40.00000000000012790, -20.00000000003928236 ) ) ;
#6512=CARTESIAN_POINT ( 'NONE',  ( -114.4364955367314707, 8.064892380844273845, -20.29001642038674902 ) ) ;
#6513=CARTESIAN_POINT ( 'NONE',  ( -213.1075012329536946, -53.71589010951918652, -2.449293598294708485E-15 ) ) ;
#6514=CARTESIAN_POINT ( 'NONE',  ( 170.2234770963711128, -10.92277846919202666, 10.92277846919193962 ) ) ;
#6515=CARTESIAN_POINT ( 'NONE',  ( 155.1206158682454088, -11.51471166709232818, -27.79897307351034286 ) ) ;
#6516=CARTESIAN_POINT ( 'NONE',  ( -105.2502192157478049, 17.39781795296955735, -12.58588914168777251 ) ) ;
#6517=CARTESIAN_POINT ( 'NONE',  ( -162.0762913951020892, 4.094006889353306706E-13, -41.69427287682835015 ) ) ;
#6518=CARTESIAN_POINT ( 'NONE',  ( 146.6084372240433709, -40.00000000000001421, 5.374981219216829587 ) ) ;
#6519=CARTESIAN_POINT ( 'NONE',  ( -213.1075012329537230, 9.698598906450410340, 9.698598906450483170 ) ) ;
#6522=CARTESIAN_POINT ( 'NONE',  ( -162.0762913951020892, -29.48230308784785692, 29.48230308784751230 ) ) ;
#6524=FACE_OUTER_BOUND ( 'NONE', #21947, .T. ) ;
#6525=CARTESIAN_POINT ( 'NONE',  ( 130.1167162091014404, 29.33455044752968277, -12.15076864148447200 ) ) ;
#6526=CARTESIAN_POINT ( 'NONE',  ( 136.1360204305621266, 35.03383547441298163, -40.00000000000002132 ) ) ;
#6527=ADVANCED_FACE ( 'NONE', ( #19839 ), #11022, .T. ) ;
#6528=CARTESIAN_POINT ( 'NONE',  ( -105.4741150117383057, 8.366608964593771347, 19.60045294982731789 ) ) ;
#6529=CARTESIAN_POINT ( 'NONE',  ( 199.9999999999999432, -14.14213562373115884, 14.14213562373085153 ) ) ;
#6531=VERTEX_POINT ( 'NONE', #16873 ) ;
#6532=CARTESIAN_POINT ( 'NONE',  ( -103.9474983245025186, 8.577167319634602549, -19.92928099173750311 ) ) ;
#6533=CARTESIAN_POINT ( 'NONE',  ( -89.91498783736599876, 8.733585467966305416, -20.17141720489794210 ) ) ;
#6534=CARTESIAN_POINT ( 'NONE',  ( 22.76403192593477343, 17.88468650128198689, 43.17745271018618070 ) ) ;
#6536=ORIENTED_EDGE ( 'NONE', *, *, #24547, .T. ) ;
#6538=CARTESIAN_POINT ( 'NONE',  ( -91.56559293963834989, -44.31723036834903695, 12.25131212657476709 ) ) ;
#6540=CARTESIAN_POINT ( 'NONE',  ( -114.7248266913260295, 3.464717969334141667, 21.81737765724340861 ) ) ;
#6542=CARTESIAN_POINT ( 'NONE',  ( -105.3755690713226727, -15.38646221621786481, -15.38646221621789856 ) ) ;
#6543=CARTESIAN_POINT ( 'NONE',  ( -105.2285682121444808, 21.34137888092660518, 2.786758726753435500 ) ) ;
#6544=CARTESIAN_POINT ( 'NONE',  ( -87.13361725327072804, 21.49321519333427233, -1.448021113139547951E-30 ) ) ;
#6545=CARTESIAN_POINT ( 'NONE',  ( -109.1264249741455217, 33.12752917269229158, -13.72187187124002783 ) ) ;
#6546=CARTESIAN_POINT ( 'NONE',  ( -259.2033419157646676, 2.741182173978444749E-13, -30.48217210827739621 ) ) ;
#6547=CARTESIAN_POINT ( 'NONE',  ( -105.3755690713226727, -2.472783935621397949E-13, 21.75974354311649961 ) ) ;
#6549=DIRECTION ( 'NONE',  ( 1.000000000000000000, 0.000000000000000000, 0.000000000000000000 ) ) ;
#6551=CARTESIAN_POINT ( 'NONE',  ( -189.1288337602708509, 13.87115233298066030, 47.28029723722608679 ) ) ;
#6552=CARTESIAN_POINT ( 'NONE',  ( 151.7948205124836250, 23.49921654116328540, 23.49921654116366554 ) ) ;
#6554=CARTESIAN_POINT ( 'NONE',  ( -208.1127848780264742, -10.60833733268345469, 67.17687982760682530 ) ) ;
#6555=CARTESIAN_POINT ( 'NONE',  ( -77.90255099907052738, 8.064892378688679031, 20.29001641119211641 ) ) ;
#6556=CARTESIAN_POINT ( 'NONE',  ( 130.8568914410475088, 52.36146031193427319, -4.207082182989173802 ) ) ;
#6557=DIRECTION ( 'NONE',  ( -0.7071067811865501263, 0.7071067811865449082, 8.659560562354902043E-17 ) ) ;
#6558=CARTESIAN_POINT ( 'NONE',  ( -100.7734535825088500, 22.67402823373189591, -0.000000000000000000 ) ) ;
#6559=CARTESIAN_POINT ( 'NONE',  ( 0.2972598230769886718, 38.42060263243643448, 18.14793986248763957 ) ) ;
#6560=CARTESIAN_POINT ( 'NONE',  ( 19.06497207195981503, -14.19242893257840166, 0.000000000000000000 ) ) ;
#6561=CARTESIAN_POINT ( 'NONE',  ( -88.39148973765139772, 20.15708830332379975, -8.027153355909627308 ) ) ;
#6562=CARTESIAN_POINT ( 'NONE',  ( -30.26275506840323359, -39.99999999999959499, -41.69427246844670520 ) ) ;
#6566=ORIENTED_EDGE ( 'NONE', *, *, #543, .F. ) ;
#6567=CARTESIAN_POINT ( 'NONE',  ( 136.1360204305621551, 4.966164525587085876, 40.00000000000002132 ) ) ;
#6568=ADVANCED_FACE ( 'NONE', ( #23391 ), #9703, .T. ) ;
#6570=CARTESIAN_POINT ( 'NONE',  ( -213.1075012329537230, 37.98287015391280619, -37.98287015391192512 ) ) ;
#6571=CARTESIAN_POINT ( 'NONE',  ( -114.7248266913117760, -21.81737765723738320, 3.464717969335482373 ) ) ;
#6576=B_SPLINE_CURVE_WITH_KNOTS ( 'NONE', 3,
 ( #23225, #5130, #9107, #6714, #2878, #14828 ),
 .UNSPECIFIED., .F., .F.,
 ( 4, 2, 4 ),
 ( 0.000000000000000000, 0.004167810130244177513, 0.008335620260488355027 ),
 .UNSPECIFIED. ) ;
#6578=CARTESIAN_POINT ( 'NONE',  ( -238.4067589809705794, -27.60227080167029001, -28.96627169325357798 ) ) ;
#6579=CARTESIAN_POINT ( 'NONE',  ( -30.26275506840324070, -1.198031551616016266, -1.198031551616031587 ) ) ;
#6580=CARTESIAN_POINT ( 'NONE',  ( 170.0000000000000284, -22.62041470344884431, 9.369682556672202622 ) ) ;
#6581=CARTESIAN_POINT ( 'NONE',  ( -86.96347745069645896, 39.99999999999977973, 21.75974354311691883 ) ) ;
#6582=CARTESIAN_POINT ( 'NONE',  ( -89.92902785008683963, -8.088236460650220394, 20.44110050034126758 ) ) ;
#6583=CARTESIAN_POINT ( 'NONE',  ( 22.82385994800817386, 13.83113328680598464, 47.01156385802197235 ) ) ;
#6584=CARTESIAN_POINT ( 'NONE',  ( 199.9999999999999432, -14.14213562373115884, 14.14213562373085153 ) ) ;
#6585=CARTESIAN_POINT ( 'NONE',  ( 199.9999999999999432, -14.14213562373093680, 14.14213562373082311 ) ) ;
#6587=CARTESIAN_POINT ( 'NONE',  ( -105.3755690713226727, -8.549198663894545631E-14, 18.24025645688352881 ) ) ;
#6588=CARTESIAN_POINT ( 'NONE',  ( 22.78333232259046071, 43.17211919388257257, -17.88247728649356461 ) ) ;
#6589=CARTESIAN_POINT ( 'NONE',  ( -213.1075012329537230, 13.71589010951907994, 0.000000000000000000 ) ) ;
#6590=CARTESIAN_POINT ( 'NONE',  ( 0.2972598230769990524, -18.14793986248724522, 38.42060263243662632 ) ) ;
#6591=CARTESIAN_POINT ( 'NONE',  ( -198.0356074513804572, 15.37879056873066830, 40.00000000000002132 ) ) ;
#6592=CARTESIAN_POINT ( 'NONE',  ( -4.439300432583311640, -42.88738538954532942, 23.37136716947943071 ) ) ;
#6595=CARTESIAN_POINT ( 'NONE',  ( 136.1360204305621551, 4.966164525587085876, 40.00000000000002132 ) ) ;
#6596=ORIENTED_EDGE ( 'NONE', *, *, #19245, .F. ) ;
#6597=CARTESIAN_POINT ( 'NONE',  ( -199.9999999999999432, 35.57044988732131685, 42.45148791631880414 ) ) ;
#6598=CARTESIAN_POINT ( 'NONE',  ( -91.56559293963834989, -44.31723036834903695, 12.25131212657476709 ) ) ;
#6599=CARTESIAN_POINT ( 'NONE',  ( -4.421177063218048708, -23.37490463203918267, 42.89273859401259870 ) ) ;
#6600=CARTESIAN_POINT ( 'NONE',  ( -4.076660308449207903, 23.44206949513791116, -42.99426297939334773 ) ) ;
#6602=CARTESIAN_POINT ( 'NONE',  ( -213.1075012329537230, 37.98287015391211696, 18.58567234101190735 ) ) ;
#6603=CARTESIAN_POINT ( 'NONE',  ( -82.24465949241034934, -20.03613703209230579, 2.525178489117738678 ) ) ;
#6605=CARTESIAN_POINT ( 'NONE',  ( -192.9370379451729036, -14.03127537977607453, 48.35015161801144501 ) ) ;
#6606=CARTESIAN_POINT ( 'NONE',  ( 19.06497207195981147, 1.521599808664285085E-13, -14.19242893257840521 ) ) ;
#6607=CARTESIAN_POINT ( 'NONE',  ( 146.6084372240433709, -52.76785682606510619, -3.800685668859292043 ) ) ;
#6608=CARTESIAN_POINT ( 'NONE',  ( -105.3755690713226585, 43.67073346367988051, -12.89780903124366418 ) ) ;
#6611=CARTESIAN_POINT ( 'NONE',  ( 146.6084372240433993, 24.48358557860307272, 24.48358557860347418 ) ) ;
#6612=CARTESIAN_POINT ( 'NONE',  ( -238.4067589809705794, 28.96627169325354956, -28.96627169325289231 ) ) ;
#6613=CARTESIAN_POINT ( 'NONE',  ( -105.3755690713226585, 12.89780903124349720, 43.67073346367994446 ) ) ;
#6614=EDGE_CURVE ( 'NONE', #15079, #1078, #23514, .T. ) ;
#6615=CARTESIAN_POINT ( 'NONE',  ( 130.8568914410475088, -5.949712681206664300, -40.00000000000002132 ) ) ;
#6616=CARTESIAN_POINT ( 'NONE',  ( 130.8568914410475088, 5.949712681206712261, 40.00000000000002132 ) ) ;
#6617=CARTESIAN_POINT ( 'NONE',  ( 91.82158438592159655, -40.00000000000017764, 17.20528682183258340 ) ) ;
#6618=CARTESIAN_POINT ( 'NONE',  ( -213.1075012329537230, 9.698598906450410340, 9.698598906450483170 ) ) ;
#6619=CARTESIAN_POINT ( 'NONE',  ( -105.4741150117378936, 19.60045294982725750, -8.366608964594151487 ) ) ;
#6620=CARTESIAN_POINT ( 'NONE',  ( -105.3755690713226727, -12.89780903124395550, -12.89780903124416511 ) ) ;
#6621=CARTESIAN_POINT ( 'NONE',  ( -114.7756899093956946, 1.373957298918453418, 22.09342955265359620 ) ) ;
#6622=EDGE_LOOP ( 'NONE', ( #10364, #7395, #22213, #26292, #9192, #24198, #17046, #1460, #10674 ) ) ;
#6624=CARTESIAN_POINT ( 'NONE',  ( 0.2972598230769959993, 38.42060263243659080, 38.42060263243672580 ) ) ;
#6625=CARTESIAN_POINT ( 'NONE',  ( -96.94449363884535842, 8.590991631016400731, 20.74048850978408964 ) ) ;
#6627=CARTESIAN_POINT ( 'NONE',  ( 19.06497207195982568, -38.31983398719646061, 38.31983398719606271 ) ) ;
#6628=CARTESIAN_POINT ( 'NONE',  ( 20.16956056503547856, -43.71646652951510958, -23.97604322319288528 ) ) ;
#6629=EDGE_CURVE ( 'NONE', #19209, #8490, #7252, .T. ) ;
#6630=EDGE_LOOP ( 'NONE', ( #25495, #11988 ) ) ;
#6632=CARTESIAN_POINT ( 'NONE',  ( -200.0000000000000000, -35.57044988732172186, 42.45148791632026075 ) ) ;
#6636=CARTESIAN_POINT ( 'NONE',  ( 4.995406935893288214, 55.24977328853207581, 40.00000000000002132 ) ) ;
#6640=CARTESIAN_POINT ( 'NONE',  ( -30.26275506840324070, -29.48230279907817675, 27.08623969584564151 ) ) ;
#6641=CARTESIAN_POINT ( 'NONE',  ( -238.4067589809705794, 39.99999999999983658, 40.96449428006354765 ) ) ;
#6642=CARTESIAN_POINT ( 'NONE',  ( 146.6084372240433709, 40.00000000000017053, -34.62501878078291639 ) ) ;
#6643=CARTESIAN_POINT ( 'NONE',  ( -3.903133374353591645, 47.03983734332609146, -13.83543723425202465 ) ) ;
#6644=CARTESIAN_POINT ( 'NONE',  ( -213.1075012329537230, -13.71589010951915810, 0.000000000000000000 ) ) ;
#6646=CARTESIAN_POINT ( 'NONE',  ( -259.2033419157646676, -30.48217210827744239, -2.449293598294708485E-15 ) ) ;
#6647=CARTESIAN_POINT ( 'NONE',  ( 4.995406935893301537, -10.78321810390187530, 67.35176059882529387 ) ) ;
#6648=CARTESIAN_POINT ( 'NONE',  ( 133.2080217031555662, -12.38638889282717415, -29.90338805389119869 ) ) ;
#6649=CARTESIAN_POINT ( 'NONE',  ( -114.7827252410365020, 16.13252424104745941, -15.16659028662510877 ) ) ;
#6650=CARTESIAN_POINT ( 'NONE',  ( -198.0356074513804572, 40.00000000000056843, -55.37879056871282302 ) ) ;
#6651=CARTESIAN_POINT ( 'NONE',  ( -105.3755690713226585, 39.99999999999993605, 18.24025645688366737 ) ) ;
#6652=CARTESIAN_POINT ( 'NONE',  ( 57.59792236341147031, -1.722363176415032004, -1.722363176415048880 ) ) ;
#6655=CARTESIAN_POINT ( 'NONE',  ( 4.995406935893305977, -39.06748935135212264, 39.06748935135171763 ) ) ;
#6657=CARTESIAN_POINT ( 'NONE',  ( 130.8568914410475372, 24.07718906447210472, 24.07718906447249907 ) ) ;
#6658=CARTESIAN_POINT ( 'NONE',  ( -62.79433447044806371, 25.93934121804208104, -9.335111860717981713 ) ) ;
#6660=CARTESIAN_POINT ( 'NONE',  ( -56.48582580120558561, -30.84685318188645553, -40.00000000000002132 ) ) ;
#6665=CARTESIAN_POINT ( 'NONE',  ( 48.46159092537990887, -11.89574569450918062, 37.63079858261905741 ) ) ;
#6666=CARTESIAN_POINT ( 'NONE',  ( -100.0957100001467381, 8.517115559260357571, -20.56213589538073094 ) ) ;
#6667=CARTESIAN_POINT ( 'NONE',  ( 12.96694272570842799, 14.15914421029697579, 49.19577900137000626 ) ) ;
#6670=ORIENTED_EDGE ( 'NONE', *, *, #14441, .F. ) ;
#6671=CARTESIAN_POINT ( 'NONE',  ( -91.56559293963834989, -16.03295912088716335, 40.53558337403673306 ) ) ;
#6673=CARTESIAN_POINT ( 'NONE',  ( -105.4741150117371262, -7.943527260734682294, 19.77569912955828357 ) ) ;
#6674=CARTESIAN_POINT ( 'NONE',  ( 170.2234770963711128, -45.64576402573183600, 10.92277846919191653 ) ) ;
#6676=CARTESIAN_POINT ( 'NONE',  ( -86.96347745069645896, 39.99999999999994316, 18.24025645688366737 ) ) ;
#6679=CARTESIAN_POINT ( 'NONE',  ( -100.7734535825088358, 1.654174317907124744E-13, -17.32597176626811120 ) ) ;
#6680=CARTESIAN_POINT ( 'NONE',  ( -30.26275506840325136, 40.00000000000003553, -1.694272468445841007 ) ) ;
#6684=CARTESIAN_POINT ( 'NONE',  ( -187.3036811847924810, 13.75782060303311738, 46.64553187116074895 ) ) ;
#6685=B_SPLINE_CURVE_WITH_KNOTS ( 'NONE', 3,
 ( #7940, #5958, #20462, #14067, #22464, #775 ),
 .UNSPECIFIED., .F., .F.,
 ( 4, 2, 4 ),
 ( 0.000000000000000000, 0.004089982295592885925, 0.008179964591185771849 ),
 .UNSPECIFIED. ) ;
#6686=CARTESIAN_POINT ( 'NONE',  ( -208.1127848780265026, -10.60833733269537227, -10.60833733269551793 ) ) ;
#6687=CARTESIAN_POINT ( 'NONE',  ( -105.4741150117383057, 8.366608964593771347, 19.60045294982731789 ) ) ;
#6688=CARTESIAN_POINT ( 'NONE',  ( -259.2033419157646676, 35.01439189186528722, 21.55415060305857011 ) ) ;
#6689=CARTESIAN_POINT ( 'NONE',  ( -77.56366795221718746, 1.395416561020218715, 22.09173432935380887 ) ) ;
#6690=CARTESIAN_POINT ( 'NONE',  ( -135.8532207217289738, 6.472252184284583265, -50.09629031063960980 ) ) ;
#6692=CARTESIAN_POINT ( 'NONE',  ( 98.29820294273291381, -18.47759065023123526, -7.653668647304108674 ) ) ;
#6693=CARTESIAN_POINT ( 'NONE',  ( 4.995406935893283773, 39.06748935135171052, 17.50105314357239195 ) ) ;
#6694=B_SPLINE_CURVE_WITH_KNOTS ( 'NONE', 3,
 ( #13553, #25683, #5578, #7431, #15545, #15422, #11182, #11306, #25813, #13430, #7064, #21806 ),
 .UNSPECIFIED., .F., .F.,
 ( 4, 2, 2, 2, 2, 4 ),
 ( 1.158526472511095878E-15, 0.004680202113614856732, 0.009360404227228554669, 0.01170050528403540277, 0.01404060634084225261, 0.01872080845445590891 ),
 .UNSPECIFIED. ) ;
#6695=CARTESIAN_POINT ( 'NONE',  ( -56.48582580120559982, 9.153146818113574668, 40.00000000000002132 ) ) ;
#6698=CARTESIAN_POINT ( 'NONE',  ( -105.3755690713226585, -40.00000000000027711, 21.75974354311608749 ) ) ;
#6703=CARTESIAN_POINT ( 'NONE',  ( -135.8532207217289738, 30.84685318188643066, 2.449293598294708485E-15 ) ) ;
#6705=CARTESIAN_POINT ( 'NONE',  ( -105.4741150117398405, -19.77569912953930142, 7.943527260776874321 ) ) ;
#6706=EDGE_CURVE ( 'NONE', #961, #13948, #1603, .T. ) ;
#6707=CARTESIAN_POINT ( 'NONE',  ( -109.1264249741452090, 13.72187187126506025, -33.12752917268247188 ) ) ;
#6708=CARTESIAN_POINT ( 'NONE',  ( 0.2972598230770030492, -40.00000000000007816, 14.33493731733919496 ) ) ;
#6711=CARTESIAN_POINT ( 'NONE',  ( -105.2054292635176864, 1.371497798096047660, -21.49321519473980757 ) ) ;
#6712=CARTESIAN_POINT ( 'NONE',  ( 170.2234770963711128, -45.64576402573167258, -10.92277846919254891 ) ) ;
#6713=CARTESIAN_POINT ( 'NONE',  ( -238.4067589809705794, -0.6820004457913585449, -0.6820004457913265705 ) ) ;
#6714=CARTESIAN_POINT ( 'NONE',  ( -77.70105001122996669, -18.98740555847804856, -11.20619870950665309 ) ) ;
#6715=CARTESIAN_POINT ( 'NONE',  ( 0.2972598230769883387, 40.00000000000017053, -14.33493731733891607 ) ) ;
#6716=CARTESIAN_POINT ( 'NONE',  ( 57.59792236341147031, 1.722363176415040886, 1.722363176415060426 ) ) ;
#6717=CARTESIAN_POINT ( 'NONE',  ( -3.903133374380808984, 13.83543723414519810, 47.03983734341694856 ) ) ;
#6718=CARTESIAN_POINT ( 'NONE',  ( 192.4448373802100889, -14.14213562375896061, 14.14213562375865330 ) ) ;
#6719=ADVANCED_FACE ( 'NONE', ( #13680 ), #11400, .T. ) ;
#6721=CARTESIAN_POINT ( 'NONE',  ( 136.1360204305621266, -3.511608612530682905, 3.511608612530666917 ) ) ;
#6724=CARTESIAN_POINT ( 'NONE',  ( -30.26275506840324070, -1.147469862568086380E-14, 1.694272468446259783 ) ) ;
#6725=CARTESIAN_POINT ( 'NONE',  ( 67.79414719560435287, 30.31905270963685339, -10.30785037341317611 ) ) ;
#6726=CARTESIAN_POINT ( 'NONE',  ( 163.1118516004056573, -27.26290988616869626, -40.00000000000002132 ) ) ;
#6727=CARTESIAN_POINT ( 'NONE',  ( 19.06497207195980792, 10.03556273973433299, 10.03556273973436319 ) ) ;
#6728=CARTESIAN_POINT ( 'NONE',  ( 151.7948205124836250, -33.23291073765550863, 0.000000000000000000 ) ) ;
#6729=ORIENTED_EDGE ( 'NONE', *, *, #18576, .F. ) ;
#6730=( BOUNDED_SURFACE ( )  B_SPLINE_SURFACE ( 3, 3, ( 
 ( #9123, #1154, #17235, #13125, #15487, #21620, #9507, #9258, #19364, #11247, #23371, #3144, #21246, #9379, #7376, #11491, #17364, #5267, #25501, #11002, #7248, #5396, #15370, #11128, #19241, #19490, #2894, #1406, #1022, #12995 ),
 ( #15110, #13370, #25376, #895, #23245, #5146, #15239, #21496, #13498, #3395, #19621, #19112, #13252, #21375, #17612, #25756, #7504, #23116, #4888, #21117, #25242, #9005, #17110, #14028, #12170, #9774, #22024, #1666, #19883, #5783 ),
 ( #3937, #64, #1802, #4067, #9905, #3795, #26295, #26025, #1933, #22157, #20152, #22291, #19746, #23738, #18146, #18011, #13890, #17874, #26157, #16019, #7762, #7900, #11898, #21879, #20289, #24002, #24144, #15874, #2068, #11625 ),
 ( #15741, #10175, #20021, #5920, #3657, #12033, #18279, #10039, #15614, #8035, #16154, #5519, #24285, #6055, #14159, #13623, #21750, #3524, #1536, #9641, #17744, #25885, #7628, #23871, #5646, #13752, #11764, #15055, #12939, #24415 ),
 ( #20929, #21054, #2708, #24925, #968, #7073, #21317, #2839, #4833, #23061, #8812, #14922, #6676, #13072, #2960, #23313, #10949, #17054, #19055, #22428, #837, #19185, #8946, #16789, #4700, #23184, #14293, #13194, #14791, #6180 ),
 ( #4964, #25188, #15187, #6937, #574, #19305, #9072, #8173, #16288, #21188, #22921, #11070, #2565, #10813, #12806, #4203, #8679, #18924, #17179, #16923, #12667, #25314, #5090, #708, #3090, #11190, #20794, #10682, #18793, #25057 ),
 ( #6808, #5331, #17554, #21689, #15556, #1346, #13440, #21954, #7569, #19433, #9448, #9322, #15682, #7192, #5715, #25692, #11316, #11562, #3728, #13695, #19556, #21818, #9574, #1090, #7442, #23681, #3335, #5460, #9198, #19682 ) ),
 .UNSPECIFIED., .T., .F., .T. ) 
 B_SPLINE_SURFACE_WITH_KNOTS ( ( 4, 3, 4 ),
 ( 4, 2, 2, 2, 2, 2, 2, 2, 2, 2, 2, 2, 2, 2, 4 ),
 ( 0.000000000000000000, 0.5000000000000000000, 1.000000000000000000 ),
 ( 0.000000000000000000, 0.1357259735107005372, 0.1651108541090157700, 0.1944957347073310028, 0.3598804999793158710, 0.3867117631979620773, 0.4135430264166082281, 0.5789277916885930964, 0.6062785021374117456, 0.6336292125862302838, 0.8508620842112317728, 0.8814014469398914198, 0.9119408096685510667, 0.9559704048342755334, 1.000000000000000000 ),
 .UNSPECIFIED. ) 
 GEOMETRIC_REPRESENTATION_ITEM ( )  RATIONAL_B_SPLINE_SURFACE ( (
 ( 1.000000000000000000, 1.000000000000000000, 1.000000000000000000, 1.000000000000000000, 1.000000000000000000, 1.000000000000000000, 1.000000000000000000, 1.000000000000000000, 1.000000000000000000, 1.000000000000000000, 1.000000000000000000, 1.000000000000000000, 1.000000000000000000, 1.000000000000000000, 1.000000000000000000, 1.000000000000000000, 1.000000000000000000, 1.000000000000000000, 1.000000000000000000, 1.000000000000000000, 1.000000000000000000, 1.000000000000000000, 1.000000000000000000, 1.000000000000000000, 1.000000000000000000, 1.000000000000000000, 1.000000000000000000, 1.000000000000000000, 1.000000000000000000, 1.000000000000000000),
 ( 0.3333333333333333703, 0.3333333333333333703, 0.3333333333333333703, 0.3333333333333333703, 0.3333333333333333703, 0.3333333333333333703, 0.3333333333333333703, 0.3333333333333333703, 0.3333333333333333703, 0.3333333333333333703, 0.3333333333333333703, 0.3333333333333333703, 0.3333333333333333703, 0.3333333333333333703, 0.3333333333333333703, 0.3333333333333333703, 0.3333333333333333703, 0.3333333333333333703, 0.3333333333333333703, 0.3333333333333333703, 0.3333333333333333703, 0.3333333333333333703, 0.3333333333333333703, 0.3333333333333333703, 0.3333333333333333703, 0.3333333333333333703, 0.3333333333333333703, 0.3333333333333333703, 0.3333333333333333703, 0.3333333333333333703),
 ( 0.3333333333333333703, 0.3333333333333333703, 0.3333333333333333703, 0.3333333333333333703, 0.3333333333333333703, 0.3333333333333333703, 0.3333333333333333703, 0.3333333333333333703, 0.3333333333333333703, 0.3333333333333333703, 0.3333333333333333703, 0.3333333333333333703, 0.3333333333333333703, 0.3333333333333333703, 0.3333333333333333703, 0.3333333333333333703, 0.3333333333333333703, 0.3333333333333333703, 0.3333333333333333703, 0.3333333333333333703, 0.3333333333333333703, 0.3333333333333333703, 0.3333333333333333703, 0.3333333333333333703, 0.3333333333333333703, 0.3333333333333333703, 0.3333333333333333703, 0.3333333333333333703, 0.3333333333333333703, 0.3333333333333333703),
 ( 1.000000000000000000, 1.000000000000000000, 1.000000000000000000, 1.000000000000000000, 1.000000000000000000, 1.000000000000000000, 1.000000000000000000, 1.000000000000000000, 1.000000000000000000, 1.000000000000000000, 1.000000000000000000, 1.000000000000000000, 1.000000000000000000, 1.000000000000000000, 1.000000000000000000, 1.000000000000000000, 1.000000000000000000, 1.000000000000000000, 1.000000000000000000, 1.000000000000000000, 1.000000000000000000, 1.000000000000000000, 1.000000000000000000, 1.000000000000000000, 1.000000000000000000, 1.000000000000000000, 1.000000000000000000, 1.000000000000000000, 1.000000000000000000, 1.000000000000000000),
 ( 0.3333333333333333703, 0.3333333333333333703, 0.3333333333333333703, 0.3333333333333333703, 0.3333333333333333703, 0.3333333333333333703, 0.3333333333333333703, 0.3333333333333333703, 0.3333333333333333703, 0.3333333333333333703, 0.3333333333333333703, 0.3333333333333333703, 0.3333333333333333703, 0.3333333333333333703, 0.3333333333333333703, 0.3333333333333333703, 0.3333333333333333703, 0.3333333333333333703, 0.3333333333333333703, 0.3333333333333333703, 0.3333333333333333703, 0.3333333333333333703, 0.3333333333333333703, 0.3333333333333333703, 0.3333333333333333703, 0.3333333333333333703, 0.3333333333333333703, 0.3333333333333333703, 0.3333333333333333703, 0.3333333333333333703),
 ( 0.3333333333333333703, 0.3333333333333333703, 0.3333333333333333703, 0.3333333333333333703, 0.3333333333333333703, 0.3333333333333333703, 0.3333333333333333703, 0.3333333333333333703, 0.3333333333333333703, 0.3333333333333333703, 0.3333333333333333703, 0.3333333333333333703, 0.3333333333333333703, 0.3333333333333333703, 0.3333333333333333703, 0.3333333333333333703, 0.3333333333333333703, 0.3333333333333333703, 0.3333333333333333703, 0.3333333333333333703, 0.3333333333333333703, 0.3333333333333333703, 0.3333333333333333703, 0.3333333333333333703, 0.3333333333333333703, 0.3333333333333333703, 0.3333333333333333703, 0.3333333333333333703, 0.3333333333333333703, 0.3333333333333333703),
 ( 1.000000000000000000, 1.000000000000000000, 1.000000000000000000, 1.000000000000000000, 1.000000000000000000, 1.000000000000000000, 1.000000000000000000, 1.000000000000000000, 1.000000000000000000, 1.000000000000000000, 1.000000000000000000, 1.000000000000000000, 1.000000000000000000, 1.000000000000000000, 1.000000000000000000, 1.000000000000000000, 1.000000000000000000, 1.000000000000000000, 1.000000000000000000, 1.000000000000000000, 1.000000000000000000, 1.000000000000000000, 1.000000000000000000, 1.000000000000000000, 1.000000000000000000, 1.000000000000000000, 1.000000000000000000, 1.000000000000000000, 1.000000000000000000, 1.000000000000000000) ) ) 
 REPRESENTATION_ITEM ( '' )  SURFACE ( )  );
#6731=CARTESIAN_POINT ( 'NONE',  ( 6.615221834162048786, -49.23097633541600260, 14.16446777330088658 ) ) ;
#6732=CARTESIAN_POINT ( 'NONE',  ( 0.2972598230769930017, 14.33493731733933352, 40.00000000000002132 ) ) ;
#6735=CARTESIAN_POINT ( 'NONE',  ( -86.96347745069644475, -15.38646221621786125, -15.38646221621789856 ) ) ;
#6736=CARTESIAN_POINT ( 'NONE',  ( -47.45115950054488252, -14.84795788660673388, 29.80449331795290746 ) ) ;
#6737=CARTESIAN_POINT ( 'NONE',  ( -30.26275506840324070, 1.198031551616013601, 1.198031551616023371 ) ) ;
#6738=CARTESIAN_POINT ( 'NONE',  ( -2.164901439688427409, 13.92557459412259391, -47.64638340556017226 ) ) ;
#6740=CARTESIAN_POINT ( 'NONE',  ( 146.6084372240433709, 3.800685668858042821, 52.76785682606522698 ) ) ;
#6743=CARTESIAN_POINT ( 'NONE',  ( -188.3066136396993784, -13.82848859481211967, 46.99300418776426369 ) ) ;
#6744=CIRCLE ( 'NONE', #9286, 30.00000000000003908 ) ;
#6745=CARTESIAN_POINT ( 'NONE',  ( -162.0762913951020892, -1.198031840385767266, -1.198031840385758384 ) ) ;
#6746=B_SPLINE_CURVE_WITH_KNOTS ( 'NONE', 3,
 ( #2431, #14653, #23185, #8680, #16790, #8407 ),
 .UNSPECIFIED., .F., .F.,
 ( 4, 2, 4 ),
 ( 0.3689590070116580689, 0.3867117631979620773, 0.4044645193949217843 ),
 .UNSPECIFIED. ) ;
#6747=CARTESIAN_POINT ( 'NONE',  ( 151.7948205124835681, 51.78348778862537927, 4.785054706298732086 ) ) ;
#6748=CARTESIAN_POINT ( 'NONE',  ( 170.2234770963711128, -45.64576402573167258, -10.92277846919254891 ) ) ;
#6749=CARTESIAN_POINT ( 'NONE',  ( 163.1118516004056573, 19.27778845538753316, 19.27778845538783870 ) ) ;
#6750=CARTESIAN_POINT ( 'NONE',  ( -238.4067589809705794, -0.6820004457913585449, -0.6820004457913265705 ) ) ;
#6751=CARTESIAN_POINT ( 'NONE',  ( -56.48582580120559271, 21.81201906317798489, -21.81201906317746619 ) ) ;
#6752=CARTESIAN_POINT ( 'NONE',  ( 192.4448373802100889, -14.14213562375896061, 14.14213562375865330 ) ) ;
#6753=CARTESIAN_POINT ( 'NONE',  ( 14.38125909742181285, -15.17850393972633505, 40.00000000000002132 ) ) ;
#6754=CARTESIAN_POINT ( 'NONE',  ( -100.7734535825088500, -22.67402823373193499, -40.00000000000002132 ) ) ;
#6755=CARTESIAN_POINT ( 'NONE',  ( 19.06497207195980792, 10.03556273973433299, 10.03556273973436319 ) ) ;
#6757=CARTESIAN_POINT ( 'NONE',  ( -162.0762913951020892, -1.198031840315659124, -57.76657433523998009 ) ) ;
#6758=CARTESIAN_POINT ( 'NONE',  ( -166.3490444790731431, 36.43931842064077387, -19.13701437385414295 ) ) ;
#6760=CARTESIAN_POINT ( 'NONE',  ( -105.3755690713226585, -15.38646221621796251, 41.18208027870593924 ) ) ;
#6762=CARTESIAN_POINT ( 'NONE',  ( -198.0356074513804288, -39.15871834505936278, 39.15871834505892224 ) ) ;
#6763=CARTESIAN_POINT ( 'NONE',  ( 11.71430589700012526, -49.28686712665649594, -14.17293196763931462 ) ) ;
#6765=CARTESIAN_POINT ( 'NONE',  ( -102.4068193528139972, -20.44188272012875984, 8.088405365068716435 ) ) ;
#6766=CARTESIAN_POINT ( 'NONE',  ( -82.24286367748180737, -12.41697925881799947, -15.97558298110162411 ) ) ;
#6770=CARTESIAN_POINT ( 'NONE',  ( 199.9999999999999432, 19.99999999999996092, 2.449293598294708485E-15 ) ) ;
#6773=CARTESIAN_POINT ( 'NONE',  ( 14.38125909742183062, -67.30136555895943218, -10.73282306403629605 ) ) ;
#6774=CARTESIAN_POINT ( 'NONE',  ( 151.7948205124836534, -40.00000000000001421, 6.767089262348889633 ) ) ;
#6775=CARTESIAN_POINT ( 'NONE',  ( -238.4067589809705794, -4.716212492215116094E-14, 0.9644942799825824142 ) ) ;
#6776=CARTESIAN_POINT ( 'NONE',  ( -196.0240701931631691, -24.63338802862617172, -44.60678453686448108 ) ) ;
#6777=CARTESIAN_POINT ( 'NONE',  ( 14.38125909742182884, -55.17850393972636169, -2.449293598294708485E-15 ) ) ;
#6778=CARTESIAN_POINT ( 'NONE',  ( 23.05038679986266459, -17.85133178553819988, -43.09692730307060060 ) ) ;
#6779=CARTESIAN_POINT ( 'NONE',  ( -30.26275506840324070, -1.198031551616032919, 1.198031551616014712 ) ) ;
#6780=CARTESIAN_POINT ( 'NONE',  ( -30.26275506840322649, -41.69427246844630019, -2.449293598294708485E-15 ) ) ;
#6781=CARTESIAN_POINT ( 'NONE',  ( -198.0356074513804572, -10.87444709760996986, 67.44298959253333692 ) ) ;
#6782=CARTESIAN_POINT ( 'NONE',  ( -105.3755690713226727, -2.472783935621397949E-13, 21.75974354311649961 ) ) ;
#6783=CARTESIAN_POINT ( 'NONE',  ( -105.3394646353463600, 10.54672847198930796, -18.62482576791553868 ) ) ;
#6784=CARTESIAN_POINT ( 'NONE',  ( 136.1360204305621551, 39.99999999999968026, 35.03383547441337953 ) ) ;
#6787=CARTESIAN_POINT ( 'NONE',  ( -102.4068193528165693, -8.735227608996721571, -20.17396017424868759 ) ) ;
#6788=CARTESIAN_POINT ( 'NONE',  ( 14.38125909742183062, -67.30136555898262429, 10.73282306405838682 ) ) ;
#6789=EDGE_LOOP ( 'NONE', ( #922, #13297, #29, #8963, #21305, #5042, #3190 ) ) ;
#6790=CARTESIAN_POINT ( 'NONE',  ( 91.82158438592158234, 12.16597498397756993, 12.16597498397776356 ) ) ;
#6791=CARTESIAN_POINT ( 'NONE',  ( -189.4799804244524637, 23.69387126430460455, -43.33513910317138595 ) ) ;
#6793=CARTESIAN_POINT ( 'NONE',  ( 91.82158438592159655, -22.79471317813468545, -40.00000000000002132 ) ) ;
#6795=CARTESIAN_POINT ( 'NONE',  ( -126.6834154283321112, -24.04426794716115623, 11.16464792285850471 ) ) ;
#6796=CARTESIAN_POINT ( 'NONE',  ( 170.2234770963711128, -17.36149277827010096, 17.36149277826970660 ) ) ;
#6798=ORIENTED_EDGE ( 'NONE', *, *, #11501, .T. ) ;
#6800=CARTESIAN_POINT ( 'NONE',  ( -103.9663809734325497, 8.574562933842363677, -19.92521373320581546 ) ) ;
#6801=EDGE_LOOP ( 'NONE', ( #22734, #13558, #23865, #16077, #3711, #10171, #25272, #15979, #10431, #7557 ) ) ;
#6802=VERTEX_POINT ( 'NONE', #26077 ) ;
#6803=CARTESIAN_POINT ( 'NONE',  ( 19.06497207195980792, -18.24870850772763475, 38.31983398719622613 ) ) ;
#6806=CARTESIAN_POINT ( 'NONE',  ( 184.8905102610680444, -14.79361573936379415, -14.79361573936387941 ) ) ;
#6807=CARTESIAN_POINT ( 'NONE',  ( -30.26275506840324070, 1.198031551616013601, 1.198031551616023371 ) ) ;
#6808=CARTESIAN_POINT ( 'NONE',  ( -280.0000000000000000, 1.839446121267387017E-14, -20.00000000000001421 ) ) ;
#6810=CARTESIAN_POINT ( 'NONE',  ( -88.38011429793466789, -8.298859913938862576, -20.03522015793668842 ) ) ;
#6812=CARTESIAN_POINT ( 'NONE',  ( 57.59792236341148453, -40.00000000000003553, 2.435789363417741438 ) ) ;
#6813=CARTESIAN_POINT ( 'NONE',  ( -86.96347745069645896, 39.99999999999977973, 21.75974354311691883 ) ) ;
#6814=CARTESIAN_POINT ( 'NONE',  ( -82.28544635048413625, 18.14459473659407962, 8.922251332909290511 ) ) ;
#6817=CARTESIAN_POINT ( 'NONE',  ( -188.2956751479415232, 13.82790121914897341, 46.98904240251096809 ) ) ;
#6818=CARTESIAN_POINT ( 'NONE',  ( -213.1075012329537230, -9.698598906450422774, -9.698598906450550672 ) ) ;
#6819=CARTESIAN_POINT ( 'NONE',  ( 98.29820294270297154, 18.47759065022021474, -7.653668647299666006 ) ) ;
#6820=CARTESIAN_POINT ( 'NONE',  ( -135.8532207217289738, 34.75652343174594705, 21.81201906317792449 ) ) ;
#6821=CARTESIAN_POINT ( 'NONE',  ( -86.90968602926041342, -19.36074508460288257, 9.002619558043598147 ) ) ;
#6822=CARTESIAN_POINT ( 'NONE',  ( -192.9588430854689705, -38.51493924976909966, -38.51493924976973915 ) ) ;
#6824=CARTESIAN_POINT ( 'NONE',  ( 4.995406935893294431, -15.24977328854832415, 40.00000000000002132 ) ) ;
#6825=CARTESIAN_POINT ( 'NONE',  ( -135.8532207217289738, 50.09629031063956006, 6.472252184284782217 ) ) ;
#6826=CARTESIAN_POINT ( 'NONE',  ( 91.82158438592156813, 17.20528682183302038, 40.00000000000002132 ) ) ;
#6829=CARTESIAN_POINT ( 'NONE',  ( -280.0000000000000568, -40.00000000000028422, 19.99999999999959499 ) ) ;
#6833=ORIENTED_EDGE ( 'NONE', *, *, #3799, .F. ) ;
#6835=CARTESIAN_POINT ( 'NONE',  ( -56.48582580120559982, 30.84685318188643421, 40.00000000000002132 ) ) ;
#6837=( BOUNDED_SURFACE ( )  B_SPLINE_SURFACE ( 3, 3, ( 
 ( #272, #14626, #24498, #2403, #22632, #8380, #24627, #10653, #25029, #6782, #4809, #4407, #16633, #6384, #14501, #12640, #20629, #18628, #411, #13541, #25161, #21541, #21162, #23159, #17406, #5063, #3315, #15284, #23535, #3441 ),
 ( #23660, #15029, #9426, #9302, #21667, #11413, #17285, #7417, #19535, #4938, #1320, #6912, #13044, #19663, #3064, #19156, #11045, #15532, #23415, #2935, #17533, #21290, #13169, #15410, #5191, #11295, #7296, #11166, #25671, #7045 ),
 ( #11539, #25547, #5306, #19282, #940, #17154, #1065, #13418, #1450, #5440, #17025, #9172, #9049, #25288, #15162, #23287, #13293, #25419, #7168, #21414, #3187, #19413, #1197, #17659, #14075, #15923, #25800, #18189, #3842, #16201 ),
 ( #24334, #22339, #24056, #7548, #5567, #12078, #5832, #7807, #12212, #26340, #17791, #20200, #17925, #26069, #9822, #23917, #13935, #9550, #22070, #9685, #11946, #1712, #20071, #1847, #4115, #9950, #8082, #15790, #15660, #16064 ),
 ( #5692, #22206, #18059, #24191, #20334, #5964, #26210, #7946, #1979, #10085, #25936, #3981, #7678, #6098, #14205, #23786, #13673, #21795, #3567, #13797, #11671, #19795, #1582, #21932, #11809, #3707, #19929, #10220, #24732, #8350 ),
 ( #10618, #20468, #24462, #6488, #16731, #18732, #22603, #22730, #12609, #108, #16471, #18599, #20597, #515, #8620, #6227, #24862, #2243, #14470, #8215, #6617, #12745, #16333, #14340, #14734, #20865, #16599, #4508, #10350, #24596 ),
 ( #2111, #22866, #22471, #4250, #14600, #6351, #4643, #2373, #20738, #2649, #2507, #377, #18327, #12340, #18460, #8482, #238, #4379, #12470, #10485, #23873, #15743, #3659, #18013, #7764, #26297, #11766, #12035, #14295, #1804 ) ),
 .UNSPECIFIED., .T., .F., .F. ) 
 B_SPLINE_SURFACE_WITH_KNOTS ( ( 4, 3, 4 ),
 ( 4, 2, 2, 2, 2, 2, 2, 2, 2, 2, 2, 2, 2, 2, 4 ),
 ( 0.000000000000000000, 0.5000000000000000000, 1.000000000000000000 ),
 ( 0.000000000000000000, 0.1357259735107005372, 0.1651108541090157700, 0.1944957347073310028, 0.3598804999793158710, 0.3867117631979620773, 0.4135430264166082281, 0.5789277916885930964, 0.6062785021374117456, 0.6336292125862302838, 0.8508620842112317728, 0.8814014469398914198, 0.9119408096685510667, 0.9559704048342755334, 1.000000000000000000 ),
 .UNSPECIFIED. ) 
 GEOMETRIC_REPRESENTATION_ITEM ( )  RATIONAL_B_SPLINE_SURFACE ( (
 ( 1.000000000000000000, 1.000000000000000000, 1.000000000000000000, 1.000000000000000000, 1.000000000000000000, 1.000000000000000000, 1.000000000000000000, 1.000000000000000000, 1.000000000000000000, 1.000000000000000000, 1.000000000000000000, 1.000000000000000000, 1.000000000000000000, 1.000000000000000000, 1.000000000000000000, 1.000000000000000000, 1.000000000000000000, 1.000000000000000000, 1.000000000000000000, 1.000000000000000000, 1.000000000000000000, 1.000000000000000000, 1.000000000000000000, 1.000000000000000000, 1.000000000000000000, 1.000000000000000000, 1.000000000000000000, 1.000000000000000000, 1.000000000000000000, 1.000000000000000000),
 ( 0.3333333333333333703, 0.3333333333333333703, 0.3333333333333333703, 0.3333333333333333703, 0.3333333333333333703, 0.3333333333333333703, 0.3333333333333333703, 0.3333333333333333703, 0.3333333333333333703, 0.3333333333333333703, 0.3333333333333333703, 0.3333333333333333703, 0.3333333333333333703, 0.3333333333333333703, 0.3333333333333333703, 0.3333333333333333703, 0.3333333333333333703, 0.3333333333333333703, 0.3333333333333333703, 0.3333333333333333703, 0.3333333333333333703, 0.3333333333333333703, 0.3333333333333333703, 0.3333333333333333703, 0.3333333333333333703, 0.3333333333333333703, 0.3333333333333333703, 0.3333333333333333703, 0.3333333333333333703, 0.3333333333333333703),
 ( 0.3333333333333333703, 0.3333333333333333703, 0.3333333333333333703, 0.3333333333333333703, 0.3333333333333333703, 0.3333333333333333703, 0.3333333333333333703, 0.3333333333333333703, 0.3333333333333333703, 0.3333333333333333703, 0.3333333333333333703, 0.3333333333333333703, 0.3333333333333333703, 0.3333333333333333703, 0.3333333333333333703, 0.3333333333333333703, 0.3333333333333333703, 0.3333333333333333703, 0.3333333333333333703, 0.3333333333333333703, 0.3333333333333333703, 0.3333333333333333703, 0.3333333333333333703, 0.3333333333333333703, 0.3333333333333333703, 0.3333333333333333703, 0.3333333333333333703, 0.3333333333333333703, 0.3333333333333333703, 0.3333333333333333703),
 ( 1.000000000000000000, 1.000000000000000000, 1.000000000000000000, 1.000000000000000000, 1.000000000000000000, 1.000000000000000000, 1.000000000000000000, 1.000000000000000000, 1.000000000000000000, 1.000000000000000000, 1.000000000000000000, 1.000000000000000000, 1.000000000000000000, 1.000000000000000000, 1.000000000000000000, 1.000000000000000000, 1.000000000000000000, 1.000000000000000000, 1.000000000000000000, 1.000000000000000000, 1.000000000000000000, 1.000000000000000000, 1.000000000000000000, 1.000000000000000000, 1.000000000000000000, 1.000000000000000000, 1.000000000000000000, 1.000000000000000000, 1.000000000000000000, 1.000000000000000000),
 ( 0.3333333333333333703, 0.3333333333333333703, 0.3333333333333333703, 0.3333333333333333703, 0.3333333333333333703, 0.3333333333333333703, 0.3333333333333333703, 0.3333333333333333703, 0.3333333333333333703, 0.3333333333333333703, 0.3333333333333333703, 0.3333333333333333703, 0.3333333333333333703, 0.3333333333333333703, 0.3333333333333333703, 0.3333333333333333703, 0.3333333333333333703, 0.3333333333333333703, 0.3333333333333333703, 0.3333333333333333703, 0.3333333333333333703, 0.3333333333333333703, 0.3333333333333333703, 0.3333333333333333703, 0.3333333333333333703, 0.3333333333333333703, 0.3333333333333333703, 0.3333333333333333703, 0.3333333333333333703, 0.3333333333333333703),
 ( 0.3333333333333333703, 0.3333333333333333703, 0.3333333333333333703, 0.3333333333333333703, 0.3333333333333333703, 0.3333333333333333703, 0.3333333333333333703, 0.3333333333333333703, 0.3333333333333333703, 0.3333333333333333703, 0.3333333333333333703, 0.3333333333333333703, 0.3333333333333333703, 0.3333333333333333703, 0.3333333333333333703, 0.3333333333333333703, 0.3333333333333333703, 0.3333333333333333703, 0.3333333333333333703, 0.3333333333333333703, 0.3333333333333333703, 0.3333333333333333703, 0.3333333333333333703, 0.3333333333333333703, 0.3333333333333333703, 0.3333333333333333703, 0.3333333333333333703, 0.3333333333333333703, 0.3333333333333333703, 0.3333333333333333703),
 ( 1.000000000000000000, 1.000000000000000000, 1.000000000000000000, 1.000000000000000000, 1.000000000000000000, 1.000000000000000000, 1.000000000000000000, 1.000000000000000000, 1.000000000000000000, 1.000000000000000000, 1.000000000000000000, 1.000000000000000000, 1.000000000000000000, 1.000000000000000000, 1.000000000000000000, 1.000000000000000000, 1.000000000000000000, 1.000000000000000000, 1.000000000000000000, 1.000000000000000000, 1.000000000000000000, 1.000000000000000000, 1.000000000000000000, 1.000000000000000000, 1.000000000000000000, 1.000000000000000000, 1.000000000000000000, 1.000000000000000000, 1.000000000000000000, 1.000000000000000000) ) ) 
 REPRESENTATION_ITEM ( '' )  SURFACE ( )  );
#6838=CARTESIAN_POINT ( 'NONE',  ( -110.0947178154516877, -20.04333087340630115, 2.529241932050243058 ) ) ;
#6839=CARTESIAN_POINT ( 'NONE',  ( -199.9999999999999716, 51.72223107510019702, 14.31382256974095490 ) ) ;
#6840=CARTESIAN_POINT ( 'NONE',  ( -105.3755690713226585, -39.99999999999996447, -21.75974354311664527 ) ) ;
#6845=CARTESIAN_POINT ( 'NONE',  ( -208.1127848780264742, -17.67593391476605547, -38.89260858015755673 ) ) ;
#6846=CARTESIAN_POINT ( 'NONE',  ( 170.2234770963711128, -10.92277846919235529, 45.64576402573175073 ) ) ;
#6849=CARTESIAN_POINT ( 'NONE',  ( -100.7734535825088500, -39.99999999999986500, -17.32597176626853397 ) ) ;
#6851=CARTESIAN_POINT ( 'NONE',  ( 0.2972598230769983307, -14.33493731733933352, 0.000000000000000000 ) ) ;
#6852=CARTESIAN_POINT ( 'NONE',  ( -238.4067589809705794, -28.96627169325343942, 28.96627169325309126 ) ) ;
#6855=CARTESIAN_POINT ( 'NONE',  ( -100.7734535825088358, 6.065416334915073333E-14, -22.67402823373191723 ) ) ;
#6856=CARTESIAN_POINT ( 'NONE',  ( -259.2033419157646676, -9.517827891722680178, 0.000000000000000000 ) ) ;
#6857=CARTESIAN_POINT ( 'NONE',  ( 146.6084372240433993, -24.48358557860319706, -24.48358557860330720 ) ) ;
#6858=CARTESIAN_POINT ( 'NONE',  ( -259.2033419157646676, 30.48217210827734647, 40.00000000000002132 ) ) ;
#6859=EDGE_LOOP ( 'NONE', ( #21551, #9429, #11241, #12552 ) ) ;
#6861=CARTESIAN_POINT ( 'NONE',  ( -2.557884977069448063, -43.43882039328137523, 23.77085849409481000 ) ) ;
#6863=CARTESIAN_POINT ( 'NONE',  ( -105.3755690713226585, -21.75974354311652448, -40.00000000000002132 ) ) ;
#6864=DIRECTION ( 'NONE',  ( 0.000000000000000000, -0.3656393565653622280, 0.9307566067079341421 ) ) ;
#6865=CARTESIAN_POINT ( 'NONE',  ( 19.06497207195981858, 10.03556273973424062, 66.60410523465820631 ) ) ;
#6866=CARTESIAN_POINT ( 'NONE',  ( -62.69292774211698571, -9.343531400666156728, 25.97703433363412628 ) ) ;
#6867=CARTESIAN_POINT ( 'NONE',  ( -77.60240544034114407, 21.88152835081340797, 3.050660596052795714 ) ) ;
#6868=EDGE_CURVE ( 'NONE', #9833, #25465, #15521, .T. ) ;
#6870=CARTESIAN_POINT ( 'NONE',  ( -7.726389047741937688, 17.45517700520669280, -42.14052505958233041 ) ) ;
#6872=CARTESIAN_POINT ( 'NONE',  ( 130.8568914410475372, -24.07718906447255947, 24.07718906447199458 ) ) ;
#6874=CARTESIAN_POINT ( 'NONE',  ( -188.3611024622287857, -13.83140737835751821, 47.01268868735293438 ) ) ;
#6875=CARTESIAN_POINT ( 'NONE',  ( 151.7948205124836534, 23.49921654116009506, 33.06932595376371609 ) ) ;
#6876=CARTESIAN_POINT ( 'NONE',  ( 200.0000000000000000, -14.14213562373046784, -42.42640687119298804 ) ) ;
#6878=CARTESIAN_POINT ( 'NONE',  ( -200.4318156386405008, 14.17468120671562737, -49.29858106685321673 ) ) ;
#6879=CARTESIAN_POINT ( 'NONE',  ( -208.1127848780264742, 67.17687982763172272, -10.60833733270698254 ) ) ;
#6880=CARTESIAN_POINT ( 'NONE',  ( -280.0000000000000568, -14.14213562373049449, -42.42640687119305198 ) ) ;
#6881=CARTESIAN_POINT ( 'NONE',  ( -100.7734535825088500, 22.67402823373189946, 40.00000000000002132 ) ) ;
#6882=CARTESIAN_POINT ( 'NONE',  ( 4.995406935893289102, 55.24977328856464709, -40.00000000000002132 ) ) ;
#6883=B_SPLINE_CURVE_WITH_KNOTS ( 'NONE', 3,
 ( #21090, #602, #10714, #12698, #19217, #741, #23094, #25091, #16824, #19090 ),
 .UNSPECIFIED., .F., .F.,
 ( 4, 2, 2, 2, 4 ),
 ( 0.7921542097164085972, 0.8508620842112317728, 0.8814014469398914198, 0.9119408096685510667, 0.9406682828394935525 ),
 .UNSPECIFIED. ) ;
#6884=CARTESIAN_POINT ( 'NONE',  ( -162.0762913951020892, 1.198031840385716418, 1.198031840385750169 ) ) ;
#6885=( BOUNDED_CURVE ( )  B_SPLINE_CURVE ( 3, ( #2465, #18964, #474, #8580 ),
 .UNSPECIFIED., .F., .F. ) 
 B_SPLINE_CURVE_WITH_KNOTS ( ( 4, 4 ),
 ( 0.01388163287021778290, 0.02359082919309994641 ),
 .UNSPECIFIED. ) 
 CURVE ( )  GEOMETRIC_REPRESENTATION_ITEM ( )  RATIONAL_B_SPLINE_CURVE ( ( 1.000000000000000000, 0.8672072324488997452, 0.7608653435686203448, 0.6809743333591616876 ) ) 
 REPRESENTATION_ITEM ( '' )  );
#6887=CARTESIAN_POINT ( 'NONE',  ( -135.8532207217289738, -21.81201906317806305, 34.75652343174590442 ) ) ;
#6888=CARTESIAN_POINT ( 'NONE',  ( -188.3120147333423233, 46.99495896211633550, -13.82877842034795002 ) ) ;
#6890=CARTESIAN_POINT ( 'NONE',  ( 163.1118516004056573, -19.27778845539233998, 37.29075403953149959 ) ) ;
#6892=CARTESIAN_POINT ( 'NONE',  ( -82.23726319241512783, -15.17211809665081290, -13.38817034152228480 ) ) ;
#6893=CARTESIAN_POINT ( 'NONE',  ( -105.3755690713226585, 15.38646221621762678, 41.18208027870604582 ) ) ;
#6894=CARTESIAN_POINT ( 'NONE',  ( -47.45115950031290453, -31.57405104348713110, -10.57586762648235634 ) ) ;
#6896=CARTESIAN_POINT ( 'NONE',  ( -151.4802849341727438, -31.86309571749480796, 16.17241510390670456 ) ) ;
#6897=CARTESIAN_POINT ( 'NONE',  ( -110.0961828203647741, -12.41698901629497520, -15.97557204180744961 ) ) ;
#6900=CARTESIAN_POINT ( 'NONE',  ( -135.8532207217289738, 30.84685318188643777, -40.00000000000002132 ) ) ;
#6903=CARTESIAN_POINT ( 'NONE',  ( -259.2033419157646676, 6.730120644403426944, 6.730120644403592145 ) ) ;
#6904=CARTESIAN_POINT ( 'NONE',  ( 192.4448373802100889, -3.692737725850373501E-14, 19.99999999996060751 ) ) ;
#6905=CARTESIAN_POINT ( 'NONE',  ( 130.8568914410475088, 40.00000000000002842, 5.949712681206834830 ) ) ;
#6906=CARTESIAN_POINT ( 'NONE',  ( -3.763361371728497051, 47.08953757622920477, -13.84281709279659189 ) ) ;
#6907=CARTESIAN_POINT ( 'NONE',  ( 91.82158438592156813, 17.20528682183302038, -40.00000000000002132 ) ) ;
#6908=CARTESIAN_POINT ( 'NONE',  ( 22.57783252600391322, -17.90541116499574414, -43.22748647439809133 ) ) ;
#6910=CARTESIAN_POINT ( 'NONE',  ( -105.3755690713226585, -18.24025645688355013, 40.00000000000002132 ) ) ;
#6911=CARTESIAN_POINT ( 'NONE',  ( 91.82158438592156813, 40.45024623143950038, 16.11829626348447420 ) ) ;
#6912=CARTESIAN_POINT ( 'NONE',  ( -91.56559293963836410, 39.99999999999976552, 22.67402823373234000 ) ) ;
#6913=CARTESIAN_POINT ( 'NONE',  ( -110.0574180502660653, 18.01801597164610413, -9.169691069488823842 ) ) ;
#6914=CARTESIAN_POINT ( 'NONE',  ( 14.38125909742182529, -39.99999999999944578, -55.17850393971050238 ) ) ;
#6915=CARTESIAN_POINT ( 'NONE',  ( 163.1118516004056573, -19.27778845538761132, -19.27778845538770724 ) ) ;
#6918=CARTESIAN_POINT ( 'NONE',  ( 163.1118516004056573, 19.27778845539212327, 37.29075403953164169 ) ) ;
#6920=CARTESIAN_POINT ( 'NONE',  ( -86.91014751117377557, 19.35827336066830995, -9.009177718430029458 ) ) ;
#6921=CARTESIAN_POINT ( 'NONE',  ( -5.866564133101147327, 42.46617576964662533, -23.09290806363647874 ) ) ;
#6923=CARTESIAN_POINT ( 'NONE',  ( 151.7948205124836534, -6.767089262349006873, 40.00000000000002132 ) ) ;
#6924=CARTESIAN_POINT ( 'NONE',  ( -114.5450021253294892, 9.945938879699479429, -19.55077795857054213 ) ) ;
#6925=CARTESIAN_POINT ( 'NONE',  ( -189.5227390968178725, 43.46195835885794168, -18.00253259953321461 ) ) ;
#6926=VERTEX_POINT ( 'NONE', #4124 ) ;
#6927=VERTEX_POINT ( 'NONE', #4517 ) ;
#6929=CARTESIAN_POINT ( 'NONE',  ( 98.29820294267857150, 5.170639833979637778, 19.50609486047177299 ) ) ;
#6930=ORIENTED_EDGE ( 'NONE', *, *, #15342, .F. ) ;
#6931=ORIENTED_EDGE ( 'NONE', *, *, #11657, .T. ) ;
#6932=CARTESIAN_POINT ( 'NONE',  ( -105.3755690713226585, -43.67073346367983788, 12.89780903124397149 ) ) ;
#6934=CARTESIAN_POINT ( 'NONE',  ( -110.0368417077423118, -7.441767002991612756, 18.74474319003509137 ) ) ;
#6935=CARTESIAN_POINT ( 'NONE',  ( 130.8568914410475372, -24.07718906447222551, -24.07718906447233209 ) ) ;
#6936=CARTESIAN_POINT ( 'NONE',  ( 136.1360204305621266, -24.77266263493116583, -24.77266263493127951 ) ) ;
#6937=CARTESIAN_POINT ( 'NONE',  ( -213.1075012329537230, 39.99999999999992895, 13.71589010951925935 ) ) ;
#6940=CARTESIAN_POINT ( 'NONE',  ( 200.0000000000000000, -40.00000000000019185, 19.99999999999968381 ) ) ;
#6941=CARTESIAN_POINT ( 'NONE',  ( 184.8905102610680444, 40.00000000000025580, -19.07866798485515503 ) ) ;
#6942=CARTESIAN_POINT ( 'NONE',  ( -82.24337801438862527, 15.81455109355221111, 12.55991608931321224 ) ) ;
#6945=CARTESIAN_POINT ( 'NONE',  ( -175.9235632132996443, 39.35891845671766731, -21.03681927240882743 ) ) ;
#6946=CARTESIAN_POINT ( 'NONE',  ( -238.4067589809705794, -0.6820004457913585449, -0.6820004457913265705 ) ) ;
#6948=PLANE ( 'NONE',  #10594 ) ;
#6949=CARTESIAN_POINT ( 'NONE',  ( -77.59802414163006290, 21.90520607601874659, 2.969683337867993878 ) ) ;
#6950=CARTESIAN_POINT ( 'NONE',  ( 19.06497207195981858, -10.03556273973377166, -66.60410523465827737 ) ) ;
#6952=CARTESIAN_POINT ( 'NONE',  ( -77.90255099906772784, 8.644468104261493480, 20.04994828523958361 ) ) ;
#6953=ADVANCED_FACE ( 'NONE', ( #6495 ), #22311, .T. ) ;
#6954=EDGE_LOOP ( 'NONE', ( #6267, #5844, #14388, #18509 ) ) ;
#6955=CARTESIAN_POINT ( 'NONE',  ( 0.2972598230769907257, 66.70487387989869887, -10.13633138497392494 ) ) ;
#6956=CARTESIAN_POINT ( 'NONE',  ( -30.26275506840324070, -1.694272468446265112, 0.000000000000000000 ) ) ;
#6958=EDGE_LOOP ( 'NONE', ( #20047, #1295, #8364, #21718 ) ) ;
#6959=CARTESIAN_POINT ( 'NONE',  ( 19.06497207195982924, -39.99999999999945288, -54.19242893257885640 ) ) ;
#6963=VERTEX_POINT ( 'NONE', #522 ) ;
#6966=CARTESIAN_POINT ( 'NONE',  ( 4.995406935893288214, 55.24977328854835434, 2.449293598294708485E-15 ) ) ;
#6972=CARTESIAN_POINT ( 'NONE',  ( -208.1127848780264742, -40.00000000000011369, 15.00245453012655439 ) ) ;
#6975=CARTESIAN_POINT ( 'NONE',  ( 146.6084372240433709, -24.48358557860284179, -32.08495691632087699 ) ) ;
#6976=CARTESIAN_POINT ( 'NONE',  ( 146.6084372240433993, 24.48358557860307272, 24.48358557860347418 ) ) ;
#6977=CARTESIAN_POINT ( 'NONE',  ( -88.37548150066159280, 20.03288105173027844, 8.297891025033743873 ) ) ;
#6978=CARTESIAN_POINT ( 'NONE',  ( 136.1360204305621266, 7.947488714877270288E-14, -4.966164525587064560 ) ) ;
#6979=CARTESIAN_POINT ( 'NONE',  ( -86.96347745069644475, 15.38646221621772092, 15.38646221621800336 ) ) ;
#6980=CARTESIAN_POINT ( 'NONE',  ( 57.59792236341147031, 2.435789363418171760, 0.000000000000000000 ) ) ;
#6981=CARTESIAN_POINT ( 'NONE',  ( 184.8905102610680444, -13.49065550809810965, 13.49065550809799596 ) ) ;
#6982=CARTESIAN_POINT ( 'NONE',  ( -135.8532207217289738, 9.153146818113546246, -0.000000000000000000 ) ) ;
#6984=CARTESIAN_POINT ( 'NONE',  ( 19.06497207195981147, -4.605042221739098431E-14, 14.19242893257840521 ) ) ;
#6985=CARTESIAN_POINT ( 'NONE',  ( -135.8532207217289738, -9.153146818113595984, 0.000000000000000000 ) ) ;
#6986=CARTESIAN_POINT ( 'NONE',  ( -208.1127848780264742, 10.60833733270764867, 67.17687982763166588 ) ) ;
#6987=CARTESIAN_POINT ( 'NONE',  ( 136.1360204305621551, -35.03383547441293899, 40.00000000000002132 ) ) ;
#6988=EDGE_LOOP ( 'NONE', ( #4306, #1368, #2701, #10269 ) ) ;
#6989=CARTESIAN_POINT ( 'NONE',  ( 20.17262239844370697, -43.80323544018611415, 18.14389419513820201 ) ) ;
#6990=( BOUNDED_SURFACE ( )  B_SPLINE_SURFACE ( 3, 3, ( 
 ( #6429, #2058, #20005, #24272, #6044, #10164, #8287, #22545, #4325, #2314, #12416, #10422, #14547, #12546, #8964, #10829, #20678, #13090, #25074, #11087, #24807, #19203, #590, #9090, #14943, #2585, #16676, #21074, #18810, #25334 ),
 ( #12683, #15072, #12825, #20946, #4719, #8697, #2724, #4451, #18944, #4586, #725, #22939, #16808, #23078, #24946, #6559, #6693, #12955, #17197, #14807, #14674, #4983, #2447, #22810, #21207, #4850, #985, #10699, #7091, #10558 ),
 ( #20813, #17073, #8829, #16939, #15205, #18671, #457, #8561, #6825, #2859, #10966, #23203, #19073, #855, #25207, #6955, #2979, #5108, #15577, #1238, #17328, #5609, #17702, #5229, #11583, #13581, #5354, #7463, #23701, #5481 ),
 ( #11719, #19450, #1624, #21708, #21455, #9217, #3486, #11334, #17833, #25590, #19703, #3230, #13213, #19838, #19578, #17574, #1491, #9597, #9343, #7336, #25846, #1369, #23577, #7590, #11454, #15328, #9467, #15702, #19325, #17451 ),
 ( #23826, #21335, #25462, #13715, #21840, #9731, #15450, #3609, #3106, #25980, #7721, #23333, #11210, #13461, #1109, #7213, #23455, #13333, #21581, #3353, #25711, #21975, #12122, #12381, #282, #18103, #26253, #20379, #20112, #11989 ),
 ( #24508, #10263, #24097, #19973, #16245, #6268, #152, #16107, #14245, #12256, #3747, #1889, #10129, #22247, #8256, #18373, #4292, #5872, #24238, #26112, #11853, #16374, #2281, #13841, #1754, #20509, #18501, #8128, #22385, #13979 ),
 ( #22112, #6011, #9994, #14120, #15972, #6137, #10390, #24374, #3889, #14382, #2153, #9863, #4022, #17965, #22514, #7851, #20247, #2027, #7988, #15831, #23961, #18231, #5736, #17, #4161, #22641, #14510, #20775, #2690, #14773 ) ),
 .UNSPECIFIED., .T., .F., .F. ) 
 B_SPLINE_SURFACE_WITH_KNOTS ( ( 4, 3, 4 ),
 ( 4, 2, 2, 2, 2, 2, 2, 2, 2, 2, 2, 2, 2, 2, 4 ),
 ( 0.000000000000000000, 0.5000000000000000000, 1.000000000000000000 ),
 ( 0.000000000000000000, 0.1357259735107005372, 0.1651108541090157700, 0.1944957347073310028, 0.3598804999793158710, 0.3867117631979620773, 0.4135430264166082281, 0.5789277916885930964, 0.6062785021374117456, 0.6336292125862302838, 0.8508620842112317728, 0.8814014469398914198, 0.9119408096685510667, 0.9559704048342755334, 1.000000000000000000 ),
 .UNSPECIFIED. ) 
 GEOMETRIC_REPRESENTATION_ITEM ( )  RATIONAL_B_SPLINE_SURFACE ( (
 ( 1.000000000000000000, 1.000000000000000000, 1.000000000000000000, 1.000000000000000000, 1.000000000000000000, 1.000000000000000000, 1.000000000000000000, 1.000000000000000000, 1.000000000000000000, 1.000000000000000000, 1.000000000000000000, 1.000000000000000000, 1.000000000000000000, 1.000000000000000000, 1.000000000000000000, 1.000000000000000000, 1.000000000000000000, 1.000000000000000000, 1.000000000000000000, 1.000000000000000000, 1.000000000000000000, 1.000000000000000000, 1.000000000000000000, 1.000000000000000000, 1.000000000000000000, 1.000000000000000000, 1.000000000000000000, 1.000000000000000000, 1.000000000000000000, 1.000000000000000000),
 ( 0.3333333333333333703, 0.3333333333333333703, 0.3333333333333333703, 0.3333333333333333703, 0.3333333333333333703, 0.3333333333333333703, 0.3333333333333333703, 0.3333333333333333703, 0.3333333333333333703, 0.3333333333333333703, 0.3333333333333333703, 0.3333333333333333703, 0.3333333333333333703, 0.3333333333333333703, 0.3333333333333333703, 0.3333333333333333703, 0.3333333333333333703, 0.3333333333333333703, 0.3333333333333333703, 0.3333333333333333703, 0.3333333333333333703, 0.3333333333333333703, 0.3333333333333333703, 0.3333333333333333703, 0.3333333333333333703, 0.3333333333333333703, 0.3333333333333333703, 0.3333333333333333703, 0.3333333333333333703, 0.3333333333333333703),
 ( 0.3333333333333333703, 0.3333333333333333703, 0.3333333333333333703, 0.3333333333333333703, 0.3333333333333333703, 0.3333333333333333703, 0.3333333333333333703, 0.3333333333333333703, 0.3333333333333333703, 0.3333333333333333703, 0.3333333333333333703, 0.3333333333333333703, 0.3333333333333333703, 0.3333333333333333703, 0.3333333333333333703, 0.3333333333333333703, 0.3333333333333333703, 0.3333333333333333703, 0.3333333333333333703, 0.3333333333333333703, 0.3333333333333333703, 0.3333333333333333703, 0.3333333333333333703, 0.3333333333333333703, 0.3333333333333333703, 0.3333333333333333703, 0.3333333333333333703, 0.3333333333333333703, 0.3333333333333333703, 0.3333333333333333703),
 ( 1.000000000000000000, 1.000000000000000000, 1.000000000000000000, 1.000000000000000000, 1.000000000000000000, 1.000000000000000000, 1.000000000000000000, 1.000000000000000000, 1.000000000000000000, 1.000000000000000000, 1.000000000000000000, 1.000000000000000000, 1.000000000000000000, 1.000000000000000000, 1.000000000000000000, 1.000000000000000000, 1.000000000000000000, 1.000000000000000000, 1.000000000000000000, 1.000000000000000000, 1.000000000000000000, 1.000000000000000000, 1.000000000000000000, 1.000000000000000000, 1.000000000000000000, 1.000000000000000000, 1.000000000000000000, 1.000000000000000000, 1.000000000000000000, 1.000000000000000000),
 ( 0.3333333333333333703, 0.3333333333333333703, 0.3333333333333333703, 0.3333333333333333703, 0.3333333333333333703, 0.3333333333333333703, 0.3333333333333333703, 0.3333333333333333703, 0.3333333333333333703, 0.3333333333333333703, 0.3333333333333333703, 0.3333333333333333703, 0.3333333333333333703, 0.3333333333333333703, 0.3333333333333333703, 0.3333333333333333703, 0.3333333333333333703, 0.3333333333333333703, 0.3333333333333333703, 0.3333333333333333703, 0.3333333333333333703, 0.3333333333333333703, 0.3333333333333333703, 0.3333333333333333703, 0.3333333333333333703, 0.3333333333333333703, 0.3333333333333333703, 0.3333333333333333703, 0.3333333333333333703, 0.3333333333333333703),
 ( 0.3333333333333333703, 0.3333333333333333703, 0.3333333333333333703, 0.3333333333333333703, 0.3333333333333333703, 0.3333333333333333703, 0.3333333333333333703, 0.3333333333333333703, 0.3333333333333333703, 0.3333333333333333703, 0.3333333333333333703, 0.3333333333333333703, 0.3333333333333333703, 0.3333333333333333703, 0.3333333333333333703, 0.3333333333333333703, 0.3333333333333333703, 0.3333333333333333703, 0.3333333333333333703, 0.3333333333333333703, 0.3333333333333333703, 0.3333333333333333703, 0.3333333333333333703, 0.3333333333333333703, 0.3333333333333333703, 0.3333333333333333703, 0.3333333333333333703, 0.3333333333333333703, 0.3333333333333333703, 0.3333333333333333703),
 ( 1.000000000000000000, 1.000000000000000000, 1.000000000000000000, 1.000000000000000000, 1.000000000000000000, 1.000000000000000000, 1.000000000000000000, 1.000000000000000000, 1.000000000000000000, 1.000000000000000000, 1.000000000000000000, 1.000000000000000000, 1.000000000000000000, 1.000000000000000000, 1.000000000000000000, 1.000000000000000000, 1.000000000000000000, 1.000000000000000000, 1.000000000000000000, 1.000000000000000000, 1.000000000000000000, 1.000000000000000000, 1.000000000000000000, 1.000000000000000000, 1.000000000000000000, 1.000000000000000000, 1.000000000000000000, 1.000000000000000000, 1.000000000000000000, 1.000000000000000000) ) ) 
 REPRESENTATION_ITEM ( '' )  SURFACE ( )  );
#6991=CARTESIAN_POINT ( 'NONE',  ( -280.0000000000000568, 19.99999999999996447, -40.00000000000002132 ) ) ;
#6993=CARTESIAN_POINT ( 'NONE',  ( 136.1360204305621266, 3.511608612530704665, 3.511608612530695339 ) ) ;
#6995=CARTESIAN_POINT ( 'NONE',  ( -1.258540240222670414, -13.96099832920753769, -47.88180740053038420 ) ) ;
#6997=CARTESIAN_POINT ( 'NONE',  ( 57.59792236341147031, 26.56190807104652052, 30.00663442387728708 ) ) ;
#6998=CARTESIAN_POINT ( 'NONE',  ( -77.90255099906852365, -20.29001641120231625, 8.064892378667423145 ) ) ;
#6999=CARTESIAN_POINT ( 'NONE',  ( -86.86493150571115507, 7.943527260496353826, 19.77569912839162569 ) ) ;
#7000=CARTESIAN_POINT ( 'NONE',  ( -200.4318156386405576, -14.17468120671533960, 49.29858106685333752 ) ) ;
#7001=CARTESIAN_POINT ( 'NONE',  ( 91.82158438592158234, -1.633484621919921769E-13, 17.20528682183300262 ) ) ;
#7003=CARTESIAN_POINT ( 'NONE',  ( -192.9588430854690273, 18.05360324515418924, 38.51493924976949756 ) ) ;
#7004=CARTESIAN_POINT ( 'NONE',  ( -77.70150415247218234, 11.19846400430064648, -18.99169997608993299 ) ) ;
#7005=CARTESIAN_POINT ( 'NONE',  ( 14.38125909742181285, -10.73282306404712472, -10.73282306404731301 ) ) ;
#7006=CARTESIAN_POINT ( 'NONE',  ( -198.0356074513804572, -10.87444709759714634, -10.87444709759729911 ) ) ;
#7007=CARTESIAN_POINT ( 'NONE',  ( 192.4448373802101173, 42.42640687116487896, 14.14213562375934075 ) ) ;
#7008=CARTESIAN_POINT ( 'NONE',  ( 57.59792236341147031, 54.84617931850878136, 1.722363176415705910 ) ) ;
#7009=CARTESIAN_POINT ( 'NONE',  ( 14.38125909742180752, 55.17850393971008316, -40.00000000000002132 ) ) ;
#7010=CARTESIAN_POINT ( 'NONE',  ( 0.2972598230769886718, 38.42060263243669027, -18.14793986248710667 ) ) ;
#7012=CARTESIAN_POINT ( 'NONE',  ( 146.6084372240433709, -32.08495691632075619, 24.48358557860298035 ) ) ;
#7013=EDGE_CURVE ( 'NONE', #7472, #22554, #7287, .T. ) ;
#7014=CARTESIAN_POINT ( 'NONE',  ( -183.1090696432183904, 41.47043467738880196, -22.43564075023506277 ) ) ;
#7015=ORIENTED_EDGE ( 'NONE', *, *, #24602, .T. ) ;
#7016=CARTESIAN_POINT ( 'NONE',  ( -91.56559293963834989, 12.25131212657480440, 12.25131212657486834 ) ) ;
#7018=CARTESIAN_POINT ( 'NONE',  ( -198.0356074513804572, 17.40982414986446969, 39.15871834505921356 ) ) ;
#7019=CARTESIAN_POINT ( 'NONE',  ( -6.754359963570706782, -42.40682816666050314, -17.56548336385882791 ) ) ;
#7021=CARTESIAN_POINT ( 'NONE',  ( -188.3508614409240067, -43.15762572182580215, 17.87647389380253315 ) ) ;
#7022=B_SPLINE_CURVE_WITH_KNOTS ( 'NONE', 3,
 ( #23920, #7300, #3712, #11813, #19933, #24060 ),
 .UNSPECIFIED., .F., .F.,
 ( 4, 2, 4 ),
 ( -5.998621905159389411E-08, 0.03937827992696039947, 0.07875661984013984651 ),
 .UNSPECIFIED. ) ;
#7025=CARTESIAN_POINT ( 'NONE',  ( 36.88256715608616076, -16.19941669834411968, 39.10885149554682272 ) ) ;
#7026=CARTESIAN_POINT ( 'NONE',  ( -135.8532207217289738, -9.153146818113595984, -40.00000000000002132 ) ) ;
#7027=CARTESIAN_POINT ( 'NONE',  ( 45.01779936573458230, 18.90344565805356325, -36.09695843560584194 ) ) ;
#7031=B_SPLINE_CURVE_WITH_KNOTS ( 'NONE', 3,
 ( #23281, #21408, #13534, #15404, #3560, #25282, #13287, #3181, #25539, #11287, #7290, #23529, #21659, #3431 ),
 .UNSPECIFIED., .F., .F.,
 ( 4, 2, 2, 2, 2, 2, 4 ),
 ( 6.938893903907228378E-18, 0.002941681445496982863, 0.004412522168245476030, 0.005883362890993969196, 0.008825044336490964203, 0.01029588505923946344, 0.01176672578198796094 ),
 .UNSPECIFIED. ) ;
#7032=B_SPLINE_CURVE_WITH_KNOTS ( 'NONE', 3,
 ( #9818, #22067, #21792, #22203, #11668, #11942, #3978, #7943 ),
 .UNSPECIFIED., .F., .F.,
 ( 4, 2, 2, 4 ),
 ( -5.298247996756991549E-05, 0.001923793760059295263, 0.003900570000086160151, 0.007854122480139891227 ),
 .UNSPECIFIED. ) ;
#7033=CARTESIAN_POINT ( 'NONE',  ( 0.2972598230770027716, -38.42060263243681817, 18.14793986248684377 ) ) ;
#7034=CARTESIAN_POINT ( 'NONE',  ( -30.26275506840324425, 39.99999999999987210, 41.69427246844643520 ) ) ;
#7035=CARTESIAN_POINT ( 'NONE',  ( -56.48582580120559271, 2.158176344243877536E-14, -9.153146818113587102 ) ) ;
#7036=EDGE_CURVE ( 'NONE', #6050, #4035, #20315, .T. ) ;
#7037=( BOUNDED_SURFACE ( )  B_SPLINE_SURFACE ( 3, 3, ( 
 ( #3958, #1959, #10065, #26319, #24313, #2091, #8061, #6079, #18301, #16313, #355, #24437, #6205, #4229, #12318, #2223, #8325, #5013, #10733, #11120, #16846, #622, #13118, #21239, #6728, #757, #19105, #24709, #889, #23237 ),
 ( #1014, #3014, #15102, #18708, #4882, #6591, #12987, #14579, #12586, #14976, #20715, #2756, #23110, #20844, #2619, #19234, #18844, #20975, #8728, #14713, #25109, #24979, #6987, #16578, #12857, #4751, #14840, #22973, #10859, #18978 ),
 ( #8861, #6858, #16973, #4484, #21109, #4620, #6464, #22708, #2888, #2481, #10593, #10996, #22845, #491, #8998, #24840, #8598, #16708, #12716, #17102, #25235, #19741, #21873, #7122, #9501, #3138, #3261, #13364, #15608, #7243 ),
 ( #21614, #15482, #15232, #25878, #13493, #19358, #11240, #3519, #17607, #7497, #5641, #11365, #17228, #19483, #11619, #7622, #1148, #15737, #9252, #3388, #17358, #9635, #25494, #15364, #23363, #5513, #1530, #23864, #1269, #17737 ),
 ( #11486, #23488, #25368, #13747, #25749, #19877, #3651, #5388, #5262, #5140, #23609, #21487, #9373, #13246, #21370, #17482, #25624, #11758, #9117, #7371, #23732, #19614, #1400, #13616, #21744, #26150, #14021, #26290, #16013, #24409 ),
 ( #6049, #11891, #3788, #22422, #10169, #59, #24548, #22150, #9768, #12028, #4198, #185, #20011, #18005, #16148, #14420, #20419, #7757, #7894, #26019, #18142, #15868, #24139, #13884, #8168, #16419, #8292, #12291, #5777, #17869 ),
 ( #24280, #2063, #20148, #20284, #14154, #5913, #6302, #22019, #3930, #1927, #22550, #23996, #2196, #10305, #1796, #9900, #10033, #4331, #18410, #8029, #22286, #4060, #12162, #18272, #16281, #14286, #6175, #12421, #1659, #4990 ) ),
 .UNSPECIFIED., .T., .F., .F. ) 
 B_SPLINE_SURFACE_WITH_KNOTS ( ( 4, 3, 4 ),
 ( 4, 2, 2, 2, 2, 2, 2, 2, 2, 2, 2, 2, 2, 2, 4 ),
 ( 0.000000000000000000, 0.5000000000000000000, 1.000000000000000000 ),
 ( 0.000000000000000000, 0.1357259735107005372, 0.1651108541090157700, 0.1944957347073310028, 0.3598804999793158710, 0.3867117631979620773, 0.4135430264166082281, 0.5789277916885930964, 0.6062785021374117456, 0.6336292125862302838, 0.8508620842112317728, 0.8814014469398914198, 0.9119408096685510667, 0.9559704048342755334, 1.000000000000000000 ),
 .UNSPECIFIED. ) 
 GEOMETRIC_REPRESENTATION_ITEM ( )  RATIONAL_B_SPLINE_SURFACE ( (
 ( 1.000000000000000000, 1.000000000000000000, 1.000000000000000000, 1.000000000000000000, 1.000000000000000000, 1.000000000000000000, 1.000000000000000000, 1.000000000000000000, 1.000000000000000000, 1.000000000000000000, 1.000000000000000000, 1.000000000000000000, 1.000000000000000000, 1.000000000000000000, 1.000000000000000000, 1.000000000000000000, 1.000000000000000000, 1.000000000000000000, 1.000000000000000000, 1.000000000000000000, 1.000000000000000000, 1.000000000000000000, 1.000000000000000000, 1.000000000000000000, 1.000000000000000000, 1.000000000000000000, 1.000000000000000000, 1.000000000000000000, 1.000000000000000000, 1.000000000000000000),
 ( 0.3333333333333333703, 0.3333333333333333703, 0.3333333333333333703, 0.3333333333333333703, 0.3333333333333333703, 0.3333333333333333703, 0.3333333333333333703, 0.3333333333333333703, 0.3333333333333333703, 0.3333333333333333703, 0.3333333333333333703, 0.3333333333333333703, 0.3333333333333333703, 0.3333333333333333703, 0.3333333333333333703, 0.3333333333333333703, 0.3333333333333333703, 0.3333333333333333703, 0.3333333333333333703, 0.3333333333333333703, 0.3333333333333333703, 0.3333333333333333703, 0.3333333333333333703, 0.3333333333333333703, 0.3333333333333333703, 0.3333333333333333703, 0.3333333333333333703, 0.3333333333333333703, 0.3333333333333333703, 0.3333333333333333703),
 ( 0.3333333333333333703, 0.3333333333333333703, 0.3333333333333333703, 0.3333333333333333703, 0.3333333333333333703, 0.3333333333333333703, 0.3333333333333333703, 0.3333333333333333703, 0.3333333333333333703, 0.3333333333333333703, 0.3333333333333333703, 0.3333333333333333703, 0.3333333333333333703, 0.3333333333333333703, 0.3333333333333333703, 0.3333333333333333703, 0.3333333333333333703, 0.3333333333333333703, 0.3333333333333333703, 0.3333333333333333703, 0.3333333333333333703, 0.3333333333333333703, 0.3333333333333333703, 0.3333333333333333703, 0.3333333333333333703, 0.3333333333333333703, 0.3333333333333333703, 0.3333333333333333703, 0.3333333333333333703, 0.3333333333333333703),
 ( 1.000000000000000000, 1.000000000000000000, 1.000000000000000000, 1.000000000000000000, 1.000000000000000000, 1.000000000000000000, 1.000000000000000000, 1.000000000000000000, 1.000000000000000000, 1.000000000000000000, 1.000000000000000000, 1.000000000000000000, 1.000000000000000000, 1.000000000000000000, 1.000000000000000000, 1.000000000000000000, 1.000000000000000000, 1.000000000000000000, 1.000000000000000000, 1.000000000000000000, 1.000000000000000000, 1.000000000000000000, 1.000000000000000000, 1.000000000000000000, 1.000000000000000000, 1.000000000000000000, 1.000000000000000000, 1.000000000000000000, 1.000000000000000000, 1.000000000000000000),
 ( 0.3333333333333333703, 0.3333333333333333703, 0.3333333333333333703, 0.3333333333333333703, 0.3333333333333333703, 0.3333333333333333703, 0.3333333333333333703, 0.3333333333333333703, 0.3333333333333333703, 0.3333333333333333703, 0.3333333333333333703, 0.3333333333333333703, 0.3333333333333333703, 0.3333333333333333703, 0.3333333333333333703, 0.3333333333333333703, 0.3333333333333333703, 0.3333333333333333703, 0.3333333333333333703, 0.3333333333333333703, 0.3333333333333333703, 0.3333333333333333703, 0.3333333333333333703, 0.3333333333333333703, 0.3333333333333333703, 0.3333333333333333703, 0.3333333333333333703, 0.3333333333333333703, 0.3333333333333333703, 0.3333333333333333703),
 ( 0.3333333333333333703, 0.3333333333333333703, 0.3333333333333333703, 0.3333333333333333703, 0.3333333333333333703, 0.3333333333333333703, 0.3333333333333333703, 0.3333333333333333703, 0.3333333333333333703, 0.3333333333333333703, 0.3333333333333333703, 0.3333333333333333703, 0.3333333333333333703, 0.3333333333333333703, 0.3333333333333333703, 0.3333333333333333703, 0.3333333333333333703, 0.3333333333333333703, 0.3333333333333333703, 0.3333333333333333703, 0.3333333333333333703, 0.3333333333333333703, 0.3333333333333333703, 0.3333333333333333703, 0.3333333333333333703, 0.3333333333333333703, 0.3333333333333333703, 0.3333333333333333703, 0.3333333333333333703, 0.3333333333333333703),
 ( 1.000000000000000000, 1.000000000000000000, 1.000000000000000000, 1.000000000000000000, 1.000000000000000000, 1.000000000000000000, 1.000000000000000000, 1.000000000000000000, 1.000000000000000000, 1.000000000000000000, 1.000000000000000000, 1.000000000000000000, 1.000000000000000000, 1.000000000000000000, 1.000000000000000000, 1.000000000000000000, 1.000000000000000000, 1.000000000000000000, 1.000000000000000000, 1.000000000000000000, 1.000000000000000000, 1.000000000000000000, 1.000000000000000000, 1.000000000000000000, 1.000000000000000000, 1.000000000000000000, 1.000000000000000000, 1.000000000000000000, 1.000000000000000000, 1.000000000000000000) ) ) 
 REPRESENTATION_ITEM ( '' )  SURFACE ( )  );
#7038=CARTESIAN_POINT ( 'NONE',  ( 22.40986519363265117, 47.15972762675190211, -13.85314893102512990 ) ) ;
#7039=CARTESIAN_POINT ( 'NONE',  ( -135.8532207217289454, -30.84685318188648750, -40.00000000000002132 ) ) ;
#7040=CARTESIAN_POINT ( 'NONE',  ( 22.72189371636289934, -23.48424859981544088, -43.05215026464033201 ) ) ;
#7042=CARTESIAN_POINT ( 'NONE',  ( 91.82158438592159655, -22.79471317813468900, 40.00000000000002132 ) ) ;
#7043=AXIS2_PLACEMENT_3D ( 'NONE', #10046, #7632, #21622 ) ;
#7044=CARTESIAN_POINT ( 'NONE',  ( -259.2033419157646676, 6.730120644403521979, -6.730120644403498886 ) ) ;
#7045=CARTESIAN_POINT ( 'NONE',  ( 200.0000000000000000, 39.99999999999985079, 20.00000000000052225 ) ) ;
#7046=CARTESIAN_POINT ( 'NONE',  ( -114.6659165474109727, 11.80608088193438476, -18.60032035377434312 ) ) ;
#7047=CARTESIAN_POINT ( 'NONE',  ( -259.2033419157646676, -39.99999999999975131, -30.48217210827782608 ) ) ;
#7049=CARTESIAN_POINT ( 'NONE',  ( 154.0335631730542332, -28.18627069283355979, -11.67513559369096754 ) ) ;
#7051=CARTESIAN_POINT ( 'NONE',  ( 151.7948205124836250, -4.785054706301671068, 4.785054706301645311 ) ) ;
#7052=EDGE_CURVE ( 'NONE', #5232, #13725, #15854, .T. ) ;
#7053=ADVANCED_FACE ( 'NONE', ( #19011 ), #25046, .T. ) ;
#7055=CARTESIAN_POINT ( 'NONE',  ( -77.84460141634583863, -7.435777209860166437, -20.59121244913221815 ) ) ;
#7056=CARTESIAN_POINT ( 'NONE',  ( 6.615221834200135653, 44.82734842560610389, -24.79576599683312566 ) ) ;
#7057=CARTESIAN_POINT ( 'NONE',  ( 57.59792236341147031, 2.435789363418170872, 40.00000000000002132 ) ) ;
#7059=CARTESIAN_POINT ( 'NONE',  ( -188.9524464570941689, 47.22058047019630322, -13.86227157644267649 ) ) ;
#7061=ORIENTED_EDGE ( 'NONE', *, *, #20049, .F. ) ;
#7062=ORIENTED_EDGE ( 'NONE', *, *, #14093, .F. ) ;
#7063=CIRCLE ( 'NONE', #17647, 14.99999999999999645 ) ;
#7064=CARTESIAN_POINT ( 'NONE',  ( -103.9474983244998469, -19.92928099173819589, 8.577167319634416032 ) ) ;
#7065=CARTESIAN_POINT ( 'NONE',  ( 85.88436334094248537, -22.72801779304886338, -10.32541289898071035 ) ) ;
#7069=DIRECTION ( 'NONE',  ( 0.9352143328346382845, 0.3271292286583122322, -0.1355013631594907397 ) ) ;
#7071=CARTESIAN_POINT ( 'NONE',  ( 14.38125909742181463, 10.73282306405862485, 67.30136555898259587 ) ) ;
#7073=CARTESIAN_POINT ( 'NONE',  ( -198.0356074513804572, 39.99999999999979394, 55.37879056874835726 ) ) ;
#7074=CARTESIAN_POINT ( 'NONE',  ( -199.9999999999999432, -44.86667451853065813, 23.83166235904703356 ) ) ;
#7075=CARTESIAN_POINT ( 'NONE',  ( 98.29820294267490510, 4.808046699556526995E-12, 20.00000000000513722 ) ) ;
#7076=CARTESIAN_POINT ( 'NONE',  ( -56.48582580120558561, -40.00000000000012790, 9.153146818113166105 ) ) ;
#7077=CARTESIAN_POINT ( 'NONE',  ( 14.38125909742181818, 5.830552384690105017E-13, -55.17850393972636880 ) ) ;
#7078=CARTESIAN_POINT ( 'NONE',  ( -199.9999999999998010, 49.28189405767604114, -14.17215463606931181 ) ) ;
#7079=CIRCLE ( 'NONE', #15544, 15.00000000000000178 ) ;
#7080=CARTESIAN_POINT ( 'NONE',  ( -238.4067589809705794, -28.96627169325313389, -27.60227080167074831 ) ) ;
#7081=CARTESIAN_POINT ( 'NONE',  ( -56.48582580120559271, 2.158176344243877536E-14, -9.153146818113587102 ) ) ;
#7084=CARTESIAN_POINT ( 'NONE',  ( -190.6721449140024163, -47.76494005424141420, 13.94344083317857574 ) ) ;
#7085=CARTESIAN_POINT ( 'NONE',  ( 163.1118516004056573, 19.27778845538780317, -19.27778845538757224 ) ) ;
#7086=CARTESIAN_POINT ( 'NONE',  ( -87.12812962369609693, -14.21201470106591991, 16.13326835690859440 ) ) ;
#7087=CARTESIAN_POINT ( 'NONE',  ( -213.1075012329537230, -37.98287015391257881, 18.58567234101111509 ) ) ;
#7090=VERTEX_POINT ( 'NONE', #21269 ) ;
#7091=CARTESIAN_POINT ( 'NONE',  ( 192.4448373802101173, 14.14213562370261279, 42.42640687122091236 ) ) ;
#7096=CARTESIAN_POINT ( 'NONE',  ( 163.1118516004056573, 1.658263919738574066E-13, -12.73709011382475254 ) ) ;
#7098=CARTESIAN_POINT ( 'NONE',  ( -199.9999999999998863, -10.02640517461913738, -53.44529986889384077 ) ) ;
#7099=B_SPLINE_CURVE_WITH_KNOTS ( 'NONE', 3,
 ( #21313, #25955, #3205, #13191, #11432, #5208 ),
 .UNSPECIFIED., .F., .F.,
 ( 4, 2, 4 ),
 ( -6.000000006192509110E-08, 0.03937727993095045675, 0.07875461986190096519 ),
 .UNSPECIFIED. ) ;
#7101=ORIENTED_EDGE ( 'NONE', *, *, #7370, .T. ) ;
#7102=CARTESIAN_POINT ( 'NONE',  ( -105.3755690713226727, 18.24025645688350750, 2.449293598294708485E-15 ) ) ;
#7103=CARTESIAN_POINT ( 'NONE',  ( -102.4294859496614265, -20.29697089065278703, -8.407280618127234817 ) ) ;
#7105=CARTESIAN_POINT ( 'NONE',  ( -77.78673448795234435, -9.959188558496027355, 19.58653132801459762 ) ) ;
#7106=CARTESIAN_POINT ( 'NONE',  ( -198.0356074513804572, -40.00000000000011369, 15.37879056873056527 ) ) ;
#7108=CARTESIAN_POINT ( 'NONE',  ( -82.28158588894086733, 9.172127817915399106, 18.01698387549497937 ) ) ;
#7109=CARTESIAN_POINT ( 'NONE',  ( -24.51100708723331323, -15.48921386291974400, -37.39427017791097541 ) ) ;
#7110=CARTESIAN_POINT ( 'NONE',  ( 146.6084372240433993, 24.48358557860307272, 24.48358557860347418 ) ) ;
#7112=CARTESIAN_POINT ( 'NONE',  ( 57.59792236341149163, -39.99999999999961631, -37.56421063658228832 ) ) ;
#7113=CARTESIAN_POINT ( 'NONE',  ( -56.48582580120559271, 6.472252184284121412, 6.472252184284244869 ) ) ;
#7114=CARTESIAN_POINT ( 'NONE',  ( -86.96347745069645896, 21.75974354311648895, -40.00000000000002132 ) ) ;
#7115=CARTESIAN_POINT ( 'NONE',  ( 0.2972598230770100991, -38.42060263243686791, 38.42060263243645579 ) ) ;
#7116=CARTESIAN_POINT ( 'NONE',  ( 19.06497207195980792, -14.19242893257839988, -40.00000000000002132 ) ) ;
#7119=CARTESIAN_POINT ( 'NONE',  ( -213.1075012329537230, 39.99999999999992895, 13.71589010951925935 ) ) ;
#7120=CARTESIAN_POINT ( 'NONE',  ( -30.26275506840324425, 1.694272468446254232, -40.00000000000002132 ) ) ;
#7121=CARTESIAN_POINT ( 'NONE',  ( 136.1360204305621551, -53.05693388239313890, 3.511608612530593199 ) ) ;
#7122=CARTESIAN_POINT ( 'NONE',  ( 146.6084372240433709, 5.374981219216996564, 40.00000000000002132 ) ) ;
#7123=ORIENTED_EDGE ( 'NONE', *, *, #21362, .F. ) ;
#7124=CARTESIAN_POINT ( 'NONE',  ( -3.993758944537062483, -43.01863922058820577, 23.45926997169917172 ) ) ;
#7125=CARTESIAN_POINT ( 'NONE',  ( 91.82158438592158234, 22.79471317813472098, 2.449293598294708485E-15 ) ) ;
#7126=CARTESIAN_POINT ( 'NONE',  ( 23.37394308801977871, 23.33966569535068203, 42.85717664514594816 ) ) ;
#7127=CARTESIAN_POINT ( 'NONE',  ( -280.0000000000000568, -14.14213562373108601, 42.42640687119285303 ) ) ;
#7128=FACE_OUTER_BOUND ( 'NONE', #19944, .T. ) ;
#7129=CARTESIAN_POINT ( 'NONE',  ( -77.84359416767949824, 20.59644767746334892, -7.424842266730552254 ) ) ;
#7130=CARTESIAN_POINT ( 'NONE',  ( -3.903133374378768838, -13.83543723415285598, -47.03983734341025524 ) ) ;
#7133=CARTESIAN_POINT ( 'NONE',  ( -77.70150415251713127, 5.510650003026252186, -21.34766967565243689 ) ) ;
#7134=CARTESIAN_POINT ( 'NONE',  ( 163.1118516004056573, -19.27778845538787422, 19.27778845538743724 ) ) ;
#7135=CARTESIAN_POINT ( 'NONE',  ( -105.3755690713226727, 15.38646221621771737, 15.38646221621800514 ) ) ;
#7136=CARTESIAN_POINT ( 'NONE',  ( -30.26275506840325136, 27.08623969584573388, 29.48230279907808793 ) ) ;
#7137=CARTESIAN_POINT ( 'NONE',  ( 163.1118516004056573, -19.27778845538787422, 19.27778845538743724 ) ) ;
#7138=CARTESIAN_POINT ( 'NONE',  ( 170.2234770963711128, 17.36149277826980253, 17.36149277827007253 ) ) ;
#7139=CARTESIAN_POINT ( 'NONE',  ( -192.9588430854689989, -10.23066800230742501, -10.23066800230756712 ) ) ;
#7140=CARTESIAN_POINT ( 'NONE',  ( -162.0762913951020892, 1.198031840456041497, -57.76657433537918251 ) ) ;
#7141=CARTESIAN_POINT ( 'NONE',  ( 151.7948205124836534, 33.06932595376333239, 23.49921654116065284 ) ) ;
#7142=CARTESIAN_POINT ( 'NONE',  ( -208.1127848780265026, 15.00245453012665564, 0.000000000000000000 ) ) ;
#7143=CARTESIAN_POINT ( 'NONE',  ( 163.1118516004056573, 9.006482792074356425, -47.56205970284957374 ) ) ;
#7144=CARTESIAN_POINT ( 'NONE',  ( -105.3755690713226727, 5.661656051307470077E-14, -21.75974354311649961 ) ) ;
#7145=CARTESIAN_POINT ( 'NONE',  ( -280.0000000000000568, -14.14213562373137556, 42.42640687119276066 ) ) ;
#7146=CARTESIAN_POINT ( 'NONE',  ( -173.7925187070230493, 38.69492115310539049, -20.60915802527609486 ) ) ;
#7148=CARTESIAN_POINT ( 'NONE',  ( -135.8532207217289738, -6.472252184284287502, 50.09629031063965243 ) ) ;
#7149=CARTESIAN_POINT ( 'NONE',  ( -192.1131137119205050, 24.17676406461165683, 43.98782916596407944 ) ) ;
#7150=CARTESIAN_POINT ( 'NONE',  ( 22.90311673803691406, 23.44499648834731431, 42.99920082299472313 ) ) ;
#7151=CARTESIAN_POINT ( 'NONE',  ( -4.151555265633191105, -42.97219445042051689, -23.42746911247791886 ) ) ;
#7153=CARTESIAN_POINT ( 'NONE',  ( -83.21262154144253032, -13.72187187061453706, -33.12752917118435647 ) ) ;
#7155=CARTESIAN_POINT ( 'NONE',  ( 23.30336656375605742, -13.80490921643078117, 46.83484695576456147 ) ) ;
#7157=CARTESIAN_POINT ( 'NONE',  ( 37.37129771749314244, 12.75330473306422618, -41.71823991406499488 ) ) ;
#7159=CARTESIAN_POINT ( 'NONE',  ( 127.8236149080042310, -28.75948073575762720, 11.91256696755838362 ) ) ;
#7160=CARTESIAN_POINT ( 'NONE',  ( -56.48582580120559271, 2.158176344243877536E-14, -9.153146818113587102 ) ) ;
#7161=DIRECTION ( 'NONE',  ( 0.2259624731721235902, 0.000000000000000000, -0.9741360072997697905 ) ) ;
#7163=CARTESIAN_POINT ( 'NONE',  ( 170.2234770963711128, 24.55285855007190676, -40.00000000000002132 ) ) ;
#7164=CARTESIAN_POINT ( 'NONE',  ( 37.15749683985377061, -20.52531616267859604, -38.58455518502878334 ) ) ;
#7166=CARTESIAN_POINT ( 'NONE',  ( -238.4067589809705794, -0.9644942799826262680, 0.000000000000000000 ) ) ;
#7167=CARTESIAN_POINT ( 'NONE',  ( -86.96347745069644475, 15.38646221621793586, -15.38646221621778842 ) ) ;
#7168=CARTESIAN_POINT ( 'NONE',  ( 19.06497207195980792, 40.00000000000059686, -54.19242893257802507 ) ) ;
#7169=CARTESIAN_POINT ( 'NONE',  ( -86.96347745069643054, -40.00000000000026290, 21.75974354311608749 ) ) ;
#7170=CARTESIAN_POINT ( 'NONE',  ( 151.0849710023778414, -29.07003783291312971, -12.04120392909159776 ) ) ;
#7172=VERTEX_POINT ( 'NONE', #11150 ) ;
#7173=CARTESIAN_POINT ( 'NONE',  ( -77.55625318716882077, 0.6712688186143358493, -22.13218714683804933 ) ) ;
#7174=CARTESIAN_POINT ( 'NONE',  ( -2.557884977170212792, 47.52441970259129533, -13.90734923103464560 ) ) ;
#7175=CARTESIAN_POINT ( 'NONE',  ( -192.9588430854690273, -14.46834944099973264, 40.00000000000002132 ) ) ;
#7177=CARTESIAN_POINT ( 'NONE',  ( -114.5520593196434618, 6.810303045868788097, -20.89066532546352306 ) ) ;
#7181=CARTESIAN_POINT ( 'NONE',  ( 57.59792236341147031, 1.722363176415065089, -1.722363176415036445 ) ) ;
#7182=CARTESIAN_POINT ( 'NONE',  ( 156.5537079553355113, 11.28159757857233814, -27.23618587942430480 ) ) ;
#7184=CARTESIAN_POINT ( 'NONE',  ( -196.0240759113457045, 44.60678620512916837, -24.63338926175146071 ) ) ;
#7188=CARTESIAN_POINT ( 'NONE',  ( -193.0908541284701982, 14.03723495791108000, 48.38978395451673720 ) ) ;
#7190=CARTESIAN_POINT ( 'NONE',  ( -280.0000000000000568, 42.42640687119285303, -14.14213562373088351 ) ) ;
#7191=CARTESIAN_POINT ( 'NONE',  ( -105.3174555396234240, -5.405828096113452830, -20.76745762185852939 ) ) ;
#7192=CARTESIAN_POINT ( 'NONE',  ( -56.48582580120559271, 2.158176344243877536E-14, -9.153146818113587102 ) ) ;
#7193=CARTESIAN_POINT ( 'NONE',  ( -190.1935349183499682, -23.83022391594521139, 43.51927535257657098 ) ) ;
#7195=EDGE_CURVE ( 'NONE', #11726, #7299, #13015, .T. ) ;
#7197=CARTESIAN_POINT ( 'NONE',  ( -259.2033419157646676, -39.99999999999975131, -30.48217210827782608 ) ) ;
#7198=CARTESIAN_POINT ( 'NONE',  ( 136.1360204305621551, 40.00000000000009948, -4.966164525586641787 ) ) ;
#7199=CARTESIAN_POINT ( 'NONE',  ( -110.0737093975828316, -17.41451009903333613, 10.28294049095705986 ) ) ;
#7200=CARTESIAN_POINT ( 'NONE',  ( 57.59792236341147031, -26.56190807104670171, -30.00663442387710234 ) ) ;
#7201=CARTESIAN_POINT ( 'NONE',  ( 200.0000000000000000, 40.00000000000012790, -19.99999999999996092 ) ) ;
#7202=CARTESIAN_POINT ( 'NONE',  ( 4.995406935893293543, -10.78321810389005364, 10.78321810388994173 ) ) ;
#7203=CARTESIAN_POINT ( 'NONE',  ( -86.86493150571121191, -19.77569912839188149, -7.943527260495856446 ) ) ;
#7205=CARTESIAN_POINT ( 'NONE',  ( -77.56334768864763873, 14.65129183226247278, -16.59360462361560451 ) ) ;
#7206=CARTESIAN_POINT ( 'NONE',  ( 163.1118516004056573, 47.56205970284957374, 9.006482792074494981 ) ) ;
#7207=CARTESIAN_POINT ( 'NONE',  ( -77.55461540593363168, 22.14110896975470411, -1.281724172690315244 ) ) ;
#7208=CARTESIAN_POINT ( 'NONE',  ( -91.56559293963834989, 12.25131212657480440, 12.25131212657486834 ) ) ;
#7209=CARTESIAN_POINT ( 'NONE',  ( 130.8568914410475088, -32.49135343045495006, 24.07718906446878648 ) ) ;
#7210=CARTESIAN_POINT ( 'NONE',  ( -187.3037411062501576, -23.25513534570995944, -42.71163782368778783 ) ) ;
#7213=CARTESIAN_POINT ( 'NONE',  ( 0.2972598230770011618, 10.13633138497555919, -66.70487387989845729 ) ) ;
#7216=ORIENTED_EDGE ( 'NONE', *, *, #12400, .F. ) ;
#7217=CARTESIAN_POINT ( 'NONE',  ( -100.7734535825088358, -2.560096224687585342E-13, 22.67402823373191723 ) ) ;
#7219=CARTESIAN_POINT ( 'NONE',  ( -1.821043593238315328, -43.61003463695182347, 23.89737153267518721 ) ) ;
#7223=CARTESIAN_POINT ( 'NONE',  ( -238.4067589809705794, -0.6820004457913680929, 0.6820004457913170226 ) ) ;
#7224=CARTESIAN_POINT ( 'NONE',  ( 146.6084372240433993, 5.715592784339989804E-15, 5.374981219216972583 ) ) ;
#7225=CARTESIAN_POINT ( 'NONE',  ( -99.31267923331543557, -20.62886818715002235, -8.544756979596986213 ) ) ;
#7227=CARTESIAN_POINT ( 'NONE',  ( 170.0000000000000000, 3.122849337825751958E-14, 0.000000000000000000 ) ) ;
#7228=CARTESIAN_POINT ( 'NONE',  ( 19.06497207195981147, -4.605042221739098431E-14, 14.19242893257840521 ) ) ;
#7230=CARTESIAN_POINT ( 'NONE',  ( -87.13361725334107177, 14.23662800447680610, 16.15936842096636283 ) ) ;
#7231=CARTESIAN_POINT ( 'NONE',  ( 14.38125909742180752, 10.73282306404735387, -10.73282306404708919 ) ) ;
#7232=CARTESIAN_POINT ( 'NONE',  ( 14.38125909742181996, -10.73282306405815234, -67.30136555898266693 ) ) ;
#7234=CARTESIAN_POINT ( 'NONE',  ( 0.2972598230770030492, 5.716321584140269555E-13, -54.33493731733936016 ) ) ;
#7235=CARTESIAN_POINT ( 'NONE',  ( -105.3220005116013880, -20.73876282934127246, -5.373930277613494511 ) ) ;
#7236=CARTESIAN_POINT ( 'NONE',  ( -91.56559293963836410, 22.67402823373190301, -40.00000000000002132 ) ) ;
#7237=CARTESIAN_POINT ( 'NONE',  ( -238.4067589809705794, 27.60227080167040370, 28.96627169325338613 ) ) ;
#7238=CARTESIAN_POINT ( 'NONE',  ( 91.82158438592156813, 17.20528682183302038, -40.00000000000002132 ) ) ;
#7239=CARTESIAN_POINT ( 'NONE',  ( 12.01361959687203296, -44.88892880200806701, -24.84115733209536714 ) ) ;
#7240=CARTESIAN_POINT ( 'NONE',  ( 184.8905102610680444, 1.070102760522089011E-13, -20.92133201514444352 ) ) ;
#7241=CARTESIAN_POINT ( 'NONE',  ( -162.0762913951020892, -1.202636532414034422E-14, -1.694272876828323948 ) ) ;
#7242=CARTESIAN_POINT ( 'NONE',  ( -208.1127848780265026, 38.89260858015724409, 38.89260858015741462 ) ) ;
#7243=CARTESIAN_POINT ( 'NONE',  ( 200.0000000000000000, 19.99999999999995737, 40.00000000000002132 ) ) ;
#7244=ORIENTED_EDGE ( 'NONE', *, *, #17579, .F. ) ;
#7245=CARTESIAN_POINT ( 'NONE',  ( 23.17367289775000216, -46.88342923877002022, 13.81211338457517535 ) ) ;
#7246=CARTESIAN_POINT ( 'NONE',  ( -87.08883615166492120, -12.58652615577264022, 17.39726528837622865 ) ) ;
#7247=CARTESIAN_POINT ( 'NONE',  ( 151.7948205124836534, -23.49921654116027980, 33.06932595376354556 ) ) ;
#7248=CARTESIAN_POINT ( 'NONE',  ( 91.82158438592158234, 7.693928927950222250E-14, -17.20528682183300262 ) ) ;
#7249=CARTESIAN_POINT ( 'NONE',  ( -82.28657550317936398, 19.11315898605473862, 6.589961070193250947 ) ) ;
#7252=CIRCLE ( 'NONE', #23010, 15.00000000000000178 ) ;
#7253=CARTESIAN_POINT ( 'NONE',  ( -7.297127544326129645, 22.81351773422571583, -42.04314499753679968 ) ) ;
#7257=CARTESIAN_POINT ( 'NONE',  ( -82.28266731795157796, -6.247331033611341233, -19.19528918669051265 ) ) ;
#7258=CARTESIAN_POINT ( 'NONE',  ( 151.7948205124836534, 4.785054706297857230, 51.78348778862544322 ) ) ;
#7259=CARTESIAN_POINT ( 'NONE',  ( -259.2033419157646676, -21.55415060305824326, -21.55415060305857367 ) ) ;
#7260=CARTESIAN_POINT ( 'NONE',  ( -100.7734535825088500, 44.31723036834890905, 12.25131212657507795 ) ) ;
#7262=CARTESIAN_POINT ( 'NONE',  ( -91.56559293963834989, -12.25131212657475466, -12.25131212657495361 ) ) ;
#7263=CARTESIAN_POINT ( 'NONE',  ( -238.4067589809705794, -28.96627169325303797, -28.96627169325349627 ) ) ;
#7264=CARTESIAN_POINT ( 'NONE',  ( 184.8905102610680444, -14.79361573936330565, -41.77492675556016621 ) ) ;
#7265=CARTESIAN_POINT ( 'NONE',  ( 130.8568914410475088, 32.49135343045448820, 24.07718906446946860 ) ) ;
#7266=CARTESIAN_POINT ( 'NONE',  ( -280.0000000000000568, -20.00000000000006750, -40.00000000000002132 ) ) ;
#7267=CARTESIAN_POINT ( 'NONE',  ( 200.0000000000000000, 3.673940397442060756E-14, 0.000000000000000000 ) ) ;
#7269=CARTESIAN_POINT ( 'NONE',  ( 146.6084372240433709, -3.800685668859084210, 52.76785682606516303 ) ) ;
#7271=CARTESIAN_POINT ( 'NONE',  ( -188.8948201289232998, 43.30398576617499629, -17.93709820916102871 ) ) ;
#7273=ADVANCED_FACE ( 'NONE', ( #5672 ), #1403, .T. ) ;
#7274=CARTESIAN_POINT ( 'NONE',  ( -213.1075012329537230, 37.98287015391236565, -18.58567234101138510 ) ) ;
#7275=CARTESIAN_POINT ( 'NONE',  ( -199.9999999999998579, 24.82633483071252201, 44.86878812508700776 ) ) ;
#7278=ORIENTED_EDGE ( 'NONE', *, *, #15894, .F. ) ;
#7279=CARTESIAN_POINT ( 'NONE',  ( -187.7698581930727073, -46.80706826624575712, 13.79076165501089335 ) ) ;
#7281=CARTESIAN_POINT ( 'NONE',  ( 83.11963132822124578, -10.90660717645929090, 23.63628489315943781 ) ) ;
#7283=CARTESIAN_POINT ( 'NONE',  ( 170.0000000000000853, -9.369682556672300322, 22.62041470344878746 ) ) ;
#7285=CIRCLE ( 'NONE', #21330, 14.99999999999999822 ) ;
#7286=CARTESIAN_POINT ( 'NONE',  ( -102.4068193528161999, -20.17396017424868404, -8.735227608996884996 ) ) ;
#7287=B_SPLINE_CURVE_WITH_KNOTS ( 'NONE', 3,
 ( #8893, #9279, #7149, #23394, #12889, #7275 ),
 .UNSPECIFIED., .F., .F.,
 ( 4, 2, 4 ),
 ( -5.998616618535840220E-08, 0.005994953700759713192, 0.01198996738768561172 ),
 .UNSPECIFIED. ) ;
#7288=CARTESIAN_POINT ( 'NONE',  ( 19.06497207195980792, 39.99999999999983658, 54.19242893257857929 ) ) ;
#7290=CARTESIAN_POINT ( 'NONE',  ( -199.9999999999999716, -15.65821854886078057, -47.96425349429453178 ) ) ;
#7291=CARTESIAN_POINT ( 'NONE',  ( 184.8905102610680444, -19.07866798485555293, -2.449293598294708485E-15 ) ) ;
#7292=CARTESIAN_POINT ( 'NONE',  ( -121.8281150760809339, 10.16552079391129304, -22.46071699682265788 ) ) ;
#7293=LINE ( 'NONE', #5188, #9592 ) ;
#7294=CARTESIAN_POINT ( 'NONE',  ( -86.96347745069645896, 21.75974354311648895, 40.00000000000002132 ) ) ;
#7295=CARTESIAN_POINT ( 'NONE',  ( -192.9588430854689989, -14.46834944099973086, 0.000000000000000000 ) ) ;
#7296=CARTESIAN_POINT ( 'NONE',  ( 170.2234770963711128, 39.99999999999980105, 24.55285855007229401 ) ) ;
#7297=CARTESIAN_POINT ( 'NONE',  ( 136.1360204305621551, -40.00000000000036238, 35.03383547441254109 ) ) ;
#7299=VERTEX_POINT ( 'NONE', #19879 ) ;
#7300=CARTESIAN_POINT ( 'NONE',  ( -16.41594856534389990, 39.35878123533669282, -21.03672846690459863 ) ) ;
#7301=CARTESIAN_POINT ( 'NONE',  ( -4.439300432586822609, 42.88738538954446256, -23.37136716947834003 ) ) ;
#7302=CARTESIAN_POINT ( 'NONE',  ( -105.3755690713226585, -18.24025645688355013, 40.00000000000002132 ) ) ;
#7303=CARTESIAN_POINT ( 'NONE',  ( -188.2995950289364941, -46.99046209955528042, 13.82811170417144453 ) ) ;
#7304=CARTESIAN_POINT ( 'NONE',  ( -192.6562840316691734, 44.11756026580140144, -18.27409180090461760 ) ) ;
#7309=CARTESIAN_POINT ( 'NONE',  ( 128.5824617753799828, 11.99766463964419749, -28.96492468983268509 ) ) ;
#7310=CARTESIAN_POINT ( 'NONE',  ( -97.72675010090323156, 8.185591577777252326, -20.89622088363367070 ) ) ;
#7311=VERTEX_POINT ( 'NONE', #24551 ) ;
#7314=CARTESIAN_POINT ( 'NONE',  ( 57.59792236341147031, 54.84617931850881689, -1.722363176414946073 ) ) ;
#7315=CARTESIAN_POINT ( 'NONE',  ( -114.4388184736423142, -20.16431396440720292, -8.352332320002245680 ) ) ;
#7316=CARTESIAN_POINT ( 'NONE',  ( -280.0000000000000000, 1.839446121267387017E-14, -20.00000000000001421 ) ) ;
#7318=DIRECTION ( 'NONE',  ( 1.000000000000000000, 1.836970198721030181E-16, -0.000000000000000000 ) ) ;
#7320=CARTESIAN_POINT ( 'NONE',  ( 163.1118516004056573, -39.99999999999986500, -12.73709011382517353 ) ) ;
#7321=CARTESIAN_POINT ( 'NONE',  ( -259.2033419157646676, 2.741182173978444749E-13, -30.48217210827739621 ) ) ;
#7322=CARTESIAN_POINT ( 'NONE',  ( -87.07288175661508944, 17.66871184921714644, 12.16928828659077766 ) ) ;
#7323=CARTESIAN_POINT ( 'NONE',  ( -91.56559293963836410, -12.25131212657462321, -44.31723036834905827 ) ) ;
#7324=CARTESIAN_POINT ( 'NONE',  ( -83.21262154144250189, -33.12752917118416462, -13.72187187061501668 ) ) ;
#7325=CARTESIAN_POINT ( 'NONE',  ( 57.59792236341147031, 1.722363176415065089, -1.722363176415036445 ) ) ;
#7326=CARTESIAN_POINT ( 'NONE',  ( 156.5537079553356534, 27.23618587942429770, 11.28159757857223688 ) ) ;
#7327=ADVANCED_FACE ( 'NONE', ( #12424 ), #21644, .T. ) ;
#7328=DIRECTION ( 'NONE',  ( -7.401486830834375884E-15, -0.3656393565658525024, -0.9307566067077415184 ) ) ;
#7330=CARTESIAN_POINT ( 'NONE',  ( -82.27051431267241810, -17.53273480388464023, 9.999544339283986005 ) ) ;
#7331=CARTESIAN_POINT ( 'NONE',  ( -86.96347745069644475, -15.38646221621796073, 41.18208027870593924 ) ) ;
#7332=CARTESIAN_POINT ( 'NONE',  ( 151.7948205124836534, -33.06932595376376582, 23.49921654115996006 ) ) ;
#7336=CARTESIAN_POINT ( 'NONE',  ( 57.59792236341147031, 26.56190807104720975, -26.56190807104655249 ) ) ;
#7337=EDGE_CURVE ( 'NONE', #15141, #18174, #14944, .T. ) ;
#7339=DIRECTION ( 'NONE',  ( 0.000000000000000000, 1.000000000000000000, 0.000000000000000000 ) ) ;
#7341=CARTESIAN_POINT ( 'NONE',  ( 163.1118516004056573, -2.556006622855449647E-13, 27.26290988616872824 ) ) ;
#7344=CARTESIAN_POINT ( 'NONE',  ( -77.90022806219164409, 8.352332316460230999, 20.16431395584620390 ) ) ;
#7345=ORIENTED_EDGE ( 'NONE', *, *, #18835, .T. ) ;
#7347=CARTESIAN_POINT ( 'NONE',  ( -199.0730705748055982, -44.83667434817697028, -18.57195860671723864 ) ) ;
#7348=CARTESIAN_POINT ( 'NONE',  ( -56.48582580120560692, 40.00000000000004263, -9.153146818113443217 ) ) ;
#7351=CARTESIAN_POINT ( 'NONE',  ( -208.1127848780264742, -40.00000000000025580, 55.00245453014408525 ) ) ;
#7354=CARTESIAN_POINT ( 'NONE',  ( -24.88648382749493848, -12.31763033312684286, -39.69105101983515027 ) ) ;
#7355=B_SPLINE_CURVE_WITH_KNOTS ( 'NONE', 3,
 ( #6454, #12440, #4348, #4474, #20436, #16838 ),
 .UNSPECIFIED., .F., .F.,
 ( 4, 2, 4 ),
 ( 1.631784767670790744E-15, 0.03937685683732423253, 0.07875371367464684136 ),
 .UNSPECIFIED. ) ;
#7356=CARTESIAN_POINT ( 'NONE',  ( -86.96347745069645896, 43.67073346367988762, -12.89780903124366418 ) ) ;
#7358=CARTESIAN_POINT ( 'NONE',  ( -86.86493150571118349, -19.60045294882770506, 8.366608963953762412 ) ) ;
#7359=CARTESIAN_POINT ( 'NONE',  ( 170.2234770963711128, 1.955190573858485757E-13, -15.44714144992816074 ) ) ;
#7361=CARTESIAN_POINT ( 'NONE',  ( 200.0000000000000000, -19.99999999999989342, 40.00000000000002132 ) ) ;
#7363=CARTESIAN_POINT ( 'NONE',  ( 184.8905102610680444, -19.07866798485553872, -40.00000000000002132 ) ) ;
#7364=CARTESIAN_POINT ( 'NONE',  ( -213.1075012329537230, -9.698598906450557777, 9.698598906450415669 ) ) ;
#7365=CARTESIAN_POINT ( 'NONE',  ( -135.8532207217289738, 9.153146818113548022, -40.00000000000002132 ) ) ;
#7367=DIRECTION ( 'NONE',  ( 0.9352143328345526863, 0.1355013631511626238, -0.3271292286620064993 ) ) ;
#7368=CARTESIAN_POINT ( 'NONE',  ( -30.26275506840324070, 1.218738420030236455E-14, -1.694272468446259783 ) ) ;
#7369=CARTESIAN_POINT ( 'NONE',  ( 14.38125909742181108, 39.01709431150907648, 39.01709431150921858 ) ) ;
#7370=EDGE_CURVE ( 'NONE', #2226, #10098, #13650, .T. ) ;
#7371=CARTESIAN_POINT ( 'NONE',  ( 57.59792236341147031, 37.56421063658187620, -40.00000000000002132 ) ) ;
#7373=CARTESIAN_POINT ( 'NONE',  ( 23.49666234703822809, -42.81942870555059244, 23.31470603676244480 ) ) ;
#7374=CARTESIAN_POINT ( 'NONE',  ( 132.4338126186516718, 12.33615677966314195, 29.78211700502430759 ) ) ;
#7375=CARTESIAN_POINT ( 'NONE',  ( -56.48582580120559271, 21.81201906317768291, 21.81201906317777173 ) ) ;
#7376=CARTESIAN_POINT ( 'NONE',  ( -30.26275506840324070, -1.147469862568086380E-14, 1.694272468446259783 ) ) ;
#7377=CARTESIAN_POINT ( 'NONE',  ( -77.70542728667135179, 21.32786667381274270, -5.408320660863019214 ) ) ;
#7378=CARTESIAN_POINT ( 'NONE',  ( 0.4289713102705769998, -14.02712011273541037, -48.32239598606157926 ) ) ;
#7380=FACE_OUTER_BOUND ( 'NONE', #10896, .T. ) ;
#7381=CARTESIAN_POINT ( 'NONE',  ( -87.13368444201113050, 0.6697911384492148956, -21.49365365690828256 ) ) ;
#7382=FACE_OUTER_BOUND ( 'NONE', #22648, .T. ) ;
#7383=CARTESIAN_POINT ( 'NONE',  ( -135.8532207217289738, -21.81201906317757633, -21.81201906317793515 ) ) ;
#7384=CARTESIAN_POINT ( 'NONE',  ( 136.1360204305621266, 24.77266263493138965, -24.77266263493110188 ) ) ;
#7386=CARTESIAN_POINT ( 'NONE',  ( 0.2972598230769923355, 18.14793986248751168, -38.42060263243650553 ) ) ;
#7387=CARTESIAN_POINT ( 'NONE',  ( -91.56559293963834989, -12.25131212657475466, -12.25131212657495361 ) ) ;
#7388=CARTESIAN_POINT ( 'NONE',  ( 136.1360204305621551, -24.77266263493081766, -31.79587985999290112 ) ) ;
#7389=CARTESIAN_POINT ( 'NONE',  ( -30.26275506840323715, 29.48230279907829754, -29.48230279907758344 ) ) ;
#7392=CARTESIAN_POINT ( 'NONE',  ( 57.59792236341148453, -40.00000000000000000, -2.435789363418300546 ) ) ;
#7393=CARTESIAN_POINT ( 'NONE',  ( -86.96347745069645896, -12.89780903124443689, 43.67073346367968156 ) ) ;
#7394=CARTESIAN_POINT ( 'NONE',  ( -280.0000000000000000, 19.99999999999996092, 2.449293598294708485E-15 ) ) ;
#7395=ORIENTED_EDGE ( 'NONE', *, *, #8830, .T. ) ;
#7396=CARTESIAN_POINT ( 'NONE',  ( 184.8905102610680444, 41.77492675556005253, -14.79361573936377461 ) ) ;
#7397=CARTESIAN_POINT ( 'NONE',  ( 62.42050862285469748, 30.90338125512822387, 12.80059963906062315 ) ) ;
#7399=CARTESIAN_POINT ( 'NONE',  ( -5.379830816903821145, -42.60994460517692062, -23.18791234549714986 ) ) ;
#7401=CARTESIAN_POINT ( 'NONE',  ( -144.1957000274121867, -30.13184844814661645, 12.48102028665973506 ) ) ;
#7402=B_SPLINE_CURVE_WITH_KNOTS ( 'NONE', 3,
 ( #7868, #24524, #1906, #6282, #14397, #22529 ),
 .UNSPECIFIED., .F., .F.,
 ( 4, 2, 4 ),
 ( -5.998616622604924294E-08, 0.005994953700759752223, 0.01198996738768573142 ),
 .UNSPECIFIED. ) ;
#7404=CARTESIAN_POINT ( 'NONE',  ( 60.28378959952933513, -15.72633063269985421, 31.18416451510499954 ) ) ;
#7407=CARTESIAN_POINT ( 'NONE',  ( -89.92902785008701017, -20.17328762787301955, -8.734793929541259772 ) ) ;
#7408=CARTESIAN_POINT ( 'NONE',  ( 170.2234770963711128, 40.00000000000014211, -24.55285855007172913 ) ) ;
#7409=CARTESIAN_POINT ( 'NONE',  ( 136.1360204305621266, 1.473277640373554421E-13, -35.03383547441296741 ) ) ;
#7411=CARTESIAN_POINT ( 'NONE',  ( 163.1118516004056573, -12.73709011382472234, -2.449293598294708485E-15 ) ) ;
#7412=CARTESIAN_POINT ( 'NONE',  ( -144.1957134275961323, 12.48102206801882552, -30.13185274904616406 ) ) ;
#7414=CARTESIAN_POINT ( 'NONE',  ( 151.7948205124836534, -6.767089262349006873, 40.00000000000002132 ) ) ;
#7415=CARTESIAN_POINT ( 'NONE',  ( -192.9588430854690273, -14.46834944099973264, -40.00000000000002132 ) ) ;
#7416=CARTESIAN_POINT ( 'NONE',  ( 136.1360204305621266, -35.03383547441293899, 0.000000000000000000 ) ) ;
#7417=CARTESIAN_POINT ( 'NONE',  ( -162.0762913951021176, 40.00000000000001421, -1.694272876827905394 ) ) ;
#7418=CARTESIAN_POINT ( 'NONE',  ( 163.1118516004056573, 1.658263919738574066E-13, -12.73709011382475254 ) ) ;
#7419=CARTESIAN_POINT ( 'NONE',  ( -86.86493150571114086, -19.60045294882784717, -8.366608963953355627 ) ) ;
#7421=CARTESIAN_POINT ( 'NONE',  ( 98.29850319135208281, 8.262390927745583369, -18.22532005587680359 ) ) ;
#7422=CARTESIAN_POINT ( 'NONE',  ( 1.925538622597735339, 44.35335385591526602, -24.44644315488994479 ) ) ;
#7423=CARTESIAN_POINT ( 'NONE',  ( -208.1127848780264742, -55.00245453010926866, 40.00000000000002132 ) ) ;
#7426=CARTESIAN_POINT ( 'NONE',  ( -195.1686598214107846, 48.78512304063578853, -14.09692385499625900 ) ) ;
#7431=CARTESIAN_POINT ( 'NONE',  ( -93.02511667907101867, -20.50052124204851367, 8.946512270084788554 ) ) ;
#7432=CARTESIAN_POINT ( 'NONE',  ( 155.4809970915716519, 11.45899766888377869, -27.66446758342027934 ) ) ;
#7434=CARTESIAN_POINT ( 'NONE',  ( -96.93773665438905596, 8.190703376740906094, -20.92028269119429496 ) ) ;
#7440=CARTESIAN_POINT ( 'NONE',  ( -100.7734535825088358, 12.25131212657480440, 12.25131212657487012 ) ) ;
#7441=CARTESIAN_POINT ( 'NONE',  ( -200.0000000000000853, 44.88127304973836118, -30.70179486994623375 ) ) ;
#7442=CARTESIAN_POINT ( 'NONE',  ( 151.7948205124836250, 1.439163438361279259E-13, -33.23291073765553705 ) ) ;
#7443=CARTESIAN_POINT ( 'NONE',  ( -188.2995950289364657, -23.44932284466040784, 43.00522595870950937 ) ) ;
#7446=CARTESIAN_POINT ( 'NONE',  ( -198.0356074513804572, 1.247057299367198800E-13, -15.37879056873070560 ) ) ;
#7447=PRODUCT_DEFINITION_FORMATION_WITH_SPECIFIED_SOURCE ( 'ANY', '', #10401, .NOT_KNOWN. ) ;
#7448=CARTESIAN_POINT ( 'NONE',  ( -208.1127848780264742, -39.99999999999948841, -55.00245453010965235 ) ) ;
#7449=CARTESIAN_POINT ( 'NONE',  ( -114.7465989397656756, -17.47221266594894473, 13.54917888340187204 ) ) ;
#7450=CARTESIAN_POINT ( 'NONE',  ( 136.1360204305621266, 24.77266263493138965, -24.77266263493110188 ) ) ;
#7451=CARTESIAN_POINT ( 'NONE',  ( -91.56559293963834989, 6.234561990864368500E-14, -22.67402823373191723 ) ) ;
#7452=CARTESIAN_POINT ( 'NONE',  ( -192.1963514251162621, 24.16258207727632978, 43.96876056339223027 ) ) ;
#7454=CARTESIAN_POINT ( 'NONE',  ( -86.84962968273566730, 19.67999904273991163, 8.151722510992470916 ) ) ;
#7455=CARTESIAN_POINT ( 'NONE',  ( 151.7948205124836250, 23.49921654116361225, -23.49921654116333514 ) ) ;
#7456=CARTESIAN_POINT ( 'NONE',  ( -162.0762913951021176, -40.00000000000005684, 1.694272876828184504 ) ) ;
#7457=CARTESIAN_POINT ( 'NONE',  ( 4.995406935893297096, 10.78321810387837232, 67.35176059880234334 ) ) ;
#7460=CARTESIAN_POINT ( 'NONE',  ( -56.48582580120558561, -21.81201906317755146, -21.81201906317792449 ) ) ;
#7461=CARTESIAN_POINT ( 'NONE',  ( 116.7964245048382850, -2.716484884814708943E-13, 27.98274000340149925 ) ) ;
#7462=VERTEX_POINT ( 'NONE', #4391 ) ;
#7463=CARTESIAN_POINT ( 'NONE',  ( 184.8905102610680444, 41.77492675555983936, 14.79361573936436081 ) ) ;
#7467=CARTESIAN_POINT ( 'NONE',  ( 4.995406935893297984, -39.99999999999986500, -15.24977328854874870 ) ) ;
#7469=CARTESIAN_POINT ( 'NONE',  ( -40.07203023071645021, 16.33025453615710632, 32.10811084141644045 ) ) ;
#7472=VERTEX_POINT ( 'NONE', #24609 ) ;
#7473=CARTESIAN_POINT ( 'NONE',  ( -197.4153392275794658, -49.11379398046383216, -14.14666332908225321 ) ) ;
#7474=CARTESIAN_POINT ( 'NONE',  ( -86.96347745069645896, 39.99999999999994316, 18.24025645688366737 ) ) ;
#7478=CARTESIAN_POINT ( 'NONE',  ( 0.2972598230770030492, -1.921041075453695163E-13, 54.33493731733936016 ) ) ;
#7480=CARTESIAN_POINT ( 'NONE',  ( 130.8568914410475372, 1.429239637432775288E-13, -34.05028731879788495 ) ) ;
#7482=SPHERICAL_SURFACE ( 'NONE', #17277, 15.00000000000000000 ) ;
#7483=CARTESIAN_POINT ( 'NONE',  ( -5.152948516943947510, -13.74948675458091785, -46.60473671797106476 ) ) ;
#7484=CARTESIAN_POINT ( 'NONE',  ( -162.0762913951020892, -1.198031840315659124, -57.76657433523998009 ) ) ;
#7486=CARTESIAN_POINT ( 'NONE',  ( -105.2054292635175585, -21.49321519473986442, -7.030298963786045751E-29 ) ) ;
#7487=CARTESIAN_POINT ( 'NONE',  ( 136.1360204305621551, -40.00000000000036238, 35.03383547441254109 ) ) ;
#7488=CARTESIAN_POINT ( 'NONE',  ( 35.93675087557281245, -42.26938917802861084, -12.87543817561850723 ) ) ;
#7489=CARTESIAN_POINT ( 'NONE',  ( 91.82158438592156813, 17.20528682183302038, 40.00000000000002132 ) ) ;
#7490=CARTESIAN_POINT ( 'NONE',  ( -56.48582580120558561, -30.84685318188645553, -40.00000000000002132 ) ) ;
#7491=CARTESIAN_POINT ( 'NONE',  ( 0.2972598230769976091, -10.13633138497479180, 10.13633138497468522 ) ) ;
#7492=CARTESIAN_POINT ( 'NONE',  ( 170.2234770963711128, 24.55285855007190321, 0.000000000000000000 ) ) ;
#7493=CARTESIAN_POINT ( 'NONE',  ( 23.23639021239542046, -42.89921396172177026, -23.37084785298091205 ) ) ;
#7495=CARTESIAN_POINT ( 'NONE',  ( -56.48582580120559271, -1.062504017861011783E-13, 9.153146818113587102 ) ) ;
#7496=CARTESIAN_POINT ( 'NONE',  ( 192.4448373802100889, 14.14213562370310662, 14.14213562370312438 ) ) ;
#7497=CARTESIAN_POINT ( 'NONE',  ( -105.3755690713226727, 18.24025645688350750, 2.449293598294708485E-15 ) ) ;
#7499=CARTESIAN_POINT ( 'NONE',  ( 83.06440094974429655, -23.65491511365441113, 10.91839312112026050 ) ) ;
#7500=CARTESIAN_POINT ( 'NONE',  ( -83.21262154144274348, 13.72187187063241609, 33.12752917117732210 ) ) ;
#7502=EDGE_CURVE ( 'NONE', #16387, #18786, #3823, .T. ) ;
#7503=CARTESIAN_POINT ( 'NONE',  ( 0.2972598230769907257, 66.70487387989857098, 10.13633138497486641 ) ) ;
#7504=CARTESIAN_POINT ( 'NONE',  ( 4.995406935893297984, -40.00000000000007816, 15.24977328854818914 ) ) ;
#7505=CARTESIAN_POINT ( 'NONE',  ( -213.1075012329537230, 37.98287015391211696, 18.58567234101190735 ) ) ;
#7507=CARTESIAN_POINT ( 'NONE',  ( 200.0000000000000000, 19.99999999999996447, -40.00000000000002132 ) ) ;
#7508=CARTESIAN_POINT ( 'NONE',  ( -163.5815439468644854, -35.61501074489159180, -18.59457101073931540 ) ) ;
#7511=EDGE_CURVE ( 'NONE', #12221, #2784, #10071, .T. ) ;
#7512=CARTESIAN_POINT ( 'NONE',  ( 170.0000000000000000, 12.70659020859086574, 21.59613885783099718 ) ) ;
#7513=CARTESIAN_POINT ( 'NONE',  ( -56.48582580120559982, 21.81201906317729922, 34.75652343174635917 ) ) ;
#7514=CARTESIAN_POINT ( 'NONE',  ( -198.0356074513804288, -39.15871834505882276, -39.15871834505946936 ) ) ;
#7515=DIRECTION ( 'NONE',  ( 0.000000000000000000, 1.000000000000000000, 0.000000000000000000 ) ) ;
#7516=CARTESIAN_POINT ( 'NONE',  ( -82.28162732578149985, 9.169756991572501903, -18.01798805106890811 ) ) ;
#7517=CARTESIAN_POINT ( 'NONE',  ( 170.2234770963711128, 17.36149277827028925, -39.20704971665377059 ) ) ;
#7518=CARTESIAN_POINT ( 'NONE',  ( 4.995406935893300648, -10.78321810387790514, -67.35176059880241439 ) ) ;
#7519=CARTESIAN_POINT ( 'NONE',  ( 170.2234770963711128, -45.64576402573167258, -10.92277846919254891 ) ) ;
#7520=CARTESIAN_POINT ( 'NONE',  ( 14.38125909742181285, -17.55144818341421598, -39.01709431150935359 ) ) ;
#7521=CARTESIAN_POINT ( 'NONE',  ( -105.2274517607656463, -13.17594969608524735, 17.01575307706266571 ) ) ;
#7523=CARTESIAN_POINT ( 'NONE',  ( 4.995406935893297984, -40.00000000000007816, 15.24977328854818914 ) ) ;
#7524=CARTESIAN_POINT ( 'NONE',  ( -100.7734535825088500, 16.03295912088683295, 40.53558337403684675 ) ) ;
#7526=CARTESIAN_POINT ( 'NONE',  ( -238.4067589809705794, 40.96449427990177128, 40.00000000000002132 ) ) ;
#7528=CARTESIAN_POINT ( 'NONE',  ( 0.2972598230769886718, 38.42060263243669027, -18.14793986248710667 ) ) ;
#7529=CARTESIAN_POINT ( 'NONE',  ( 24.48536172914053566, 41.83775886953835510, 17.32976714305807775 ) ) ;
#7531=CARTESIAN_POINT ( 'NONE',  ( 98.29820294267335612, -19.49240851343218850, -4.524526698153942483 ) ) ;
#7533=CARTESIAN_POINT ( 'NONE',  ( -188.9001212172966291, -43.30535683045341955, 17.93766612257997295 ) ) ;
#7535=CARTESIAN_POINT ( 'NONE',  ( 23.13330272892053330, -17.84165608060301622, 43.07356808498551715 ) ) ;
#7536=CARTESIAN_POINT ( 'NONE',  ( 11.71430589693755131, 24.82930166508055692, -44.87285427231127954 ) ) ;
#7538=CARTESIAN_POINT ( 'NONE',  ( -96.93773665438882858, -20.58457565566404313, -9.001171854902130676 ) ) ;
#7539=CARTESIAN_POINT ( 'NONE',  ( 192.4448373802101173, 39.99999999999998579, 19.99999999996075317 ) ) ;
#7540=CARTESIAN_POINT ( 'NONE',  ( 170.0000000000000000, -24.95097643316997704, 0.000000000000000000 ) ) ;
#7542=CARTESIAN_POINT ( 'NONE',  ( -208.1127848780264742, -15.00245453012673202, 40.00000000000002132 ) ) ;
#7543=CARTESIAN_POINT ( 'NONE',  ( 98.29820294267328507, -7.653668647303858208, -18.47759065023126723 ) ) ;
#7546=CARTESIAN_POINT ( 'NONE',  ( -135.8532207217289454, -30.84685318188648750, -40.00000000000002132 ) ) ;
#7547=CARTESIAN_POINT ( 'NONE',  ( 151.7948205124836534, -33.23291073765550863, 40.00000000000002132 ) ) ;
#7548=CARTESIAN_POINT ( 'NONE',  ( -213.1075012329537230, 5.259461644596141978E-13, -53.71589010951915100 ) ) ;
#7549=CARTESIAN_POINT ( 'NONE',  ( 19.06497207195981147, 1.521599808664285085E-13, -14.19242893257840521 ) ) ;
#7555=CARTESIAN_POINT ( 'NONE',  ( -96.94475454968979022, -8.190683501892733531, 20.92018922310777285 ) ) ;
#7557=ORIENTED_EDGE ( 'NONE', *, *, #22503, .T. ) ;
#7559=CARTESIAN_POINT ( 'NONE',  ( -100.7734535825088500, 16.03295912088713848, -16.03295912088698927 ) ) ;
#7561=ORIENTED_EDGE ( 'NONE', *, *, #18243, .F. ) ;
#7562=CARTESIAN_POINT ( 'NONE',  ( -259.2033419157646676, -9.517827891722680178, -40.00000000000002132 ) ) ;
#7563=CARTESIAN_POINT ( 'NONE',  ( -94.58414068588119505, -20.73981583676798479, 8.590713000820761280 ) ) ;
#7564=ORIENTED_EDGE ( 'NONE', *, *, #8835, .F. ) ;
#7567=CARTESIAN_POINT ( 'NONE',  ( -162.0762913951020892, 29.48230308784758691, 29.48230308784772191 ) ) ;
#7569=CARTESIAN_POINT ( 'NONE',  ( -135.8532207217289738, 7.002209520526292428E-15, -9.153146818113572891 ) ) ;
#7570=CARTESIAN_POINT ( 'NONE',  ( -189.4799804244525490, -23.69387126430439494, 43.33513910317159201 ) ) ;
#7574=CARTESIAN_POINT ( 'NONE',  ( 184.8905102610680444, -40.00000000000021316, 20.92133201514402430 ) ) ;
#7575=ADVANCED_FACE ( 'NONE', ( #19516 ), #4136, .T. ) ;
#7576=CARTESIAN_POINT ( 'NONE',  ( -105.2055636155751728, -14.22328983910611555, 16.17146666061736937 ) ) ;
#7577=CARTESIAN_POINT ( 'NONE',  ( 0.2972598230769976091, -10.13633138497479180, 10.13633138497468522 ) ) ;
#7578=CARTESIAN_POINT ( 'NONE',  ( 163.1118516004056573, 40.00000000000014921, -27.26290988616858968 ) ) ;
#7579=CARTESIAN_POINT ( 'NONE',  ( 91.82158438592156813, -16.11829626348402655, -40.45024623143966380 ) ) ;
#7580=CARTESIAN_POINT ( 'NONE',  ( 155.4809970915716235, 27.66446758342027223, 11.45899766888373783 ) ) ;
#7583=CARTESIAN_POINT ( 'NONE',  ( 14.38125909742180220, 40.00000000000017764, -15.17850393972591760 ) ) ;
#7584=CARTESIAN_POINT ( 'NONE',  ( -259.2033419157646676, -40.00000000000017764, 30.48217210827725054 ) ) ;
#7585=CARTESIAN_POINT ( 'NONE',  ( -30.26275506840324070, -27.08623969584595770, 29.48230279907789608 ) ) ;
#7586=CARTESIAN_POINT ( 'NONE',  ( 192.4448373802101173, -42.42640687116510634, 14.14213562375845257 ) ) ;
#7587=CARTESIAN_POINT ( 'NONE',  ( -183.1091233173586090, -22.43565125817906392, -41.47045062402216331 ) ) ;
#7588=CARTESIAN_POINT ( 'NONE',  ( 192.4448373802100889, 14.14213562375893574, -14.14213562375874922 ) ) ;
#7590=CARTESIAN_POINT ( 'NONE',  ( 146.6084372240433993, 3.800685668858732935, -3.800685668858610367 ) ) ;
#7591=CARTESIAN_POINT ( 'NONE',  ( 170.2234770963711128, 24.55285855007190321, 0.000000000000000000 ) ) ;
#7593=CARTESIAN_POINT ( 'NONE',  ( -135.8532207217289738, -6.472252184283586729, -50.09629031063973770 ) ) ;
#7594=CARTESIAN_POINT ( 'NONE',  ( -87.02123777084361222, 5.414077845889153195, 20.76518631983113750 ) ) ;
#7596=CARTESIAN_POINT ( 'NONE',  ( -109.1264249741485060, 13.72187187123402907, -33.12752917269585851 ) ) ;
#7598=CARTESIAN_POINT ( 'NONE',  ( -40.07203023092437633, 11.15662918590678565, 34.25109662808139177 ) ) ;
#7601=CARTESIAN_POINT ( 'NONE',  ( 136.1360204305621266, 4.966164525587089429, 2.449293598294708485E-15 ) ) ;
#7602=CARTESIAN_POINT ( 'NONE',  ( -194.7884774423165197, -44.44046305923735929, -18.40784251728739562 ) ) ;
#7603=CARTESIAN_POINT ( 'NONE',  ( -135.8532207217289738, 40.00000000000002842, -9.153146818113432559 ) ) ;
#7606=CARTESIAN_POINT ( 'NONE',  ( -259.2033419157646676, 39.99999999999987921, 9.517827891723049660 ) ) ;
#7608=CARTESIAN_POINT ( 'NONE',  ( 146.6084372240433993, 1.478241399363601114E-13, -34.62501878078305850 ) ) ;
#7609=CARTESIAN_POINT ( 'NONE',  ( -198.1130638040447423, 43.61599283946033268, 18.06633577047154304 ) ) ;
#7610=CARTESIAN_POINT ( 'NONE',  ( -4.037857402784342575, -13.82822410908647903, -46.99101396955030907 ) ) ;
#7611=CARTESIAN_POINT ( 'NONE',  ( -213.1075012329537230, 18.58567234101174037, -37.98287015391222354 ) ) ;
#7612=CARTESIAN_POINT ( 'NONE',  ( -87.13361725327075646, -15.19799821270861706, 15.19799821270823159 ) ) ;
#7615=CARTESIAN_POINT ( 'NONE',  ( 19.06497207195980792, -14.19242893257839988, 40.00000000000002132 ) ) ;
#7616=CARTESIAN_POINT ( 'NONE',  ( -280.0000000000000568, 19.99999999999996092, -40.00000000000002132 ) ) ;
#7617=CARTESIAN_POINT ( 'NONE',  ( -238.4067589809705794, -0.6820004457913680929, 0.6820004457913170226 ) ) ;
#7618=CARTESIAN_POINT ( 'NONE',  ( 136.1360204305621266, 35.03383547441298873, 0.000000000000000000 ) ) ;
#7619=CARTESIAN_POINT ( 'NONE',  ( -105.2502153031283143, 3.401878988843269003, 21.20171025720689784 ) ) ;
#7620=CARTESIAN_POINT ( 'NONE',  ( -77.90255099906769942, 20.29001641120678201, -8.064892378658056415 ) ) ;
#7621=CARTESIAN_POINT ( 'NONE',  ( 200.0000000000000000, -14.14213562373106114, 42.42640687119278908 ) ) ;
#7622=CARTESIAN_POINT ( 'NONE',  ( 0.2972598230769930572, 54.33493731733936016, 2.449293598294708485E-15 ) ) ;
#7624=AXIS2_PLACEMENT_3D ( 'NONE', #16907, #4819, #8390 ) ;
#7625=CARTESIAN_POINT ( 'NONE',  ( 83.01683444506817011, -24.01517293250395824, 9.947410331339252565 ) ) ;
#7626=CARTESIAN_POINT ( 'NONE',  ( -4.039451493210485467, -13.82811171175474207, 46.99046209229799587 ) ) ;
#7627=CARTESIAN_POINT ( 'NONE',  ( -91.56559293963834989, 12.25131212657490209, -44.31723036834897300 ) ) ;
#7628=CARTESIAN_POINT ( 'NONE',  ( 136.1360204305621266, 5.219216885335291329E-15, 4.966164525587064560 ) ) ;
#7629=CARTESIAN_POINT ( 'NONE',  ( 14.38125909742180752, 10.73282306404735387, -10.73282306404708919 ) ) ;
#7630=CARTESIAN_POINT ( 'NONE',  ( -238.4067589809705794, 0.9644942799825385604, 40.00000000000002132 ) ) ;
#7631=CARTESIAN_POINT ( 'NONE',  ( -213.1075012329537230, 13.71589010951907994, 0.000000000000000000 ) ) ;
#7632=DIRECTION ( 'NONE',  ( 0.01051738792038020565, -0.9166396752531025260, 0.3995761383056042337 ) ) ;
#7635=CARTESIAN_POINT ( 'NONE',  ( -30.26275506840322649, -29.48230279907769358, -29.48230279907820162 ) ) ;
#7637=CARTESIAN_POINT ( 'NONE',  ( -114.7292050955122278, 21.84104191940862449, -3.341916304163401463 ) ) ;
#7638=CARTESIAN_POINT ( 'NONE',  ( 130.8568914410475372, -3.326198072800416995E-13, 34.05028731879788495 ) ) ;
#7639=CARTESIAN_POINT ( 'NONE',  ( 192.4448373802101173, 14.14213562375922884, -42.42640687116488607 ) ) ;
#7640=CARTESIAN_POINT ( 'NONE',  ( -56.48582580120558561, -21.81201906317755146, -21.81201906317792449 ) ) ;
#7641=CARTESIAN_POINT ( 'NONE',  ( -208.1127848780265026, 10.60833733269551615, -10.60833733269529766 ) ) ;
#7642=CARTESIAN_POINT ( 'NONE',  ( -91.56559293963834989, -44.31723036834885932, -12.25131212657538171 ) ) ;
#7643=CARTESIAN_POINT ( 'NONE',  ( -114.7539999065896126, -2.778737770292790898, -21.97438050586149316 ) ) ;
#7647=CARTESIAN_POINT ( 'NONE',  ( 91.82158438592159655, -40.00000000000008527, 22.79471317813456110 ) ) ;
#7648=CARTESIAN_POINT ( 'NONE',  ( 192.4448373802101173, 14.14213562375862665, 42.42640687116509213 ) ) ;
#7650=CARTESIAN_POINT ( 'NONE',  ( -56.48582580120559982, 30.84685318188643421, 40.00000000000002132 ) ) ;
#7652=CARTESIAN_POINT ( 'NONE',  ( 57.59792236341147031, 54.84617931850881689, -1.722363176414946073 ) ) ;
#7653=EDGE_CURVE ( 'NONE', #7864, #23212, #1300, .T. ) ;
#7654=CARTESIAN_POINT ( 'NONE',  ( 36.90243737664644641, 38.55584411169299841, 15.97035353980611205 ) ) ;
#7655=CARTESIAN_POINT ( 'NONE',  ( 67.79414719548810808, 14.15005687161725589, 28.72755866868557106 ) ) ;
#7656=CARTESIAN_POINT ( 'NONE',  ( -192.9588430854690273, 14.46834944099966336, 40.00000000000002132 ) ) ;
#7657=EDGE_CURVE ( 'NONE', #22554, #19424, #9538, .T. ) ;
#7658=ADVANCED_FACE ( 'NONE', ( #16317 ), #16455, .T. ) ;
#7660=CARTESIAN_POINT ( 'NONE',  ( -189.0115211946963427, -43.33403054566051793, 17.94954316430237284 ) ) ;
#7663=CARTESIAN_POINT ( 'NONE',  ( -3.966425590329079931, -23.46521855348130714, 43.02666064534189871 ) ) ;
#7664=CARTESIAN_POINT ( 'NONE',  ( 22.95085416411744461, 17.86294511971856380, -43.12496437194744203 ) ) ;
#7666=CARTESIAN_POINT ( 'NONE',  ( 125.5832160019859884, -28.05309928654004281, 11.61997419108369733 ) ) ;
#7669=CARTESIAN_POINT ( 'NONE',  ( -213.1075012329537230, 9.698598906438871126, -66.26714140136179765 ) ) ;
#7670=CARTESIAN_POINT ( 'NONE',  ( 130.8568914410475372, -5.949712681206667853, -2.449293598294708485E-15 ) ) ;
#7672=CARTESIAN_POINT ( 'NONE',  ( -144.0562696877211124, 14.68019673968441552, -29.54283206240011950 ) ) ;
#7674=CARTESIAN_POINT ( 'NONE',  ( 170.2234770963711128, 24.55285855007190321, 0.000000000000000000 ) ) ;
#7675=CARTESIAN_POINT ( 'NONE',  ( 91.82158438592156813, 17.20528682183302038, -40.00000000000002132 ) ) ;
#7677=CARTESIAN_POINT ( 'NONE',  ( -213.1075012329537230, 53.71589010953660193, 40.00000000000002132 ) ) ;
#7678=CARTESIAN_POINT ( 'NONE',  ( -86.96347745069643054, -39.99999999999985079, -18.24025645688394448 ) ) ;
#7679=CARTESIAN_POINT ( 'NONE',  ( 136.1360204305621266, -3.419521671106983309E-13, 35.03383547441296741 ) ) ;
#7680=CARTESIAN_POINT ( 'NONE',  ( 130.8568914410475088, 52.36146031193427319, -4.207082182989173802 ) ) ;
#7681=ORIENTED_EDGE ( 'NONE', *, *, #3619, .F. ) ;
#7682=DIRECTION ( 'NONE',  ( 0.000000000000000000, -0.9166903767145597737, 0.3995982397845596612 ) ) ;
#7683=CARTESIAN_POINT ( 'NONE',  ( -259.2033419157646676, -6.730120644403570829, -6.730120644403545960 ) ) ;
#7685=CARTESIAN_POINT ( 'NONE',  ( -94.58360650948853277, -9.000712009830975191, 20.58386743644871331 ) ) ;
#7689=CARTESIAN_POINT ( 'NONE',  ( -91.56559293963836410, -12.25131212657462321, -44.31723036834905827 ) ) ;
#7690=CARTESIAN_POINT ( 'NONE',  ( 20.38198589864675014, -43.75891014378044019, -18.12553405624110781 ) ) ;
#7693=CARTESIAN_POINT ( 'NONE',  ( 130.8568914410475088, 5.949712681206719367, -40.00000000000002132 ) ) ;
#7694=CARTESIAN_POINT ( 'NONE',  ( -88.37877758187065069, -19.92653024478079615, 8.575405934537359443 ) ) ;
#7695=ORIENTED_EDGE ( 'NONE', *, *, #8822, .T. ) ;
#7699=CARTESIAN_POINT ( 'NONE',  ( 151.7948205124836250, 4.785054706301690608, 4.785054706301682614 ) ) ;
#7701=CARTESIAN_POINT ( 'NONE',  ( 170.2234770963711128, 1.169953928977015745E-13, -24.55285855007187124 ) ) ;
#7702=CARTESIAN_POINT ( 'NONE',  ( 146.6084372240433993, -34.62501878078303008, 0.000000000000000000 ) ) ;
#7706=CARTESIAN_POINT ( 'NONE',  ( -213.1075012329537230, -39.99999999999991473, -13.71589010951953647 ) ) ;
#7707=CARTESIAN_POINT ( 'NONE',  ( -110.0960685945389343, -12.40690815812826386, 15.98210693808425376 ) ) ;
#7708=CARTESIAN_POINT ( 'NONE',  ( -91.56559293963834989, -40.53558337403669753, -16.03295912088728770 ) ) ;
#7709=CARTESIAN_POINT ( 'NONE',  ( 151.7948205124836250, 33.23291073765556547, 0.000000000000000000 ) ) ;
#7710=CARTESIAN_POINT ( 'NONE',  ( 163.1118516004056573, -9.006482792073960297, -47.56205970284963769 ) ) ;
#7712=CARTESIAN_POINT ( 'NONE',  ( -77.78673448795234435, 9.959188558496546051, -19.58653132801435959 ) ) ;
#7713=CARTESIAN_POINT ( 'NONE',  ( -213.1075012329537230, 1.045191102001431893E-13, -13.71589010951911902 ) ) ;
#7714=CARTESIAN_POINT ( 'NONE',  ( 199.9999999999999432, 1.065690307512836407E-13, -20.00000000000010303 ) ) ;
#7715=CARTESIAN_POINT ( 'NONE',  ( 130.8568914410475372, 4.207082182992862407, 4.207082182992856190 ) ) ;
#7717=CARTESIAN_POINT ( 'NONE',  ( -114.7410223956348148, 17.58920299499807172, 13.38943653989989890 ) ) ;
#7718=CARTESIAN_POINT ( 'NONE',  ( -195.1685814578900420, -24.52825302095775939, -44.46431112711859157 ) ) ;
#7719=CARTESIAN_POINT ( 'NONE',  ( -238.4067589809705794, -0.6820004457913680929, 0.6820004457913170226 ) ) ;
#7721=CARTESIAN_POINT ( 'NONE',  ( -100.7734535825088500, -16.03295912088659492, -40.53558337403696044 ) ) ;
#7722=CARTESIAN_POINT ( 'NONE',  ( 0.2972598230769983307, -14.33493731733933352, -40.00000000000002132 ) ) ;
#7723=( BOUNDED_SURFACE ( )  B_SPLINE_SURFACE ( 3, 2, ( 
 ( #6155, #20264, #4041 ),
 ( #20129, #10407, #8408 ),
 ( #8273, #2043, #24389 ),
 ( #18524, #16397, #20662 ),
 ( #10149, #14532, #14401 ),
 ( #18252, #14265, #22530 ),
 ( #10012, #6414, #4312 ),
 ( #20527, #305, #1908 ),
 ( #16530, #18120, #26272 ),
 ( #8010, #24255, #8545 ),
 ( #4703, #6810, #14926 ),
 ( #2710, #23063, #8948 ) ),
 .UNSPECIFIED., .F., .F., .F. ) 
 B_SPLINE_SURFACE_WITH_KNOTS ( ( 4, 2, 2, 2, 2, 4 ),
 ( 3, 3 ),
 ( 0.006022589392325016291, 0.01254516766564325869, 0.01580645680230238076, 0.01906774593896149936, 0.02559032421227974002, 0.03211290248559798416 ),
 ( 0.000000000000000000, 1.000000000000000000 ),
 .UNSPECIFIED. ) 
 GEOMETRIC_REPRESENTATION_ITEM ( )  RATIONAL_B_SPLINE_SURFACE ( (
 ( 1.000000000000000000, 0.9998834880171258988, 1.000000000000000000),
 ( 1.000000000000000000, 0.9998139205012253061, 1.000000000000000000),
 ( 1.000000000000000000, 0.9997315632444677691, 1.000000000000000000),
 ( 1.000000000000000000, 0.9996405464946958030, 1.000000000000000000),
 ( 1.000000000000000000, 0.9996155081776924023, 1.000000000000000000),
 ( 1.000000000000000000, 0.9995814087511104562, 1.000000000000000000),
 ( 1.000000000000000000, 0.9995724100939918921, 1.000000000000000000),
 ( 1.000000000000000000, 0.9995726760936894939, 1.000000000000000000),
 ( 1.000000000000000000, 0.9996103361816741639, 1.000000000000000000),
 ( 1.000000000000000000, 0.9997312749796802844, 1.000000000000000000),
 ( 1.000000000000000000, 0.9998135910914284219, 1.000000000000000000),
 ( 1.000000000000000000, 0.9998834880173383954, 1.000000000000000000) ) ) 
 REPRESENTATION_ITEM ( '' )  SURFACE ( )  );
#7724=CARTESIAN_POINT ( 'NONE',  ( 200.0000000000000000, -14.14213562373046784, -42.42640687119298804 ) ) ;
#7725=CARTESIAN_POINT ( 'NONE',  ( -87.13361725327075646, -2.411356650979015128E-13, 21.49321519333430430 ) ) ;
#7727=CARTESIAN_POINT ( 'NONE',  ( -259.2033419157646676, -1.473088368616265084E-13, 9.517827891722632216 ) ) ;
#7729=CARTESIAN_POINT ( 'NONE',  ( -4.027137536850666777, 13.82877337592787015, 46.99492183298313819 ) ) ;
#7732=CARTESIAN_POINT ( 'NONE',  ( 163.1118516004056573, 12.73709011382478273, 2.449293598294708485E-15 ) ) ;
#7733=CARTESIAN_POINT ( 'NONE',  ( -195.5008451367067721, -44.52806290063275441, -18.44412755964722450 ) ) ;
#7734=CARTESIAN_POINT ( 'NONE',  ( -30.26275506840325136, 40.00000000000001421, 1.694272468446399227 ) ) ;
#7735=CARTESIAN_POINT ( 'NONE',  ( -114.4364955367327497, -20.04994829327637262, -8.644468109209869411 ) ) ;
#7736=LINE ( 'NONE', #25860, #4087 ) ;
#7737=CARTESIAN_POINT ( 'NONE',  ( 48.46158794344649579, 18.19743102720972416, -35.02055625264701888 ) ) ;
#7741=CARTESIAN_POINT ( 'NONE',  ( -195.2739252856439407, 43.39389462262437291, 17.97433967688010270 ) ) ;
#7742=CARTESIAN_POINT ( 'NONE',  ( 6.762329110801217347, -18.56720258520416067, -44.82519229650321790 ) ) ;
#7743=CARTESIAN_POINT ( 'NONE',  ( 163.1118516004056573, -37.29075403953166301, 19.27778845539196695 ) ) ;
#7744=CARTESIAN_POINT ( 'NONE',  ( 116.7964245048381429, -19.78678521258544620, 19.78678521258498435 ) ) ;
#7745=CARTESIAN_POINT ( 'NONE',  ( -208.1127848780264742, -67.17687982763172272, 10.60833733270744617 ) ) ;
#7746=CARTESIAN_POINT ( 'NONE',  ( 91.82158438592159655, -40.00000000000017764, 17.20528682183258340 ) ) ;
#7747=DIRECTION ( 'NONE',  ( -1.000000000000000000, -1.836970198721024264E-16, 0.000000000000000000 ) ) ;
#7749=CARTESIAN_POINT ( 'NONE',  ( -259.2033419157646676, -30.48217210827744950, 40.00000000000002132 ) ) ;
#7751=CARTESIAN_POINT ( 'NONE',  ( 136.1360204305621551, 24.77266263493108411, 31.79587985999273769 ) ) ;
#7752=CARTESIAN_POINT ( 'NONE',  ( 14.38125909742182884, -55.17850393974264733, -40.00000000000002132 ) ) ;
#7754=CARTESIAN_POINT ( 'NONE',  ( -213.1075012329537230, 40.00000000000012790, -13.71589010951869980 ) ) ;
#7755=CARTESIAN_POINT ( 'NONE',  ( 4.995406935893290878, 39.06748935135185263, 39.06748935135198764 ) ) ;
#7756=EDGE_CURVE ( 'NONE', #24877, #4727, #12083, .T. ) ;
#7757=CARTESIAN_POINT ( 'NONE',  ( 14.38125909742180752, 15.17850393972634038, -40.00000000000002132 ) ) ;
#7760=CARTESIAN_POINT ( 'NONE',  ( 44.82887508593488946, -38.96139886170605848, 12.17256213108278828 ) ) ;
#7761=CARTESIAN_POINT ( 'NONE',  ( -213.1075012329537230, 66.26714140136188291, 9.698598906438215650 ) ) ;
#7762=CARTESIAN_POINT ( 'NONE',  ( 91.82158438592159655, -40.00000000000008527, 22.79471317813456110 ) ) ;
#7763=CARTESIAN_POINT ( 'NONE',  ( -192.9588430854689989, 10.23066800230756712, -10.23066800230735396 ) ) ;
#7764=CARTESIAN_POINT ( 'NONE',  ( 151.7948205124836250, -3.202120068677277203E-13, 33.23291073765553705 ) ) ;
#7765=CARTESIAN_POINT ( 'NONE',  ( 14.38125909742180752, 15.17850393972634038, 0.000000000000000000 ) ) ;
#7769=CARTESIAN_POINT ( 'NONE',  ( -91.56559293963834989, 40.53558337403654832, 16.03295912088756481 ) ) ;
#7770=CARTESIAN_POINT ( 'NONE',  ( 170.2234770963711128, 45.64576402573196390, -10.92277846919159856 ) ) ;
#7771=CARTESIAN_POINT ( 'NONE',  ( -77.58504657351252831, -21.97438139950685354, -2.778622652594447295 ) ) ;
#7772=CARTESIAN_POINT ( 'NONE',  ( -82.28266731796803413, 17.99064928892941140, -9.155589012553823736 ) ) ;
#7773=CARTESIAN_POINT ( 'NONE',  ( -86.96347745069644475, -12.89780903124395195, -12.89780903124416511 ) ) ;
#7774=CARTESIAN_POINT ( 'NONE',  ( 130.8568914410475088, 24.07718906446937623, -32.49135343045455215 ) ) ;
#7775=CARTESIAN_POINT ( 'NONE',  ( 4.995406935893289102, 10.78321810389013002, -10.78321810388986712 ) ) ;
#7776=CARTESIAN_POINT ( 'NONE',  ( 151.7948205124836534, -51.78348778862529400, -4.785054706299085581 ) ) ;
#7777=CARTESIAN_POINT ( 'NONE',  ( 184.8905102610680444, -20.92133201514440799, 0.000000000000000000 ) ) ;
#7780=CARTESIAN_POINT ( 'NONE',  ( 192.4448373802101173, -39.99999999999991473, -20.00000000003956302 ) ) ;
#7781=CARTESIAN_POINT ( 'NONE',  ( 0.2972598230769923355, 18.14793986248697166, 38.42060263243675422 ) ) ;
#7783=CARTESIAN_POINT ( 'NONE',  ( 0.2972598230769930017, 54.33493731733936016, 40.00000000000002132 ) ) ;
#7785=CARTESIAN_POINT ( 'NONE',  ( 136.1360204305621551, 3.511608612530801032, -53.05693388239316022 ) ) ;
#7786=CARTESIAN_POINT ( 'NONE',  ( 94.73518454776767328, 19.78402239393997419, 8.194810393863161124 ) ) ;
#7787=CARTESIAN_POINT ( 'NONE',  ( 23.49666234703747847, 13.79192166426321720, 46.76389514419428650 ) ) ;
#7788=CARTESIAN_POINT ( 'NONE',  ( -162.0762913951020892, 1.694272876828294194, 0.000000000000000000 ) ) ;
#7789=ORIENTED_EDGE ( 'NONE', *, *, #7052, .T. ) ;
#7790=CARTESIAN_POINT ( 'NONE',  ( -189.5227390968213115, -43.46195835885610137, 18.00253259953374751 ) ) ;
#7792=CARTESIAN_POINT ( 'NONE',  ( 3.869409319468993580, -14.12455301873678515, 48.96737585073453403 ) ) ;
#7793=EDGE_CURVE ( 'NONE', #14842, #10807, #853, .T. ) ;
#7794=CARTESIAN_POINT ( 'NONE',  ( 23.36927571439210993, 13.80130822340207430, -46.80992244775424638 ) ) ;
#7798=CARTESIAN_POINT ( 'NONE',  ( -129.2303573021155216, -11.67678754051281409, 24.84170325990223205 ) ) ;
#7799=CARTESIAN_POINT ( 'NONE',  ( -91.56559293963834989, -16.03295912088659492, -40.53558337403696044 ) ) ;
#7800=CARTESIAN_POINT ( 'NONE',  ( 91.82158438592156813, 17.20528682183302038, 40.00000000000002132 ) ) ;
#7801=CARTESIAN_POINT ( 'NONE',  ( -174.2682069750576659, 16.26528465553901981, -39.26787081121104706 ) ) ;
#7803=EDGE_CURVE ( 'NONE', #10709, #4560, #10679, .T. ) ;
#7804=CARTESIAN_POINT ( 'NONE',  ( 163.1118516004056573, 27.26290988616875310, 0.000000000000000000 ) ) ;
#7805=CARTESIAN_POINT ( 'NONE',  ( -105.3755690713226585, -18.24025645688353947, -40.00000000000002132 ) ) ;
#7806=CARTESIAN_POINT ( 'NONE',  ( -30.26275506840324070, 1.694272468446254232, 0.000000000000000000 ) ) ;
#7807=CARTESIAN_POINT ( 'NONE',  ( -162.0762913951020892, 4.094006889353306706E-13, -41.69427287682835015 ) ) ;
#7808=CARTESIAN_POINT ( 'NONE',  ( -238.4067589809705794, -3.369206980223063916E-14, -0.9644942799825824142 ) ) ;
#7809=CARTESIAN_POINT ( 'NONE',  ( 19.06497207195980792, 18.24870850772790831, -38.31983398719609824 ) ) ;
#7811=CARTESIAN_POINT ( 'NONE',  ( -86.91014751117378978, 20.05881702300802516, -7.317915707774923284 ) ) ;
#7812=CARTESIAN_POINT ( 'NONE',  ( -208.1127848780265026, -15.00245453012673202, 0.000000000000000000 ) ) ;
#7817=CARTESIAN_POINT ( 'NONE',  ( 57.59792236341148453, -54.84617931850877426, -1.722363176415331099 ) ) ;
#7818=CARTESIAN_POINT ( 'NONE',  ( 23.54890483848240379, -42.80335737019201758, -23.30407993985230064 ) ) ;
#7820=CARTESIAN_POINT ( 'NONE',  ( -162.0762913951021176, 1.694272876828294194, -40.00000000000002132 ) ) ;
#7821=CARTESIAN_POINT ( 'NONE',  ( -94.58360650941220626, -20.58386743640747341, 9.000712009939409342 ) ) ;
#7824=( BOUNDED_CURVE ( )  B_SPLINE_CURVE ( 3, ( #17572, #15203, #15326, #17194 ),
 .UNSPECIFIED., .F., .F. ) 
 B_SPLINE_CURVE_WITH_KNOTS ( ( 4, 4 ),
 ( 0.004183487405659220247, 0.01388163287021914813 ),
 .UNSPECIFIED. ) 
 CURVE ( )  GEOMETRIC_REPRESENTATION_ITEM ( )  RATIONAL_B_SPLINE_CURVE ( ( 0.6809743333591556924, 0.7608653435686150157, 0.8672072324488964146, 1.000000000000000000 ) ) 
 REPRESENTATION_ITEM ( '' )  );
#7825=DIRECTION ( 'NONE',  ( 1.000000000000000000, 1.836970198721030181E-16, 0.000000000000000000 ) ) ;
#7826=CARTESIAN_POINT ( 'NONE',  ( 19.06497207195979726, 38.31983398719629719, -18.24870850772750686 ) ) ;
#7827=CARTESIAN_POINT ( 'NONE',  ( -144.0562696871581920, -29.54283206217719382, -14.68019673973296868 ) ) ;
#7829=CARTESIAN_POINT ( 'NONE',  ( -280.0000000000000000, -1.237140859393462838E-13, 20.00000000000001421 ) ) ;
#7830=CARTESIAN_POINT ( 'NONE',  ( -91.56559293963834989, 17.32597176626808988, 40.00000000000002132 ) ) ;
#7832=CARTESIAN_POINT ( 'NONE',  ( -83.28983882461062649, 25.45044590560994990, 25.45044590561006004 ) ) ;
#7833=CARTESIAN_POINT ( 'NONE',  ( 14.38125909742181818, -40.00000000000007816, 15.17850393972619649 ) ) ;
#7834=CARTESIAN_POINT ( 'NONE',  ( -208.1127848780264742, -39.99999999999990763, -15.00245453012711394 ) ) ;
#7836=CARTESIAN_POINT ( 'NONE',  ( -280.0000000000000000, -14.14213562373108779, 14.14213562373088529 ) ) ;
#7837=EDGE_CURVE ( 'NONE', #20782, #6050, #18307, .T. ) ;
#7838=CARTESIAN_POINT ( 'NONE',  ( 57.59792236341147031, 2.435789363418170872, -40.00000000000002132 ) ) ;
#7840=CARTESIAN_POINT ( 'NONE',  ( -86.96347745069645896, -12.89780903124382938, -43.67073346367985920 ) ) ;
#7842=CARTESIAN_POINT ( 'NONE',  ( 17.75917311731582160, -48.46615948699198384, 14.04884443869907606 ) ) ;
#7843=CARTESIAN_POINT ( 'NONE',  ( -213.1075012329537230, 40.00000000000012790, -13.71589010951869980 ) ) ;
#7844=CARTESIAN_POINT ( 'NONE',  ( 146.6084372240433709, -39.99999999999987921, -34.62501878078319351 ) ) ;
#7846=CARTESIAN_POINT ( 'NONE',  ( -56.48582580120559982, 21.81201906317778594, -34.75652343174606074 ) ) ;
#7847=CARTESIAN_POINT ( 'NONE',  ( 4.995406935893297984, -39.06748935135205869, 17.50105314357158193 ) ) ;
#7848=CARTESIAN_POINT ( 'NONE',  ( -190.0144721487477852, -23.79987203023481968, -43.47822244618638621 ) ) ;
#7850=ORIENTED_EDGE ( 'NONE', *, *, #12009, .F. ) ;
#7851=CARTESIAN_POINT ( 'NONE',  ( 0.2972598230769938343, 10.13633138497486286, -10.13633138497461594 ) ) ;
#7852=CARTESIAN_POINT ( 'NONE',  ( 14.38125909742180752, 17.55144818341448953, 39.01709431150923280 ) ) ;
#7855=CARTESIAN_POINT ( 'NONE',  ( -135.8532207217289738, -34.75652343174584757, -21.81201906317816253 ) ) ;
#7856=CARTESIAN_POINT ( 'NONE',  ( -200.4318156386388523, -14.17468120671733089, -49.29858106685323804 ) ) ;
#7857=CARTESIAN_POINT ( 'NONE',  ( -77.70139926391286167, 5.508459030575254545, 21.34823270895579839 ) ) ;
#7862=CARTESIAN_POINT ( 'NONE',  ( 98.29820294268191105, -7.653668647302824368, -18.47759065022797031 ) ) ;
#7863=CARTESIAN_POINT ( 'NONE',  ( -4.037857402786239724, 13.82822410908674904, 46.99101396954952037 ) ) ;
#7864=VERTEX_POINT ( 'NONE', #19362 ) ;
#7866=CARTESIAN_POINT ( 'NONE',  ( 184.8905102610680444, -20.92133201514440799, 0.000000000000000000 ) ) ;
#7868=CARTESIAN_POINT ( 'NONE',  ( -188.2995950289364941, -43.00522595870984333, 23.44932284465888728 ) ) ;
#7869=CARTESIAN_POINT ( 'NONE',  ( -97.73860346104962105, -20.56359266935174901, -8.987542150724097567 ) ) ;
#7870=CARTESIAN_POINT ( 'NONE',  ( 1.564253033640318868, 44.28527310957349528, -24.39614062124454108 ) ) ;
#7871=CARTESIAN_POINT ( 'NONE',  ( 136.1360204305621266, -3.419521671106983309E-13, 35.03383547441296741 ) ) ;
#7878=CARTESIAN_POINT ( 'NONE',  ( -166.3490444787485387, 12.23457652163751419, 39.29840179234926723 ) ) ;
#7879=CARTESIAN_POINT ( 'NONE',  ( -3.524834090817713150, -17.92814044289628583, -43.28235980537089489 ) ) ;
#7880=CARTESIAN_POINT ( 'NONE',  ( -105.3755690713226727, -12.89780903124395550, -12.89780903124416511 ) ) ;
#7881=( BOUNDED_SURFACE ( )  B_SPLINE_SURFACE ( 3, 3, ( 
 ( #24240, #14121, #12258, #9865, #5610, #26114, #19, #14247, #9997, #1892, #22115, #19975, #16247, #21841, #21977, #19840, #18105, #22249, #1756, #17967, #10265, #26255, #7990, #16110, #3749, #24376, #22387, #2155, #4024, #12124 ),
 ( #23963, #11855, #3610, #20249, #10131, #4164, #2029, #6139, #20381, #1626, #9733, #13716, #18375, #17835, #154, #7722, #15833, #10931, #14637, #22774, #22516, #22905, #6526, #10665, #24905, #2547, #2692, #4555, #4683, #19042 ),
 ( #14775, #16771, #4294, #20640, #10525, #20777, #4418, #10392, #24773, #12652, #18503, #284, #10798, #6660, #12786, #4820, #2416, #16376, #18639, #18908, #6793, #18775, #558, #8527, #12512, #686, #14384, #14512, #6270, #8663 ),
 ( #16908, #22643, #12383, #20913, #8391, #20511, #16513, #422, #8796, #25040, #14905, #16644, #23045, #12923, #21039, #2822, #2283, #8258, #24510, #24639, #6396, #3321, #19541, #17037, #4949, #13055, #11545, #25299, #5446, #15292 ),
 ( #11302, #11421, #8928, #1327, #7423, #5313, #9308, #25172, #13424, #7302, #9432, #13300, #17539, #21547, #15538, #21300, #25677, #23666, #13547, #3075, #21675, #821, #15416, #5197, #6923, #21421, #15040, #19419, #17296, #23422 ),
 ( #3449, #23171, #3193, #1205, #17414, #1074, #7175, #11176, #9183, #19168, #952, #25554, #23542, #21173, #2946, #11056, #15172, #9060, #17165, #7057, #23297, #5074, #13179, #19291, #25428, #26076, #1587, #11676, #25806, #17664 ),
 ( #14451, #15928, #16070, #4483, #7812, #25941, #26216, #1855, #15665, #5697, #21937, #5837, #15797, #21800, #9827, #24061, #3573, #19801, #22578, #9958, #18065, #16577, #13802, #1456, #3713, #4357, #18574, #13941, #22076, #19934 ) ),
 .UNSPECIFIED., .T., .F., .F. ) 
 B_SPLINE_SURFACE_WITH_KNOTS ( ( 4, 3, 4 ),
 ( 4, 2, 2, 2, 2, 2, 2, 2, 2, 2, 2, 2, 2, 2, 4 ),
 ( 0.000000000000000000, 0.5000000000000000000, 1.000000000000000000 ),
 ( 0.000000000000000000, 0.1357259735107005372, 0.1651108541090157700, 0.1944957347073310028, 0.3598804999793158710, 0.3867117631979620773, 0.4135430264166082281, 0.5789277916885930964, 0.6062785021374117456, 0.6336292125862302838, 0.8508620842112317728, 0.8814014469398914198, 0.9119408096685510667, 0.9559704048342755334, 1.000000000000000000 ),
 .UNSPECIFIED. ) 
 GEOMETRIC_REPRESENTATION_ITEM ( )  RATIONAL_B_SPLINE_SURFACE ( (
 ( 1.000000000000000000, 1.000000000000000000, 1.000000000000000000, 1.000000000000000000, 1.000000000000000000, 1.000000000000000000, 1.000000000000000000, 1.000000000000000000, 1.000000000000000000, 1.000000000000000000, 1.000000000000000000, 1.000000000000000000, 1.000000000000000000, 1.000000000000000000, 1.000000000000000000, 1.000000000000000000, 1.000000000000000000, 1.000000000000000000, 1.000000000000000000, 1.000000000000000000, 1.000000000000000000, 1.000000000000000000, 1.000000000000000000, 1.000000000000000000, 1.000000000000000000, 1.000000000000000000, 1.000000000000000000, 1.000000000000000000, 1.000000000000000000, 1.000000000000000000),
 ( 0.3333333333333333703, 0.3333333333333333703, 0.3333333333333333703, 0.3333333333333333703, 0.3333333333333333703, 0.3333333333333333703, 0.3333333333333333703, 0.3333333333333333703, 0.3333333333333333703, 0.3333333333333333703, 0.3333333333333333703, 0.3333333333333333703, 0.3333333333333333703, 0.3333333333333333703, 0.3333333333333333703, 0.3333333333333333703, 0.3333333333333333703, 0.3333333333333333703, 0.3333333333333333703, 0.3333333333333333703, 0.3333333333333333703, 0.3333333333333333703, 0.3333333333333333703, 0.3333333333333333703, 0.3333333333333333703, 0.3333333333333333703, 0.3333333333333333703, 0.3333333333333333703, 0.3333333333333333703, 0.3333333333333333703),
 ( 0.3333333333333333703, 0.3333333333333333703, 0.3333333333333333703, 0.3333333333333333703, 0.3333333333333333703, 0.3333333333333333703, 0.3333333333333333703, 0.3333333333333333703, 0.3333333333333333703, 0.3333333333333333703, 0.3333333333333333703, 0.3333333333333333703, 0.3333333333333333703, 0.3333333333333333703, 0.3333333333333333703, 0.3333333333333333703, 0.3333333333333333703, 0.3333333333333333703, 0.3333333333333333703, 0.3333333333333333703, 0.3333333333333333703, 0.3333333333333333703, 0.3333333333333333703, 0.3333333333333333703, 0.3333333333333333703, 0.3333333333333333703, 0.3333333333333333703, 0.3333333333333333703, 0.3333333333333333703, 0.3333333333333333703),
 ( 1.000000000000000000, 1.000000000000000000, 1.000000000000000000, 1.000000000000000000, 1.000000000000000000, 1.000000000000000000, 1.000000000000000000, 1.000000000000000000, 1.000000000000000000, 1.000000000000000000, 1.000000000000000000, 1.000000000000000000, 1.000000000000000000, 1.000000000000000000, 1.000000000000000000, 1.000000000000000000, 1.000000000000000000, 1.000000000000000000, 1.000000000000000000, 1.000000000000000000, 1.000000000000000000, 1.000000000000000000, 1.000000000000000000, 1.000000000000000000, 1.000000000000000000, 1.000000000000000000, 1.000000000000000000, 1.000000000000000000, 1.000000000000000000, 1.000000000000000000),
 ( 0.3333333333333333703, 0.3333333333333333703, 0.3333333333333333703, 0.3333333333333333703, 0.3333333333333333703, 0.3333333333333333703, 0.3333333333333333703, 0.3333333333333333703, 0.3333333333333333703, 0.3333333333333333703, 0.3333333333333333703, 0.3333333333333333703, 0.3333333333333333703, 0.3333333333333333703, 0.3333333333333333703, 0.3333333333333333703, 0.3333333333333333703, 0.3333333333333333703, 0.3333333333333333703, 0.3333333333333333703, 0.3333333333333333703, 0.3333333333333333703, 0.3333333333333333703, 0.3333333333333333703, 0.3333333333333333703, 0.3333333333333333703, 0.3333333333333333703, 0.3333333333333333703, 0.3333333333333333703, 0.3333333333333333703),
 ( 0.3333333333333333703, 0.3333333333333333703, 0.3333333333333333703, 0.3333333333333333703, 0.3333333333333333703, 0.3333333333333333703, 0.3333333333333333703, 0.3333333333333333703, 0.3333333333333333703, 0.3333333333333333703, 0.3333333333333333703, 0.3333333333333333703, 0.3333333333333333703, 0.3333333333333333703, 0.3333333333333333703, 0.3333333333333333703, 0.3333333333333333703, 0.3333333333333333703, 0.3333333333333333703, 0.3333333333333333703, 0.3333333333333333703, 0.3333333333333333703, 0.3333333333333333703, 0.3333333333333333703, 0.3333333333333333703, 0.3333333333333333703, 0.3333333333333333703, 0.3333333333333333703, 0.3333333333333333703, 0.3333333333333333703),
 ( 1.000000000000000000, 1.000000000000000000, 1.000000000000000000, 1.000000000000000000, 1.000000000000000000, 1.000000000000000000, 1.000000000000000000, 1.000000000000000000, 1.000000000000000000, 1.000000000000000000, 1.000000000000000000, 1.000000000000000000, 1.000000000000000000, 1.000000000000000000, 1.000000000000000000, 1.000000000000000000, 1.000000000000000000, 1.000000000000000000, 1.000000000000000000, 1.000000000000000000, 1.000000000000000000, 1.000000000000000000, 1.000000000000000000, 1.000000000000000000, 1.000000000000000000, 1.000000000000000000, 1.000000000000000000, 1.000000000000000000, 1.000000000000000000, 1.000000000000000000) ) ) 
 REPRESENTATION_ITEM ( '' )  SURFACE ( )  );
#7882=CARTESIAN_POINT ( 'NONE',  ( -200.0000000000000284, 15.65821854886104880, 47.96425349429443941 ) ) ;
#7883=CARTESIAN_POINT ( 'NONE',  ( -30.26275506840322649, -29.48230279907810925, 29.48230279907778950 ) ) ;
#7884=CARTESIAN_POINT ( 'NONE',  ( 146.6084372240433993, -3.357462877844280890E-13, 34.62501878078305850 ) ) ;
#7885=CARTESIAN_POINT ( 'NONE',  ( 91.82158438592158234, 12.16597498397756993, 12.16597498397776356 ) ) ;
#7886=CARTESIAN_POINT ( 'NONE',  ( 151.7948205124836534, -6.767089262349006873, 40.00000000000002132 ) ) ;
#7889=CARTESIAN_POINT ( 'NONE',  ( 130.8568914410475088, -5.949712681206664300, -40.00000000000002132 ) ) ;
#7890=CARTESIAN_POINT ( 'NONE',  ( -114.6336192494810575, 11.25681893587175608, 18.90533938101397737 ) ) ;
#7892=CARTESIAN_POINT ( 'NONE',  ( 163.1118516004056573, 40.00000000000017764, -12.73709011382432976 ) ) ;
#7893=CARTESIAN_POINT ( 'NONE',  ( -100.7734535825088358, -16.03295912088706743, -16.03295912088710296 ) ) ;
#7894=CARTESIAN_POINT ( 'NONE',  ( 19.06497207195980792, 14.19242893257840699, -40.00000000000002132 ) ) ;
#7895=ORIENTED_EDGE ( 'NONE', *, *, #3211, .T. ) ;
#7896=CARTESIAN_POINT ( 'NONE',  ( 23.38399212876581146, -42.85408588822665621, 23.33762193384644590 ) ) ;
#7897=CIRCLE ( 'NONE', #4548, 30.00000000000003908 ) ;
#7899=CARTESIAN_POINT ( 'NONE',  ( 19.06497207195979726, 38.31983398719629719, -18.24870850772750686 ) ) ;
#7900=CARTESIAN_POINT ( 'NONE',  ( 130.8568914410475088, -40.00000000000001421, 5.949712681206549725 ) ) ;
#7901=CARTESIAN_POINT ( 'NONE',  ( -135.8532207217289738, 21.81201906317729566, 34.75652343174635917 ) ) ;
#7902=CARTESIAN_POINT ( 'NONE',  ( -100.7734535825088358, -22.67402823373193499, 0.000000000000000000 ) ) ;
#7903=CARTESIAN_POINT ( 'NONE',  ( 130.8568914410475088, 5.949712681206719367, -40.00000000000002132 ) ) ;
#7907=CARTESIAN_POINT ( 'NONE',  ( -105.3755690713226727, 12.89780903124418998, -12.89780903124389155 ) ) ;
#7908=CARTESIAN_POINT ( 'NONE',  ( 200.0000000000000000, -42.42640687119290988, 14.14213562373064903 ) ) ;
#7910=CARTESIAN_POINT ( 'NONE',  ( 199.9999999999999432, 14.14213562373113398, -14.14213562373094923 ) ) ;
#7911=CARTESIAN_POINT ( 'NONE',  ( -86.86493150571119770, 19.60045294882776901, -8.366608963953506617 ) ) ;
#7912=CARTESIAN_POINT ( 'NONE',  ( -259.2033419157646676, -49.83842185052040463, 6.730120644403092101 ) ) ;
#7914=CARTESIAN_POINT ( 'NONE',  ( -30.26275506840324070, 1.198031551616030033, -1.198031551616006496 ) ) ;
#7915=CARTESIAN_POINT ( 'NONE',  ( 151.7948205124835681, -4.785054706298153882, -51.78348778862540058 ) ) ;
#7916=B_SPLINE_CURVE_WITH_KNOTS ( 'NONE', 3,
 ( #14009, #24265, #14275, #2307, #10021, #10415 ),
 .UNSPECIFIED., .F., .F.,
 ( 4, 2, 4 ),
 ( 0.000000000000000000, 0.004167651203541847087, 0.008335302407083694173 ),
 .UNSPECIFIED. ) ;
#7919=CARTESIAN_POINT ( 'NONE',  ( -259.2033419157646676, -40.00000000000003553, -9.517827891722768996 ) ) ;
#7920=CARTESIAN_POINT ( 'NONE',  ( 192.4448373802101173, 42.42640687122070631, 14.14213562370331623 ) ) ;
#7921=CARTESIAN_POINT ( 'NONE',  ( -30.26275506840324070, -1.198031551616016266, -1.198031551616031587 ) ) ;
#7922=CARTESIAN_POINT ( 'NONE',  ( -4.201409602818262812, 46.93439176590655393, -13.81669219312473906 ) ) ;
#7923=CARTESIAN_POINT ( 'NONE',  ( 170.2234770963711128, -24.55285855007184281, 40.00000000000002132 ) ) ;
#7924=ORIENTED_EDGE ( 'NONE', *, *, #20019, .F. ) ;
#7925=CARTESIAN_POINT ( 'NONE',  ( -30.26275506840324070, 1.198031551616013601, 1.198031551616023371 ) ) ;
#7926=AXIS2_PLACEMENT_3D ( 'NONE', #15349, #11227, #9104 ) ;
#7927=CARTESIAN_POINT ( 'NONE',  ( 29.55251326303118375, 40.53812068415412995, 16.79143938049396567 ) ) ;
#7928=B_SPLINE_CURVE_WITH_KNOTS ( 'NONE', 3,
 ( #23551, #23178, #19550, #7184, #2954, #11064 ),
 .UNSPECIFIED., .F., .F.,
 ( 4, 2, 4 ),
 ( -5.998616615737899812E-08, 0.005994953700759804265, 0.01198996738768576611 ),
 .UNSPECIFIED. ) ;
#7930=CARTESIAN_POINT ( 'NONE',  ( -259.2033419157646676, -9.517827891722680178, 0.000000000000000000 ) ) ;
#7931=ORIENTED_EDGE ( 'NONE', *, *, #3619, .T. ) ;
#7934=CARTESIAN_POINT ( 'NONE',  ( 11.71430589694271340, -14.17293196763458596, 49.28686712666256398 ) ) ;
#7935=CARTESIAN_POINT ( 'NONE',  ( 23.84827734669562460, 23.24317830786175421, -42.71123329578252026 ) ) ;
#7938=CARTESIAN_POINT ( 'NONE',  ( -187.8779108535583191, -17.82355704115829553, 43.02987313850725570 ) ) ;
#7939=CARTESIAN_POINT ( 'NONE',  ( 0.2972598230769907257, 66.70487387989869887, -10.13633138497392494 ) ) ;
#7940=CARTESIAN_POINT ( 'NONE',  ( -87.13361725327072804, 8.813415818526478339E-15, 21.49321519333429009 ) ) ;
#7941=CARTESIAN_POINT ( 'NONE',  ( -187.7699188115598474, 13.79076593539120310, -46.80708926515250567 ) ) ;
#7942=CARTESIAN_POINT ( 'NONE',  ( 199.9999999999999432, -14.14213562373115884, 14.14213562373085153 ) ) ;
#7943=CARTESIAN_POINT ( 'NONE',  ( 98.29820294267528880, -14.14213562373450017, -14.14213562373441668 ) ) ;
#7944=CARTESIAN_POINT ( 'NONE',  ( -280.0000000000000568, -20.00000000000006395, -40.00000000000002132 ) ) ;
#7945=CARTESIAN_POINT ( 'NONE',  ( -162.0762913951020892, 1.694272876828294194, 0.000000000000000000 ) ) ;
#7946=CARTESIAN_POINT ( 'NONE',  ( -162.0762913951020892, -39.99999999999961631, -41.69427287692722928 ) ) ;
#7947=CARTESIAN_POINT ( 'NONE',  ( -280.0000000000000568, 42.42640687119285303, -14.14213562373088351 ) ) ;
#7948=CARTESIAN_POINT ( 'NONE',  ( 190.0000000000000000, -69.99999999999987210, 8.572527594031463526E-15 ) ) ;
#7949=CARTESIAN_POINT ( 'NONE',  ( -135.8532207217289738, 34.75652343174625258, -21.81201906317744132 ) ) ;
#7951=CARTESIAN_POINT ( 'NONE',  ( -280.0000000000000568, -42.42640687119295251, 14.14213562373088351 ) ) ;
#7957=CARTESIAN_POINT ( 'NONE',  ( 91.82158438592156813, -16.11829626348402655, -40.45024623143966380 ) ) ;
#7958=CARTESIAN_POINT ( 'NONE',  ( 25.88393124173831339, -45.90075965690534332, -13.61573025393274072 ) ) ;
#7959=ORIENTED_EDGE ( 'NONE', *, *, #26226, .T. ) ;
#7960=CARTESIAN_POINT ( 'NONE',  ( -238.4067589809705794, 0.9644942799825386714, 0.000000000000000000 ) ) ;
#7961=CARTESIAN_POINT ( 'NONE',  ( -93.01741312762746361, -20.50009083233623386, 8.946232117507843640 ) ) ;
#7962=ORIENTED_EDGE ( 'NONE', *, *, #6706, .F. ) ;
#7965=CARTESIAN_POINT ( 'NONE',  ( -162.0762913951020892, 1.198031840385716418, 1.198031840385750169 ) ) ;
#7966=CARTESIAN_POINT ( 'NONE',  ( -188.2957210513884831, -46.98905903629623282, -13.82790368522444169 ) ) ;
#7967=CARTESIAN_POINT ( 'NONE',  ( 170.2234770963711128, -40.00000000000004263, 15.44714144992801685 ) ) ;
#7968=CARTESIAN_POINT ( 'NONE',  ( 200.0000000000000000, -20.00000000000006750, 40.00000000000002132 ) ) ;
#7972=CARTESIAN_POINT ( 'NONE',  ( -135.8532207217289738, -40.00000000000014921, 30.84685318188631697 ) ) ;
#7973=CARTESIAN_POINT ( 'NONE',  ( 136.1360204305621266, 5.219216885335291329E-15, 4.966164525587064560 ) ) ;
#7974=CARTESIAN_POINT ( 'NONE',  ( -259.2033419157646676, -1.473088368616265084E-13, 9.517827891722632216 ) ) ;
#7975=CARTESIAN_POINT ( 'NONE',  ( -110.0947178154763719, -15.96121929952994378, 12.38433105677422574 ) ) ;
#7976=CARTESIAN_POINT ( 'NONE',  ( 0.2972598230770153171, -66.70487387989861361, 10.13633138497438324 ) ) ;
#7977=CARTESIAN_POINT ( 'NONE',  ( -30.26275506840324425, -1.694272468446265334, -40.00000000000002132 ) ) ;
#7978=CARTESIAN_POINT ( 'NONE',  ( -162.0762913951021176, -29.48230308784755493, -27.08623940707632372 ) ) ;
#7979=CARTESIAN_POINT ( 'NONE',  ( -103.9474983245025044, -8.577167319634718012, 19.92928099173747114 ) ) ;
#7980=CARTESIAN_POINT ( 'NONE',  ( 21.15737826136109589, -47.57244852138556013, 13.91467835516659513 ) ) ;
#7981=CARTESIAN_POINT ( 'NONE',  ( -198.0356074513804572, 40.00000000000014921, -15.37879056873028816 ) ) ;
#7982=CARTESIAN_POINT ( 'NONE',  ( -280.0000000000000000, 1.839446121267387017E-14, -20.00000000000001421 ) ) ;
#7983=CARTESIAN_POINT ( 'NONE',  ( -198.0356074513804572, 67.44298959253333692, 10.87444709760969452 ) ) ;
#7984=CARTESIAN_POINT ( 'NONE',  ( -238.4067589809705794, -0.6820004457913585449, -0.6820004457913265705 ) ) ;
#7985=CARTESIAN_POINT ( 'NONE',  ( -188.8532066752252376, -17.93248812771238221, -43.29285604501852447 ) ) ;
#7986=CARTESIAN_POINT ( 'NONE',  ( -135.8532207217289738, 6.472252184284186249, -6.472252184284142729 ) ) ;
#7988=CARTESIAN_POINT ( 'NONE',  ( 19.06497207195980792, 10.03556273973447155, -10.03556273973422286 ) ) ;
#7990=CARTESIAN_POINT ( 'NONE',  ( 136.1360204305621266, 35.03383547441298873, 0.000000000000000000 ) ) ;
#7991=EDGE_CURVE ( 'NONE', #2026, #15674, #12559, .T. ) ;
#7993=CARTESIAN_POINT ( 'NONE',  ( -208.1127848780264742, 10.60833733268383483, -67.17687982760675425 ) ) ;
#7994=CARTESIAN_POINT ( 'NONE',  ( 0.000000000000000000, 0.000000000000000000, 0.000000000000000000 ) ) ;
#7996=ORIENTED_EDGE ( 'NONE', *, *, #3959, .T. ) ;
#7998=CARTESIAN_POINT ( 'NONE',  ( 73.43438336400350863, -9.843172575685745329, -28.18283891303412858 ) ) ;
#7999=EDGE_CURVE ( 'NONE', #1453, #8799, #15107, .T. ) ;
#8000=CARTESIAN_POINT ( 'NONE',  ( -4.915070467882389771, 23.27857837408975783, 42.74707758271485858 ) ) ;
#8003=CARTESIAN_POINT ( 'NONE',  ( 184.8905102610680444, -20.92133201514440799, -40.00000000000002132 ) ) ;
#8005=CARTESIAN_POINT ( 'NONE',  ( -114.6375327213287818, 5.510795915284336211, 21.34761811097288486 ) ) ;
#8008=CARTESIAN_POINT ( 'NONE',  ( 73.43438336401153776, 28.18283891303104483, -9.843172575685235515 ) ) ;
#8009=CIRCLE ( 'NONE', #16080, 15.00000000000000000 ) ;
#8010=CARTESIAN_POINT ( 'NONE',  ( -89.91498783730708055, -8.733585467785214718, -20.17141720495975576 ) ) ;
#8011=CARTESIAN_POINT ( 'NONE',  ( -198.0356074513804572, 40.00000000000014921, -15.37879056873028816 ) ) ;
#8013=CARTESIAN_POINT ( 'NONE',  ( -77.55640685876512919, -22.13135000837101529, -2.449293598294708880E-15 ) ) ;
#8016=DIRECTION ( 'NONE',  ( -0.2259624731720487056, 0.9741360072997872210, 0.000000000000000000 ) ) ;
#8017=CARTESIAN_POINT ( 'NONE',  ( -4.439300432586843037, -13.79990882516970352, -46.85201324744510742 ) ) ;
#8018=CARTESIAN_POINT ( 'NONE',  ( -208.1127848780264742, -38.89260858015704514, -38.89260858015768463 ) ) ;
#8019=CARTESIAN_POINT ( 'NONE',  ( -4.039451493210485467, -13.82811171175474207, 46.99046209229799587 ) ) ;
#8020=CARTESIAN_POINT ( 'NONE',  ( -56.48582580120558561, -50.09629031063963112, -6.472252184284449150 ) ) ;
#8021=CARTESIAN_POINT ( 'NONE',  ( 91.82158438592158234, -1.633484621919921769E-13, 17.20528682183300262 ) ) ;
#8022=CARTESIAN_POINT ( 'NONE',  ( 57.59792236341147031, 1.722363176415040886, 1.722363176415060426 ) ) ;
#8023=CARTESIAN_POINT ( 'NONE',  ( -162.0762913951020607, -41.69427287692683848, 40.00000000000002132 ) ) ;
#8024=CARTESIAN_POINT ( 'NONE',  ( 160.7895100361087657, 20.14405787076037413, -20.14405787076013254 ) ) ;
#8025=CARTESIAN_POINT ( 'NONE',  ( 151.7948205124836250, -6.767089262349004208, -2.449293598294708485E-15 ) ) ;
#8026=CARTESIAN_POINT ( 'NONE',  ( -114.4954523681517458, 9.313731507797939457, 19.81404414622909016 ) ) ;
#8027=CARTESIAN_POINT ( 'NONE',  ( -56.48582580120559982, 40.00000000000034106, -30.84685318188602210 ) ) ;
#8028=CARTESIAN_POINT ( 'NONE',  ( -105.3755690713226727, -15.38646221621786481, -15.38646221621789856 ) ) ;
#8029=CARTESIAN_POINT ( 'NONE',  ( 57.59792236341147031, -2.435789363418150444, 0.000000000000000000 ) ) ;
#8031=VERTEX_POINT ( 'NONE', #1272 ) ;
#8032=CARTESIAN_POINT ( 'NONE',  ( 0.2972598230769930017, 14.33493731733933352, 40.00000000000002132 ) ) ;
#8034=CARTESIAN_POINT ( 'NONE',  ( -96.93773665438791909, -8.190703376740877673, -20.92028269119433403 ) ) ;
#8035=CARTESIAN_POINT ( 'NONE',  ( -105.3755690713226727, -8.549198663894545631E-14, 18.24025645688352881 ) ) ;
#8036=CARTESIAN_POINT ( 'NONE',  ( -259.2033419157646676, -6.730120644403663199, 6.730120644403451813 ) ) ;
#8038=CARTESIAN_POINT ( 'NONE',  ( -188.5332406156555010, -43.07394490460117709, -23.50029615581455644 ) ) ;
#8039=( BOUNDED_SURFACE ( )  B_SPLINE_SURFACE ( 3, 2, ( 
 ( #17122, #905, #3405 ),
 ( #11506, #7516, #15624 ),
 ( #7004, #15124, #23255 ),
 ( #21257, #1033, #9133 ),
 ( #14169, #16165, #5793 ),
 ( #1945, #11634, #17886 ),
 ( #25897, #15887, #13901 ),
 ( #13764, #22034, #15753 ),
 ( #3807, #11912, #18289 ),
 ( #21891, #20034, #1812 ),
 ( #9915, #24015, #1679 ),
 ( #23881, #18021, #8048 ),
 ( #11776, #26170, #16301 ),
 ( #10052, #7772, #8184 ),
 ( #9651, #12180, #3534 ),
 ( #24154, #22302, #7911 ) ),
 .UNSPECIFIED., .F., .F., .F. ) 
 B_SPLINE_SURFACE_WITH_KNOTS ( ( 4, 2, 2, 2, 2, 2, 2, 4 ),
 ( 3, 3 ),
 ( 0.04143342415445357141, 0.04844559399082577766, 0.05195167890901188079, 0.05545776382719797698, 0.06246993366357017630, 0.06422297612266322786, 0.06597601858175627942, 0.06948210349994238255 ),
 ( 0.000000000000000000, 1.000000000000000000 ),
 .UNSPECIFIED. ) 
 GEOMETRIC_REPRESENTATION_ITEM ( )  RATIONAL_B_SPLINE_SURFACE ( (
 ( 1.000000000000000000, 0.9541700779530604137, 1.000000000000000000),
 ( 1.000000000000000000, 0.9520168980299437145, 1.000000000000000000),
 ( 1.000000000000000000, 0.9503263051600997491, 1.000000000000000000),
 ( 1.000000000000000000, 0.9485964699097189090, 1.000000000000000000),
 ( 1.000000000000000000, 0.9481599523400192631, 1.000000000000000000),
 ( 1.000000000000000000, 0.9475783919167657388, 1.000000000000000000),
 ( 1.000000000000000000, 0.9474332805886016562, 1.000000000000000000),
 ( 1.000000000000000000, 0.9474385816642081348, 1.000000000000000000),
 ( 1.000000000000000000, 0.9480200071122316663, 1.000000000000000000),
 ( 1.000000000000000000, 0.9494436219491265705, 1.000000000000000000),
 ( 1.000000000000000000, 0.9497633688929369988, 1.000000000000000000),
 ( 1.000000000000000000, 0.9504729676351979517, 1.000000000000000000),
 ( 1.000000000000000000, 0.9508638236297854984, 1.000000000000000000),
 ( 1.000000000000000000, 0.9521268919818318688, 1.000000000000000000),
 ( 1.000000000000000000, 0.9530924015899474577, 1.000000000000000000),
 ( 1.000000000000000000, 0.9541700779530456478, 1.000000000000000000) ) ) 
 REPRESENTATION_ITEM ( '' )  SURFACE ( )  );
#8041=DIRECTION ( 'NONE',  ( 0.01051738792037396585, -0.9307051272719674140, 0.3656191332808000904 ) ) ;
#8043=UNCERTAINTY_MEASURE_WITH_UNIT (LENGTH_MEASURE( 1.000000000000000082E-05 ), #13101, 'distance_accuracy_value', 'NONE');
#8045=CARTESIAN_POINT ( 'NONE',  ( 136.1360204305621266, 3.511608612530757068, -3.511608612530642937 ) ) ;
#8046=CARTESIAN_POINT ( 'NONE',  ( -30.26275506840322294, -57.76657404653985139, -1.198031551616531853 ) ) ;
#8047=CARTESIAN_POINT ( 'NONE',  ( -114.4008591471760923, 20.10521893440135699, 8.440277345772122075 ) ) ;
#8048=CARTESIAN_POINT ( 'NONE',  ( -87.01506749150125586, 18.46228859042466652, -10.84947533657426000 ) ) ;
#8049=CARTESIAN_POINT ( 'NONE',  ( -213.1075012329537230, -66.26714140136188291, -9.698598906438677503 ) ) ;
#8051=CARTESIAN_POINT ( 'NONE',  ( 200.0000000000000000, -14.14213562373046784, -42.42640687119298804 ) ) ;
#8052=CARTESIAN_POINT ( 'NONE',  ( -208.1127848780264742, -67.17687982763172272, 10.60833733270744617 ) ) ;
#8053=CARTESIAN_POINT ( 'NONE',  ( -114.4364955367327497, -20.04994829327637262, -8.644468109209869411 ) ) ;
#8056=CARTESIAN_POINT ( 'NONE',  ( 136.1360204305621551, 40.00000000000002842, 4.966164525587208445 ) ) ;
#8058=CARTESIAN_POINT ( 'NONE',  ( 22.17571259162450303, 43.20787961118990950, -23.59965736304651784 ) ) ;
#8059=CARTESIAN_POINT ( 'NONE',  ( 4.995406935893289102, 55.24977328856464709, -40.00000000000002132 ) ) ;
#8060=ORIENTED_EDGE ( 'NONE', *, *, #4040, .T. ) ;
#8061=CARTESIAN_POINT ( 'NONE',  ( -192.9588430854689989, 14.46834944099965981, 0.000000000000000000 ) ) ;
#8062=CARTESIAN_POINT ( 'NONE',  ( -77.90255099906765679, -20.29001641120677846, 8.064892378658099048 ) ) ;
#8065=CARTESIAN_POINT ( 'NONE',  ( -192.6562840317106691, -44.11756026581168300, 18.27409180090121410 ) ) ;
#8068=CARTESIAN_POINT ( 'NONE',  ( 21.80484139881139782, -17.98806631652405486, 43.42703366220045780 ) ) ;
#8069=CARTESIAN_POINT ( 'NONE',  ( 23.72853009152708736, 13.77482773664671711, -46.68009952139264840 ) ) ;
#8071=CARTESIAN_POINT ( 'NONE',  ( 23.37394308801977871, -13.80096434448300613, 46.80823611210190904 ) ) ;
#8074=CARTESIAN_POINT ( 'NONE',  ( 146.6084372240433993, 3.800685668858732935, -3.800685668858610367 ) ) ;
#8075=CARTESIAN_POINT ( 'NONE',  ( 19.06497207195981503, -14.19242893257840166, 0.000000000000000000 ) ) ;
#8076=CARTESIAN_POINT ( 'NONE',  ( -194.4222169614336622, 24.44978956118432123, -44.35789444896231259 ) ) ;
#8077=CARTESIAN_POINT ( 'NONE',  ( 19.06497207195980792, 10.03556273973447155, -10.03556273973422286 ) ) ;
#8078=FACE_OUTER_BOUND ( 'NONE', #8667, .T. ) ;
#8079=EDGE_CURVE ( 'NONE', #16477, #15766, #23515, .T. ) ;
#8080=CARTESIAN_POINT ( 'NONE',  ( -56.48582580120557850, -30.84685318188645198, -2.449293598294708485E-15 ) ) ;
#8081=CARTESIAN_POINT ( 'NONE',  ( 57.59792236341147031, 37.56421063658187620, 40.00000000000002132 ) ) ;
#8082=CARTESIAN_POINT ( 'NONE',  ( 170.2234770963711128, 1.955190573858485757E-13, -15.44714144992816074 ) ) ;
#8083=CARTESIAN_POINT ( 'NONE',  ( 184.8905102610680444, -14.79361573936389540, 41.77492675555996016 ) ) ;
#8084=CARTESIAN_POINT ( 'NONE',  ( 192.4448373802100889, -1.741373372144848397E-13, 20.00000000003942091 ) ) ;
#8085=CARTESIAN_POINT ( 'NONE',  ( 0.2972598230769976091, -10.13633138497465147, -10.13633138497482733 ) ) ;
#8087=FACE_OUTER_BOUND ( 'NONE', #21679, .T. ) ;
#8088=CARTESIAN_POINT ( 'NONE',  ( -97.73860346104329722, -8.987542150717732881, 20.56359266935457342 ) ) ;
#8091=ORIENTED_EDGE ( 'NONE', *, *, #10586, .F. ) ;
#8092=CARTESIAN_POINT ( 'NONE',  ( -213.1075012329537230, -66.26714140138676612, 9.698598906462487790 ) ) ;
#8093=CARTESIAN_POINT ( 'NONE',  ( 23.41418334855299221, -42.84479974151761184, -23.33148157649304366 ) ) ;
#8095=CARTESIAN_POINT ( 'NONE',  ( 151.7948205124836534, 6.767089262349062828, -40.00000000000002132 ) ) ;
#8096=CARTESIAN_POINT ( 'NONE',  ( -100.0968563617800271, -20.41799937591574832, 8.893120081479189309 ) ) ;
#8098=VERTEX_POINT ( 'NONE', #7126 ) ;
#8101=CARTESIAN_POINT ( 'NONE',  ( -100.7734535825088500, 12.25131212657490209, -44.31723036834897300 ) ) ;
#8102=CARTESIAN_POINT ( 'NONE',  ( -188.8384220655415788, -43.28887647197276323, -17.93083973458484692 ) ) ;
#8103=CARTESIAN_POINT ( 'NONE',  ( -91.56559293963834989, -39.99999999999995737, -22.67402823373205933 ) ) ;
#8104=CARTESIAN_POINT ( 'NONE',  ( -259.2033419157646676, -9.517827891722680178, 40.00000000000002132 ) ) ;
#8110=CARTESIAN_POINT ( 'NONE',  ( -56.48582580120559271, 2.158176344243877536E-14, -9.153146818113587102 ) ) ;
#8111=CARTESIAN_POINT ( 'NONE',  ( -192.9588430854689989, -2.280704836619014309E-13, 54.46834944099972375 ) ) ;
#8113=CARTESIAN_POINT ( 'NONE',  ( 57.59792236341149163, -39.99999999999961631, -37.56421063658228832 ) ) ;
#8114=CARTESIAN_POINT ( 'NONE',  ( -280.0000000000000568, 40.00000000000004263, -19.99999999999987210 ) ) ;
#8116=CARTESIAN_POINT ( 'NONE',  ( 57.59792236341148453, -54.84617931850877426, -1.722363176415331099 ) ) ;
#8117=CARTESIAN_POINT ( 'NONE',  ( -135.8532207217289738, 9.153146818113548022, -40.00000000000002132 ) ) ;
#8118=CARTESIAN_POINT ( 'NONE',  ( 0.2972598230770153171, -66.70487387989861361, 10.13633138497438324 ) ) ;
#8119=CARTESIAN_POINT ( 'NONE',  ( 200.0000000000000000, 40.00000000000006395, 0.000000000000000000 ) ) ;
#8120=CARTESIAN_POINT ( 'NONE',  ( 3.854699808470075428, -48.95177852071786617, 14.12217777258779172 ) ) ;
#8121=CARTESIAN_POINT ( 'NONE',  ( -91.56559293963834989, -2.543181659092656077E-13, 22.67402823373191723 ) ) ;
#8122=CARTESIAN_POINT ( 'NONE',  ( 151.7948205124836250, 1.807796684091926154E-15, 6.767089262349031742 ) ) ;
#8123=CARTESIAN_POINT ( 'NONE',  ( -56.48582580120559982, 50.09629031063966664, -6.472252184284094767 ) ) ;
#8124=CARTESIAN_POINT ( 'NONE',  ( 4.995406935893293543, -10.78321810388990265, -10.78321810389009272 ) ) ;
#8125=CARTESIAN_POINT ( 'NONE',  ( -192.1964066537693441, -24.16259023441511644, -43.96877160660515216 ) ) ;
#8126=CARTESIAN_POINT ( 'NONE',  ( -192.9588430854690273, -38.51493924976932703, -18.05360324515463688 ) ) ;
#8128=CARTESIAN_POINT ( 'NONE',  ( 184.8905102610680444, -43.07788698682556827, -13.49065550809859104 ) ) ;
#8131=CARTESIAN_POINT ( 'NONE',  ( -87.13361725327074225, 15.19799821270847850, -15.19799821270833284 ) ) ;
#8132=CARTESIAN_POINT ( 'NONE',  ( -280.0000000000000568, -14.14213562373049449, -42.42640687119305198 ) ) ;
#8133=CARTESIAN_POINT ( 'NONE',  ( -87.08748155317879025, 3.397954955031054158, 21.19318107435227816 ) ) ;
#8137=CARTESIAN_POINT ( 'NONE',  ( 18.90082831370061101, -24.18116416851801276, 43.99399836018049825 ) ) ;
#8138=CARTESIAN_POINT ( 'NONE',  ( -3.406542234096830768, 17.94112998239669565, 43.31371932780069045 ) ) ;
#8139=ORIENTED_EDGE ( 'NONE', *, *, #17195, .F. ) ;
#8141=CARTESIAN_POINT ( 'NONE',  ( -192.9588430854689989, 14.46834944099965981, 0.000000000000000000 ) ) ;
#8146=CARTESIAN_POINT ( 'NONE',  ( -4.039451493210501454, 43.00522595894040734, -23.44932283416630270 ) ) ;
#8147=CARTESIAN_POINT ( 'NONE',  ( -105.3755690713226727, -2.472783935621397949E-13, 21.75974354311649961 ) ) ;
#8153=CARTESIAN_POINT ( 'NONE',  ( -192.4602856790872067, 43.06412164779830221, 17.83774323820395935 ) ) ;
#8154=CARTESIAN_POINT ( 'NONE',  ( 12.77879914700383601, -18.55776024548864100, -44.80239647190805385 ) ) ;
#8155=CARTESIAN_POINT ( 'NONE',  ( 151.7948205124836250, -4.785054706301600902, -4.785054706301715477 ) ) ;
#8156=B_SPLINE_CURVE_WITH_KNOTS ( 'NONE', 3,
 ( #23217, #9234, #13102, #21223, #11224, #11100, #2600, #998, #8845, #9101, #17210, #12841, #21350, #25348, #7105, #19340 ),
 .UNSPECIFIED., .F., .F.,
 ( 4, 2, 2, 2, 2, 2, 2, 4 ),
 ( 0.0003146141176185928779, 0.002410294611460639825, 0.003458134858381662919, 0.004505975105302687314, 0.008697336092986771017, 0.01079301658682881374, 0.01288869708067085298, 0.01708005806835492801 ),
 .UNSPECIFIED. ) ;
#8157=CARTESIAN_POINT ( 'NONE',  ( -114.6380801921473136, 5.502540229729388166, -21.35054024078830182 ) ) ;
#8158=CARTESIAN_POINT ( 'NONE',  ( -135.8532207217289738, -50.09629031063965243, -6.472252184284438492 ) ) ;
#8160=CARTESIAN_POINT ( 'NONE',  ( -86.96347745069644475, 15.38646221621772092, 15.38646221621800336 ) ) ;
#8161=CARTESIAN_POINT ( 'NONE',  ( 14.38125909742182884, -55.17850393972636169, -2.449293598294708485E-15 ) ) ;
#8162=EDGE_CURVE ( 'NONE', #11812, #7311, #10369, .T. ) ;
#8163=CARTESIAN_POINT ( 'NONE',  ( 98.29820294267436509, 14.14213562374297695, -14.14213562372651189 ) ) ;
#8164=CARTESIAN_POINT ( 'NONE',  ( -30.26275506840322649, -41.69427246844630019, -2.449293598294708485E-15 ) ) ;
#8165=CARTESIAN_POINT ( 'NONE',  ( -105.2066640875961667, 15.82458427809276635, 14.56001627727798997 ) ) ;
#8166=CARTESIAN_POINT ( 'NONE',  ( -259.2033419157646676, 2.741182173978444749E-13, -30.48217210827739621 ) ) ;
#8167=CARTESIAN_POINT ( 'NONE',  ( 151.7948205124836250, -23.49921654116339553, -23.49921654116350211 ) ) ;
#8168=CARTESIAN_POINT ( 'NONE',  ( 151.7948205124836534, -33.23291073765550863, -40.00000000000002132 ) ) ;
#8169=ORIENTED_EDGE ( 'NONE', *, *, #5638, .T. ) ;
#8171=CARTESIAN_POINT ( 'NONE',  ( 19.06497207195980792, 14.19242893257840699, 40.00000000000002132 ) ) ;
#8173=CARTESIAN_POINT ( 'NONE',  ( -162.0762913951021176, 39.99999999999998579, 1.694272876828463614 ) ) ;
#8174=CARTESIAN_POINT ( 'NONE',  ( -259.2033419157646676, 49.83842185052017015, 6.730120644404137487 ) ) ;
#8175=CARTESIAN_POINT ( 'NONE',  ( -259.2033419157646676, -9.517827891722680178, 40.00000000000002132 ) ) ;
#8177=CARTESIAN_POINT ( 'NONE',  ( -199.9999999999999432, -55.16984130226904171, -4.865628651906555469 ) ) ;
#8181=CARTESIAN_POINT ( 'NONE',  ( 0.2972598230769959993, 38.42060263243713081, -38.42060263243619289 ) ) ;
#8182=CARTESIAN_POINT ( 'NONE',  ( 4.995406935893312195, -67.35176059882525124, -10.78321810390210445 ) ) ;
#8183=CARTESIAN_POINT ( 'NONE',  ( -114.6510887843185458, 21.42093443206506365, 5.129768820901790427 ) ) ;
#8184=CARTESIAN_POINT ( 'NONE',  ( -86.94888381183984905, 19.08739374734031102, -9.627065680628259514 ) ) ;
#8185=CARTESIAN_POINT ( 'NONE',  ( -192.9588430854690273, -66.79921049721887982, -10.23066800229569040 ) ) ;
#8186=CARTESIAN_POINT ( 'NONE',  ( 14.38125909742180752, 10.73282306404735387, -10.73282306404708919 ) ) ;
#8187=CARTESIAN_POINT ( 'NONE',  ( -208.1127848780264742, -17.67593391476659548, 38.89260858015730804 ) ) ;
#8189=CARTESIAN_POINT ( 'NONE',  ( 130.8568914410475088, -4.207082182989324792, -52.36146031193423056 ) ) ;
#8192=CARTESIAN_POINT ( 'NONE',  ( 184.8905102610680444, -3.509827109981123710E-14, 19.07866798485558490 ) ) ;
#8194=CARTESIAN_POINT ( 'NONE',  ( 22.98934664983196896, 43.11412319250747771, -17.85845455615981692 ) ) ;
#8195=CARTESIAN_POINT ( 'NONE',  ( -208.1127848780264742, 55.00245453010919050, -40.00000000000002132 ) ) ;
#8197=CARTESIAN_POINT ( 'NONE',  ( 22.27781863241737881, -23.58928354682958428, -43.19367102561737681 ) ) ;
#8198=CARTESIAN_POINT ( 'NONE',  ( -24.51100708749678958, -37.39427017799431496, 15.48921386276234635 ) ) ;
#8199=CARTESIAN_POINT ( 'NONE',  ( -162.0762913951020892, 41.69427287682832173, 2.449293598294708485E-15 ) ) ;
#8202=CARTESIAN_POINT ( 'NONE',  ( 8.602182264134457412, -18.59145335917481390, 44.88373884392621704 ) ) ;
#8203=CARTESIAN_POINT ( 'NONE',  ( 7.112934525910308281, 18.57375239870144057, -44.84100494513564428 ) ) ;
#8205=CARTESIAN_POINT ( 'NONE',  ( -87.13361725327075646, -15.19799821270861706, 15.19799821270823159 ) ) ;
#8207=CARTESIAN_POINT ( 'NONE',  ( 14.38125909742181108, -5.035366881890652543E-14, 15.17850393972633682 ) ) ;
#8208=CARTESIAN_POINT ( 'NONE',  ( -280.0000000000000568, -14.14213562373049449, -42.42640687119305198 ) ) ;
#8209=CARTESIAN_POINT ( 'NONE',  ( -30.26275506840324070, -1.694272468446265112, 0.000000000000000000 ) ) ;
#8210=CARTESIAN_POINT ( 'NONE',  ( -188.6013942375886643, 23.51434495930266166, -43.09289976588191706 ) ) ;
#8211=CARTESIAN_POINT ( 'NONE',  ( -213.1075012329537230, 9.698598906450543566, -9.698598906450348167 ) ) ;
#8212=CARTESIAN_POINT ( 'NONE',  ( -280.0000000000000568, 14.14213562373038968, 42.42640687119305198 ) ) ;
#8213=CARTESIAN_POINT ( 'NONE',  ( -91.56559293963834989, -17.32597176626812896, -2.449293598294708485E-15 ) ) ;
#8214=CARTESIAN_POINT ( 'NONE',  ( -198.0356074513804572, 55.37879056874818673, -40.00000000000002132 ) ) ;
#8215=CARTESIAN_POINT ( 'NONE',  ( 57.59792236341148453, -40.00000000000003553, 2.435789363417741438 ) ) ;
#8216=CARTESIAN_POINT ( 'NONE',  ( 91.82158438592158234, -12.16597498400057198, 44.40256751092329779 ) ) ;
#8217=CARTESIAN_POINT ( 'NONE',  ( -96.94475454973485284, 20.92018922310817430, -8.190683501891818707 ) ) ;
#8218=CARTESIAN_POINT ( 'NONE',  ( -198.0356074513804572, -10.87444709758429262, -67.44298959250878056 ) ) ;
#8220=CARTESIAN_POINT ( 'NONE',  ( -259.2033419157646676, -6.730120644403570829, -6.730120644403545960 ) ) ;
#8221=CARTESIAN_POINT ( 'NONE',  ( -94.58360650938116976, 9.000712009833122806, 20.58386743644784289 ) ) ;
#8225=CARTESIAN_POINT ( 'NONE',  ( -280.0000000000000568, -42.42640687119285303, -14.14213562373118371 ) ) ;
#8226=CARTESIAN_POINT ( 'NONE',  ( 21.45050411889744879, -43.51299627225506583, -18.02367319544785218 ) ) ;
#8227=ORIENTED_EDGE ( 'NONE', *, *, #8079, .F. ) ;
#8228=CARTESIAN_POINT ( 'NONE',  ( 192.4448373802100889, -20.00000000003938538, 0.000000000000000000 ) ) ;
#8230=VERTEX_POINT ( 'NONE', #23999 ) ;
#8232=CARTESIAN_POINT ( 'NONE',  ( -105.2054292635175869, -15.19799821370180126, -15.19799821370278892 ) ) ;
#8233=CARTESIAN_POINT ( 'NONE',  ( -91.56559293963834989, -16.03295912088706388, -16.03295912088710651 ) ) ;
#8234=CARTESIAN_POINT ( 'NONE',  ( -188.9001659262688406, -43.30536839095038459, -17.93767091109504008 ) ) ;
#8235=CARTESIAN_POINT ( 'NONE',  ( 57.59792236341148453, -40.00000000000000000, -2.435789363418300546 ) ) ;
#8236=CARTESIAN_POINT ( 'NONE',  ( 19.06497207195980792, 14.19242893257840876, 0.000000000000000000 ) ) ;
#8239=CARTESIAN_POINT ( 'NONE',  ( 57.59792236341148453, -40.00000000000000000, -2.435789363418300546 ) ) ;
#8240=CARTESIAN_POINT ( 'NONE',  ( 0.2972598230770103767, -40.00000000000021316, 54.33493731733921805 ) ) ;
#8241=CARTESIAN_POINT ( 'NONE',  ( 4.995406935893283773, 39.99999999999997158, 15.24977328854846803 ) ) ;
#8242=CARTESIAN_POINT ( 'NONE',  ( -105.3755690713226869, 21.75974354311648540, -0.000000000000000000 ) ) ;
#8243=CARTESIAN_POINT ( 'NONE',  ( -213.1075012329536946, -37.98287015391263566, 37.98287015391218802 ) ) ;
#8244=CARTESIAN_POINT ( 'NONE',  ( -105.3755690713226585, 21.75974354311648185, -40.00000000000002132 ) ) ;
#8245=CARTESIAN_POINT ( 'NONE',  ( -30.26275506840322649, -29.48230279907810925, 29.48230279907778950 ) ) ;
#8247=ADVANCED_FACE ( 'NONE', ( #5644 ), #3793, .T. ) ;
#8249=CARTESIAN_POINT ( 'NONE',  ( -135.8532207217289738, 3.005970985514575011E-13, -30.84685318188645553 ) ) ;
#8250=CARTESIAN_POINT ( 'NONE',  ( -192.9588430854690273, -40.00000000000024158, 54.46834944101708231 ) ) ;
#8251=CARTESIAN_POINT ( 'NONE',  ( -208.1127848780264742, 38.89260858015732936, -17.67593391476642140 ) ) ;
#8252=CARTESIAN_POINT ( 'NONE',  ( -83.21262154144099554, -33.12752917118399409, 13.72187187061446956 ) ) ;
#8253=CARTESIAN_POINT ( 'NONE',  ( -192.9370379451175097, -24.26711011075247271, -44.11033005021999998 ) ) ;
#8254=CARTESIAN_POINT ( 'NONE',  ( -259.2033419157646676, -21.55415060305854524, 21.55415060305827524 ) ) ;
#8255=ORIENTED_EDGE ( 'NONE', *, *, #20606, .F. ) ;
#8256=CARTESIAN_POINT ( 'NONE',  ( -30.26275506840324070, -27.08623969584554558, -29.48230279907826912 ) ) ;
#8258=CARTESIAN_POINT ( 'NONE',  ( 14.38125909742182884, -55.17850393972636169, -2.449293598294708485E-15 ) ) ;
#8261=ORIENTED_EDGE ( 'NONE', *, *, #22837, .F. ) ;
#8262=ORIENTED_EDGE ( 'NONE', *, *, #21113, .F. ) ;
#8264=CARTESIAN_POINT ( 'NONE',  ( 4.990269915386278399, -24.74342916192414776, 44.75621547178053561 ) ) ;
#8265=CARTESIAN_POINT ( 'NONE',  ( -4.112199523541869794, 13.82298295336142324, 46.96527782736819034 ) ) ;
#8269=CARTESIAN_POINT ( 'NONE',  ( 146.6084372240433709, -34.62501878078303008, -40.00000000000002132 ) ) ;
#8271=CARTESIAN_POINT ( 'NONE',  ( -77.55640685876515761, -15.64922766773196905, -15.64922766773223195 ) ) ;
#8272=CARTESIAN_POINT ( 'NONE',  ( -259.2033419157646676, -6.730120644403570829, -6.730120644403545960 ) ) ;
#8273=CARTESIAN_POINT ( 'NONE',  ( -102.4309680866095817, -8.733065089892845023, -20.17061239845038756 ) ) ;
#8274=CARTESIAN_POINT ( 'NONE',  ( 91.82158438592158234, 2.580785920671402147E-13, -22.79471317813470321 ) ) ;
#8275=CARTESIAN_POINT ( 'NONE',  ( 192.4448373802101173, 39.99999999999985079, 20.00000000003984013 ) ) ;
#8276=CARTESIAN_POINT ( 'NONE',  ( -126.6834154282237250, 24.89646316986586783, -9.107266658309480789 ) ) ;
#8277=DIRECTION ( 'NONE',  ( 0.000000000000000000, 1.000000000000000000, 0.000000000000000000 ) ) ;
#8279=CARTESIAN_POINT ( 'NONE',  ( -188.8948201289223618, 17.93709820916097186, 43.30398576617481154 ) ) ;
#8280=CARTESIAN_POINT ( 'NONE',  ( 23.36462152323051811, -23.34178792078175491, -42.86003749000681751 ) ) ;
#8281=CARTESIAN_POINT ( 'NONE',  ( 136.1360204305621551, -31.79587985999279454, 24.77266263493094911 ) ) ;
#8282=CARTESIAN_POINT ( 'NONE',  ( -88.39148973765144035, 19.92926839984422926, -8.577159256668510423 ) ) ;
#8283=CARTESIAN_POINT ( 'NONE',  ( -213.1075012329536946, -37.98287015391263566, 37.98287015391218802 ) ) ;
#8286=CARTESIAN_POINT ( 'NONE',  ( -213.1075012329537230, -53.71589010950170717, 40.00000000000002132 ) ) ;
#8287=CARTESIAN_POINT ( 'NONE',  ( -192.9588430854689989, 10.23066800230756712, -10.23066800230735396 ) ) ;
#8288=CARTESIAN_POINT ( 'NONE',  ( -280.0000000000000568, -20.00000000000007105, 40.00000000000002132 ) ) ;
#8289=CARTESIAN_POINT ( 'NONE',  ( -105.2034101837812727, 14.35414403269573391, 16.06048591665815906 ) ) ;
#8290=CARTESIAN_POINT ( 'NONE',  ( 146.6084372240433709, 39.99999999999968026, 34.62501878078347772 ) ) ;
#8291=CARTESIAN_POINT ( 'NONE',  ( 184.8905102610680444, -14.79361573936379415, -14.79361573936387941 ) ) ;
#8292=CARTESIAN_POINT ( 'NONE',  ( 170.2234770963711128, -24.55285855007184281, -40.00000000000002132 ) ) ;
#8294=ADVANCED_FACE ( 'NONE', ( #22022 ), #11489, .T. ) ;
#8295=ORIENTED_EDGE ( 'NONE', *, *, #24365, .T. ) ;
#8297=CARTESIAN_POINT ( 'NONE',  ( -91.56559293963834989, -22.67402823373193499, 0.000000000000000000 ) ) ;
#8301=CARTESIAN_POINT ( 'NONE',  ( 57.59792236341147031, 54.84617931850878136, 1.722363176415705910 ) ) ;
#8302=CARTESIAN_POINT ( 'NONE',  ( -105.3901353553978737, -20.30436174851991282, -6.689050419658350677 ) ) ;
#8303=CARTESIAN_POINT ( 'NONE',  ( -114.4364955367327497, -8.064892380842218600, -20.29001642038850406 ) ) ;
#8309=CARTESIAN_POINT ( 'NONE',  ( 184.8905102610680444, 41.77492675555983936, 14.79361573936436081 ) ) ;
#8311=CARTESIAN_POINT ( 'NONE',  ( 151.7948205124836250, -4.785054706301600902, -4.785054706301715477 ) ) ;
#8313=CARTESIAN_POINT ( 'NONE',  ( -208.1127848780264742, 40.00000000000055422, -55.00245453014380814 ) ) ;
#8314=CARTESIAN_POINT ( 'NONE',  ( -91.56559293963836410, -12.25131212657524138, 44.31723036834888774 ) ) ;
#8315=CARTESIAN_POINT ( 'NONE',  ( -91.56559293963834989, -16.03295912088728414, 16.03295912088688269 ) ) ;
#8316=CARTESIAN_POINT ( 'NONE',  ( 151.7948205124836250, -23.49921654116339553, -23.49921654116350211 ) ) ;
#8317=CARTESIAN_POINT ( 'NONE',  ( 192.4448373802101173, -14.14213562370283128, -42.42640687122081999 ) ) ;
#8320=CARTESIAN_POINT ( 'NONE',  ( -162.0762913951020892, -1.777970010055771463E-13, 41.69427287682835015 ) ) ;
#8322=AXIS2_PLACEMENT_3D ( 'NONE', #3838, #4246, #6222 ) ;
#8323=CARTESIAN_POINT ( 'NONE',  ( 23.36462152323054653, 42.86003749000685303, -23.34178792078203912 ) ) ;
#8324=CARTESIAN_POINT ( 'NONE',  ( -105.3755690713226727, 18.24025645688350750, 2.449293598294708485E-15 ) ) ;
#8325=CARTESIAN_POINT ( 'NONE',  ( 4.995406935893288214, 15.24977328854832770, 0.000000000000000000 ) ) ;
#8327=CARTESIAN_POINT ( 'NONE',  ( -3.449394506061680854, -43.30266483527573484, 17.93655106166770707 ) ) ;
#8328=CARTESIAN_POINT ( 'NONE',  ( -56.48582580120559271, 30.84685318188643066, 2.449293598294708485E-15 ) ) ;
#8332=CARTESIAN_POINT ( 'NONE',  ( 17.76569343199605200, 24.33587863439607801, -44.20364726159859003 ) ) ;
#8333=CARTESIAN_POINT ( 'NONE',  ( -162.0762913951021176, -27.08623940707624911, 29.48230308784761888 ) ) ;
#8334=CARTESIAN_POINT ( 'NONE',  ( -77.90255099906870839, -8.064892378658434779, 20.29001641120621713 ) ) ;
#8336=EDGE_CURVE ( 'NONE', #3196, #14641, #19726, .T. ) ;
#8337=CARTESIAN_POINT ( 'NONE',  ( -4.022465846214160479, 23.45302613997645125, -43.01021959554122276 ) ) ;
#8340=CARTESIAN_POINT ( 'NONE',  ( -105.3755690713226727, -2.472783935621397949E-13, 21.75974354311649961 ) ) ;
#8341=CARTESIAN_POINT ( 'NONE',  ( 170.0000000000000284, -22.62041470344884431, 9.369682556672202622 ) ) ;
#8342=CARTESIAN_POINT ( 'NONE',  ( -188.6013942375983561, -13.84412886956598499, 47.09843442133357883 ) ) ;
#8343=CARTESIAN_POINT ( 'NONE',  ( 184.8905102610680444, -14.79361573936330565, -41.77492675556016621 ) ) ;
#8344=CARTESIAN_POINT ( 'NONE',  ( 199.9999999999999432, 20.00000000000013856, 0.000000000000000000 ) ) ;
#8345=CARTESIAN_POINT ( 'NONE',  ( -195.1685814578025600, 24.52825302092950110, -44.46431112710755684 ) ) ;
#8346=CARTESIAN_POINT ( 'NONE',  ( 184.8905102610680444, -14.79361573936399665, 14.79361573936367158 ) ) ;
#8347=CARTESIAN_POINT ( 'NONE',  ( -100.7734535825088500, 40.53558337403654832, 16.03295912088756481 ) ) ;
#8348=CARTESIAN_POINT ( 'NONE',  ( -86.96347745069643054, -18.24025645688353947, 40.00000000000002132 ) ) ;
#8349=CARTESIAN_POINT ( 'NONE',  ( -100.7734535825088500, 17.32597176626809699, -40.00000000000002132 ) ) ;
#8350=CARTESIAN_POINT ( 'NONE',  ( 200.0000000000000000, -39.99999999999977973, -20.00000000000034817 ) ) ;
#8351=CARTESIAN_POINT ( 'NONE',  ( -198.0356074513804572, 39.15871834505901461, 39.15871834505919935 ) ) ;
#8352=AXIS2_PLACEMENT_3D ( 'NONE', #21830, #3600, #19829 ) ;
#8353=CARTESIAN_POINT ( 'NONE',  ( -97.73860346100398999, 20.89580782304006590, -8.185503821071858255 ) ) ;
#8354=CARTESIAN_POINT ( 'NONE',  ( -86.96347745069643054, 15.38646221621821297, -41.18208027870583265 ) ) ;
#8355=CARTESIAN_POINT ( 'NONE',  ( -114.7469200037856041, 2.762404124414770568, 21.93717741968527335 ) ) ;
#8357=CARTESIAN_POINT ( 'NONE',  ( 184.8905102610680444, -43.07788698682576722, 13.49065550809799063 ) ) ;
#8358=CARTESIAN_POINT ( 'NONE',  ( -96.94475454968154793, 8.190683501883270878, 20.92018922311200413 ) ) ;
#8359=CARTESIAN_POINT ( 'NONE',  ( 130.8568914410475088, 24.07718906446891793, 32.49135343045489321 ) ) ;
#8360=CARTESIAN_POINT ( 'NONE',  ( -4.031723327955742064, -46.99313739789356248, -13.82865651623149894 ) ) ;
#8361=ORIENTED_EDGE ( 'NONE', *, *, #15865, .T. ) ;
#8362=CARTESIAN_POINT ( 'NONE',  ( -91.56559293963834989, -22.67402823373193499, 0.000000000000000000 ) ) ;
#8364=ORIENTED_EDGE ( 'NONE', *, *, #19523, .T. ) ;
#8368=CARTESIAN_POINT ( 'NONE',  ( -188.6013942376021362, -47.09843442133525571, -13.84412886956576827 ) ) ;
#8370=CARTESIAN_POINT ( 'NONE',  ( -135.8532207217289738, -40.00000000000014921, 30.84685318188631697 ) ) ;
#8371=CARTESIAN_POINT ( 'NONE',  ( 57.59792236341147031, 37.56421063658187620, 40.00000000000002132 ) ) ;
#8374=CARTESIAN_POINT ( 'NONE',  ( -135.8532207217289738, 7.002209520526292428E-15, -9.153146818113572891 ) ) ;
#8375=CARTESIAN_POINT ( 'NONE',  ( -280.0000000000000568, 39.99999999999990763, 20.00000000000015987 ) ) ;
#8376=CARTESIAN_POINT ( 'NONE',  ( -56.48582580120560692, 40.00000000000004263, -9.153146818113443217 ) ) ;
#8377=CARTESIAN_POINT ( 'NONE',  ( 136.1360204305621266, 35.03383547441298873, 0.000000000000000000 ) ) ;
#8378=CARTESIAN_POINT ( 'NONE',  ( 136.1360204305621266, -4.966164525587039691, -2.449293598294708485E-15 ) ) ;
#8379=CARTESIAN_POINT ( 'NONE',  ( -213.1075012329537230, 18.58567234101121102, 37.98287015391247223 ) ) ;
#8380=CARTESIAN_POINT ( 'NONE',  ( -198.0356074513804572, 1.247057299367198800E-13, -15.37879056873070560 ) ) ;
#8381=CARTESIAN_POINT ( 'NONE',  ( 23.37394308801980713, -42.85717664514568526, -23.33966569535099822 ) ) ;
#8382=CARTESIAN_POINT ( 'NONE',  ( 146.6084372240433993, 8.568076647504290689E-14, -5.374981219216972583 ) ) ;
#8383=CARTESIAN_POINT ( 'NONE',  ( -86.96347745069644475, -8.210974027862429531E-14, 18.24025645688352881 ) ) ;
#8384=CARTESIAN_POINT ( 'NONE',  ( 0.2972598230769938343, 10.13633138497472252, 10.13633138497475628 ) ) ;
#8387=CARTESIAN_POINT ( 'NONE',  ( 130.8568914410475088, -4.207082182989324792, -52.36146031193423056 ) ) ;
#8389=CARTESIAN_POINT ( 'NONE',  ( -8.720657192084441789, 45.36528685024551066, -13.49580954686349799 ) ) ;
#8390=DIRECTION ( 'NONE',  ( -0.3301743753960648675, 0.000000000000000000, -0.9439199552037336183 ) ) ;
#8391=CARTESIAN_POINT ( 'NONE',  ( -208.1127848780264742, -55.00245453012676222, -2.449293598294708485E-15 ) ) ;
#8392=CARTESIAN_POINT ( 'NONE',  ( -87.13361725327077068, -1.365653317460838734, -21.49321519333430075 ) ) ;
#8393=CARTESIAN_POINT ( 'NONE',  ( 136.1360204305621266, -24.77266263493151044, 24.77266263493093135 ) ) ;
#8395=ORIENTED_EDGE ( 'NONE', *, *, #8523, .T. ) ;
#8397=CARTESIAN_POINT ( 'NONE',  ( -100.0968563617631020, 8.149320301509460407, -20.72609133246983149 ) ) ;
#8398=CARTESIAN_POINT ( 'NONE',  ( 21.80824205439920505, 13.88338701302733469, 47.36272483143116574 ) ) ;
#8400=ORIENTED_EDGE ( 'NONE', *, *, #1588, .T. ) ;
#8401=CARTESIAN_POINT ( 'NONE',  ( -86.96347745069644475, -15.38646221621786125, -15.38646221621789856 ) ) ;
#8403=CARTESIAN_POINT ( 'NONE',  ( -105.2054292635175585, 5.571723593410045370E-14, -21.49321519473985731 ) ) ;
#8404=DIRECTION ( 'NONE',  ( 0.000000000000000000, 0.7071067811865364705, 0.7071067811865586750 ) ) ;
#8405=CARTESIAN_POINT ( 'NONE',  ( -213.1075012329537230, 37.98287015391236565, -18.58567234101138510 ) ) ;
#8407=CARTESIAN_POINT ( 'NONE',  ( -87.13361725327072804, 5.903697393916396424E-14, -21.49321519333428299 ) ) ;
#8408=CARTESIAN_POINT ( 'NONE',  ( -103.9663809734738464, -8.026122149642342052, -20.15238534419602701 ) ) ;
#8409=CARTESIAN_POINT ( 'NONE',  ( 163.1118516004056573, 1.658263919738574066E-13, -12.73709011382475254 ) ) ;
#8410=CARTESIAN_POINT ( 'NONE',  ( 163.1118516004056573, 39.99999999999976552, 27.26290988616914746 ) ) ;
#8414=CARTESIAN_POINT ( 'NONE',  ( -188.8842190493876103, 17.93596163623949735, 43.30124183641348878 ) ) ;
#8415=CARTESIAN_POINT ( 'NONE',  ( 192.4448373802101173, -14.14213562370342281, 42.42640687122062104 ) ) ;
#8416=CARTESIAN_POINT ( 'NONE',  ( -200.0000000000000284, 19.98641303047029893, 45.65206365911533481 ) ) ;
#8417=CARTESIAN_POINT ( 'NONE',  ( 57.59792236341147031, 30.00663442387683588, 26.56190807104703211 ) ) ;
#8419=CARTESIAN_POINT ( 'NONE',  ( 14.38125909742180752, 17.55144818341503665, -39.01709431150898411 ) ) ;
#8421=CARTESIAN_POINT ( 'NONE',  ( 184.8905102610680444, 20.92133201514447194, 40.00000000000002132 ) ) ;
#8423=CARTESIAN_POINT ( 'NONE',  ( 151.7948205124836250, 23.49921654116361225, -23.49921654116333514 ) ) ;
#8424=CARTESIAN_POINT ( 'NONE',  ( 170.2234770963711128, 24.55285855007190676, 40.00000000000002132 ) ) ;
#8426=CARTESIAN_POINT ( 'NONE',  ( -208.1127848780264742, 40.00000000000055422, -55.00245453014380814 ) ) ;
#8427=CARTESIAN_POINT ( 'NONE',  ( 163.1118516004056573, 37.29075403953160617, -19.27778845539222985 ) ) ;
#8428=EDGE_CURVE ( 'NONE', #23960, #7172, #18616, .T. ) ;
#8429=CARTESIAN_POINT ( 'NONE',  ( 153.3020327024397318, -11.77299484472972857, 28.42252382389407472 ) ) ;
#8433=CARTESIAN_POINT ( 'NONE',  ( 170.2234770963711128, -24.55285855007184281, 40.00000000000002132 ) ) ;
#8435=CARTESIAN_POINT ( 'NONE',  ( 167.0466155511622048, 9.710058186601536079, 23.44215416552595954 ) ) ;
#8437=CARTESIAN_POINT ( 'NONE',  ( -86.96347745069644475, 12.89780903124419353, -12.89780903124389333 ) ) ;
#8438=CARTESIAN_POINT ( 'NONE',  ( -114.7465989397488926, -21.93543632637401330, 2.774003790514562251 ) ) ;
#8439=CARTESIAN_POINT ( 'NONE',  ( -199.9999999999999432, -55.16984130226965277, -2.449293598294708091E-15 ) ) ;
#8443=CARTESIAN_POINT ( 'NONE',  ( -162.0762913951020892, 1.198031840456041497, -57.76657433537918251 ) ) ;
#8444=CARTESIAN_POINT ( 'NONE',  ( -259.2033419157646676, -21.55415060305872998, 35.01439189186525880 ) ) ;
#8445=DIRECTION ( 'NONE',  ( 1.000000000000000000, 1.836970198721030181E-16, 0.000000000000000000 ) ) ;
#8446=CARTESIAN_POINT ( 'NONE',  ( 184.8905102610680444, -1.851754852062639767E-13, 20.92133201514444352 ) ) ;
#8447=CARTESIAN_POINT ( 'NONE',  ( 146.6084372240433709, -32.08495691632075619, 24.48358557860298035 ) ) ;
#8448=CARTESIAN_POINT ( 'NONE',  ( 136.1360204305621266, 35.03383547441298873, 0.000000000000000000 ) ) ;
#8449=CARTESIAN_POINT ( 'NONE',  ( 98.29820294270304259, -18.47759065022024672, 7.653668647299475047 ) ) ;
#8450=CARTESIAN_POINT ( 'NONE',  ( -91.56559293963836410, 16.03295912088714203, -16.03295912088699282 ) ) ;
#8451=CARTESIAN_POINT ( 'NONE',  ( -192.9588430854689989, -14.46834944099973086, 0.000000000000000000 ) ) ;
#8454=CARTESIAN_POINT ( 'NONE',  ( -238.4067589809705794, 39.99999999999983658, 40.96449428006354765 ) ) ;
#8456=CARTESIAN_POINT ( 'NONE',  ( 27.55177309528179208, 45.29548561696966402, -13.49150912998460683 ) ) ;
#8457=CARTESIAN_POINT ( 'NONE',  ( 163.1118516004056573, 12.73709011382478806, -40.00000000000002132 ) ) ;
#8458=CARTESIAN_POINT ( 'NONE',  ( -100.7734535825088358, -16.03295912088706743, -16.03295912088710296 ) ) ;
#8459=CARTESIAN_POINT ( 'NONE',  ( 5.009866156928156400, -24.71463403307551587, -44.71726210619360131 ) ) ;
#8461=CARTESIAN_POINT ( 'NONE',  ( -24.88648382771649636, -36.77569126515327724, 19.35593139197868240 ) ) ;
#8462=CARTESIAN_POINT ( 'NONE',  ( 57.59792236341147031, -2.435789363418150000, 40.00000000000002132 ) ) ;
#8463=ORIENTED_EDGE ( 'NONE', *, *, #2459, .F. ) ;
#8465=CARTESIAN_POINT ( 'NONE',  ( -30.26275506840324070, 1.198031551616013601, 1.198031551616023371 ) ) ;
#8467=CARTESIAN_POINT ( 'NONE',  ( 9.349823541344651545, 18.59402391556963252, -44.88994471603341196 ) ) ;
#8470=CARTESIAN_POINT ( 'NONE',  ( -16.41582555400823651, -39.35881747749594695, -21.03675245716867792 ) ) ;
#8471=CARTESIAN_POINT ( 'NONE',  ( -188.3066136396866170, -23.45085387054212589, 43.00728998844440554 ) ) ;
#8474=CARTESIAN_POINT ( 'NONE',  ( -135.8532207217289738, -6.472252184284280396, 6.472252184284099208 ) ) ;
#8475=CARTESIAN_POINT ( 'NONE',  ( -86.96347745069645896, 21.75974354311648895, -0.000000000000000000 ) ) ;
#8476=CARTESIAN_POINT ( 'NONE',  ( -188.8384220655398451, 17.93083973458498903, -43.28887647197245059 ) ) ;
#8477=CARTESIAN_POINT ( 'NONE',  ( -105.3755690713226727, 12.89780903124418998, -12.89780903124389155 ) ) ;
#8478=CARTESIAN_POINT ( 'NONE',  ( -100.7734535825088500, 12.25131212657428748, 44.31723036834913643 ) ) ;
#8479=CARTESIAN_POINT ( 'NONE',  ( 19.06497207195982924, -54.19242893257843008, -2.449293598294708485E-15 ) ) ;
#8480=CARTESIAN_POINT ( 'NONE',  ( 151.7948205124836250, 6.767089262349059275, 2.449293598294708485E-15 ) ) ;
#8482=CARTESIAN_POINT ( 'NONE',  ( 0.2972598230769957217, 1.502051041545559470E-13, -14.33493731733933352 ) ) ;
#8483=CARTESIAN_POINT ( 'NONE',  ( 14.38125909742181108, 39.01709431150907648, 39.01709431150921858 ) ) ;
#8484=CARTESIAN_POINT ( 'NONE',  ( 98.29820294267304348, -6.423630604792074372, 18.95183585406402571 ) ) ;
#8485=CARTESIAN_POINT ( 'NONE',  ( 151.7948205124836534, 23.49921654116056047, -33.06932595376338213 ) ) ;
#8487=EDGE_CURVE ( 'NONE', #3577, #4428, #4359, .T. ) ;
#8488=CARTESIAN_POINT ( 'NONE',  ( -259.2033419157646676, 6.730120644403521979, -6.730120644403498886 ) ) ;
#8490=VERTEX_POINT ( 'NONE', #24414 ) ;
#8491=CARTESIAN_POINT ( 'NONE',  ( -162.0762913951020892, 1.198031840385716418, 1.198031840385750169 ) ) ;
#8492=CARTESIAN_POINT ( 'NONE',  ( -100.0968563617871183, 8.893120081520745401, 20.41799937589878411 ) ) ;
#8495=CARTESIAN_POINT ( 'NONE',  ( 151.7948205124836534, 23.49921654116009506, 33.06932595376371609 ) ) ;
#8496=CARTESIAN_POINT ( 'NONE',  ( 6.984886629849392570, -49.25486234614436398, -14.16808340396968013 ) ) ;
#8502=CARTESIAN_POINT ( 'NONE',  ( 14.33519811653600229, 14.14278418308735574, -49.08818492847909454 ) ) ;
#8503=CARTESIAN_POINT ( 'NONE',  ( -191.2490444016914637, -43.85246840376581190, -18.16428715638521041 ) ) ;
#8504=CARTESIAN_POINT ( 'NONE',  ( -100.7734535825088358, -8.145438380286941744E-14, 17.32597176626811120 ) ) ;
#8505=CARTESIAN_POINT ( 'NONE',  ( 0.2972598230769930017, 54.33493731733938148, -40.00000000000002132 ) ) ;
#8508=CARTESIAN_POINT ( 'NONE',  ( -56.48582580120557850, -40.00000000000014211, 30.84685318188629921 ) ) ;
#8509=CARTESIAN_POINT ( 'NONE',  ( -192.9588430854690273, 39.99999999999980105, 54.46834944098235809 ) ) ;
#8511=CARTESIAN_POINT ( 'NONE',  ( 170.2234770963711128, 24.55285855007190321, 0.000000000000000000 ) ) ;
#8512=CARTESIAN_POINT ( 'NONE',  ( -135.8532207217289454, -30.84685318188648750, -40.00000000000002132 ) ) ;
#8513=CARTESIAN_POINT ( 'NONE',  ( -135.8532207217289738, 6.472252184283881604, 50.09629031063969506 ) ) ;
#8514=CARTESIAN_POINT ( 'NONE',  ( 98.29820294268191105, -7.653668647302824368, -18.47759065022797031 ) ) ;
#8517=CARTESIAN_POINT ( 'NONE',  ( 0.2972598230769956662, 40.00000000000058975, -54.33493731733894094 ) ) ;
#8518=CARTESIAN_POINT ( 'NONE',  ( -135.8532207217289738, -40.00000000000014921, 30.84685318188631697 ) ) ;
#8521=CARTESIAN_POINT ( 'NONE',  ( -99.29480781227209718, -8.934325994365195811, -20.48155342677144475 ) ) ;
#8522=CARTESIAN_POINT ( 'NONE',  ( -280.0000000000000000, -14.14213562373108779, 14.14213562373088529 ) ) ;
#8523=EDGE_CURVE ( 'NONE', #15766, #25369, #22465, .T. ) ;
#8524=VERTEX_POINT ( 'NONE', #2200 ) ;
#8525=CARTESIAN_POINT ( 'NONE',  ( -17.28139728229472993, 42.38047544420368240, -12.88180358348748378 ) ) ;
#8526=CARTESIAN_POINT ( 'NONE',  ( 126.3230993689413708, 28.30579214049057413, -11.72464299830486389 ) ) ;
#8527=CARTESIAN_POINT ( 'NONE',  ( 146.6084372240433709, -5.374981219216942385, -40.00000000000002132 ) ) ;
#8528=CARTESIAN_POINT ( 'NONE',  ( -83.21262154144248768, -33.12752917118415752, -13.72187187061501490 ) ) ;
#8529=CARTESIAN_POINT ( 'NONE',  ( -213.1075012329537230, 9.698598906450543566, -9.698598906450348167 ) ) ;
#8532=ORIENTED_EDGE ( 'NONE', *, *, #23375, .F. ) ;
#8533=CARTESIAN_POINT ( 'NONE',  ( 98.29820294273281434, -7.653668647304240125, 18.47759065023114644 ) ) ;
#8534=CARTESIAN_POINT ( 'NONE',  ( -96.94475454972737793, 8.190683501884381101, -20.92018922311151741 ) ) ;
#8535=CARTESIAN_POINT ( 'NONE',  ( 22.72189371635669985, 13.83659596079057685, 47.04833883279033557 ) ) ;
#8537=ORIENTED_EDGE ( 'NONE', *, *, #21911, .F. ) ;
#8538=CARTESIAN_POINT ( 'NONE',  ( 199.9999999999999432, -14.14213562373096345, -14.14213562373104871 ) ) ;
#8540=CARTESIAN_POINT ( 'NONE',  ( -110.0791661673311950, -4.394837301258886164, 19.70411816748108436 ) ) ;
#8543=CARTESIAN_POINT ( 'NONE',  ( 146.6084372240433993, -24.48358557860319706, -24.48358557860330720 ) ) ;
#8545=CARTESIAN_POINT ( 'NONE',  ( -89.91498783730511946, -8.087768383079360746, -20.43892340026755150 ) ) ;
#8546=CARTESIAN_POINT ( 'NONE',  ( -162.0762913951021176, 40.00000000000042633, -41.69427287672947102 ) ) ;
#8547=CARTESIAN_POINT ( 'NONE',  ( -280.0000000000000568, 39.99999999999976552, 20.00000000000043343 ) ) ;
#8552=CARTESIAN_POINT ( 'NONE',  ( -189.2667466962307401, 17.97628569363215689, 43.39859272266379975 ) ) ;
#8553=CARTESIAN_POINT ( 'NONE',  ( 4.995406935893297984, -39.06748935135205869, 17.50105314357158193 ) ) ;
#8554=CARTESIAN_POINT ( 'NONE',  ( -102.4068193528169957, 8.735227608996499526, 20.17396017424870536 ) ) ;
#8555=CARTESIAN_POINT ( 'NONE',  ( 136.1360204305621266, -3.511608612530682905, 3.511608612530666917 ) ) ;
#8556=CARTESIAN_POINT ( 'NONE',  ( 98.29820294267869940, -15.90088694521850776, 12.38338430224809983 ) ) ;
#8558=CARTESIAN_POINT ( 'NONE',  ( -162.0762913951020892, -29.48230308784744125, -29.48230308784792442 ) ) ;
#8559=CARTESIAN_POINT ( 'NONE',  ( -199.9999999999999432, 45.24754806069008595, -21.40989205436294540 ) ) ;
#8560=CARTESIAN_POINT ( 'NONE',  ( -135.8532207217289738, 9.153146818113548022, 40.00000000000002132 ) ) ;
#8561=CARTESIAN_POINT ( 'NONE',  ( -162.0762913951021176, 57.76657433523994456, -1.198031840315424867 ) ) ;
#8563=CARTESIAN_POINT ( 'NONE',  ( -213.1075012329537230, -13.71589010951915810, 0.000000000000000000 ) ) ;
#8565=CARTESIAN_POINT ( 'NONE',  ( -91.56559293963834989, 1.671088883502053755E-13, -17.32597176626811120 ) ) ;
#8567=CARTESIAN_POINT ( 'NONE',  ( 128.5824617753799544, -11.99766463964432717, 28.96492468983260338 ) ) ;
#8569=VERTEX_POINT ( 'NONE', #14955 ) ;
#8570=CARTESIAN_POINT ( 'NONE',  ( -213.1075012329537230, 13.71589010951907817, 40.00000000000002132 ) ) ;
#8573=CARTESIAN_POINT ( 'NONE',  ( 19.06497207195980792, 66.60410523465830579, -10.03556273973354251 ) ) ;
#8574=CARTESIAN_POINT ( 'NONE',  ( 90.68848816928600343, 21.08311784208570572, -9.291443205936941396 ) ) ;
#8577=CARTESIAN_POINT ( 'NONE',  ( -114.4364955367314707, 8.064892380844273845, -20.29001642038674902 ) ) ;
#8578=DIRECTION ( 'NONE',  ( 0.000000000000000000, 1.000000000000000000, 0.000000000000000000 ) ) ;
#8580=CARTESIAN_POINT ( 'NONE',  ( 170.0000000000000853, -9.369682556672300322, 22.62041470344878746 ) ) ;
#8581=CARTESIAN_POINT ( 'NONE',  ( 146.6084372240433709, -52.76785682606510619, -3.800685668859292043 ) ) ;
#8582=CARTESIAN_POINT ( 'NONE',  ( 130.8568914410475372, 24.07718906447210472, 24.07718906447249907 ) ) ;
#8583=DIRECTION ( 'NONE',  ( 0.01051738792039683817, -0.9166396752530959757, -0.3995761383056185556 ) ) ;
#8584=CARTESIAN_POINT ( 'NONE',  ( 163.1118516004056573, 40.00000000000017764, -12.73709011382432976 ) ) ;
#8585=CARTESIAN_POINT ( 'NONE',  ( -100.7734535825088500, 16.03295912088691821, 16.03295912088721309 ) ) ;
#8586=CARTESIAN_POINT ( 'NONE',  ( 8.517493190815724091, 14.17913040910384836, 49.32792454093237211 ) ) ;
#8587=CARTESIAN_POINT ( 'NONE',  ( -238.4067589809705794, 0.6820004457912757223, 0.6820004457913219076 ) ) ;
#8589=CARTESIAN_POINT ( 'NONE',  ( -105.3755690713226727, -12.89780903124413847, 12.89780903124398037 ) ) ;
#8590=CARTESIAN_POINT ( 'NONE',  ( -91.56559293963836410, 22.67402823373189946, -0.000000000000000000 ) ) ;
#8593=CARTESIAN_POINT ( 'NONE',  ( -91.56559293963834989, -7.976292724337646577E-14, 17.32597176626811120 ) ) ;
#8595=CARTESIAN_POINT ( 'NONE',  ( 23.40652632867984195, 42.84715492600962250, -23.33303889678548160 ) ) ;
#8597=CARTESIAN_POINT ( 'NONE',  ( -91.56559293963834989, -44.31723036834903695, 12.25131212657476709 ) ) ;
#8598=CARTESIAN_POINT ( 'NONE',  ( 4.995406935893288214, 55.24977328853207581, 40.00000000000002132 ) ) ;
#8599=( BOUNDED_CURVE ( )  B_SPLINE_CURVE ( 3, ( #19057, #2843, #8814, #10951, #10815, #839, #4835 ),
 .UNSPECIFIED., .F., .F. ) 
 B_SPLINE_CURVE_WITH_KNOTS ( ( 4, 3, 4 ),
 ( 0.007504510840757262248, 0.02318599846099208411, 0.03886748608122998772 ),
 .UNSPECIFIED. ) 
 CURVE ( )  GEOMETRIC_REPRESENTATION_ITEM ( )  RATIONAL_B_SPLINE_CURVE ( ( 0.5852718452494399815, 0.6660804010233956074, 0.8043231192735822432, 1.000000000000000000, 0.8043231192735437185, 0.6660804010233410954, 0.5852718452493922419 ) ) 
 REPRESENTATION_ITEM ( '' )  );
#8600=CARTESIAN_POINT ( 'NONE',  ( -4.558244102846159329, -46.81081390833291067, 13.79151199599502675 ) ) ;
#8601=CARTESIAN_POINT ( 'NONE',  ( -198.0356074513804572, 55.37879056871320671, 40.00000000000002132 ) ) ;
#8603=CARTESIAN_POINT ( 'NONE',  ( -199.9999999999999147, -49.28189405767606956, -14.17215463606684267 ) ) ;
#8604=CARTESIAN_POINT ( 'NONE',  ( -198.0356074513804572, 10.87444709759714989, 10.87444709759722450 ) ) ;
#8605=CARTESIAN_POINT ( 'NONE',  ( -3.443169733045703396, -17.93724492941688453, 43.30433998020581754 ) ) ;
#8606=MANIFOLD_SOLID_BREP ( 'Chamfer3', #10037 ) ;
#8607=CARTESIAN_POINT ( 'NONE',  ( -3.117754532606111795, 17.97158175134361002, -43.38723640139075854 ) ) ;
#8609=CARTESIAN_POINT ( 'NONE',  ( -162.0762913951021176, 29.48230308784730980, 27.08623940707652622 ) ) ;
#8611=CARTESIAN_POINT ( 'NONE',  ( -188.9524938556156712, -23.58789616779396425, 43.19211203808070820 ) ) ;
#8612=CARTESIAN_POINT ( 'NONE',  ( -259.2033419157646676, 35.01439189186559275, -21.55415060305807984 ) ) ;
#8613=CARTESIAN_POINT ( 'NONE',  ( 19.06497207195980792, -18.24870850772710540, -38.31983398719647482 ) ) ;
#8614=DIRECTION ( 'NONE',  ( 1.000000000000000000, 1.836970198721030181E-16, 0.000000000000000000 ) ) ;
#8615=CARTESIAN_POINT ( 'NONE',  ( 91.82158438592158234, 12.16597498397756993, 12.16597498397776356 ) ) ;
#8616=CARTESIAN_POINT ( 'NONE',  ( 151.7948205124836250, 4.785054706301759886, -4.785054706301612448 ) ) ;
#8617=CARTESIAN_POINT ( 'NONE',  ( -280.0000000000000568, 42.42640687119265408, 14.14213562373147504 ) ) ;
#8618=CARTESIAN_POINT ( 'NONE',  ( -30.26275506840322649, -41.69427246844630019, -2.449293598294708485E-15 ) ) ;
#8619=CARTESIAN_POINT ( 'NONE',  ( 200.0000000000000000, 19.99999999999995737, 40.00000000000002132 ) ) ;
#8620=CARTESIAN_POINT ( 'NONE',  ( -30.26275506840324070, -40.00000000000001421, -1.694272468446678559 ) ) ;
#8621=CARTESIAN_POINT ( 'NONE',  ( 170.2234770963711128, 39.20704971665398375, -17.36149277826984871 ) ) ;
#8622=CARTESIAN_POINT ( 'NONE',  ( -100.0968563617870899, 20.41799937589586378, -8.893120081528337550 ) ) ;
#8623=CARTESIAN_POINT ( 'NONE',  ( 184.8905102610680444, 14.79361573936424890, -41.77492675555986068 ) ) ;
#8624=CARTESIAN_POINT ( 'NONE',  ( 136.1360204305621266, 24.77266263493138965, -24.77266263493110188 ) ) ;
#8625=ORIENTED_EDGE ( 'NONE', *, *, #5241, .T. ) ;
#8626=CARTESIAN_POINT ( 'NONE',  ( -259.2033419157646676, -6.730120644403667640, 49.83842185052029805 ) ) ;
#8627=CARTESIAN_POINT ( 'NONE',  ( -198.0012279374161324, -14.15883993131235030, -49.19397028145281325 ) ) ;
#8628=CARTESIAN_POINT ( 'NONE',  ( -259.2033419157646676, 35.01439189186528722, 21.55415060305857011 ) ) ;
#8629=CARTESIAN_POINT ( 'NONE',  ( -2.164901439741091060, -43.53794903249359294, -23.84421257765930591 ) ) ;
#8630=EDGE_LOOP ( 'NONE', ( #21454, #2660, #2620, #16915 ) ) ;
#8631=CARTESIAN_POINT ( 'NONE',  ( 12.01361943528962151, -49.30661675909293962, -14.17591515420096648 ) ) ;
#8632=CARTESIAN_POINT ( 'NONE',  ( -87.13361725327074225, -15.19799821270821560, -15.19799821270861884 ) ) ;
#8634=ORIENTED_EDGE ( 'NONE', *, *, #13844, .F. ) ;
#8638=CARTESIAN_POINT ( 'NONE',  ( -86.96347745069644475, 18.24025645688351105, 2.449293598294708485E-15 ) ) ;
#8641=B_SPLINE_CURVE_WITH_KNOTS ( 'NONE', 3,
 ( #14412, #10554, #6689, #4322, #46, #2309, #10417, #6555 ),
 .UNSPECIFIED., .F., .F.,
 ( 4, 2, 2, 4 ),
 ( 0.000000000000000000, 0.002089226651506802951, 0.004178453303013605034, 0.008356906606027208334 ),
 .UNSPECIFIED. ) ;
#8642=CARTESIAN_POINT ( 'NONE',  ( -280.0000000000000568, -14.14213562373137556, 42.42640687119276066 ) ) ;
#8643=CARTESIAN_POINT ( 'NONE',  ( -135.8532207217289738, -1.351063376314938213E-13, 30.84685318188645553 ) ) ;
#8644=CARTESIAN_POINT ( 'NONE',  ( 14.38125909742180220, 39.99999999999997158, 15.17850393972647716 ) ) ;
#8646=CARTESIAN_POINT ( 'NONE',  ( 184.8905102610680444, 20.92133201514447549, 0.000000000000000000 ) ) ;
#8647=B_SPLINE_CURVE_WITH_KNOTS ( 'NONE', 3,
 ( #18909, #14777, #24641, #16773, #12787, #12513, #8392, #2693 ),
 .UNSPECIFIED., .F., .F.,
 ( 4, 2, 2, 4 ),
 ( 0.0002291277466111981624, 0.002289782534336058661, 0.004350437322060919133, 0.008471746897510642679 ),
 .UNSPECIFIED. ) ;
#8648=CARTESIAN_POINT ( 'NONE',  ( 184.8905102610680444, 14.79361573936396113, -14.79361573936377461 ) ) ;
#8649=CARTESIAN_POINT ( 'NONE',  ( -56.48582580120558561, -30.84685318188645553, -40.00000000000002132 ) ) ;
#8650=CARTESIAN_POINT ( 'NONE',  ( 136.1360204305621266, -3.511608612530682905, 3.511608612530666917 ) ) ;
#8651=CARTESIAN_POINT ( 'NONE',  ( -88.39148973765142614, -8.577159256668775100, 19.92926839984414755 ) ) ;
#8653=CARTESIAN_POINT ( 'NONE',  ( -135.8532207217289738, 40.00000000000031974, -30.84685318188603986 ) ) ;
#8654=CARTESIAN_POINT ( 'NONE',  ( -86.96347745069643054, -40.00000000000009948, 18.24025645688337960 ) ) ;
#8655=CARTESIAN_POINT ( 'NONE',  ( -105.3755690713226727, -15.38646221621786481, -15.38646221621789856 ) ) ;
#8658=CARTESIAN_POINT ( 'NONE',  ( -30.26275506840322649, -29.48230279907810925, 29.48230279907778950 ) ) ;
#8660=CARTESIAN_POINT ( 'NONE',  ( -77.70896657118109374, -5.469334093952031850, -21.30899064119132547 ) ) ;
#8661=CARTESIAN_POINT ( 'NONE',  ( -62.72988123315526821, 25.36777511009515962, -10.50767649768604173 ) ) ;
#8662=CARTESIAN_POINT ( 'NONE',  ( 140.2235668266256710, 30.42137084504312128, -12.60094438999823296 ) ) ;
#8663=CARTESIAN_POINT ( 'NONE',  ( 200.0000000000000000, -19.99999999999988631, -40.00000000000002132 ) ) ;
#8664=CARTESIAN_POINT ( 'NONE',  ( -86.95492415319874624, -20.33918386409409962, -6.698383215768170196 ) ) ;
#8665=CARTESIAN_POINT ( 'NONE',  ( -162.0762913951020892, 1.198031840385732849, -1.198031840385733515 ) ) ;
#8667=EDGE_LOOP ( 'NONE', ( #12093, #8060, #8169, #26349 ) ) ;
#8669=CARTESIAN_POINT ( 'NONE',  ( -105.4741150117382062, 8.366608964593805098, -19.60045294982731079 ) ) ;
#8670=CARTESIAN_POINT ( 'NONE',  ( 17.65190073993491637, 24.35922420889580664, 44.23515346912942192 ) ) ;
#8671=ORIENTED_EDGE ( 'NONE', *, *, #16818, .F. ) ;
#8673=ORIENTED_EDGE ( 'NONE', *, *, #6472, .T. ) ;
#8674=CARTESIAN_POINT ( 'NONE',  ( 151.7948205124836534, -51.78348778862535795, 4.785054706298367044 ) ) ;
#8676=CARTESIAN_POINT ( 'NONE',  ( -105.3394646353391266, -5.712077376943455853, 20.62740382081718238 ) ) ;
#8677=CARTESIAN_POINT ( 'NONE',  ( -192.9588430854690273, 10.23066800231970319, 66.79921049724369198 ) ) ;
#8679=CARTESIAN_POINT ( 'NONE',  ( 4.995406935893283773, 39.99999999999997158, 15.24977328854846803 ) ) ;
#8680=CARTESIAN_POINT ( 'NONE',  ( -93.12335834970889437, 6.205946304515388538E-14, -22.67402823373191723 ) ) ;
#8681=ADVANCED_FACE ( 'NONE', ( #9100 ), #2628, .T. ) ;
#8683=CARTESIAN_POINT ( 'NONE',  ( -4.039451493210489907, 13.82811171175507603, -46.99046209229789639 ) ) ;
#8684=CARTESIAN_POINT ( 'NONE',  ( 151.7948205124836534, 40.00000000000012079, -6.767089262348609857 ) ) ;
#8685=CARTESIAN_POINT ( 'NONE',  ( -192.9588430854689989, 1.161019517985663313E-13, -14.46834944099969533 ) ) ;
#8687=CARTESIAN_POINT ( 'NONE',  ( -87.13361725327077068, 14.22820505596910756, 16.16779136944769846 ) ) ;
#8689=CARTESIAN_POINT ( 'NONE',  ( -188.8383598209451861, 17.93083279444609701, 43.28885971699654789 ) ) ;
#8690=CARTESIAN_POINT ( 'NONE',  ( -86.86493150571114086, -7.943527260496002107, 19.77569912839178912 ) ) ;
#8691=CARTESIAN_POINT ( 'NONE',  ( -77.90255099906769942, -8.644468104261466834, -20.04994828523962980 ) ) ;
#8692=CARTESIAN_POINT ( 'NONE',  ( 57.59792236341148453, 1.722363176414758668, 54.84617931850880268 ) ) ;
#8693=CARTESIAN_POINT ( 'NONE',  ( -109.1264249741460617, 13.72187187123938656, 33.12752917269246211 ) ) ;
#8694=CARTESIAN_POINT ( 'NONE',  ( 163.1118516004056573, 47.56205970284970164, -9.006482792073828847 ) ) ;
#8696=CARTESIAN_POINT ( 'NONE',  ( -213.1075012329537230, -13.71589010951915810, 0.000000000000000000 ) ) ;
#8697=CARTESIAN_POINT ( 'NONE',  ( -198.0356074513804572, 39.15871834505887250, 17.40982414986519089 ) ) ;
#8698=CARTESIAN_POINT ( 'NONE',  ( -238.4067589809705794, -0.9644942799826263791, 40.00000000000002132 ) ) ;
#8701=CARTESIAN_POINT ( 'NONE',  ( -208.1127848780264742, -39.99999999999990763, -15.00245453012711394 ) ) ;
#8703=CARTESIAN_POINT ( 'NONE',  ( 98.29820294273281434, -7.653668647304240125, 18.47759065023114644 ) ) ;
#8704=ORIENTED_EDGE ( 'NONE', *, *, #1436, .F. ) ;
#8706=CARTESIAN_POINT ( 'NONE',  ( -91.56559293963834989, 17.32597176626809343, 2.449293598294708485E-15 ) ) ;
#8708=( BOUNDED_SURFACE ( )  B_SPLINE_SURFACE ( 3, 3, ( 
 ( #11363, #23730, #21612, #19481, #22015, #25492, #11484, #7241, #11617, #1267, #17480, #17604, #19612, #7495, #7368, #17735, #5775, #25876, #15480, #3649, #13745, #23607, #5511, #15735, #23861, #5639, #23485, #1657, #15606, #3786 ),
 ( #21742, #3517, #26017, #7754, #18140, #16417, #2061, #4196, #20417, #12289, #18543, #22284, #325, #6432, #55, #9898, #16011, #22548, #24278, #18002, #24137, #4329, #20547, #8290, #5909, #4454, #10167, #20009, #12419, #22420 ),
 ( #10425, #26288, #18270, #2194, #8426, #10301, #14019, #16546, #18408, #183, #14152, #22148, #20146, #8027, #24545, #1794, #24676, #26148, #14550, #12026, #2317, #4058, #3928, #6173, #14418, #7892, #22680, #1924, #10031, #12160 ),
 ( #6300, #8166, #16144, #6047, #20282, #16279, #24407, #14283, #25339, #18949, #2451, #8565, #15076, #16812, #10561, #16679, #23207, #13094, #859, #24810, #23337, #20950, #12549, #4988, #14948, #7096, #12830, #22944, #9094, #2728 ),
 ( #20681, #17201, #10704, #19078, #15210, #18674, #12959, #594, #17077, #10833, #8968, #460, #25211, #8834, #6562, #730, #21212, #4854, #6959, #20817, #16943, #989, #14678, #22813, #4590, #4723, #2589, #21078, #12687, #25078 ),
 ( #6829, #18814, #2984, #24950, #8701, #10970, #23082, #2863, #11091, #6698, #19207, #14811, #23581, #9223, #9738, #15839, #7467, #21339, #17578, #15582, #3110, #5358, #9347, #17332, #5113, #3234, #13465, #17455, #25466, #1373 ),
 ( #19846, #7727, #23706, #11588, #11339, #25595, #3357, #21713, #13217, #5485, #7217, #11215, #1631, #1114, #19329, #25715, #13585, #15333, #19454, #1498, #21586, #3491, #19710, #9604, #3617, #7341, #11727, #17840, #11459, #23461 ) ),
 .UNSPECIFIED., .T., .F., .T. ) 
 B_SPLINE_SURFACE_WITH_KNOTS ( ( 4, 3, 4 ),
 ( 4, 2, 2, 2, 2, 2, 2, 2, 2, 2, 2, 2, 2, 2, 4 ),
 ( 0.000000000000000000, 0.5000000000000000000, 1.000000000000000000 ),
 ( 0.000000000000000000, 0.1357259735107005372, 0.1651108541090157700, 0.1944957347073310028, 0.3598804999793158710, 0.3867117631979620773, 0.4135430264166082281, 0.5789277916885930964, 0.6062785021374117456, 0.6336292125862302838, 0.8508620842112317728, 0.8814014469398914198, 0.9119408096685510667, 0.9559704048342755334, 1.000000000000000000 ),
 .UNSPECIFIED. ) 
 GEOMETRIC_REPRESENTATION_ITEM ( )  RATIONAL_B_SPLINE_SURFACE ( (
 ( 1.000000000000000000, 1.000000000000000000, 1.000000000000000000, 1.000000000000000000, 1.000000000000000000, 1.000000000000000000, 1.000000000000000000, 1.000000000000000000, 1.000000000000000000, 1.000000000000000000, 1.000000000000000000, 1.000000000000000000, 1.000000000000000000, 1.000000000000000000, 1.000000000000000000, 1.000000000000000000, 1.000000000000000000, 1.000000000000000000, 1.000000000000000000, 1.000000000000000000, 1.000000000000000000, 1.000000000000000000, 1.000000000000000000, 1.000000000000000000, 1.000000000000000000, 1.000000000000000000, 1.000000000000000000, 1.000000000000000000, 1.000000000000000000, 1.000000000000000000),
 ( 0.3333333333333333703, 0.3333333333333333703, 0.3333333333333333703, 0.3333333333333333703, 0.3333333333333333703, 0.3333333333333333703, 0.3333333333333333703, 0.3333333333333333703, 0.3333333333333333703, 0.3333333333333333703, 0.3333333333333333703, 0.3333333333333333703, 0.3333333333333333703, 0.3333333333333333703, 0.3333333333333333703, 0.3333333333333333703, 0.3333333333333333703, 0.3333333333333333703, 0.3333333333333333703, 0.3333333333333333703, 0.3333333333333333703, 0.3333333333333333703, 0.3333333333333333703, 0.3333333333333333703, 0.3333333333333333703, 0.3333333333333333703, 0.3333333333333333703, 0.3333333333333333703, 0.3333333333333333703, 0.3333333333333333703),
 ( 0.3333333333333333703, 0.3333333333333333703, 0.3333333333333333703, 0.3333333333333333703, 0.3333333333333333703, 0.3333333333333333703, 0.3333333333333333703, 0.3333333333333333703, 0.3333333333333333703, 0.3333333333333333703, 0.3333333333333333703, 0.3333333333333333703, 0.3333333333333333703, 0.3333333333333333703, 0.3333333333333333703, 0.3333333333333333703, 0.3333333333333333703, 0.3333333333333333703, 0.3333333333333333703, 0.3333333333333333703, 0.3333333333333333703, 0.3333333333333333703, 0.3333333333333333703, 0.3333333333333333703, 0.3333333333333333703, 0.3333333333333333703, 0.3333333333333333703, 0.3333333333333333703, 0.3333333333333333703, 0.3333333333333333703),
 ( 1.000000000000000000, 1.000000000000000000, 1.000000000000000000, 1.000000000000000000, 1.000000000000000000, 1.000000000000000000, 1.000000000000000000, 1.000000000000000000, 1.000000000000000000, 1.000000000000000000, 1.000000000000000000, 1.000000000000000000, 1.000000000000000000, 1.000000000000000000, 1.000000000000000000, 1.000000000000000000, 1.000000000000000000, 1.000000000000000000, 1.000000000000000000, 1.000000000000000000, 1.000000000000000000, 1.000000000000000000, 1.000000000000000000, 1.000000000000000000, 1.000000000000000000, 1.000000000000000000, 1.000000000000000000, 1.000000000000000000, 1.000000000000000000, 1.000000000000000000),
 ( 0.3333333333333333703, 0.3333333333333333703, 0.3333333333333333703, 0.3333333333333333703, 0.3333333333333333703, 0.3333333333333333703, 0.3333333333333333703, 0.3333333333333333703, 0.3333333333333333703, 0.3333333333333333703, 0.3333333333333333703, 0.3333333333333333703, 0.3333333333333333703, 0.3333333333333333703, 0.3333333333333333703, 0.3333333333333333703, 0.3333333333333333703, 0.3333333333333333703, 0.3333333333333333703, 0.3333333333333333703, 0.3333333333333333703, 0.3333333333333333703, 0.3333333333333333703, 0.3333333333333333703, 0.3333333333333333703, 0.3333333333333333703, 0.3333333333333333703, 0.3333333333333333703, 0.3333333333333333703, 0.3333333333333333703),
 ( 0.3333333333333333703, 0.3333333333333333703, 0.3333333333333333703, 0.3333333333333333703, 0.3333333333333333703, 0.3333333333333333703, 0.3333333333333333703, 0.3333333333333333703, 0.3333333333333333703, 0.3333333333333333703, 0.3333333333333333703, 0.3333333333333333703, 0.3333333333333333703, 0.3333333333333333703, 0.3333333333333333703, 0.3333333333333333703, 0.3333333333333333703, 0.3333333333333333703, 0.3333333333333333703, 0.3333333333333333703, 0.3333333333333333703, 0.3333333333333333703, 0.3333333333333333703, 0.3333333333333333703, 0.3333333333333333703, 0.3333333333333333703, 0.3333333333333333703, 0.3333333333333333703, 0.3333333333333333703, 0.3333333333333333703),
 ( 1.000000000000000000, 1.000000000000000000, 1.000000000000000000, 1.000000000000000000, 1.000000000000000000, 1.000000000000000000, 1.000000000000000000, 1.000000000000000000, 1.000000000000000000, 1.000000000000000000, 1.000000000000000000, 1.000000000000000000, 1.000000000000000000, 1.000000000000000000, 1.000000000000000000, 1.000000000000000000, 1.000000000000000000, 1.000000000000000000, 1.000000000000000000, 1.000000000000000000, 1.000000000000000000, 1.000000000000000000, 1.000000000000000000, 1.000000000000000000, 1.000000000000000000, 1.000000000000000000, 1.000000000000000000, 1.000000000000000000, 1.000000000000000000, 1.000000000000000000) ) ) 
 REPRESENTATION_ITEM ( '' )  SURFACE ( )  );
#8709=FACE_OUTER_BOUND ( 'NONE', #4593, .T. ) ;
#8710=FACE_OUTER_BOUND ( 'NONE', #23838, .T. ) ;
#8714=CARTESIAN_POINT ( 'NONE',  ( 91.82158438592158234, -40.45024623143936537, -16.11829626348475131 ) ) ;
#8715=CARTESIAN_POINT ( 'NONE',  ( -100.7734535825088500, 16.03295912088691821, 16.03295912088721309 ) ) ;
#8717=CARTESIAN_POINT ( 'NONE',  ( -192.9588430854690273, 40.00000000000014211, -14.46834944099927966 ) ) ;
#8718=CARTESIAN_POINT ( 'NONE',  ( -30.26275506840324070, -1.198031551616016266, -1.198031551616031587 ) ) ;
#8719=CARTESIAN_POINT ( 'NONE',  ( -213.1075012329537230, -13.71589010951915810, 0.000000000000000000 ) ) ;
#8720=CARTESIAN_POINT ( 'NONE',  ( -280.0000000000000568, -42.42640687119295251, 14.14213562373088351 ) ) ;
#8721=CARTESIAN_POINT ( 'NONE',  ( -135.8532207217289738, -21.81201906317788186, 21.81201906317762962 ) ) ;
#8724=CARTESIAN_POINT ( 'NONE',  ( -213.1075012329537230, -8.703598725189323045E-14, 13.71589010951911902 ) ) ;
#8725=CARTESIAN_POINT ( 'NONE',  ( 67.79414719548314849, 28.72755866874277686, -14.15005687142633839 ) ) ;
#8727=CARTESIAN_POINT ( 'NONE',  ( -259.2033419157646676, -35.01439189186554302, 21.55415060305832498 ) ) ;
#8728=CARTESIAN_POINT ( 'NONE',  ( 19.06497207195980792, 14.19242893257840699, 40.00000000000002132 ) ) ;
#8730=CARTESIAN_POINT ( 'NONE',  ( -0.5869797817515145510, -43.96874597321873779, 18.21245090264041266 ) ) ;
#8732=CARTESIAN_POINT ( 'NONE',  ( -192.9588430854689989, 54.46834944099968823, 2.449293598294708485E-15 ) ) ;
#8734=CARTESIAN_POINT ( 'NONE',  ( 20.59039453120235663, 23.90179120638680388, -43.61606461192713624 ) ) ;
#8735=CARTESIAN_POINT ( 'NONE',  ( -105.3755690713226727, -15.38646221621786481, -15.38646221621789856 ) ) ;
#8736=CARTESIAN_POINT ( 'NONE',  ( -3.534370630407254854, -17.92707699455397119, 43.27979241395971144 ) ) ;
#8738=CARTESIAN_POINT ( 'NONE',  ( -4.061681315507501999, 13.82654462146623331, -46.98276670624658635 ) ) ;
#8740=CARTESIAN_POINT ( 'NONE',  ( 0.2972598230769886718, 38.42060263243643448, 18.14793986248763957 ) ) ;
#8742=CARTESIAN_POINT ( 'NONE',  ( -192.1964066538387783, -14.00508515770005147, 48.17614796926734755 ) ) ;
#8743=CARTESIAN_POINT ( 'NONE',  ( -280.0000000000000568, 42.42640687119294540, -14.14213562373059041 ) ) ;
#8744=CARTESIAN_POINT ( 'NONE',  ( -238.4067589809705794, -0.6820004457913680929, 0.6820004457913170226 ) ) ;
#8745=CARTESIAN_POINT ( 'NONE',  ( -192.9588430854689989, 10.23066800230756712, -10.23066800230735396 ) ) ;
#8749=CARTESIAN_POINT ( 'NONE',  ( -213.1075012329537230, 18.58567234101174037, -37.98287015391222354 ) ) ;
#8750=CARTESIAN_POINT ( 'NONE',  ( -213.1075012329537230, 66.26714140138673770, -9.698598906462034819 ) ) ;
#8751=CARTESIAN_POINT ( 'NONE',  ( -238.4067589809705794, 57.25054294065799354, -0.6820004457334954973 ) ) ;
#8752=CARTESIAN_POINT ( 'NONE',  ( 151.7948205124836534, -6.767089262349006873, 40.00000000000002132 ) ) ;
#8753=CARTESIAN_POINT ( 'NONE',  ( -238.4067589809705794, 0.9644942799825385604, -40.00000000000002132 ) ) ;
#8754=CARTESIAN_POINT ( 'NONE',  ( -30.26275506840325136, 29.48230279907798135, -27.08623969584585112 ) ) ;
#8755=( BOUNDED_SURFACE ( )  B_SPLINE_SURFACE ( 3, 2, ( 
 ( #3554, #11396, #1305 ),
 ( #25658, #5424, #25275 ),
 ( #7281, #13527, #5049 ),
 ( #15516, #17644, #21781 ),
 ( #7404, #25785, #13280 ),
 ( #19142, #23646, #23522 ),
 ( #5294, #7025, #19518 ),
 ( #15398, #3423, #926 ),
 ( #21651, #13402, #3048 ),
 ( #1052, #11525, #21526 ),
 ( #19650, #7535, #21402 ),
 ( #23274, #3302, #1435 ),
 ( #9158, #15271, #9535 ),
 ( #9036, #25533, #9413 ),
 ( #15644, #17519, #23771 ),
 ( #11155, #17140, #5549 ),
 ( #13156, #13657, #25404 ),
 ( #21276, #19270, #5177 ),
 ( #3175, #17270, #7155 ),
 ( #23401, #11279, #19401 ),
 ( #1183, #9285, #17393 ),
 ( #20056, #8068, #10206 ),
 ( #20321, #26325, #22457 ),
 ( #94, #24176, #18042 ),
 ( #16187, #1835, #15908 ),
 ( #24320, #26055, #22056 ),
 ( #5951, #9936, #24041 ),
 ( #3830, #26197, #13922 ),
 ( #19781, #22192, #7934 ),
 ( #20183, #9805, #6213 ),
 ( #11797, #8202, #5817 ),
 ( #17912, #16320, #16050 ),
 ( #6085, #14190, #14061 ),
 ( #12066, #12199, #7792 ),
 ( #22324, #11931, #14324 ),
 ( #23902, #11655, #3967 ),
 ( #1968, #15774, #4099 ),
 ( #10073, #2097, #18177 ),
 ( #18312, #1567, #24444 ),
 ( #9672, #17776, #25919 ),
 ( #7663, #5678, #13784 ),
 ( #21917, #3690, #19916 ),
 ( #1700, #8605, #16584 ),
 ( #22982, #2763, #16980 ),
 ( #499, #18713, #4491 ),
 ( #20583, #8736, #24986 ),
 ( #24846, #12727, #16715 ),
 ( #6599, #14848, #14719 ),
 ( #363, #10740, #10337 ),
 ( #2357, #20454, #10602 ),
 ( #14458, #22851, #12456 ),
 ( #14982, #4760, #4236 ),
 ( #4626, #10471, #18851 ),
 ( #221, #24717, #6471 ),
 ( #12325, #20850, #2630 ),
 ( #630, #16855, #18446 ),
 ( #6736, #12864, #16458 ),
 ( #20982, #10870, #6866 ),
 ( #18986, #2229, #764 ),
 ( #8869, #25116, #8334 ) ),
 .UNSPECIFIED., .F., .F., .T. ) 
 B_SPLINE_SURFACE_WITH_KNOTS ( ( 4, 2, 2, 2, 2, 2, 2, 2, 2, 2, 2, 2, 2, 2, 2, 2, 2, 2, 2, 2, 2, 2, 2, 2, 2, 2, 2, 2, 2, 4 ),
 ( 3, 3 ),
 ( -6.934549977324601594E-05, 0.02465257023823465635, 0.04937448597624256169, 0.07409640171425047050, 0.08027688064875244944, 0.08066316058215883267, 0.08085630054886201734, 0.08090458554053781004, 0.08095287053221361662, 0.08104944051556520201, 0.08182200038237794071, 0.08336712011600344585, 0.08645735958325442838, 0.09263783851775639344, 0.09881831745225837238, 0.1019085569195093688, 0.1049987963867603513, 0.1111792753212623164, 0.1173597542557642953, 0.1177460341891706785, 0.1179391741558738632, 0.1179874591475496559, 0.1180357441392254625, 0.1181323141225770479, 0.1189048739893897866, 0.1204499937230152917, 0.1235402331902662743, 0.1482621489282741900, 0.1729840646662820780, 0.1977059804042899938 ),
 ( 0.000000000000000000, 1.000000000000000000 ),
 .UNSPECIFIED. ) 
 GEOMETRIC_REPRESENTATION_ITEM ( )  RATIONAL_B_SPLINE_SURFACE ( (
 ( 1.000000000000000000, 1.000000000000000000, 1.000000000000000000),
 ( 1.000000000000000000, 0.9999975583948276237, 1.000000000000000000),
 ( 1.000000000000000000, 0.9982436956964818586, 1.000000000000000000),
 ( 1.000000000000000000, 0.9910288481548262807, 1.000000000000000000),
 ( 1.000000000000000000, 0.9855714588515670505, 1.000000000000000000),
 ( 1.000000000000000000, 0.9705958323316278280, 1.000000000000000000),
 ( 1.000000000000000000, 0.9610788543733380651, 1.000000000000000000),
 ( 1.000000000000000000, 0.9462867046312647412, 1.000000000000000000),
 ( 1.000000000000000000, 0.9431828180755345015, 1.000000000000000000),
 ( 1.000000000000000000, 0.9397240291170321225, 1.000000000000000000),
 ( 1.000000000000000000, 0.9395199791395947297, 1.000000000000000000),
 ( 1.000000000000000000, 0.9392130141387216025, 1.000000000000000000),
 ( 1.000000000000000000, 0.9391105441325042769, 1.000000000000000000),
 ( 1.000000000000000000, 0.9389822709566328918, 1.000000000000000000),
 ( 1.000000000000000000, 0.9389566070380596097, 1.000000000000000000),
 ( 1.000000000000000000, 0.9389052606279760793, 1.000000000000000000),
 ( 1.000000000000000000, 0.9388799835492060986, 1.000000000000000000),
 ( 1.000000000000000000, 0.9388039637710071661, 1.000000000000000000),
 ( 1.000000000000000000, 0.9387533729070444144, 1.000000000000000000),
 ( 1.000000000000000000, 0.9382988607467089848, 1.000000000000000000),
 ( 1.000000000000000000, 0.9379005790853230939, 1.000000000000000000),
 ( 1.000000000000000000, 0.9367237203702156734, 1.000000000000000000),
 ( 1.000000000000000000, 0.9359625442025921727, 1.000000000000000000),
 ( 1.000000000000000000, 0.9337619511409316342, 1.000000000000000000),
 ( 1.000000000000000000, 0.9324064515427418209, 1.000000000000000000),
 ( 1.000000000000000000, 0.9287106072118640476, 1.000000000000000000),
 ( 1.000000000000000000, 0.9267422912947972380, 1.000000000000000000),
 ( 1.000000000000000000, 0.9239539123018306599, 1.000000000000000000),
 ( 1.000000000000000000, 0.9231338493906536824, 1.000000000000000000),
 ( 1.000000000000000000, 0.9228496048507791594, 1.000000000000000000),
 ( 1.000000000000000000, 0.9229135694615112628, 1.000000000000000000),
 ( 1.000000000000000000, 0.9233494155302143236, 1.000000000000000000),
 ( 1.000000000000000000, 0.9237209353788754518, 1.000000000000000000),
 ( 1.000000000000000000, 0.9252744993862994649, 1.000000000000000000),
 ( 1.000000000000000000, 0.9268968421604496521, 1.000000000000000000),
 ( 1.000000000000000000, 0.9311673748453518362, 1.000000000000000000),
 ( 1.000000000000000000, 0.9338157035273875195, 1.000000000000000000),
 ( 1.000000000000000000, 0.9370733336298756599, 1.000000000000000000),
 ( 1.000000000000000000, 0.9372665829346552568, 1.000000000000000000),
 ( 1.000000000000000000, 0.9375588533504852773, 1.000000000000000000),
 ( 1.000000000000000000, 0.9376566762263802701, 1.000000000000000000),
 ( 1.000000000000000000, 0.9377794499114608939, 1.000000000000000000),
 ( 1.000000000000000000, 0.9378038842964712130, 1.000000000000000000),
 ( 1.000000000000000000, 0.9378536652368906212, 1.000000000000000000),
 ( 1.000000000000000000, 0.9378785472098815079, 1.000000000000000000),
 ( 1.000000000000000000, 0.9379531676447474542, 1.000000000000000000),
 ( 1.000000000000000000, 0.9380028806225414462, 1.000000000000000000),
 ( 1.000000000000000000, 0.9384499917948422310, 1.000000000000000000),
 ( 1.000000000000000000, 0.9388452506063807990, 1.000000000000000000),
 ( 1.000000000000000000, 0.9400245377240871170, 1.000000000000000000),
 ( 1.000000000000000000, 0.9408020798629985748, 1.000000000000000000),
 ( 1.000000000000000000, 0.9431089717073132261, 1.000000000000000000),
 ( 1.000000000000000000, 0.9446123105950532395, 1.000000000000000000),
 ( 1.000000000000000000, 0.9578370004756148193, 1.000000000000000000),
 ( 1.000000000000000000, 0.9674308273343072972, 1.000000000000000000),
 ( 1.000000000000000000, 0.9828254127557660702, 1.000000000000000000),
 ( 1.000000000000000000, 0.9886239107116222558, 1.000000000000000000),
 ( 1.000000000000000000, 0.9967564037645807451, 1.000000000000000000),
 ( 1.000000000000000000, 0.9990872413561198151, 1.000000000000000000),
 ( 1.000000000000000000, 0.9997813423572990965, 1.000000000000000000) ) ) 
 REPRESENTATION_ITEM ( '' )  SURFACE ( )  );
#8756=CARTESIAN_POINT ( 'NONE',  ( -89.91498783734905942, 20.43892340027597854, -8.087768383073672851 ) ) ;
#8757=CARTESIAN_POINT ( 'NONE',  ( 192.4448373802101173, 14.14213562375922884, -42.42640687116488607 ) ) ;
#8758=CARTESIAN_POINT ( 'NONE',  ( -188.8383598209457546, 43.28885971699691737, -17.93083279444630662 ) ) ;
#8760=CARTESIAN_POINT ( 'NONE',  ( -208.1127848780264742, 67.17687982760683951, 10.60833733268317403 ) ) ;
#8761=CARTESIAN_POINT ( 'NONE',  ( -102.4309680865787442, 8.733065089997754882, 20.17061239841417475 ) ) ;
#8762=CARTESIAN_POINT ( 'NONE',  ( -105.3755690713226727, -12.89780903124413847, 12.89780903124398037 ) ) ;
#8763=CARTESIAN_POINT ( 'NONE',  ( 11.71430589693571989, -44.87285427231137191, -24.82930166508382541 ) ) ;
#8766=CARTESIAN_POINT ( 'NONE',  ( 57.59792236341147031, -2.435789363418150444, 0.000000000000000000 ) ) ;
#8767=CARTESIAN_POINT ( 'NONE',  ( -93.12335834970889437, -16.03295912088706388, -16.03295912088710651 ) ) ;
#8771=CARTESIAN_POINT ( 'NONE',  ( 0.2972598230769930017, 54.33493731733936016, 40.00000000000002132 ) ) ;
#8775=CARTESIAN_POINT ( 'NONE',  ( 136.1360204305621266, -3.511608612531119000, 53.05693388239312469 ) ) ;
#8776=CARTESIAN_POINT ( 'NONE',  ( -91.56559293963836410, 39.99999999999994316, 17.32597176626825330 ) ) ;
#8777=CARTESIAN_POINT ( 'NONE',  ( -280.0000000000000568, 40.00000000000004263, -19.99999999999987210 ) ) ;
#8778=CARTESIAN_POINT ( 'NONE',  ( -105.2054292635175869, 15.19799821370233062, -15.19799821370219206 ) ) ;
#8779=CARTESIAN_POINT ( 'NONE',  ( 0.2972598230770130412, -54.33493731733936016, -2.449293598294708485E-15 ) ) ;
#8780=CARTESIAN_POINT ( 'NONE',  ( 23.46661716383002982, -23.32081713244383891, -42.82867125331112845 ) ) ;
#8781=CARTESIAN_POINT ( 'NONE',  ( 14.38125909742181285, -10.73282306404727393, 10.73282306404716380 ) ) ;
#8782=CARTESIAN_POINT ( 'NONE',  ( 146.6084372240433993, -5.374981219216945938, -2.449293598294708485E-15 ) ) ;
#8783=CARTESIAN_POINT ( 'NONE',  ( 0.2972598230770100991, -38.42060263243686791, 38.42060263243645579 ) ) ;
#8784=CARTESIAN_POINT ( 'NONE',  ( 158.3379117892985164, -10.98149362779622251, -26.51167085133963397 ) ) ;
#8785=CARTESIAN_POINT ( 'NONE',  ( -114.7824662270011657, 14.65611376398968169, -16.64100530757652052 ) ) ;
#8786=CARTESIAN_POINT ( 'NONE',  ( 0.2972598230770030492, 5.716321584140269555E-13, -54.33493731733936016 ) ) ;
#8787=CARTESIAN_POINT ( 'NONE',  ( 57.59792236341147031, 39.99999999999990763, 37.56421063658199699 ) ) ;
#8788=CARTESIAN_POINT ( 'NONE',  ( 91.82158438592158234, 16.11829626348434630, -40.45024623143955012 ) ) ;
#8790=CARTESIAN_POINT ( 'NONE',  ( -96.93773665438902754, -9.001171854902104030, -20.58457565566405734 ) ) ;
#8791=CARTESIAN_POINT ( 'NONE',  ( 4.995406935893310418, -67.35176059880237176, 10.78321810387813429 ) ) ;
#8793=CARTESIAN_POINT ( 'NONE',  ( -162.0762913951020892, -1.198031840385767266, -1.198031840385758384 ) ) ;
#8796=CARTESIAN_POINT ( 'NONE',  ( -135.8532207217289738, -30.84685318188647685, -2.449293598294708485E-15 ) ) ;
#8797=CARTESIAN_POINT ( 'NONE',  ( -105.2054292635175727, 15.19799821370213522, 15.19799821370241943 ) ) ;
#8798=CARTESIAN_POINT ( 'NONE',  ( -56.48582580120559271, -6.472252184284276844, 6.472252184284108978 ) ) ;
#8799=VERTEX_POINT ( 'NONE', #23588 ) ;
#8800=VERTEX_POINT ( 'NONE', #3628 ) ;
#8802=CARTESIAN_POINT ( 'NONE',  ( -102.4309680866255690, 8.733065090073308667, -20.17061239837894959 ) ) ;
#8806=CARTESIAN_POINT ( 'NONE',  ( 0.2972598230769990524, -18.14793986248724522, 38.42060263243662632 ) ) ;
#8809=B_SPLINE_CURVE_WITH_KNOTS ( 'NONE', 3,
 ( #10281, #12008, #24120, #6028, #22265, #24657, #12140, #12529, #17981, #24527, #4178, #7870, #12272, #5891, #18390, #8146 ),
 .UNSPECIFIED., .F., .F.,
 ( 4, 2, 2, 2, 2, 2, 2, 4 ),
 ( -5.998499568544072563E-08, 0.003520343011582062996, 0.007040746008159811872, 0.01408155200131532003, 0.01760195499789307325, 0.02112235799447082993, 0.02464276099104858314, 0.02816316398762633982 ),
 .UNSPECIFIED. ) ;
#8810=CARTESIAN_POINT ( 'NONE',  ( -91.56559293963834989, -16.03295912088716335, 40.53558337403673306 ) ) ;
#8811=CARTESIAN_POINT ( 'NONE',  ( 163.1118516004056573, -19.27778845538761132, -19.27778845538770724 ) ) ;
#8812=CARTESIAN_POINT ( 'NONE',  ( -100.7734535825088500, 39.99999999999994316, 17.32597176626825686 ) ) ;
#8813=CARTESIAN_POINT ( 'NONE',  ( -199.9999999999997726, -24.82633483071077762, 44.86878812508861358 ) ) ;
#8814=CARTESIAN_POINT ( 'NONE',  ( -199.9999999999999432, -4.865628651906739321, 55.16984130226897776 ) ) ;
#8815=CARTESIAN_POINT ( 'NONE',  ( 19.06497207195981858, 5.735870351258996432E-13, -54.19242893257843008 ) ) ;
#8816=CARTESIAN_POINT ( 'NONE',  ( 192.4448373802100889, -1.741373372144848397E-13, 20.00000000003942091 ) ) ;
#8817=CARTESIAN_POINT ( 'NONE',  ( -77.80807733969351148, 19.71366427569386559, 9.671920888572945074 ) ) ;
#8818=SPHERICAL_SURFACE ( 'NONE', #11944, 15.00000000000000000 ) ;
#8820=CARTESIAN_POINT ( 'NONE',  ( -188.3610564113221812, 13.83140491817328410, 47.01267209787948076 ) ) ;
#8821=CARTESIAN_POINT ( 'NONE',  ( -30.26275506840324070, -29.48230279907817675, 27.08623969584564151 ) ) ;
#8822=EDGE_CURVE ( 'NONE', #1453, #13720, #9569, .T. ) ;
#8824=CARTESIAN_POINT ( 'NONE',  ( 184.8905102610680444, -13.49065550809810965, 13.49065550809799596 ) ) ;
#8825=CARTESIAN_POINT ( 'NONE',  ( -87.05569247514564779, -17.94468678732216915, 11.73639047247333878 ) ) ;
#8826=CARTESIAN_POINT ( 'NONE',  ( -259.2033419157646676, -21.55415060305824326, -21.55415060305857367 ) ) ;
#8827=CARTESIAN_POINT ( 'NONE',  ( -200.0000000000000284, 45.65206365911554087, -19.98641303047023854 ) ) ;
#8828=DIRECTION ( 'NONE',  ( -1.850371707708594760E-15, -0.3995982397413175291, -0.9166903767334096953 ) ) ;
#8829=CARTESIAN_POINT ( 'NONE',  ( -238.4067589809705794, 57.25054294065799354, -0.6820004457334954973 ) ) ;
#8830=EDGE_CURVE ( 'NONE', #4362, #24911, #23703, .T. ) ;
#8831=CARTESIAN_POINT ( 'NONE',  ( 91.82158438592159655, -22.79471317813468900, 40.00000000000002132 ) ) ;
#8834=CARTESIAN_POINT ( 'NONE',  ( -56.48582580120557850, -39.99999999999970868, -30.84685318188687120 ) ) ;
#8835=EDGE_CURVE ( 'NONE', #19209, #13176, #19881, .T. ) ;
#8841=ORIENTED_EDGE ( 'NONE', *, *, #18883, .F. ) ;
#8842=CARTESIAN_POINT ( 'NONE',  ( 184.8905102610680444, 19.07866798485561333, 40.00000000000002132 ) ) ;
#8844=CARTESIAN_POINT ( 'NONE',  ( 83.06440094971527799, 23.65491511361215160, -10.91839312130610651 ) ) ;
#8845=CARTESIAN_POINT ( 'NONE',  ( -77.55672185583993894, -16.64541244686190424, 14.65061613760696524 ) ) ;
#8846=CARTESIAN_POINT ( 'NONE',  ( 4.995406935893290878, -5.232665749138292703E-14, 15.24977328854832592 ) ) ;
#8849=CARTESIAN_POINT ( 'NONE',  ( 4.995406935893297984, 10.78321810390233892, -67.35176059882522281 ) ) ;
#8850=CARTESIAN_POINT ( 'NONE',  ( -30.26275506840324070, -1.198031551616016266, -1.198031551616031587 ) ) ;
#8851=CARTESIAN_POINT ( 'NONE',  ( -110.0368417077424965, -18.51665893310755351, -7.992411109430164196 ) ) ;
#8852=CARTESIAN_POINT ( 'NONE',  ( 200.0000000000000000, 39.99999999999985079, 20.00000000000052225 ) ) ;
#8853=CARTESIAN_POINT ( 'NONE',  ( 146.6084372240433709, -3.800685668859084210, 52.76785682606516303 ) ) ;
#8854=CARTESIAN_POINT ( 'NONE',  ( -91.56559293963836410, 22.67402823373189946, -0.000000000000000000 ) ) ;
#8855=CARTESIAN_POINT ( 'NONE',  ( -198.0356074513804572, -10.87444709760996986, 67.44298959253333692 ) ) ;
#8858=CARTESIAN_POINT ( 'NONE',  ( 151.7948205124836534, 40.00000000000017053, -33.23291073765538783 ) ) ;
#8859=CARTESIAN_POINT ( 'NONE',  ( 170.2234770963711128, -24.55285855007183926, 0.000000000000000000 ) ) ;
#8860=CARTESIAN_POINT ( 'NONE',  ( -56.48582580120559982, -34.75652343174615311, 21.81201906317766870 ) ) ;
#8861=CARTESIAN_POINT ( 'NONE',  ( -280.0000000000000568, 19.99999999999995737, 40.00000000000002132 ) ) ;
#8863=CARTESIAN_POINT ( 'NONE',  ( 19.44355705749374152, -43.94967286772092052, 18.20455056366046165 ) ) ;
#8864=( BOUNDED_CURVE ( )  B_SPLINE_CURVE ( 3, ( #16486, #6364, #18879, #20884, #6632, #14611, #22743 ),
 .UNSPECIFIED., .F., .F. ) 
 B_SPLINE_CURVE_WITH_KNOTS ( ( 4, 3, 4 ),
 ( 0.007486030685209765952, 0.02316748376737289700, 0.03884893684953920345 ),
 .UNSPECIFIED. ) 
 CURVE ( )  GEOMETRIC_REPRESENTATION_ITEM ( )  RATIONAL_B_SPLINE_CURVE ( ( 0.5852718452494414247, 0.6660804010233971617, 0.8043231192735833535, 1.000000000000000000, 0.8043231192735437185, 0.6660804010233410954, 0.5852718452493922419 ) ) 
 REPRESENTATION_ITEM ( '' )  );
#8865=CARTESIAN_POINT ( 'NONE',  ( 57.59792236341147031, 37.56421063658187620, -40.00000000000002132 ) ) ;
#8868=CARTESIAN_POINT ( 'NONE',  ( -77.92915424793434909, 20.15198149301296482, 8.347224043097730473 ) ) ;
#8869=CARTESIAN_POINT ( 'NONE',  ( -77.90255099906872260, -8.644468104261276764, 20.04994828523928163 ) ) ;
#8870=CARTESIAN_POINT ( 'NONE',  ( -82.25372479520392233, 19.83917633296052685, 3.752706786415938467 ) ) ;
#8872=CARTESIAN_POINT ( 'NONE',  ( -6.754359963566859193, 17.56548336386092757, -42.40682816664624966 ) ) ;
#8874=CARTESIAN_POINT ( 'NONE',  ( -198.0356074513804572, 10.87444709759730088, -10.87444709759707173 ) ) ;
#8876=CARTESIAN_POINT ( 'NONE',  ( 116.7964245048382850, -27.98274000340147794, 0.000000000000000000 ) ) ;
#8877=CARTESIAN_POINT ( 'NONE',  ( -188.9478905404513114, -17.94277290414816406, 43.31768569177503281 ) ) ;
#8878=CARTESIAN_POINT ( 'NONE',  ( -192.9588430854689989, -10.23066800230742501, -10.23066800230756712 ) ) ;
#8879=CARTESIAN_POINT ( 'NONE',  ( -162.0762913951020892, -1.198031840385783919, 1.198031840385741731 ) ) ;
#8880=CARTESIAN_POINT ( 'NONE',  ( 146.6084372240433709, -24.48358557860284179, -32.08495691632087699 ) ) ;
#8881=FACE_OUTER_BOUND ( 'NONE', #5840, .T. ) ;
#8882=CARTESIAN_POINT ( 'NONE',  ( -105.3755690713226585, 43.67073346367988051, -12.89780903124366418 ) ) ;
#8883=CARTESIAN_POINT ( 'NONE',  ( -280.0000000000000568, 42.42640687119265408, 14.14213562373147504 ) ) ;
#8884=CARTESIAN_POINT ( 'NONE',  ( 146.6084372240433709, 32.08495691632030145, 24.48358557860365181 ) ) ;
#8885=CARTESIAN_POINT ( 'NONE',  ( -56.48582580120559982, 9.153146818113574668, 40.00000000000002132 ) ) ;
#8886=CARTESIAN_POINT ( 'NONE',  ( 170.2234770963711128, -24.55285855007184281, -40.00000000000002132 ) ) ;
#8887=CARTESIAN_POINT ( 'NONE',  ( 130.8568914410475088, 4.207082182989741348, -52.36146031193420924 ) ) ;
#8889=CARTESIAN_POINT ( 'NONE',  ( 130.8568914410475088, -32.49135343045495006, 24.07718906446878648 ) ) ;
#8890=CARTESIAN_POINT ( 'NONE',  ( -187.7698581930513058, 46.80706826624110306, -13.79076165500642404 ) ) ;
#8892=CARTESIAN_POINT ( 'NONE',  ( 14.38125909742181463, 10.73282306405862485, 67.30136555898259587 ) ) ;
#8893=CARTESIAN_POINT ( 'NONE',  ( -188.2995950289365226, 23.44932284465886241, 43.00522595870971543 ) ) ;
#8894=CARTESIAN_POINT ( 'NONE',  ( -259.2033419157646676, -21.55415060305854524, 21.55415060305827524 ) ) ;
#8895=CARTESIAN_POINT ( 'NONE',  ( -1.624577210513715730, -43.75845733971997475, -18.12534649861195035 ) ) ;
#8898=CARTESIAN_POINT ( 'NONE',  ( -114.6381211271834673, -11.20694786414384936, -18.98758604910076997 ) ) ;
#8900=CARTESIAN_POINT ( 'NONE',  ( -188.2995950289364373, 13.82811170417284075, -46.99046209955416487 ) ) ;
#8902=CARTESIAN_POINT ( 'NONE',  ( 163.1118516004056573, 12.73709011382478273, 2.449293598294708485E-15 ) ) ;
#8905=EDGE_CURVE ( 'NONE', #18174, #1858, #3633, .T. ) ;
#8906=CARTESIAN_POINT ( 'NONE',  ( 184.8905102610680444, -13.49065550809840630, 43.07788698682565354 ) ) ;
#8907=CARTESIAN_POINT ( 'NONE',  ( -91.56559293963834989, -7.976292724337646577E-14, 17.32597176626811120 ) ) ;
#8908=CARTESIAN_POINT ( 'NONE',  ( 130.8568914410475088, 40.00000000000015632, -34.05028731879774284 ) ) ;
#8909=( BOUNDED_SURFACE ( )  B_SPLINE_SURFACE ( 3, 2, ( 
 ( #15322, #10825, #4978 ),
 ( #19197, #21329, #25583 ),
 ( #13085, #21202, #25456 ),
 ( #17068, #19319, #9085 ),
 ( #11205, #8959, #3222 ),
 ( #17191, #25327, #7086 ),
 ( #18938, #3101, #25202 ),
 ( #11328, #5223, #2853 ),
 ( #1101, #19444, #13327 ),
 ( #20942, #23327, #8825 ),
 ( #5103, #21448, #1232 ),
 ( #10961, #15200, #4845 ),
 ( #9337, #7330, #16935 ),
 ( #15443, #23571, #9211 ),
 ( #17322, #25070, #6821 ),
 ( #14938, #23074, #12951 ) ),
 .UNSPECIFIED., .F., .F., .F. ) 
 B_SPLINE_SURFACE_WITH_KNOTS ( ( 4, 2, 2, 2, 2, 2, 2, 4 ),
 ( 3, 3 ),
 ( 0.04143342415446721327, 0.04844559399082600665, 0.05195167890900539986, 0.05545776382718480002, 0.06246993366354359339, 0.06422297612263329347, 0.06597601858172298661, 0.06948210349990238677 ),
 ( 0.000000000000000000, 1.000000000000000000 ),
 .UNSPECIFIED. ) 
 GEOMETRIC_REPRESENTATION_ITEM ( )  RATIONAL_B_SPLINE_SURFACE ( (
 ( 1.000000000000000000, 0.9541700779530469800, 1.000000000000000000),
 ( 1.000000000000000000, 0.9520168980296377370, 1.000000000000000000),
 ( 1.000000000000000000, 0.9503263051604914358, 1.000000000000000000),
 ( 1.000000000000000000, 0.9485964699095221775, 1.000000000000000000),
 ( 1.000000000000000000, 0.9481599523402173268, 1.000000000000000000),
 ( 1.000000000000000000, 0.9475783919165745584, 1.000000000000000000),
 ( 1.000000000000000000, 0.9474332805886676034, 1.000000000000000000),
 ( 1.000000000000000000, 0.9474385816640782387, 1.000000000000000000),
 ( 1.000000000000000000, 0.9480200071112050431, 1.000000000000000000),
 ( 1.000000000000000000, 0.9494436219493812557, 1.000000000000000000),
 ( 1.000000000000000000, 0.9497633688928907025, 1.000000000000000000),
 ( 1.000000000000000000, 0.9504729676352060563, 1.000000000000000000),
 ( 1.000000000000000000, 0.9508638236298538882, 1.000000000000000000),
 ( 1.000000000000000000, 0.9521268919816204823, 1.000000000000000000),
 ( 1.000000000000000000, 0.9530924015900935631, 1.000000000000000000),
 ( 1.000000000000000000, 0.9541700779530452037, 1.000000000000000000) ) ) 
 REPRESENTATION_ITEM ( '' )  SURFACE ( )  );
#8911=CARTESIAN_POINT ( 'NONE',  ( 19.06497207195980792, -14.19242893257839988, -40.00000000000002132 ) ) ;
#8912=CARTESIAN_POINT ( 'NONE',  ( 19.94008347559497452, -13.96811062196804443, -47.92933869853823836 ) ) ;
#8914=CARTESIAN_POINT ( 'NONE',  ( 14.38125909742182884, -55.17850393974264733, -40.00000000000002132 ) ) ;
#8915=CARTESIAN_POINT ( 'NONE',  ( -162.0762913951020892, -1.198031840385783919, 1.198031840385741731 ) ) ;
#8916=CARTESIAN_POINT ( 'NONE',  ( -126.6834154282191776, 9.107266658309034923, 24.89646316986419450 ) ) ;
#8917=CARTESIAN_POINT ( 'NONE',  ( -163.5815439468645991, -18.59457101073928342, 35.61501074489160601 ) ) ;
#8918=CARTESIAN_POINT ( 'NONE',  ( 151.7948205124836250, 1.012150473917908975E-13, -6.767089262349031742 ) ) ;
#8919=CARTESIAN_POINT ( 'NONE',  ( -56.48582580120559271, -6.472252184284187138, -6.472252184284199572 ) ) ;
#8920=CARTESIAN_POINT ( 'NONE',  ( 128.5815561518678294, -28.96468886173051516, -11.99756695644574123 ) ) ;
#8922=CARTESIAN_POINT ( 'NONE',  ( -135.8532207217289738, 6.472252184283881604, 50.09629031063969506 ) ) ;
#8923=EDGE_CURVE ( 'NONE', #6176, #23081, #17366, .T. ) ;
#8924=ORIENTED_EDGE ( 'NONE', *, *, #23767, .T. ) ;
#8925=CARTESIAN_POINT ( 'NONE',  ( -198.0356074513804572, -10.87444709759714634, -10.87444709759729911 ) ) ;
#8926=CARTESIAN_POINT ( 'NONE',  ( -6.342283169554340461, 42.32555349774960263, -23.00001740814328954 ) ) ;
#8927=CARTESIAN_POINT ( 'NONE',  ( 128.5824617753800680, 28.96492468983282009, -11.99766463964400565 ) ) ;
#8928=CARTESIAN_POINT ( 'NONE',  ( -238.4067589809705794, -40.96449428006345528, 40.00000000000002132 ) ) ;
#8930=EDGE_CURVE ( 'NONE', #13176, #21839, #18939, .T. ) ;
#8932=CARTESIAN_POINT ( 'NONE',  ( -195.5009199109406666, 44.52807166370264014, -18.44413118942395613 ) ) ;
#8934=ORIENTED_EDGE ( 'NONE', *, *, #10106, .T. ) ;
#8936=CARTESIAN_POINT ( 'NONE',  ( -100.0753760173605542, 8.894334231739680519, -20.41987330121789768 ) ) ;
#8937=B_SPLINE_CURVE_WITH_KNOTS ( 'NONE', 3,
 ( #19448, #13459, #7461, #1367, #1887, #5607, #24372, #9992, #26251, #21973 ),
 .UNSPECIFIED., .F., .F.,
 ( 4, 2, 2, 2, 4 ),
 ( 0.7921542097164080420, 0.8508620842112317728, 0.8814014469398914198, 0.9119408096685510667, 0.9406682828395580565 ),
 .UNSPECIFIED. ) ;
#8941=CARTESIAN_POINT ( 'NONE',  ( 192.4448373802100889, -14.14213562375876698, -14.14213562375885047 ) ) ;
#8943=CARTESIAN_POINT ( 'NONE',  ( -105.2833435977151737, -4.389626034945506738, 20.98775841734936165 ) ) ;
#8944=CARTESIAN_POINT ( 'NONE',  ( -280.0000000000000568, -42.42640687119295251, 14.14213562373088351 ) ) ;
#8945=CARTESIAN_POINT ( 'NONE',  ( -105.2990478492033191, 20.88641510963992332, 4.839947517601303595 ) ) ;
#8946=CARTESIAN_POINT ( 'NONE',  ( 136.1360204305621551, 40.00000000000002842, 4.966164525587208445 ) ) ;
#8947=DIRECTION ( 'NONE',  ( 1.000000000000000000, 5.508077988093228416E-14, 0.000000000000000000 ) ) ;
#8948=CARTESIAN_POINT ( 'NONE',  ( -86.86493150571119770, -7.943527260495915066, -19.77569912839184596 ) ) ;
#8950=CARTESIAN_POINT ( 'NONE',  ( 146.6084372240433709, -40.00000000000036238, 34.62501878078263218 ) ) ;
#8951=CARTESIAN_POINT ( 'NONE',  ( -135.8532207217289738, -39.99999999999972289, -30.84685318188688541 ) ) ;
#8952=CARTESIAN_POINT ( 'NONE',  ( -87.13361725336062591, 15.69997917300612933, 14.69601725244436885 ) ) ;
#8955=CARTESIAN_POINT ( 'NONE',  ( -197.6434631108650706, 18.53520396667539671, 44.74794079763712773 ) ) ;
#8956=CARTESIAN_POINT ( 'NONE',  ( -91.56559293963836410, -12.25131212657524138, 44.31723036834888774 ) ) ;
#8958=CARTESIAN_POINT ( 'NONE',  ( 192.4448373802101173, 14.14213562375862665, 42.42640687116509213 ) ) ;
#8959=CARTESIAN_POINT ( 'NONE',  ( -82.24432634622075966, -12.38461122506346435, 15.96101146153378103 ) ) ;
#8960=CARTESIAN_POINT ( 'NONE',  ( 14.38125909742181996, -10.73282306405815234, -67.30136555898266693 ) ) ;
#8963=ORIENTED_EDGE ( 'NONE', *, *, #8336, .T. ) ;
#8964=CARTESIAN_POINT ( 'NONE',  ( -30.26275506840324070, 1.198031551616030033, -1.198031551616006496 ) ) ;
#8965=CARTESIAN_POINT ( 'NONE',  ( -208.1127848780265026, -15.00245453012673202, 0.000000000000000000 ) ) ;
#8968=CARTESIAN_POINT ( 'NONE',  ( -100.7734535825088500, -39.99999999999986500, -17.32597176626853397 ) ) ;
#8971=ORIENTED_EDGE ( 'NONE', *, *, #5570, .T. ) ;
#8972=ORIENTED_EDGE ( 'NONE', *, *, #5245, .F. ) ;
#8974=CARTESIAN_POINT ( 'NONE',  ( -192.9588430854690273, 54.46834944101718889, 40.00000000000002132 ) ) ;
#8976=CARTESIAN_POINT ( 'NONE',  ( -103.9650464694441041, -20.03380587597265716, -8.298274098614912830 ) ) ;
#8977=EDGE_CURVE ( 'NONE', #13725, #8230, #1953, .T. ) ;
#8978=B_SPLINE_CURVE_WITH_KNOTS ( 'NONE', 3,
 ( #1439, #15651, #19653, #21405, #11529, #21530, #23405, #13787 ),
 .UNSPECIFIED., .F., .F.,
 ( 4, 2, 2, 4 ),
 ( 0.008471746897480886968, 0.01057975003218126868, 0.01268775316688165039, 0.01690375943628241728 ),
 .UNSPECIFIED. ) ;
#8979=CARTESIAN_POINT ( 'NONE',  ( 57.59792236341147031, 1.908507979671054758E-14, -2.435789363418160658 ) ) ;
#8981=ADVANCED_FACE ( 'NONE', ( #16658 ), #13189, .T. ) ;
#8984=CARTESIAN_POINT ( 'NONE',  ( -135.8532207217289738, -6.472252184283586729, -50.09629031063973770 ) ) ;
#8985=B_SPLINE_CURVE_WITH_KNOTS ( 'NONE', 3,
 ( #11867, #4176, #12398, #166, #1771, #8271 ),
 .UNSPECIFIED., .F., .F.,
 ( 4, 2, 4 ),
 ( 0.0003134705440570314063, 0.004478952798826419529, 0.008644435053595807272 ),
 .UNSPECIFIED. ) ;
#8986=CARTESIAN_POINT ( 'NONE',  ( 136.1360204305621266, 24.77266263493104148, 24.77266263493145004 ) ) ;
#8987=AXIS2_PLACEMENT_3D ( 'NONE', #17684, #25572, #19952 ) ;
#8988=CARTESIAN_POINT ( 'NONE',  ( -110.0574659383507878, -18.01685545903095331, -9.172431002379518361 ) ) ;
#8989=CARTESIAN_POINT ( 'NONE',  ( -56.48582580120558561, 3.151766524733697544E-13, -30.84685318188644132 ) ) ;
#8991=CARTESIAN_POINT ( 'NONE',  ( 0.4289713102705710046, 14.02712011273575676, 48.32239598606143005 ) ) ;
#8992=CARTESIAN_POINT ( 'NONE',  ( 57.59792236341148453, -54.84617931850877426, -1.722363176415331099 ) ) ;
#8995=CARTESIAN_POINT ( 'NONE',  ( 136.1360204305621551, 40.00000000000017053, -35.03383547441281820 ) ) ;
#8996=CARTESIAN_POINT ( 'NONE',  ( 146.6084372240433709, -34.62501878078303008, -40.00000000000002132 ) ) ;
#8997=CARTESIAN_POINT ( 'NONE',  ( -86.96347745069644475, -15.38646221621796073, 41.18208027870593924 ) ) ;
#8998=CARTESIAN_POINT ( 'NONE',  ( -30.26275506840324425, 41.69427246844627177, 40.00000000000002132 ) ) ;
#9000=CARTESIAN_POINT ( 'NONE',  ( 1.925538622543135903, -48.64880301058170886, 14.07631154917441663 ) ) ;
#9002=CARTESIAN_POINT ( 'NONE',  ( -100.7734535825088500, -22.67402823373193499, -40.00000000000002132 ) ) ;
#9004=CARTESIAN_POINT ( 'NONE',  ( -162.0762913951020892, 29.48230308784758691, 29.48230308784772191 ) ) ;
#9005=CARTESIAN_POINT ( 'NONE',  ( 130.8568914410475088, -39.99999999999988631, -34.05028731879802706 ) ) ;
#9006=CARTESIAN_POINT ( 'NONE',  ( -82.30220482034330587, 18.74474319042426984, -7.441767004318775136 ) ) ;
#9007=CARTESIAN_POINT ( 'NONE',  ( -47.30403195813222084, 12.59259458032456713, -30.40121262098807620 ) ) ;
#9010=CARTESIAN_POINT ( 'NONE',  ( -213.1075012329537230, 66.26714140138673770, -9.698598906462034819 ) ) ;
#9013=DIRECTION ( 'NONE',  ( 0.000000000000000000, 0.3995982397855803447, 0.9166903767141147963 ) ) ;
#9014=CARTESIAN_POINT ( 'NONE',  ( 23.37394308801977871, -23.33966569535037294, -42.85717664514612579 ) ) ;
#9015=CARTESIAN_POINT ( 'NONE',  ( -135.8532207217289738, 34.75652343174625258, -21.81201906317744132 ) ) ;
#9016=CARTESIAN_POINT ( 'NONE',  ( -238.4067589809705794, 27.60227080167040370, 28.96627169325338613 ) ) ;
#9018=CARTESIAN_POINT ( 'NONE',  ( -56.48582580120559271, 6.472252184284121412, 6.472252184284244869 ) ) ;
#9020=CARTESIAN_POINT ( 'NONE',  ( -208.1127848780265026, -10.60833733269537227, -10.60833733269551793 ) ) ;
#9021=CARTESIAN_POINT ( 'NONE',  ( 14.38125909742180397, 67.30136555898270956, -10.73282306405792319 ) ) ;
#9022=CARTESIAN_POINT ( 'NONE',  ( -100.7734535825088500, -16.03295912088659492, -40.53558337403696044 ) ) ;
#9023=CARTESIAN_POINT ( 'NONE',  ( 146.6084372240433709, 5.374981219217002781, -40.00000000000002132 ) ) ;
#9024=CARTESIAN_POINT ( 'NONE',  ( 130.8568914410475088, 32.49135343045483637, -24.07718906446901030 ) ) ;
#9026=CARTESIAN_POINT ( 'NONE',  ( -280.0000000000000568, -42.42640687119305198, 14.14213562373058686 ) ) ;
#9027=CARTESIAN_POINT ( 'NONE',  ( -144.0562564039820188, 31.27039870050057146, -10.50946916206093817 ) ) ;
#9029=CARTESIAN_POINT ( 'NONE',  ( -162.0762913951020892, 29.48230308784758691, 29.48230308784772191 ) ) ;
#9031=CARTESIAN_POINT ( 'NONE',  ( -91.56559293963836410, 44.31723036834890905, 12.25131212657507795 ) ) ;
#9034=CARTESIAN_POINT ( 'NONE',  ( -188.2652133075167455, -46.97855991888840066, 13.82568790539422388 ) ) ;
#9036=CARTESIAN_POINT ( 'NONE',  ( 23.41418334855306327, -23.33148157649288379, 42.84479974151765447 ) ) ;
#9037=CARTESIAN_POINT ( 'NONE',  ( 136.1360204305621551, -35.03383547441293899, -40.00000000000002132 ) ) ;
#9038=CARTESIAN_POINT ( 'NONE',  ( 60.07376046270519510, 13.17995839193378060, -31.81923430133271324 ) ) ;
#9040=CARTESIAN_POINT ( 'NONE',  ( -135.8532207217289738, -21.81201906317806305, 34.75652343174590442 ) ) ;
#9041=CARTESIAN_POINT ( 'NONE',  ( 170.2234770963711128, -2.511315425431857630E-14, 15.44714144992816074 ) ) ;
#9042=CARTESIAN_POINT ( 'NONE',  ( -213.1075012329537230, -8.703598725189323045E-14, 13.71589010951911902 ) ) ;
#9044=CARTESIAN_POINT ( 'NONE',  ( 130.8568914410475088, 34.05028731879790627, -40.00000000000002132 ) ) ;
#9045=CARTESIAN_POINT ( 'NONE',  ( 23.35901252181217913, -23.34306388117422060, -42.86175755505345109 ) ) ;
#9046=CARTESIAN_POINT ( 'NONE',  ( 4.995406935893293543, -10.78321810389005364, 10.78321810388994173 ) ) ;
#9047=CARTESIAN_POINT ( 'NONE',  ( -100.7734535825088500, 22.67402823373189591, -0.000000000000000000 ) ) ;
#9048=CARTESIAN_POINT ( 'NONE',  ( -135.8532207217289738, 34.75652343174594705, 21.81201906317792449 ) ) ;
#9049=CARTESIAN_POINT ( 'NONE',  ( -86.96347745069645896, 40.00000000000019895, -18.24025645688310249 ) ) ;
#9050=CARTESIAN_POINT ( 'NONE',  ( -114.7465989397677220, 17.47221266595968459, -13.54917888338830068 ) ) ;
#9051=CARTESIAN_POINT ( 'NONE',  ( -162.0762913951020892, -39.99999999999961631, -41.69427287692722928 ) ) ;
#9053=CARTESIAN_POINT ( 'NONE',  ( 149.5792919132162524, -29.41975665910036142, -12.18606220991559219 ) ) ;
#9055=CARTESIAN_POINT ( 'NONE',  ( 91.82158438592156813, 40.45024623143950038, 16.11829626348447420 ) ) ;
#9056=EDGE_LOOP ( 'NONE', ( #25818, #10832, #14814, #16874 ) ) ;
#9057=CARTESIAN_POINT ( 'NONE',  ( 4.995406935893293543, -10.78321810388990265, -10.78321810389009272 ) ) ;
#9058=CARTESIAN_POINT ( 'NONE',  ( -3.993758944536190736, 47.00698038897044739, -13.83056263162072952 ) ) ;
#9060=CARTESIAN_POINT ( 'NONE',  ( 14.38125909742181285, -15.17850393972633505, 40.00000000000002132 ) ) ;
#9061=CARTESIAN_POINT ( 'NONE',  ( -114.4364955367314707, 8.064892380844273845, -20.29001642038674902 ) ) ;
#9063=ORIENTED_EDGE ( 'NONE', *, *, #15877, .T. ) ;
#9066=CARTESIAN_POINT ( 'NONE',  ( 116.7964245048362102, 1.191563696448279148E-13, -27.98274000340060041 ) ) ;
#9069=CARTESIAN_POINT ( 'NONE',  ( -105.2276882639782656, -2.726203881901831050, 21.34721338855225881 ) ) ;
#9070=CARTESIAN_POINT ( 'NONE',  ( -213.1075012329537230, 9.698598906462684965, 66.26714140138669507 ) ) ;
#9071=CARTESIAN_POINT ( 'NONE',  ( -259.2033419157646676, -6.730120644403570829, -6.730120644403545960 ) ) ;
#9072=CARTESIAN_POINT ( 'NONE',  ( -192.9588430854690273, 39.99999999999992895, 14.46834944099983922 ) ) ;
#9074=DIRECTION ( 'NONE',  ( 0.000000000000000000, 1.000000000000000000, 0.000000000000000000 ) ) ;
#9076=CARTESIAN_POINT ( 'NONE',  ( -280.0000000000000568, -40.00000000000028422, 19.99999999999959499 ) ) ;
#9077=CARTESIAN_POINT ( 'NONE',  ( -30.26275506840324425, 40.00000000000044764, -41.69427246844585255 ) ) ;
#9080=CARTESIAN_POINT ( 'NONE',  ( -200.0000000000000000, 20.90527768611954684, -45.34857661735428280 ) ) ;
#9081=CARTESIAN_POINT ( 'NONE',  ( -195.5009199109816791, 18.44413118942227570, 44.52807166372294745 ) ) ;
#9082=CARTESIAN_POINT ( 'NONE',  ( -96.93773665438804699, 8.190703376740504638, 20.92028269119447970 ) ) ;
#9083=CARTESIAN_POINT ( 'NONE',  ( -100.0753760173626290, 8.894334231739064123, 20.41987330121790833 ) ) ;
#9084=CARTESIAN_POINT ( 'NONE',  ( 146.6084372240433993, 24.48358557860341733, -24.48358557860313311 ) ) ;
#9085=CARTESIAN_POINT ( 'NONE',  ( -87.08883489502147768, -12.58611167335523007, 17.39766501533223320 ) ) ;
#9086=CARTESIAN_POINT ( 'NONE',  ( 57.59792236341148453, -26.56190807104663421, -26.56190807104710672 ) ) ;
#9087=CARTESIAN_POINT ( 'NONE',  ( -166.7090905286406723, -15.35183918171654227, -37.06261835958360962 ) ) ;
#9088=CARTESIAN_POINT ( 'NONE',  ( -90.07798792367799479, 15.74993999324163951, 15.74993999324193084 ) ) ;
#9089=ORIENTED_EDGE ( 'NONE', *, *, #3211, .F. ) ;
#9090=CARTESIAN_POINT ( 'NONE',  ( 146.6084372240433993, -24.48358557860353457, 24.48358557860296258 ) ) ;
#9094=CARTESIAN_POINT ( 'NONE',  ( 192.4448373802100889, 2.472897170449861688E-13, -19.99999999996060751 ) ) ;
#9096=CARTESIAN_POINT ( 'NONE',  ( -199.9999999999999432, 5.435833037453086994E-13, -55.16984130226961724 ) ) ;
#9098=ORIENTED_EDGE ( 'NONE', *, *, #20796, .F. ) ;
#9099=CARTESIAN_POINT ( 'NONE',  ( 130.8568914410475372, 5.949712681206715814, 2.449293598294708485E-15 ) ) ;
#9100=FACE_OUTER_BOUND ( 'NONE', #21297, .T. ) ;
#9101=CARTESIAN_POINT ( 'NONE',  ( -77.55625318716886341, -15.17516088037291766, 16.12447834766487276 ) ) ;
#9102=CARTESIAN_POINT ( 'NONE',  ( -30.26275506840324070, -40.00000000000003553, 1.694272468446120117 ) ) ;
#9104=DIRECTION ( 'NONE',  ( -0.2259624731719848123, 0.000000000000000000, -0.9741360072998019870 ) ) ;
#9105=CARTESIAN_POINT ( 'NONE',  ( -62.72988123312369169, -10.50767649786947366, -25.36777511015252884 ) ) ;
#9106=CARTESIAN_POINT ( 'NONE',  ( 136.1360204305621266, 53.05693388239320285, -3.511608612530223716 ) ) ;
#9107=CARTESIAN_POINT ( 'NONE',  ( -77.58504660580179291, -17.50307030595003965, -13.57339709064347488 ) ) ;
#9108=CARTESIAN_POINT ( 'NONE',  ( -192.9588430854690273, -39.99999999999948841, -54.46834944098263520 ) ) ;
#9109=CARTESIAN_POINT ( 'NONE',  ( -208.1127848780265026, -10.60833733269537227, -10.60833733269551793 ) ) ;
#9110=CARTESIAN_POINT ( 'NONE',  ( -162.0762913951021176, -1.694272876828353702, -40.00000000000002132 ) ) ;
#9111=CARTESIAN_POINT ( 'NONE',  ( -56.48582580120558561, -21.81201906317785699, 21.81201906317761896 ) ) ;
#9112=CARTESIAN_POINT ( 'NONE',  ( 192.4448373802100889, 20.00000000003945644, 0.000000000000000000 ) ) ;
#9114=CARTESIAN_POINT ( 'NONE',  ( 146.6084372240433709, 40.00000000000017053, -34.62501878078291639 ) ) ;
#9116=CARTESIAN_POINT ( 'NONE',  ( 14.38125909742180752, 10.73282306404720465, 10.73282306404724018 ) ) ;
#9117=CARTESIAN_POINT ( 'NONE',  ( 19.06497207195980792, 54.19242893257844429, -40.00000000000002132 ) ) ;
#9119=CARTESIAN_POINT ( 'NONE',  ( 20.69615274314397624, -47.71500688527799383, 13.93598092273205680 ) ) ;
#9120=CARTESIAN_POINT ( 'NONE',  ( -105.3755690713226585, 18.24025645688350750, -40.00000000000002132 ) ) ;
#9122=CARTESIAN_POINT ( 'NONE',  ( 130.8568914410475088, -24.07718906446910623, 32.49135343045471558 ) ) ;
#9123=CARTESIAN_POINT ( 'NONE',  ( -280.0000000000000000, 1.839446121267387017E-14, -20.00000000000001421 ) ) ;
#9124=CARTESIAN_POINT ( 'NONE',  ( -82.24626550008051140, 20.00141108520265121, 2.782958274668472232 ) ) ;
#9125=CARTESIAN_POINT ( 'NONE',  ( -3.763361371728485061, -13.84281709279630945, -47.08953757622914083 ) ) ;
#9127=CARTESIAN_POINT ( 'NONE',  ( -192.9588430854690273, 66.79921049724377724, -10.23066800231904239 ) ) ;
#9128=CARTESIAN_POINT ( 'NONE',  ( -87.01506749150250641, -5.383071875687824637, -20.72654704132506609 ) ) ;
#9129=CARTESIAN_POINT ( 'NONE',  ( -192.9588430854689989, 10.23066800230756712, -10.23066800230735396 ) ) ;
#9130=CARTESIAN_POINT ( 'NONE',  ( 130.8568914410475372, 24.07718906447210472, 24.07718906447249907 ) ) ;
#9132=CARTESIAN_POINT ( 'NONE',  ( -105.3755690713226585, 43.67073346367970288, 12.89780903124427702 ) ) ;
#9133=CARTESIAN_POINT ( 'NONE',  ( -87.08883489501339170, 12.58611167335517855, -17.39766501532976761 ) ) ;
#9135=CARTESIAN_POINT ( 'NONE',  ( -56.48582580120559271, 6.472252184284121412, 6.472252184284244869 ) ) ;
#9136=CARTESIAN_POINT ( 'NONE',  ( -105.3755690713226585, -15.38646221621738164, -41.18208027870615240 ) ) ;
#9137=CARTESIAN_POINT ( 'NONE',  ( -238.4067589809705794, 0.6820004458491113475, -57.25054294077229144 ) ) ;
#9138=CARTESIAN_POINT ( 'NONE',  ( -238.4067589809705794, 0.9644942799825386714, 0.000000000000000000 ) ) ;
#9139=CARTESIAN_POINT ( 'NONE',  ( 14.38125909742180397, 67.30136555895953165, 10.73282306403583242 ) ) ;
#9140=ADVANCED_FACE ( 'NONE', ( #5147 ), #20652, .T. ) ;
#9141=CARTESIAN_POINT ( 'NONE',  ( -192.9588430854689989, -8.596193650988133061E-14, 14.46834944099969533 ) ) ;
#9142=CARTESIAN_POINT ( 'NONE',  ( -213.1075012329537230, -66.26714140136188291, -9.698598906438677503 ) ) ;
#9145=CARTESIAN_POINT ( 'NONE',  ( -144.0562564043591749, 29.54282788297669171, -14.68019405981451797 ) ) ;
#9146=ORIENTED_EDGE ( 'NONE', *, *, #8930, .F. ) ;
#9147=CARTESIAN_POINT ( 'NONE',  ( 163.1118516004056573, 9.006482792069629539, 9.006482792069634868 ) ) ;
#9149=CARTESIAN_POINT ( 'NONE',  ( 23.36462152322932440, 13.80148662728997699, 46.81175967489703282 ) ) ;
#9150=CARTESIAN_POINT ( 'NONE',  ( -39.81953879992323664, -32.18669035975747761, -16.38089232953674923 ) ) ;
#9151=ADVANCED_FACE ( 'NONE', ( #11493 ), #22198, .T. ) ;
#9154=CARTESIAN_POINT ( 'NONE',  ( -105.3239185089454395, 18.58330222739251525, 10.72756532555027853 ) ) ;
#9155=B_SPLINE_CURVE_WITH_KNOTS ( 'NONE', 3,
 ( #19271, #19651, #23403, #5178, #4920, #21278 ),
 .UNSPECIFIED., .F., .F.,
 ( 4, 2, 4 ),
 ( -0.0001050551439274930278, 0.04006586859758504843, 0.08023679233909759845 ),
 .UNSPECIFIED. ) ;
#9158=CARTESIAN_POINT ( 'NONE',  ( 23.48902902575118645, -23.31625887490708848, 42.82177761400734539 ) ) ;
#9159=CARTESIAN_POINT ( 'NONE',  ( 45.01779936580098962, 12.15764947728268019, -38.89115870269903752 ) ) ;
#9162=CARTESIAN_POINT ( 'NONE',  ( 184.8905102610680444, -41.77492675556007384, 14.79361573936348684 ) ) ;
#9163=CARTESIAN_POINT ( 'NONE',  ( -105.3755690713226727, 5.661656051307470077E-14, -21.75974354311649961 ) ) ;
#9164=CARTESIAN_POINT ( 'NONE',  ( 184.8905102610680444, 1.070102760522089011E-13, -20.92133201514444352 ) ) ;
#9165=CARTESIAN_POINT ( 'NONE',  ( 14.32711937312299177, 49.08922911798419619, -14.14294248749816596 ) ) ;
#9166=CARTESIAN_POINT ( 'NONE',  ( -208.1127848780264742, -55.00245453012676222, -2.449293598294708485E-15 ) ) ;
#9167=CARTESIAN_POINT ( 'NONE',  ( 21.25019396253522430, -18.04326867293554315, -43.56030393974957349 ) ) ;
#9168=CARTESIAN_POINT ( 'NONE',  ( 192.4448373802100889, 14.14213562375893574, -14.14213562375874922 ) ) ;
#9169=CARTESIAN_POINT ( 'NONE',  ( 192.4448373802101173, 20.00000000003945644, 40.00000000000002132 ) ) ;
#9171=CARTESIAN_POINT ( 'NONE',  ( -30.26275506840324070, -1.198031551616032919, 1.198031551616014712 ) ) ;
#9172=CARTESIAN_POINT ( 'NONE',  ( -91.56559293963836410, 40.00000000000019185, -17.32597176626768487 ) ) ;
#9173=CARTESIAN_POINT ( 'NONE',  ( -110.0563856372988596, 9.155970533494683039, -17.99047586673238541 ) ) ;
#9174=CARTESIAN_POINT ( 'NONE',  ( 14.38125909742181818, -39.99999999999986500, -15.17850393972675604 ) ) ;
#9175=CARTESIAN_POINT ( 'NONE',  ( -192.9588430854690273, -40.00000000000011369, 14.46834944099955855 ) ) ;
#9177=CARTESIAN_POINT ( 'NONE',  ( 130.1158308416293892, -29.33435477745536701, -12.15068759228604911 ) ) ;
#9179=CARTESIAN_POINT ( 'NONE',  ( -213.1075012329537230, 18.58567234101121102, 37.98287015391247223 ) ) ;
#9180=VERTEX_POINT ( 'NONE', #22908 ) ;
#9182=CARTESIAN_POINT ( 'NONE',  ( -4.037857402783659566, 43.00569567200389542, -23.44963359339821096 ) ) ;
#9183=CARTESIAN_POINT ( 'NONE',  ( -135.8532207217289738, 9.153146818113548022, 40.00000000000002132 ) ) ;
#9185=CARTESIAN_POINT ( 'NONE',  ( -199.9999999999998010, 49.28189405767604114, -14.17215463606931181 ) ) ;
#9189=CARTESIAN_POINT ( 'NONE',  ( -56.48582580120559271, 6.472252184284211118, -6.472252184284153387 ) ) ;
#9190=CARTESIAN_POINT ( 'NONE',  ( 98.29820294267319980, -18.47759065023120328, -7.653668647304143313 ) ) ;
#9192=ORIENTED_EDGE ( 'NONE', *, *, #18043, .T. ) ;
#9194=CARTESIAN_POINT ( 'NONE',  ( -188.7701069479165881, 13.85300054332491904, 47.15820909662593863 ) ) ;
#9196=CARTESIAN_POINT ( 'NONE',  ( 192.4448373802101173, -42.42640687122073473, 14.14213562370301780 ) ) ;
#9198=CARTESIAN_POINT ( 'NONE',  ( 192.4448373802100889, 1.051811698935164031E-13, -20.00000000003942091 ) ) ;
#9201=CARTESIAN_POINT ( 'NONE',  ( 163.1118516004056573, -40.00000000000027711, 27.26290988616830546 ) ) ;
#9202=CARTESIAN_POINT ( 'NONE',  ( 19.06497207195980792, 40.00000000000059686, -54.19242893257802507 ) ) ;
#9203=DIRECTION ( 'NONE',  ( 0.000000000000000000, 1.000000000000000000, 0.000000000000000000 ) ) ;
#9205=CARTESIAN_POINT ( 'NONE',  ( -259.2033419157646676, -49.83842185052031937, -6.730120644403796426 ) ) ;
#9206=CARTESIAN_POINT ( 'NONE',  ( 151.7948205124836250, 1.439163438361279259E-13, -33.23291073765553705 ) ) ;
#9207=CARTESIAN_POINT ( 'NONE',  ( -200.5022718138936852, 18.58571273880625085, 44.86987976039401360 ) ) ;
#9208=CARTESIAN_POINT ( 'NONE',  ( 151.0853911467767432, 29.06993079631213206, 12.04115959307993045 ) ) ;
#9209=CARTESIAN_POINT ( 'NONE',  ( -105.2054292635175727, 7.329160573984922335E-13, -21.49321519473985020 ) ) ;
#9211=CARTESIAN_POINT ( 'NONE',  ( -86.94888381181661430, -19.08739374733235650, 9.627065680632176381 ) ) ;
#9212=CARTESIAN_POINT ( 'NONE',  ( 200.0000000000000000, -14.14213562373106114, 42.42640687119278908 ) ) ;
#9213=CARTESIAN_POINT ( 'NONE',  ( -56.48582580120559982, -21.81201906317804173, 34.75652343174591152 ) ) ;
#9214=CARTESIAN_POINT ( 'NONE',  ( -114.4388184736417031, -8.352332320009672628, -20.16431396440397350 ) ) ;
#9216=VERTEX_POINT ( 'NONE', #6272 ) ;
#9217=CARTESIAN_POINT ( 'NONE',  ( -198.0356074513804572, 39.15871834505956173, -39.15871834505865223 ) ) ;
#9219=CIRCLE ( 'NONE', #23242, 15.00000000000000178 ) ;
#9223=CARTESIAN_POINT ( 'NONE',  ( -56.48582580120558561, -40.00000000000012790, 9.153146818113166105 ) ) ;
#9225=CARTESIAN_POINT ( 'NONE',  ( 5.009866156928164393, -44.71726210619349473, 24.71463403307577877 ) ) ;
#9227=VERTEX_POINT ( 'NONE', #14639 ) ;
#9228=CARTESIAN_POINT ( 'NONE',  ( -238.4067589809705794, 40.96449427990177128, 40.00000000000002132 ) ) ;
#9229=CARTESIAN_POINT ( 'NONE',  ( 199.9999999999999432, 14.14213562373113398, -14.14213562373094923 ) ) ;
#9231=CARTESIAN_POINT ( 'NONE',  ( 146.6084372240433709, 40.00000000000003553, 5.374981219217116468 ) ) ;
#9234=CARTESIAN_POINT ( 'NONE',  ( -77.84460141634575336, -19.81807444411877128, 9.302297467149831078 ) ) ;
#9235=CARTESIAN_POINT ( 'NONE',  ( -86.96347745069644475, 5.999880687339585546E-14, -21.75974354311649961 ) ) ;
#9238=CARTESIAN_POINT ( 'NONE',  ( -77.58456302900343360, 13.58506799361890671, 17.49509851286743611 ) ) ;
#9239=CARTESIAN_POINT ( 'NONE',  ( -100.7734535825088358, -16.03295912088728770, 16.03295912088687913 ) ) ;
#9240=CARTESIAN_POINT ( 'NONE',  ( 151.7948205124835681, 51.78348778862544322, -4.785054706298002891 ) ) ;
#9241=FACE_OUTER_BOUND ( 'NONE', #1108, .T. ) ;
#9242=CARTESIAN_POINT ( 'NONE',  ( -280.0000000000000000, 1.605030083646939673E-13, -20.00000000000001421 ) ) ;
#9243=CARTESIAN_POINT ( 'NONE',  ( 48.46046615278249448, 11.89583623203300888, 37.63122026539858211 ) ) ;
#9244=CARTESIAN_POINT ( 'NONE',  ( 151.7948205124836534, -6.767089262349000656, -40.00000000000002132 ) ) ;
#9245=ADVANCED_FACE ( 'NONE', ( #425 ), #13335, .T. ) ;
#9246=CARTESIAN_POINT ( 'NONE',  ( -213.1075012329537230, 18.58567234101121102, 37.98287015391247223 ) ) ;
#9247=CARTESIAN_POINT ( 'NONE',  ( -238.4067589809705794, -0.9644942799826263791, -40.00000000000002132 ) ) ;
#9248=CARTESIAN_POINT ( 'NONE',  ( -105.2110227778633487, 1.366831978265802938, 21.45666521040861241 ) ) ;
#9249=CARTESIAN_POINT ( 'NONE',  ( -162.0762913951021176, 39.99999999999998579, 1.694272876828463614 ) ) ;
#9250=CARTESIAN_POINT ( 'NONE',  ( -114.7706029183787848, 22.06581648165141374, -1.595391203485450271 ) ) ;
#9251=CARTESIAN_POINT ( 'NONE',  ( -91.56559293963834989, 12.25131212657480440, 12.25131212657486834 ) ) ;
#9252=CARTESIAN_POINT ( 'NONE',  ( 19.06497207195980792, 54.19242893257843718, 2.449293598294708485E-15 ) ) ;
#9255=CARTESIAN_POINT ( 'NONE',  ( 21.60666276257580876, -43.47550165075017503, 18.00814241471809751 ) ) ;
#9256=CARTESIAN_POINT ( 'NONE',  ( -105.3175882261743226, 18.50843658928782531, -10.85998092708147666 ) ) ;
#9257=CARTESIAN_POINT ( 'NONE',  ( -208.1127848780264742, 10.60833733270764867, 67.17687982763166588 ) ) ;
#9258=CARTESIAN_POINT ( 'NONE',  ( -162.0762913951020892, -3.568845385355699554E-14, 1.694272876828323948 ) ) ;
#9259=CARTESIAN_POINT ( 'NONE',  ( -82.23674992913811366, 20.20616381366022196, -1.119577663962783909 ) ) ;
#9260=CARTESIAN_POINT ( 'NONE',  ( -62.69292774213263897, 9.343531400584703661, -25.97703433367446380 ) ) ;
#9263=CARTESIAN_POINT ( 'NONE',  ( -77.61421004775742460, 3.464448011081117773, -21.81743058566524951 ) ) ;
#9264=CARTESIAN_POINT ( 'NONE',  ( 4.995406935893283773, 39.06748935135171052, 17.50105314357239195 ) ) ;
#9265=CARTESIAN_POINT ( 'NONE',  ( -280.0000000000000000, -14.14213562373088706, -14.14213562373108424 ) ) ;
#9266=CARTESIAN_POINT ( 'NONE',  ( -56.48582580120558561, 6.472252184283903809, 50.09629031063968796 ) ) ;
#9267=CARTESIAN_POINT ( 'NONE',  ( 146.6084372240433993, -24.48358557860353457, 24.48358557860296258 ) ) ;
#9268=CARTESIAN_POINT ( 'NONE',  ( 136.1360204305621551, 24.77266263493153176, -31.79587985999237887 ) ) ;
#9269=CARTESIAN_POINT ( 'NONE',  ( 19.06497207195981858, -10.03556273973377166, -66.60410523465827737 ) ) ;
#9270=CARTESIAN_POINT ( 'NONE',  ( -135.8532207217289738, -34.75652343174584757, -21.81201906317816253 ) ) ;
#9271=CARTESIAN_POINT ( 'NONE',  ( -208.1127848780264742, 10.60833733268383483, -67.17687982760675425 ) ) ;
#9272=CARTESIAN_POINT ( 'NONE',  ( -100.7734535825088358, -22.67402823373193499, 0.000000000000000000 ) ) ;
#9275=CARTESIAN_POINT ( 'NONE',  ( 19.06497207195981858, -38.31983398719641087, 18.24870850772724040 ) ) ;
#9276=CARTESIAN_POINT ( 'NONE',  ( -185.5190358318141932, 42.39054933786154322, -17.55874045218388346 ) ) ;
#9277=ORIENTED_EDGE ( 'NONE', *, *, #6868, .F. ) ;
#9278=CARTESIAN_POINT ( 'NONE',  ( 91.82158438592158234, 44.40256751092336884, -12.16597498400043342 ) ) ;
#9279=CARTESIAN_POINT ( 'NONE',  ( -190.1760717698577423, 23.85870456551995744, 43.55712811721888045 ) ) ;
#9280=CARTESIAN_POINT ( 'NONE',  ( 23.17367289774858108, 13.81211338457322846, 46.88342923877236501 ) ) ;
#9281=CARTESIAN_POINT ( 'NONE',  ( -87.13361725327072804, -21.49321519333431141, -3.542586001259484843E-15 ) ) ;
#9282=ORIENTED_EDGE ( 'NONE', *, *, #8487, .F. ) ;
#9283=CARTESIAN_POINT ( 'NONE',  ( -151.7004365447935754, -32.50163950444082417, 13.46261988216328120 ) ) ;
#9285=CARTESIAN_POINT ( 'NONE',  ( 22.33254948917040750, -17.93222939140373384, 43.29223140032068784 ) ) ;
#9286=AXIS2_PLACEMENT_3D ( 'NONE', #7227, #3501, #13474 ) ;
#9288=B_SPLINE_CURVE_WITH_KNOTS ( 'NONE', 3,
 ( #8813, #16924, #2295, #21055, #2840, #1472, #7193, #7570, #13316, #23436, #9575, #7443 ),
 .UNSPECIFIED., .F., .F.,
 ( 4, 2, 2, 2, 2, 4 ),
 ( 2.797157557069881010E-17, 0.005971652981263651967, 0.008957479471895464507, 0.01045039271721137121, 0.01119684933986928033, 0.01194330596252718944 ),
 .UNSPECIFIED. ) ;
#9289=CARTESIAN_POINT ( 'NONE',  ( 90.71510531247511722, 8.810647085256718469, -21.27078368625871718 ) ) ;
#9291=EDGE_CURVE ( 'NONE', #25465, #14912, #24666, .T. ) ;
#9292=CARTESIAN_POINT ( 'NONE',  ( -77.55640685876512919, -9.396736996787174904E-14, 22.13135000837103661 ) ) ;
#9293=CARTESIAN_POINT ( 'NONE',  ( 184.8905102610680444, 39.99999999999999289, 19.07866798485573057 ) ) ;
#9295=CARTESIAN_POINT ( 'NONE',  ( 7.340276806054842673, 49.28408872342602365, -14.17250878947606907 ) ) ;
#9296=CARTESIAN_POINT ( 'NONE',  ( -259.2033419157646676, -30.48217210827743884, -40.00000000000002132 ) ) ;
#9297=FACE_OUTER_BOUND ( 'NONE', #10936, .T. ) ;
#9300=CARTESIAN_POINT ( 'NONE',  ( -238.4067589809705794, -0.9644942799826263791, 40.00000000000002132 ) ) ;
#9301=CARTESIAN_POINT ( 'NONE',  ( -192.9588430854689989, -10.23066800230756890, 10.23066800230742501 ) ) ;
#9302=CARTESIAN_POINT ( 'NONE',  ( -213.1075012329537230, 40.00000000000012790, -13.71589010951869980 ) ) ;
#9303=CARTESIAN_POINT ( 'NONE',  ( -192.9588430854690273, -39.99999999999991473, -14.46834944100011633 ) ) ;
#9304=CARTESIAN_POINT ( 'NONE',  ( 110.0526450532112648, -22.72553370033782016, -9.413224270846754393 ) ) ;
#9305=EDGE_LOOP ( 'NONE', ( #23894, #12227, #19972, #9737 ) ) ;
#9307=CARTESIAN_POINT ( 'NONE',  ( -4.260882601030786532, 42.93997571557897430, -23.40615483283743714 ) ) ;
#9308=CARTESIAN_POINT ( 'NONE',  ( -192.9588430854690273, -54.46834944098226572, 40.00000000000002132 ) ) ;
#9310=CARTESIAN_POINT ( 'NONE',  ( -198.9234529669418521, 44.84148137680994495, -24.80620787425045393 ) ) ;
#9311=ORIENTED_EDGE ( 'NONE', *, *, #10302, .F. ) ;
#9312=ORIENTED_EDGE ( 'NONE', *, *, #22980, .T. ) ;
#9314=CARTESIAN_POINT ( 'NONE',  ( 137.0939645874030930, 12.56330697291270049, -30.33050608226187705 ) ) ;
#9315=AXIS2_PLACEMENT_3D ( 'NONE', #19681, #25823, #11189 ) ;
#9317=ORIENTED_EDGE ( 'NONE', *, *, #1264, .F. ) ;
#9320=CARTESIAN_POINT ( 'NONE',  ( -91.56559293963834989, 40.53558337403677569, -16.03295912088699993 ) ) ;
#9321=CARTESIAN_POINT ( 'NONE',  ( 170.0000000000000853, 9.369682556672316309, -22.62041470344884075 ) ) ;
#9322=CARTESIAN_POINT ( 'NONE',  ( -91.56559293963834989, 6.234561990864368500E-14, -22.67402823373191723 ) ) ;
#9323=CARTESIAN_POINT ( 'NONE',  ( 170.0000000000000000, 3.122849337825751958E-14, 0.000000000000000000 ) ) ;
#9324=DIRECTION ( 'NONE',  ( 9.935246354362821010E-15, 0.7071067811865517916, -0.7071067811865432429 ) ) ;
#9325=CARTESIAN_POINT ( 'NONE',  ( 98.29820294267314296, 18.47759065023127079, 7.653668647304075812 ) ) ;
#9326=CARTESIAN_POINT ( 'NONE',  ( -135.8532207217289738, -39.99999999999972289, -30.84685318188688541 ) ) ;
#9327=CARTESIAN_POINT ( 'NONE',  ( 151.7948205124836250, 1.012150473917908975E-13, -6.767089262349031742 ) ) ;
#9329=CARTESIAN_POINT ( 'NONE',  ( -198.0356074513804572, -10.87444709759729911, 10.87444709759714812 ) ) ;
#9330=CARTESIAN_POINT ( 'NONE',  ( 184.8905102610680444, 40.00000000000013500, -20.92133201514430141 ) ) ;
#9331=EDGE_CURVE ( 'NONE', #4727, #525, #16747, .T. ) ;
#9332=CARTESIAN_POINT ( 'NONE',  ( -192.9370391625440959, 24.26711063095210363, 44.11033075277109106 ) ) ;
#9333=CARTESIAN_POINT ( 'NONE',  ( 135.5356265174576151, 30.20731421070342293, 12.51227922893899525 ) ) ;
#9337=CARTESIAN_POINT ( 'NONE',  ( -77.72936527557085640, -19.09948130763599750, 10.88227939678934142 ) ) ;
#9338=CARTESIAN_POINT ( 'NONE',  ( 91.82158438592158234, -40.45024623143958564, 16.11829626348418998 ) ) ;
#9339=CARTESIAN_POINT ( 'NONE',  ( 163.1118516004056573, -37.29075403953166301, 19.27778845539196695 ) ) ;
#9340=CARTESIAN_POINT ( 'NONE',  ( -185.5190930960787057, -17.55874694108960199, -42.39056500338028854 ) ) ;
#9341=CARTESIAN_POINT ( 'NONE',  ( 8.517493242715987734, 24.85395068094660687, 44.90626920808405487 ) ) ;
#9343=CARTESIAN_POINT ( 'NONE',  ( 19.06497207195981147, 38.31983398719673772, -38.31983398719579981 ) ) ;
#9346=ORIENTED_EDGE ( 'NONE', *, *, #11744, .F. ) ;
#9347=CARTESIAN_POINT ( 'NONE',  ( 136.1360204305621551, -40.00000000000036238, 35.03383547441254109 ) ) ;
#9350=ORIENTED_EDGE ( 'NONE', *, *, #19871, .F. ) ;
#9351=CARTESIAN_POINT ( 'NONE',  ( -162.0762913951021176, -29.48230308784755493, -27.08623940707632372 ) ) ;
#9352=CARTESIAN_POINT ( 'NONE',  ( -208.1127848780264742, 39.99999999999992895, 15.00245453012683683 ) ) ;
#9353=CARTESIAN_POINT ( 'NONE',  ( -88.38011429825068888, -20.03522015641036447, -8.298859913963124058 ) ) ;
#9354=AXIS2_PLACEMENT_3D ( 'NONE', #20115, #14385, #5739 ) ;
#9356=CARTESIAN_POINT ( 'NONE',  ( -86.96347745069643054, -39.99999999999995737, -21.75974354311664527 ) ) ;
#9358=CARTESIAN_POINT ( 'NONE',  ( -82.23726319249655603, 14.28014421912408771, 14.28014421912425114 ) ) ;
#9359=CARTESIAN_POINT ( 'NONE',  ( -17.28139728231930405, -20.85871090883866685, -39.07633224428978025 ) ) ;
#9360=CARTESIAN_POINT ( 'NONE',  ( 57.59792236341147031, 30.00663442387720181, -26.56190807104661289 ) ) ;
#9361=CARTESIAN_POINT ( 'NONE',  ( -83.28983882461055543, -35.99236576815650324, -3.542586001259484843E-15 ) ) ;
#9362=CARTESIAN_POINT ( 'NONE',  ( -30.26275506840323359, -39.99999999999959499, -41.69427246844670520 ) ) ;
#9364=CARTESIAN_POINT ( 'NONE',  ( 192.4448373802101173, -19.99999999996057554, 40.00000000000002132 ) ) ;
#9365=CARTESIAN_POINT ( 'NONE',  ( 163.1118516004056573, -12.73709011382471878, -40.00000000000002132 ) ) ;
#9366=CARTESIAN_POINT ( 'NONE',  ( -135.8532207217289738, 6.472252184284186249, -6.472252184284142729 ) ) ;
#9367=CARTESIAN_POINT ( 'NONE',  ( 0.2972598230770129857, -54.33493731733936016, -40.00000000000002132 ) ) ;
#9369=DIRECTION ( 'NONE',  ( 0.2259624730582905916, 0.000000000000000000, -0.9741360073261747798 ) ) ;
#9371=CARTESIAN_POINT ( 'NONE',  ( -114.6557802242318616, 21.44605415401110093, 5.040599680926282744 ) ) ;
#9372=CARTESIAN_POINT ( 'NONE',  ( -30.26275506840323715, 29.48230279907789253, 29.48230279907799556 ) ) ;
#9373=CARTESIAN_POINT ( 'NONE',  ( -86.96347745069644475, 18.24025645688350750, -40.00000000000002132 ) ) ;
#9374=ORIENTED_EDGE ( 'NONE', *, *, #22018, .T. ) ;
#9375=CARTESIAN_POINT ( 'NONE',  ( 23.26364522860156825, -46.84987168986953776, 13.80713620122656948 ) ) ;
#9377=CARTESIAN_POINT ( 'NONE',  ( -83.21262154144250189, 33.12752917118434226, -13.72187187061452995 ) ) ;
#9378=CARTESIAN_POINT ( 'NONE',  ( 4.995406935893297096, 10.78321810387837232, 67.35176059880234334 ) ) ;
#9379=CARTESIAN_POINT ( 'NONE',  ( -56.48582580120559271, 2.158176344243877536E-14, -9.153146818113587102 ) ) ;
#9380=CARTESIAN_POINT ( 'NONE',  ( -77.81429512171635565, 20.74621013857194995, 7.173374844106962911 ) ) ;
#9383=CARTESIAN_POINT ( 'NONE',  ( -16.37606550795825200, 16.46709356870534435, -39.75508062650778385 ) ) ;
#9386=EDGE_CURVE ( 'NONE', #14641, #9227, #10713, .T. ) ;
#9387=CARTESIAN_POINT ( 'NONE',  ( -77.72936527556018405, -5.810439193549020942, -21.20030630601272748 ) ) ;
#9388=CARTESIAN_POINT ( 'NONE',  ( -86.96347745069644475, -15.38646221621807442, 15.38646221621768184 ) ) ;
#9389=CARTESIAN_POINT ( 'NONE',  ( 184.8905102610680444, 43.07788698682591644, -13.49065550809769221 ) ) ;
#9390=EDGE_CURVE ( 'NONE', #1078, #22053, #17341, .T. ) ;
#9391=CARTESIAN_POINT ( 'NONE',  ( -114.7711211671578724, 22.06863527409988990, -1.563052705007634158 ) ) ;
#9393=CARTESIAN_POINT ( 'NONE',  ( 19.06497207195980792, 18.24870850772790831, -38.31983398719609824 ) ) ;
#9394=CARTESIAN_POINT ( 'NONE',  ( -100.7734535825088500, 16.03295912088740494, -40.53558337403661938 ) ) ;
#9395=CARTESIAN_POINT ( 'NONE',  ( -86.96347745069644475, -15.38646221621738164, -41.18208027870615240 ) ) ;
#9396=CARTESIAN_POINT ( 'NONE',  ( 91.82158438592158234, 44.40256751092319121, 12.16597498400105515 ) ) ;
#9397=CARTESIAN_POINT ( 'NONE',  ( 91.82158438592158234, -17.20528682183298486, 0.000000000000000000 ) ) ;
#9400=CARTESIAN_POINT ( 'NONE',  ( -259.2033419157646676, 6.730120644403426944, 6.730120644403592145 ) ) ;
#9402=CARTESIAN_POINT ( 'NONE',  ( 136.1360204305621551, -35.03383547441293899, 40.00000000000002132 ) ) ;
#9403=B_SPLINE_CURVE_WITH_KNOTS ( 'NONE', 3,
 ( #14410, #8282, #18399, #24399, #176, #18262, #16408, #22412, #22276, #4320, #6292, #22671 ),
 .UNSPECIFIED., .F., .F.,
 ( 4, 2, 2, 2, 2, 4 ),
 ( 5.572756979560850756E-17, 0.004680202113613629415, 0.009360404227227203319, 0.01170050528403401152, 0.01404060634084081972, 0.01872080845445443439 ),
 .UNSPECIFIED. ) ;
#9404=ORIENTED_EDGE ( 'NONE', *, *, #14642, .T. ) ;
#9405=CARTESIAN_POINT ( 'NONE',  ( -280.0000000000000568, 14.14213562373097943, -42.42640687119285303 ) ) ;
#9407=CARTESIAN_POINT ( 'NONE',  ( 5.897475806298555945, 43.62364094500643574, 18.06950371951458578 ) ) ;
#9409=CARTESIAN_POINT ( 'NONE',  ( -4.810655158400459541, -42.93528531927712777, -17.78437748360806481 ) ) ;
#9410=ORIENTED_EDGE ( 'NONE', *, *, #2584, .F. ) ;
#9411=CARTESIAN_POINT ( 'NONE',  ( -188.3065677117048153, -46.99298756134898269, 13.82848612971595159 ) ) ;
#9413=CARTESIAN_POINT ( 'NONE',  ( 23.41418334855255523, -13.79799959793976960, 46.79369727367425469 ) ) ;
#9414=CARTESIAN_POINT ( 'NONE',  ( 60.28378959954358862, 10.93033916075795808, -33.17072922778727673 ) ) ;
#9417=CARTESIAN_POINT ( 'NONE',  ( 4.995406935893292655, 39.99999999999982947, 55.24977328856478209 ) ) ;
#9418=CARTESIAN_POINT ( 'NONE',  ( -105.3755690713226727, 5.661656051307470077E-14, -21.75974354311649961 ) ) ;
#9420=CARTESIAN_POINT ( 'NONE',  ( 14.38125909742182884, -55.17850393971007605, 40.00000000000002132 ) ) ;
#9421=CARTESIAN_POINT ( 'NONE',  ( -105.4741150117366431, -7.943527260727707429, 19.77569912956141707 ) ) ;
#9423=CARTESIAN_POINT ( 'NONE',  ( -198.0356074513804572, -15.37879056873074290, 0.000000000000000000 ) ) ;
#9424=CARTESIAN_POINT ( 'NONE',  ( 130.8568914410475088, 52.36146031193420924, 4.207082182989907437 ) ) ;
#9425=CARTESIAN_POINT ( 'NONE',  ( 163.1118516004056573, -27.26290988616869626, 0.000000000000000000 ) ) ;
#9426=CARTESIAN_POINT ( 'NONE',  ( -238.4067589809705794, 39.99999999999999289, -0.9644942799821634161 ) ) ;
#9427=CARTESIAN_POINT ( 'NONE',  ( -162.0762913951021176, -40.00000000000003553, -1.694272876828743168 ) ) ;
#9428=CARTESIAN_POINT ( 'NONE',  ( 98.66317599405236649, -18.61194787003555362, -7.709321229950748311 ) ) ;
#9429=ORIENTED_EDGE ( 'NONE', *, *, #18093, .F. ) ;
#9431=CARTESIAN_POINT ( 'NONE',  ( -3.993758944536740518, 43.01863922058846157, -23.45926997169882711 ) ) ;
#9432=CARTESIAN_POINT ( 'NONE',  ( -100.7734535825088500, -17.32597176626813251, 40.00000000000002132 ) ) ;
#9434=CARTESIAN_POINT ( 'NONE',  ( -188.3610564113338626, 43.02325945309135591, -23.46269903113386945 ) ) ;
#9442=ORIENTED_EDGE ( 'NONE', *, *, #26237, .F. ) ;
#9444=( BOUNDED_SURFACE ( )  B_SPLINE_SURFACE ( 3, 3, ( 
 ( #7316, #3589, #23557, #23807, #15308, #13820, #25570, #17310, #13563, #17430, #1219, #3465, #15430, #5211, #11435, #1471, #17682, #25824, #5589, #21435, #11694, #19819, #25441, #9707, #17812, #25958, #7701, #11831, #15812, #23938 ),
 ( #3208, #13315, #2132, #18351, #16492, #14096, #9175, #5987, #24216, #10108, #14225, #8103, #20224, #22225, #14489, #131, #11968, #2002, #1871, #8235, #26093, #24617, #18209, #3865, #4141, #22622, #6248, #12100, #14361, #10240 ),
 ( #16224, #12233, #24353, #26233, #6371, #6117, #22364, #4001, #8370, #15947, #22491, #12358, #9842, #24078, #5852, #4397, #18082, #19949, #20357, #13958, #4270, #16353, #24486, #20489, #2262, #10370, #7967, #17946, #18480, #16086 ),
 ( #7829, #22092, #20092, #1733, #261, #9974, #400, #20616, #6505, #24751, #8504, #14615, #16618, #22750, #10504, #12491, #2392, #18618, #13858, #15460, #17462, #5366, #17585, #7224, #9612, #15340, #23712, #17717, #23587, #13471 ),
 ( #3498, #1379, #25721, #21853, #21993, #11345, #15715, #5492, #21464, #11735, #19461, #5622, #7474, #1638, #3625, #25997, #21592, #19853, #9747, #25602, #11465, #15588, #3364, #9231, #13592, #1506, #17847, #11223, #21723, #11597 ),
 ( #3241, #19718, #1248, #23468, #9352, #19592, #9479, #25859, #7603, #5239, #23842, #13728, #1125, #7348, #7734, #15846, #23976, #19336, #5752, #17339, #25472, #13344, #25833, #11443, #1357, #7578, #23442, #9330, #15316, #7201 ),
 ( #11572, #17562, #13703, #15438, #17690, #23565, #17440, #13571, #13322, #15565, #9456, #7451, #9585, #7081, #11078, #5468, #5340, #1226, #5218, #13450, #3342, #21442, #21569, #25578, #9206, #15690, #11323, #19565, #3217, #23815 ) ),
 .UNSPECIFIED., .T., .F., .F. ) 
 B_SPLINE_SURFACE_WITH_KNOTS ( ( 4, 3, 4 ),
 ( 4, 2, 2, 2, 2, 2, 2, 2, 2, 2, 2, 2, 2, 2, 4 ),
 ( 0.000000000000000000, 0.5000000000000000000, 1.000000000000000000 ),
 ( 0.000000000000000000, 0.1357259735107005372, 0.1651108541090157700, 0.1944957347073310028, 0.3598804999793158710, 0.3867117631979620773, 0.4135430264166082281, 0.5789277916885930964, 0.6062785021374117456, 0.6336292125862302838, 0.8508620842112317728, 0.8814014469398914198, 0.9119408096685510667, 0.9559704048342755334, 1.000000000000000000 ),
 .UNSPECIFIED. ) 
 GEOMETRIC_REPRESENTATION_ITEM ( )  RATIONAL_B_SPLINE_SURFACE ( (
 ( 1.000000000000000000, 1.000000000000000000, 1.000000000000000000, 1.000000000000000000, 1.000000000000000000, 1.000000000000000000, 1.000000000000000000, 1.000000000000000000, 1.000000000000000000, 1.000000000000000000, 1.000000000000000000, 1.000000000000000000, 1.000000000000000000, 1.000000000000000000, 1.000000000000000000, 1.000000000000000000, 1.000000000000000000, 1.000000000000000000, 1.000000000000000000, 1.000000000000000000, 1.000000000000000000, 1.000000000000000000, 1.000000000000000000, 1.000000000000000000, 1.000000000000000000, 1.000000000000000000, 1.000000000000000000, 1.000000000000000000, 1.000000000000000000, 1.000000000000000000),
 ( 0.3333333333333333703, 0.3333333333333333703, 0.3333333333333333703, 0.3333333333333333703, 0.3333333333333333703, 0.3333333333333333703, 0.3333333333333333703, 0.3333333333333333703, 0.3333333333333333703, 0.3333333333333333703, 0.3333333333333333703, 0.3333333333333333703, 0.3333333333333333703, 0.3333333333333333703, 0.3333333333333333703, 0.3333333333333333703, 0.3333333333333333703, 0.3333333333333333703, 0.3333333333333333703, 0.3333333333333333703, 0.3333333333333333703, 0.3333333333333333703, 0.3333333333333333703, 0.3333333333333333703, 0.3333333333333333703, 0.3333333333333333703, 0.3333333333333333703, 0.3333333333333333703, 0.3333333333333333703, 0.3333333333333333703),
 ( 0.3333333333333333703, 0.3333333333333333703, 0.3333333333333333703, 0.3333333333333333703, 0.3333333333333333703, 0.3333333333333333703, 0.3333333333333333703, 0.3333333333333333703, 0.3333333333333333703, 0.3333333333333333703, 0.3333333333333333703, 0.3333333333333333703, 0.3333333333333333703, 0.3333333333333333703, 0.3333333333333333703, 0.3333333333333333703, 0.3333333333333333703, 0.3333333333333333703, 0.3333333333333333703, 0.3333333333333333703, 0.3333333333333333703, 0.3333333333333333703, 0.3333333333333333703, 0.3333333333333333703, 0.3333333333333333703, 0.3333333333333333703, 0.3333333333333333703, 0.3333333333333333703, 0.3333333333333333703, 0.3333333333333333703),
 ( 1.000000000000000000, 1.000000000000000000, 1.000000000000000000, 1.000000000000000000, 1.000000000000000000, 1.000000000000000000, 1.000000000000000000, 1.000000000000000000, 1.000000000000000000, 1.000000000000000000, 1.000000000000000000, 1.000000000000000000, 1.000000000000000000, 1.000000000000000000, 1.000000000000000000, 1.000000000000000000, 1.000000000000000000, 1.000000000000000000, 1.000000000000000000, 1.000000000000000000, 1.000000000000000000, 1.000000000000000000, 1.000000000000000000, 1.000000000000000000, 1.000000000000000000, 1.000000000000000000, 1.000000000000000000, 1.000000000000000000, 1.000000000000000000, 1.000000000000000000),
 ( 0.3333333333333333703, 0.3333333333333333703, 0.3333333333333333703, 0.3333333333333333703, 0.3333333333333333703, 0.3333333333333333703, 0.3333333333333333703, 0.3333333333333333703, 0.3333333333333333703, 0.3333333333333333703, 0.3333333333333333703, 0.3333333333333333703, 0.3333333333333333703, 0.3333333333333333703, 0.3333333333333333703, 0.3333333333333333703, 0.3333333333333333703, 0.3333333333333333703, 0.3333333333333333703, 0.3333333333333333703, 0.3333333333333333703, 0.3333333333333333703, 0.3333333333333333703, 0.3333333333333333703, 0.3333333333333333703, 0.3333333333333333703, 0.3333333333333333703, 0.3333333333333333703, 0.3333333333333333703, 0.3333333333333333703),
 ( 0.3333333333333333703, 0.3333333333333333703, 0.3333333333333333703, 0.3333333333333333703, 0.3333333333333333703, 0.3333333333333333703, 0.3333333333333333703, 0.3333333333333333703, 0.3333333333333333703, 0.3333333333333333703, 0.3333333333333333703, 0.3333333333333333703, 0.3333333333333333703, 0.3333333333333333703, 0.3333333333333333703, 0.3333333333333333703, 0.3333333333333333703, 0.3333333333333333703, 0.3333333333333333703, 0.3333333333333333703, 0.3333333333333333703, 0.3333333333333333703, 0.3333333333333333703, 0.3333333333333333703, 0.3333333333333333703, 0.3333333333333333703, 0.3333333333333333703, 0.3333333333333333703, 0.3333333333333333703, 0.3333333333333333703),
 ( 1.000000000000000000, 1.000000000000000000, 1.000000000000000000, 1.000000000000000000, 1.000000000000000000, 1.000000000000000000, 1.000000000000000000, 1.000000000000000000, 1.000000000000000000, 1.000000000000000000, 1.000000000000000000, 1.000000000000000000, 1.000000000000000000, 1.000000000000000000, 1.000000000000000000, 1.000000000000000000, 1.000000000000000000, 1.000000000000000000, 1.000000000000000000, 1.000000000000000000, 1.000000000000000000, 1.000000000000000000, 1.000000000000000000, 1.000000000000000000, 1.000000000000000000, 1.000000000000000000, 1.000000000000000000, 1.000000000000000000, 1.000000000000000000, 1.000000000000000000) ) ) 
 REPRESENTATION_ITEM ( '' )  SURFACE ( )  );
#9447=CARTESIAN_POINT ( 'NONE',  ( 146.6084372240433709, 32.08495691632064961, -24.48358557860320417 ) ) ;
#9448=CARTESIAN_POINT ( 'NONE',  ( -100.7734535825088358, 6.065416334915073333E-14, -22.67402823373191723 ) ) ;
#9449=CARTESIAN_POINT ( 'NONE',  ( -105.2054292635176580, -14.22820505692067528, -16.16779137048389003 ) ) ;
#9451=CARTESIAN_POINT ( 'NONE',  ( -280.0000000000000000, 1.839446121267387017E-14, -20.00000000000001421 ) ) ;
#9452=CARTESIAN_POINT ( 'NONE',  ( 19.06497207195981858, -39.99999999999987210, -14.19242893257882621 ) ) ;
#9453=CARTESIAN_POINT ( 'NONE',  ( -238.4067589809705794, -39.99999999999963762, -40.96449428006383187 ) ) ;
#9454=CARTESIAN_POINT ( 'NONE',  ( -105.2833435977022987, -11.73665196258528987, 17.94452063502825467 ) ) ;
#9455=CARTESIAN_POINT ( 'NONE',  ( 19.06497207195981858, -38.31983398719616218, -18.24870850772777331 ) ) ;
#9456=CARTESIAN_POINT ( 'NONE',  ( -100.7734535825088358, 6.065416334915073333E-14, -22.67402823373191723 ) ) ;
#9457=CARTESIAN_POINT ( 'NONE',  ( -105.3755690713226727, 15.38646221621793231, -15.38646221621779020 ) ) ;
#9458=CARTESIAN_POINT ( 'NONE',  ( 156.1979191798867532, 27.38417834433174036, 11.34289806466604134 ) ) ;
#9459=CARTESIAN_POINT ( 'NONE',  ( -77.58523997990521082, 17.50224656894025088, -13.57278374163336920 ) ) ;
#9460=CARTESIAN_POINT ( 'NONE',  ( -238.4067589809705794, -0.6820004457913680929, 0.6820004457913170226 ) ) ;
#9461=CARTESIAN_POINT ( 'NONE',  ( 184.8905102610680444, 1.070102760522089011E-13, -20.92133201514444352 ) ) ;
#9462=CARTESIAN_POINT ( 'NONE',  ( 163.1118516004056573, -47.56205970284957374, 9.006482792074162802 ) ) ;
#9463=CARTESIAN_POINT ( 'NONE',  ( -30.26275506840322649, -29.48230279907769358, -29.48230279907820162 ) ) ;
#9465=CARTESIAN_POINT ( 'NONE',  ( 3.854700064722247799, 24.62824689552012103, 44.60002223906890606 ) ) ;
#9467=CARTESIAN_POINT ( 'NONE',  ( 170.2234770963711128, 10.92277846919216522, -10.92277846919186501 ) ) ;
#9475=CARTESIAN_POINT ( 'NONE',  ( -47.65341557541689355, 14.80716566684846569, 29.74088027406873280 ) ) ;
#9478=CARTESIAN_POINT ( 'NONE',  ( 4.995406935893293543, -10.78321810389005364, 10.78321810388994173 ) ) ;
#9479=CARTESIAN_POINT ( 'NONE',  ( -192.9588430854690273, 39.99999999999992895, 14.46834944099983922 ) ) ;
#9481=EDGE_CURVE ( 'NONE', #15971, #23760, #25962, .T. ) ;
#9482=CARTESIAN_POINT ( 'NONE',  ( -86.86578273022543328, -19.68494377654098670, -8.153770686795214218 ) ) ;
#9484=CARTESIAN_POINT ( 'NONE',  ( -30.26275506840323359, -1.535832457777009877E-13, 41.69427246844629309 ) ) ;
#9486=CARTESIAN_POINT ( 'NONE',  ( 163.1118516004056573, 40.00000000000000711, 12.73709011382489642 ) ) ;
#9487=FACE_OUTER_BOUND ( 'NONE', #11308, .T. ) ;
#9488=CARTESIAN_POINT ( 'NONE',  ( -5.152948516943237856, -23.23217004668927643, -42.67688069069051693 ) ) ;
#9489=CARTESIAN_POINT ( 'NONE',  ( -259.2033419157646676, 35.01439189186559275, -21.55415060305807984 ) ) ;
#9490=CARTESIAN_POINT ( 'NONE',  ( -4.039451493210478361, -43.00522595893993838, -23.44932283416681429 ) ) ;
#9491=CARTESIAN_POINT ( 'NONE',  ( -198.0356074513804572, 1.247057299367198800E-13, -15.37879056873070560 ) ) ;
#9493=CARTESIAN_POINT ( 'NONE',  ( -238.4067589809705794, -0.9644942799826263791, 40.00000000000002132 ) ) ;
#9494=CARTESIAN_POINT ( 'NONE',  ( -198.0356074513804572, -55.37879056871328487, -40.00000000000002132 ) ) ;
#9495=CARTESIAN_POINT ( 'NONE',  ( -192.9588430854689989, -10.23066800230756890, 10.23066800230742501 ) ) ;
#9496=CARTESIAN_POINT ( 'NONE',  ( -213.1075012329537230, -13.71589010951915810, -40.00000000000002132 ) ) ;
#9497=CARTESIAN_POINT ( 'NONE',  ( 22.26816181513975224, -43.18156009806480000, -23.58015273002475354 ) ) ;
#9498=CARTESIAN_POINT ( 'NONE',  ( -80.82924211444361617, 19.36828989313945826, 8.022608353712277207 ) ) ;
#9500=CARTESIAN_POINT ( 'NONE',  ( 19.06497207195981147, 38.31983398719620482, 38.31983398719633271 ) ) ;
#9501=CARTESIAN_POINT ( 'NONE',  ( 151.7948205124836534, 6.767089262349056611, 40.00000000000002132 ) ) ;
#9503=CARTESIAN_POINT ( 'NONE',  ( 67.79414719533728828, -30.31905270963927279, 10.30785037361772005 ) ) ;
#9506=CARTESIAN_POINT ( 'NONE',  ( 200.0000000000000000, -42.42640687119293119, 14.14213562373082134 ) ) ;
#9507=CARTESIAN_POINT ( 'NONE',  ( -192.9588430854689989, -8.596193650988133061E-14, 14.46834944099969533 ) ) ;
#9508=CARTESIAN_POINT ( 'NONE',  ( -213.1075012329537230, 9.698598906450543566, -9.698598906450348167 ) ) ;
#9509=CARTESIAN_POINT ( 'NONE',  ( -198.0356074513804572, 15.37879056873066830, -40.00000000000002132 ) ) ;
#9512=CARTESIAN_POINT ( 'NONE',  ( -82.24297220888483650, -2.527436275905056817, -20.07419058344045126 ) ) ;
#9513=CARTESIAN_POINT ( 'NONE',  ( -91.56559293963834989, 12.25131212657428748, 44.31723036834913643 ) ) ;
#9514=CARTESIAN_POINT ( 'NONE',  ( 4.995406935893300648, -10.78321810387790514, -67.35176059880241439 ) ) ;
#9515=CARTESIAN_POINT ( 'NONE',  ( -199.9999999999999147, -14.17215463606695280, 49.28189405767609088 ) ) ;
#9516=CARTESIAN_POINT ( 'NONE',  ( -105.2054292635175585, -15.19799821370250825, 15.19799821370211923 ) ) ;
#9517=CARTESIAN_POINT ( 'NONE',  ( -259.2033419157646676, 6.730120644403918995, -49.83842185052024831 ) ) ;
#9518=CARTESIAN_POINT ( 'NONE',  ( 170.2234770963711128, 45.64576402573196390, -10.92277846919159856 ) ) ;
#9519=CARTESIAN_POINT ( 'NONE',  ( 146.6084372240433709, -52.76785682606510619, -3.800685668859292043 ) ) ;
#9520=CARTESIAN_POINT ( 'NONE',  ( -100.7734535825088358, -16.03295912088728770, 16.03295912088687913 ) ) ;
#9523=CARTESIAN_POINT ( 'NONE',  ( 200.0000000000000000, -39.99999999999991473, -20.00000000000024514 ) ) ;
#9525=CARTESIAN_POINT ( 'NONE',  ( -30.26275506840324425, 1.694272468446254232, 40.00000000000002132 ) ) ;
#9527=CARTESIAN_POINT ( 'NONE',  ( 200.0000000000000000, 14.14213562373100608, -42.42640687119291698 ) ) ;
#9528=CARTESIAN_POINT ( 'NONE',  ( -1.776459010276445705, 42.72191398789923511, 17.69599618432451393 ) ) ;
#9529=CARTESIAN_POINT ( 'NONE',  ( 44.82887508594575365, 18.94256811214892977, 36.15717056695527276 ) ) ;
#9530=CARTESIAN_POINT ( 'NONE',  ( -105.4288953903209318, -7.317865678924526662, 20.05883966466176815 ) ) ;
#9531=VERTEX_POINT ( 'NONE', #4601 ) ;
#9534=EDGE_CURVE ( 'NONE', #6406, #25369, #6883, .T. ) ;
#9535=CARTESIAN_POINT ( 'NONE',  ( 23.48902902575320795, -13.79248457098053215, 46.76665409567269194 ) ) ;
#9536=CARTESIAN_POINT ( 'NONE',  ( 16.03312633937180109, 18.43342098166968768, -44.50221493478129986 ) ) ;
#9538=( BOUNDED_CURVE ( )  B_SPLINE_CURVE ( 3, ( #628, #6469, #6597, #20581, #14583, #4489, #2355 ),
 .UNSPECIFIED., .F., .F. ) 
 B_SPLINE_CURVE_WITH_KNOTS ( ( 4, 3, 4 ),
 ( 0.007485919821752121811, 0.02392635744100474887, 0.04567102422631708070 ),
 .UNSPECIFIED. ) 
 CURVE ( )  GEOMETRIC_REPRESENTATION_ITEM ( )  RATIONAL_B_SPLINE_CURVE ( ( 0.5852718452494397594, 0.6660804010233953854, 0.8043231192735821322, 1.000000000000000000, 0.7411912828888134186, 0.5828554938567341859, 0.5249926329037621908 ) ) 
 REPRESENTATION_ITEM ( '' )  );
#9540=CARTESIAN_POINT ( 'NONE',  ( -77.58504658346102190, -2.778652059942609664, 21.97438119294674763 ) ) ;
#9541=CARTESIAN_POINT ( 'NONE',  ( -208.1127848780265026, -9.061048840815752106E-14, 15.00245453012669472 ) ) ;
#9542=CARTESIAN_POINT ( 'NONE',  ( 199.9999999999999432, 1.065690307512836407E-13, -20.00000000000010303 ) ) ;
#9544=CARTESIAN_POINT ( 'NONE',  ( 57.59792236341148453, -37.56421063658185489, 40.00000000000002132 ) ) ;
#9545=CARTESIAN_POINT ( 'NONE',  ( 98.29820294267327085, -7.653668647303853767, -18.47759065023127434 ) ) ;
#9547=CARTESIAN_POINT ( 'NONE',  ( 57.59792236341148453, -37.56421063658185489, 40.00000000000002132 ) ) ;
#9548=CARTESIAN_POINT ( 'NONE',  ( -100.7734535825088500, 22.67402823373189946, -40.00000000000002132 ) ) ;
#9549=CARTESIAN_POINT ( 'NONE',  ( -259.2033419157646676, -9.517827891722680178, 40.00000000000002132 ) ) ;
#9550=CARTESIAN_POINT ( 'NONE',  ( 14.38125909742181818, 5.830552384690105017E-13, -55.17850393972636880 ) ) ;
#9551=CARTESIAN_POINT ( 'NONE',  ( -213.1075012329537230, 1.045191102001431893E-13, -13.71589010951911902 ) ) ;
#9552=CARTESIAN_POINT ( 'NONE',  ( 4.995406935893293543, -10.78321810388990265, -10.78321810389009272 ) ) ;
#9553=EDGE_CURVE ( 'NONE', #7462, #10069, #26181, .T. ) ;
#9554=VERTEX_POINT ( 'NONE', #870 ) ;
#9555=CARTESIAN_POINT ( 'NONE',  ( -87.13361725327072804, 21.49321519333428299, -1.365653317446499981 ) ) ;
#9556=CARTESIAN_POINT ( 'NONE',  ( 0.2972598230769938343, 10.13633138497472252, 10.13633138497475628 ) ) ;
#9558=CARTESIAN_POINT ( 'NONE',  ( -190.6721449140022173, 47.76494005424142841, -13.94344083317845850 ) ) ;
#9562=CARTESIAN_POINT ( 'NONE',  ( -93.02511667906881598, 8.946512270084880925, -20.50052124204823656 ) ) ;
#9563=DIRECTION ( 'NONE',  ( -1.000000000000000000, -1.836970198721030181E-16, -0.000000000000000000 ) ) ;
#9565=CARTESIAN_POINT ( 'NONE',  ( -103.9663809735407369, -19.92521373251424777, 8.574562935515732676 ) ) ;
#9567=B_SPLINE_CURVE_WITH_KNOTS ( 'NONE', 3,
 ( #12911, #22505, #14372, #2810, #8916, #547 ),
 .UNSPECIFIED., .F., .F.,
 ( 4, 2, 4 ),
 ( -6.000000005839790033E-08, 0.03937727647058165970, 0.07875461294116338495 ),
 .UNSPECIFIED. ) ;
#9569=CIRCLE ( 'NONE', #10862, 15.00000000000000000 ) ;
#9571=CARTESIAN_POINT ( 'NONE',  ( -189.4799703873390797, 13.88847319136869096, 47.39666448643363594 ) ) ;
#9572=CARTESIAN_POINT ( 'NONE',  ( 184.8905102610680444, 41.77492675556005253, -14.79361573936377461 ) ) ;
#9574=CARTESIAN_POINT ( 'NONE',  ( 136.1360204305621266, 1.473277640373554421E-13, -35.03383547441296741 ) ) ;
#9575=CARTESIAN_POINT ( 'NONE',  ( -188.5332406156854006, -23.50029615566145580, 43.07394490461352632 ) ) ;
#9581=CARTESIAN_POINT ( 'NONE',  ( -184.9730489281052144, -45.83721239348559351, -13.59277546673601833 ) ) ;
#9582=CARTESIAN_POINT ( 'NONE',  ( -30.26275506840323359, -39.99999999999959499, -41.69427246844670520 ) ) ;
#9583=CARTESIAN_POINT ( 'NONE',  ( -105.2502192157150063, -17.39781795296958222, 12.58588914170264594 ) ) ;
#9584=CARTESIAN_POINT ( 'NONE',  ( -280.0000000000000568, -14.14213562373078226, -42.42640687119295251 ) ) ;
#9585=CARTESIAN_POINT ( 'NONE',  ( -86.96347745069644475, 5.999880687339585546E-14, -21.75974354311649961 ) ) ;
#9586=CARTESIAN_POINT ( 'NONE',  ( 170.2234770963711128, -39.20704971665379190, -17.36149277827012938 ) ) ;
#9588=CARTESIAN_POINT ( 'NONE',  ( -77.70077460412309733, 11.21025402036413965, -18.98542998413455507 ) ) ;
#9590=CARTESIAN_POINT ( 'NONE',  ( -105.3755690713226585, -39.99999999999996447, -21.75974354311664527 ) ) ;
#9591=CARTESIAN_POINT ( 'NONE',  ( -238.4067589809705794, 28.96627169325315165, 28.96627169325329731 ) ) ;
#9592=VECTOR ( 'NONE', #17529, 1000.000000000000000 ) ;
#9593=CARTESIAN_POINT ( 'NONE',  ( -56.48582580120558561, -50.09629031063971638, 6.472252184283745713 ) ) ;
#9594=CARTESIAN_POINT ( 'NONE',  ( -129.2920262389484662, -10.46331600572290199, -25.26067940852896854 ) ) ;
#9595=CARTESIAN_POINT ( 'NONE',  ( 170.2234770963711128, 17.36149277827004411, -17.36149277826983095 ) ) ;
#9597=CARTESIAN_POINT ( 'NONE',  ( 14.38125909742181108, 39.01709431150961649, -39.01709431150867147 ) ) ;
#9599=( BOUNDED_SURFACE ( )  B_SPLINE_SURFACE ( 3, 2, ( 
 ( #1501, #7344, #15456 ),
 ( #23583, #5360, #21588 ),
 ( #3359, #11461, #19585 ),
 ( #9475, #17581, #25717 ),
 ( #7469, #21715, #7598 ),
 ( #9606, #17711, #15710 ),
 ( #3620, #1633, #4033 ),
 ( #18112, #12133, #9872 ),
 ( #161, #17975, #10005 ),
 ( #22122, #24382, #22395 ),
 ( #26263, #15841, #6147 ),
 ( #15982, #5883, #23970 ),
 ( #8000, #14128, #16117 ),
 ( #24247, #19982, #21848 ),
 ( #6020, #16386, #18382 ),
 ( #3757, #11730, #12000 ),
 ( #5746, #19848, #9741 ),
 ( #17842, #16254, #8265 ),
 ( #22257, #25991, #26121 ),
 ( #20255, #11862, #7863 ),
 ( #1765, #2036, #7729 ),
 ( #13852, #21987, #27 ),
 ( #20122, #8138, #24111 ),
 ( #10138, #4171, #20390 ),
 ( #18242, #5617, #14257 ),
 ( #3901, #13723, #1900 ),
 ( #12265, #2164, #13990 ),
 ( #10274, #16520, #2289 ),
 ( #12519, #2556, #20786 ),
 ( #16652, #16779, #10672 ),
 ( #23395, #10398, #20649 ),
 ( #22651, #19393, #15266 ),
 ( #13275, #18646, #6667 ),
 ( #10533, #3170, #11273 ),
 ( #8670, #1047, #6277 ),
 ( #5171, #2700, #431 ),
 ( #12659, #14645, #17264 ),
 ( #24647, #18783, #8398 ),
 ( #6404, #14520, #12393 ),
 ( #19265, #21397, #8535 ),
 ( #7150, #4303, #18513 ),
 ( #1178, #24916, #9280 ),
 ( #566, #4426, #14392 ),
 ( #2424, #24782, #20518 ),
 ( #292, #6534, #9149 ),
 ( #22523, #14783, #22784 ),
 ( #4563, #4692, #22913 ),
 ( #12794, #20920, #10805 ),
 ( #25399, #24518, #19513 ),
 ( #25914, #15769, #13916 ),
 ( #19773, #23897, #7787 ),
 ( #5544, #17637, #21646 ),
 ( #23517, #23641, #15392 ),
 ( #5289, #13520, #3295 ),
 ( #5811, #15903, #19911 ),
 ( #25527, #13396, #17388 ),
 ( #9529, #13652, #19645 ),
 ( #11650, #1829, #22051 ),
 ( #7655, #15511, #11926 ),
 ( #17513, #3825, #11520 ),
 ( #5419, #3418, #20051 ),
 ( #1429, #1562, #25780 ) ),
 .UNSPECIFIED., .F., .F., .F. ) 
 B_SPLINE_SURFACE_WITH_KNOTS ( ( 4, 2, 2, 2, 2, 2, 2, 2, 2, 2, 2, 2, 2, 2, 2, 2, 2, 2, 2, 2, 2, 2, 2, 2, 2, 2, 2, 2, 2, 2, 4 ),
 ( 3, 3 ),
 ( 0.005118828937691504918, 0.02956064127318995538, 0.05400245360868840411, 0.07844426594418685283, 0.08149949248612416153, 0.08302710575709282281, 0.08379091239257714652, 0.08417281571031931531, 0.08436376736919039276, 0.08445924319862593843, 0.08450698111334370433, 0.08455471902806147022, 0.09066517211193608761, 0.09677562519581070499, 0.09983085173774799981, 0.1028860782796853085, 0.1089965313635599120, 0.1151069844474345294, 0.1181622109893718381, 0.1196898242603404994, 0.1204536308958248231, 0.1208355342135669919, 0.1208594031709258748, 0.1208832721282847578, 0.1209310100430025237, 0.1210264858724380693, 0.1212174375313091468, 0.1273278906151837642, 0.1517697029506822060, 0.1762115152861806755, 0.2006533276216791173 ),
 ( 0.000000000000000000, 1.000000000000000000 ),
 .UNSPECIFIED. ) 
 GEOMETRIC_REPRESENTATION_ITEM ( )  RATIONAL_B_SPLINE_SURFACE ( (
 ( 1.000000000000000000, 0.9997813423572993186, 1.000000000000000000),
 ( 1.000000000000000000, 0.9990919206322248503, 1.000000000000000000),
 ( 1.000000000000000000, 0.9967874177836960614, 1.000000000000000000),
 ( 1.000000000000000000, 0.9887544623284959533, 1.000000000000000000),
 ( 1.000000000000000000, 0.9830290792194851246, 1.000000000000000000),
 ( 1.000000000000000000, 0.9678345454226107147, 1.000000000000000000),
 ( 1.000000000000000000, 0.9583650305386990365, 1.000000000000000000),
 ( 1.000000000000000000, 0.9453335293273732454, 1.000000000000000000),
 ( 1.000000000000000000, 0.9438523872746359400, 1.000000000000000000),
 ( 1.000000000000000000, 0.9415799504611032100, 1.000000000000000000),
 ( 1.000000000000000000, 0.9408140170424519333, 1.000000000000000000),
 ( 1.000000000000000000, 0.9396523143998815053, 1.000000000000000000),
 ( 1.000000000000000000, 0.9392629463989758953, 1.000000000000000000),
 ( 1.000000000000000000, 0.9386756783045917540, 1.000000000000000000),
 ( 1.000000000000000000, 0.9384793862554625665, 1.000000000000000000),
 ( 1.000000000000000000, 0.9381841422087084936, 1.000000000000000000),
 ( 1.000000000000000000, 0.9380855931974712014, 1.000000000000000000),
 ( 1.000000000000000000, 0.9379375679425669965, 1.000000000000000000),
 ( 1.000000000000000000, 0.9378881925679130038, 1.000000000000000000),
 ( 1.000000000000000000, 0.9378140790407697436, 1.000000000000000000),
 ( 1.000000000000000000, 0.9377896949153108341, 1.000000000000000000),
 ( 1.000000000000000000, 0.9377409313169025040, 1.000000000000000000),
 ( 1.000000000000000000, 0.9377165729686793849, 1.000000000000000000),
 ( 1.000000000000000000, 0.9345773786259878868, 1.000000000000000000),
 ( 1.000000000000000000, 0.9318492984274234781, 1.000000000000000000),
 ( 1.000000000000000000, 0.9273872927429863688, 1.000000000000000000),
 ( 1.000000000000000000, 0.9256532593472229786, 1.000000000000000000),
 ( 1.000000000000000000, 0.9239357372750044428, 1.000000000000000000),
 ( 1.000000000000000000, 0.9235102113427005044, 1.000000000000000000),
 ( 1.000000000000000000, 0.9229728558029806074, 1.000000000000000000),
 ( 1.000000000000000000, 0.9228633126626633043, 1.000000000000000000),
 ( 1.000000000000000000, 0.9230139704736608497, 1.000000000000000000),
 ( 1.000000000000000000, 0.9237531682203802275, 1.000000000000000000),
 ( 1.000000000000000000, 0.9264156051930979574, 1.000000000000000000),
 ( 1.000000000000000000, 0.9283388455998493605, 1.000000000000000000),
 ( 1.000000000000000000, 0.9320050037531917297, 1.000000000000000000),
 ( 1.000000000000000000, 0.9333574575348343449, 1.000000000000000000),
 ( 1.000000000000000000, 0.9355411998009124375, 1.000000000000000000),
 ( 1.000000000000000000, 0.9362956009276801606, 1.000000000000000000),
 ( 1.000000000000000000, 0.9374637148015854127, 1.000000000000000000),
 ( 1.000000000000000000, 0.9378591705545192836, 1.000000000000000000),
 ( 1.000000000000000000, 0.9384610703419627997, 1.000000000000000000),
 ( 1.000000000000000000, 0.9386631562400347129, 1.000000000000000000),
 ( 1.000000000000000000, 0.9388793792114333847, 1.000000000000000000),
 ( 1.000000000000000000, 0.9388921037490437493, 1.000000000000000000),
 ( 1.000000000000000000, 0.9389175638858636708, 1.000000000000000000),
 ( 1.000000000000000000, 0.9389305010154682662, 1.000000000000000000),
 ( 1.000000000000000000, 0.9389691441647997072, 1.000000000000000000),
 ( 1.000000000000000000, 0.9389948969011567836, 1.000000000000000000),
 ( 1.000000000000000000, 0.9390721270299990930, 1.000000000000000000),
 ( 1.000000000000000000, 0.9391235763422390859, 1.000000000000000000),
 ( 1.000000000000000000, 0.9392778120326412683, 1.000000000000000000),
 ( 1.000000000000000000, 0.9393804861645803639, 1.000000000000000000),
 ( 1.000000000000000000, 0.9427638002345590795, 1.000000000000000000),
 ( 1.000000000000000000, 0.9458915987235437806, 1.000000000000000000),
 ( 1.000000000000000000, 0.9607963039197253696, 1.000000000000000000),
 ( 1.000000000000000000, 0.9703812854704935154, 1.000000000000000000),
 ( 1.000000000000000000, 0.9854660764538308859, 1.000000000000000000),
 ( 1.000000000000000000, 0.9909632567911316192, 1.000000000000000000),
 ( 1.000000000000000000, 0.9982308762617709830, 1.000000000000000000),
 ( 1.000000000000000000, 0.9999976772058264407, 1.000000000000000000),
 ( 1.000000000000000000, 1.000000000000000000, 1.000000000000000000) ) ) 
 REPRESENTATION_ITEM ( '' )  SURFACE ( )  );
#9601=CARTESIAN_POINT ( 'NONE',  ( 130.8568914410475088, -24.07718906446864793, -32.49135343045505664 ) ) ;
#9602=CARTESIAN_POINT ( 'NONE',  ( 98.29820294270304259, -18.47759065022024672, 7.653668647299475047 ) ) ;
#9604=CARTESIAN_POINT ( 'NONE',  ( 146.6084372240433993, -3.357462877844280890E-13, 34.62501878078305850 ) ) ;
#9605=CARTESIAN_POINT ( 'NONE',  ( 0.4311942631275967330, -24.25071831022400559, 44.08816696360413800 ) ) ;
#9606=CARTESIAN_POINT ( 'NONE',  ( -24.88648382770552203, 19.35593139208421931, 36.77569126514013931 ) ) ;
#9610=CARTESIAN_POINT ( 'NONE',  ( 170.2234770963711128, 15.44714144992819627, -40.00000000000002132 ) ) ;
#9611=CARTESIAN_POINT ( 'NONE',  ( -192.1964066538934617, -48.17614796929171916, -14.00508515769209339 ) ) ;
#9612=CARTESIAN_POINT ( 'NONE',  ( 151.7948205124836250, 1.807796684091926154E-15, 6.767089262349031742 ) ) ;
#9613=CARTESIAN_POINT ( 'NONE',  ( 85.88526014319977264, 8.769885380239042405, -23.37195137963415092 ) ) ;
#9616=CARTESIAN_POINT ( 'NONE',  ( -238.4067589809705794, -3.369206980223063916E-14, -0.9644942799825824142 ) ) ;
#9617=CARTESIAN_POINT ( 'NONE',  ( 170.2234770963711128, -39.99999999999991473, -24.55285855007201334 ) ) ;
#9619=CARTESIAN_POINT ( 'NONE',  ( 0.2972598230769957217, -4.999556039334937811E-14, 14.33493731733933352 ) ) ;
#9620=DIRECTION ( 'NONE',  ( 1.000000000000000000, 0.000000000000000000, 0.000000000000000000 ) ) ;
#9621=CARTESIAN_POINT ( 'NONE',  ( -4.339409867971390611, -17.83714383556709748, -43.06267456182897035 ) ) ;
#9622=EDGE_CURVE ( 'NONE', #19424, #961, #4338, .T. ) ;
#9623=CARTESIAN_POINT ( 'NONE',  ( 170.2234770963711128, 17.36149277826980253, 17.36149277827007253 ) ) ;
#9625=CARTESIAN_POINT ( 'NONE',  ( 19.06497207195981147, 1.521599808664285085E-13, -14.19242893257840521 ) ) ;
#9627=CARTESIAN_POINT ( 'NONE',  ( 192.4448373802101173, 20.00000000003945644, 40.00000000000002132 ) ) ;
#9628=CARTESIAN_POINT ( 'NONE',  ( -280.0000000000000000, -20.00000000000006750, -2.449293598294708485E-15 ) ) ;
#9630=EDGE_CURVE ( 'NONE', #12216, #12388, #8156, .T. ) ;
#9631=CARTESIAN_POINT ( 'NONE',  ( 0.2972598230769923355, 18.14793986248697166, 38.42060263243675422 ) ) ;
#9632=CARTESIAN_POINT ( 'NONE',  ( -198.0356074513804572, -15.37879056873074290, -40.00000000000002132 ) ) ;
#9634=CARTESIAN_POINT ( 'NONE',  ( 14.38125909742180397, 67.30136555895953165, 10.73282306403583242 ) ) ;
#9635=CARTESIAN_POINT ( 'NONE',  ( 130.8568914410475372, 5.949712681206715814, 2.449293598294708485E-15 ) ) ;
#9637=CARTESIAN_POINT ( 'NONE',  ( 22.80622392652957231, -43.16567765897927700, 17.87980911537442807 ) ) ;
#9638=CARTESIAN_POINT ( 'NONE',  ( 130.1167162091013836, 12.15076864148425528, 29.33455044752971119 ) ) ;
#9640=CARTESIAN_POINT ( 'NONE',  ( 200.0000000000000000, 42.42640687119288856, -14.14213562373094746 ) ) ;
#9641=CARTESIAN_POINT ( 'NONE',  ( 57.59792236341147742, -1.230234673553095937E-13, 37.56421063658186199 ) ) ;
#9642=CARTESIAN_POINT ( 'NONE',  ( -105.3755690713226585, 12.89780903124349720, 43.67073346367994446 ) ) ;
#9644=CARTESIAN_POINT ( 'NONE',  ( 192.4448373802101173, -20.00000000003938538, -40.00000000000002132 ) ) ;
#9645=CARTESIAN_POINT ( 'NONE',  ( -109.1264249741459906, -13.72187187124011132, -33.12752917269217079 ) ) ;
#9648=CARTESIAN_POINT ( 'NONE',  ( -105.3755690713226585, 12.89780903124349720, 43.67073346367994446 ) ) ;
#9649=CARTESIAN_POINT ( 'NONE',  ( -86.96347745069644475, -12.89780903124395195, -12.89780903124416511 ) ) ;
#9650=CARTESIAN_POINT ( 'NONE',  ( -77.90255099906769942, -20.29001641120677846, -8.064892378658084837 ) ) ;
#9651=CARTESIAN_POINT ( 'NONE',  ( -77.84504298474458039, 19.81984129313138965, -9.297284891551433006 ) ) ;
#9652=CARTESIAN_POINT ( 'NONE',  ( 136.1360204305621266, 53.05693388239320285, -3.511608612530223716 ) ) ;
#9653=CARTESIAN_POINT ( 'NONE',  ( -162.0762913951020892, -29.48230308784744125, -29.48230308784792442 ) ) ;
#9654=CARTESIAN_POINT ( 'NONE',  ( 170.2234770963711128, -17.36149277826940462, -39.20704971665412586 ) ) ;
#9655=CARTESIAN_POINT ( 'NONE',  ( -192.9588430854690273, -18.05360324515400094, -38.51493924976961836 ) ) ;
#9656=ADVANCED_FACE ( 'NONE', ( #8710, #17342 ), #14692, .T. ) ;
#9657=CARTESIAN_POINT ( 'NONE',  ( 170.2234770963711128, -24.55285855007183926, 0.000000000000000000 ) ) ;
#9658=CARTESIAN_POINT ( 'NONE',  ( 116.7964245048409424, 27.98274000340266809, 0.000000000000000000 ) ) ;
#9660=CARTESIAN_POINT ( 'NONE',  ( 19.06497207195982924, -40.00000000000021316, 54.19242893257830218 ) ) ;
#9661=CARTESIAN_POINT ( 'NONE',  ( 192.4448373802100889, -14.14213562370313682, 14.14213562370301958 ) ) ;
#9662=CARTESIAN_POINT ( 'NONE',  ( 146.6084372240433993, 24.48358557860307272, 24.48358557860347418 ) ) ;
#9663=CARTESIAN_POINT ( 'NONE',  ( -259.2033419157646676, 30.48217210827734647, 40.00000000000002132 ) ) ;
#9665=CARTESIAN_POINT ( 'NONE',  ( -135.8532207217289738, -6.472252184284190690, -6.472252184284188914 ) ) ;
#9666=CARTESIAN_POINT ( 'NONE',  ( -4.585253294881784569, 42.10505998758514323, 17.44048689139054176 ) ) ;
#9667=CARTESIAN_POINT ( 'NONE',  ( -65.65550967526353077, -9.107276986623745074, -24.89650881518310399 ) ) ;
#9668=CARTESIAN_POINT ( 'NONE',  ( -30.26275506840324070, 1.694272468446254232, 0.000000000000000000 ) ) ;
#9672=CARTESIAN_POINT ( 'NONE',  ( -3.921555385249984038, -23.47492146734913732, 43.03974577853593075 ) ) ;
#9673=CARTESIAN_POINT ( 'NONE',  ( 21.45050411888145092, 18.02367319545977153, -43.51299627226218547 ) ) ;
#9676=CARTESIAN_POINT ( 'NONE',  ( 163.1118516004056573, 40.00000000000000711, 12.73709011382489642 ) ) ;
#9677=CARTESIAN_POINT ( 'NONE',  ( -82.23726319241515625, -1.261450157158256591, 20.19517362732507593 ) ) ;
#9678=CARTESIAN_POINT ( 'NONE',  ( 151.7948205124836250, 4.785054706301759886, -4.785054706301612448 ) ) ;
#9679=CARTESIAN_POINT ( 'NONE',  ( -238.4067589809705794, -0.9644942799826263791, 40.00000000000002132 ) ) ;
#9680=CARTESIAN_POINT ( 'NONE',  ( -187.3037411062156821, 13.75782484034628439, -46.64555264106614629 ) ) ;
#9683=CARTESIAN_POINT ( 'NONE',  ( -105.3755690713226585, 21.75974354311648185, -40.00000000000002132 ) ) ;
#9684=CARTESIAN_POINT ( 'NONE',  ( -238.4067589809705794, 40.96449427990177128, 40.00000000000002132 ) ) ;
#9685=CARTESIAN_POINT ( 'NONE',  ( 57.59792236341147742, 4.064940816252731242E-13, -37.56421063658186199 ) ) ;
#9687=CARTESIAN_POINT ( 'NONE',  ( -162.0762913951021176, 27.08623940707639477, -29.48230308784743059 ) ) ;
#9694=ORIENTED_EDGE ( 'NONE', *, *, #14776, .T. ) ;
#9695=CARTESIAN_POINT ( 'NONE',  ( -56.48582580120559982, -21.81201906317755501, -34.75652343174621706 ) ) ;
#9696=CARTESIAN_POINT ( 'NONE',  ( 25.31597067610180929, -42.45761951829256020, -17.58652183052983276 ) ) ;
#9697=EDGE_LOOP ( 'NONE', ( #19878, #15663, #21048, #17832 ) ) ;
#9698=CARTESIAN_POINT ( 'NONE',  ( -105.3755690713226585, -21.75974354311652448, -40.00000000000002132 ) ) ;
#9703=( BOUNDED_SURFACE ( )  B_SPLINE_SURFACE ( 3, 2, ( 
 ( #21001, #21139, #25137 ),
 ( #4783, #3039, #19388 ),
 ( #12886, #25395, #17259 ),
 ( #9027, #1042, #9145 ),
 ( #15004, #651, #17131 ),
 ( #2654, #21393, #6758 ),
 ( #1174, #10759, #7146 ),
 ( #20871, #13271, #7014 ),
 ( #14870, #9276, #785 ),
 ( #23265, #10895, #23005 ),
 ( #8890, #15262, #13147 ),
 ( #5166, #8758, #15388 ),
 ( #12750, #3166, #5041 ),
 ( #4908, #23137, #17384 ),
 ( #915, #25523, #11269 ),
 ( #13019, #7271, #18871 ),
 ( #6888, #2914, #19132 ),
 ( #824, #25679, #15295 ),
 ( #25300, #13057, #9434 ),
 ( #13181, #3323, #15418 ),
 ( #25556, #21042, #2824 ),
 ( #25174, #25430, #1330 ),
 ( #23668, #17167, #10934 ),
 ( #7059, #6925, #21549 ),
 ( #21175, #17039, #23423 ),
 ( #2948, #3077, #15174 ),
 ( #11059, #3195, #17541 ),
 ( #19171, #7304, #23545 ),
 ( #17298, #19421, #1207 ),
 ( #19044, #5199, #15042 ),
 ( #7426, #8932, #12925 ),
 ( #23173, #13303, #5315 ),
 ( #21422, #11303, #9310 ),
 ( #23299, #19544, #15540 ) ),
 .UNSPECIFIED., .F., .F., .T. ) 
 B_SPLINE_SURFACE_WITH_KNOTS ( ( 4, 2, 2, 2, 2, 2, 2, 2, 2, 2, 2, 2, 2, 2, 2, 2, 4 ),
 ( 3, 3 ),
 ( 0.005135432767691730169, 0.02907015807668714841, 0.05300488338568256491, 0.07693960869467798835, 0.08292329002192683207, 0.08441921035373904647, 0.08446595786410818207, 0.08448933161929274294, 0.08451270537447730380, 0.08460620039521557501, 0.08479319043669208966, 0.08516717051964514673, 0.08591513068555126087, 0.08890697134917568967, 0.09189881201280011846, 0.09489065267642454726, 0.1008743340036734049 ),
 ( 0.000000000000000000, 1.000000000000000000 ),
 .UNSPECIFIED. ) 
 GEOMETRIC_REPRESENTATION_ITEM ( )  RATIONAL_B_SPLINE_SURFACE ( (
 ( 1.000000000000000000, 0.9997813423552075474, 1.000000000000000000),
 ( 1.000000000000000000, 0.9991063898506410412, 1.000000000000000000),
 ( 1.000000000000000000, 0.9968824705949623777, 1.000000000000000000),
 ( 1.000000000000000000, 0.9891556793369797873, 1.000000000000000000),
 ( 1.000000000000000000, 0.9836552277522164767, 1.000000000000000000),
 ( 1.000000000000000000, 0.9690805015303910475, 1.000000000000000000),
 ( 1.000000000000000000, 0.9600094330325482650, 1.000000000000000000),
 ( 1.000000000000000000, 0.9461485276691540269, 1.000000000000000000),
 ( 1.000000000000000000, 0.9432497373317602074, 1.000000000000000000),
 ( 1.000000000000000000, 0.9394620364518225797, 1.000000000000000000),
 ( 1.000000000000000000, 0.9386962831138920826, 1.000000000000000000),
 ( 1.000000000000000000, 0.9378980481303054173, 1.000000000000000000),
 ( 1.000000000000000000, 0.9378738510928928962, 1.000000000000000000),
 ( 1.000000000000000000, 0.9378375433852950138, 1.000000000000000000),
 ( 1.000000000000000000, 0.9378253334781229134, 1.000000000000000000),
 ( 1.000000000000000000, 0.9378014123365953081, 1.000000000000000000),
 ( 1.000000000000000000, 0.9377894572438933984, 1.000000000000000000),
 ( 1.000000000000000000, 0.9377297092068141993, 1.000000000000000000),
 ( 1.000000000000000000, 0.9376819985415375536, 1.000000000000000000),
 ( 1.000000000000000000, 0.9375391312191778681, 1.000000000000000000),
 ( 1.000000000000000000, 0.9374442392361990173, 1.000000000000000000),
 ( 1.000000000000000000, 0.9371606329892131493, 1.000000000000000000),
 ( 1.000000000000000000, 0.9369729884417210553, 1.000000000000000000),
 ( 1.000000000000000000, 0.9364144211479206170, 1.000000000000000000),
 ( 1.000000000000000000, 0.9360478649889876213, 1.000000000000000000),
 ( 1.000000000000000000, 0.9342453465011781866, 1.000000000000000000),
 ( 1.000000000000000000, 0.9329002455190741339, 1.000000000000000000),
 ( 1.000000000000000000, 0.9304321598238819435, 1.000000000000000000),
 ( 1.000000000000000000, 0.9293115443288706423, 1.000000000000000000),
 ( 1.000000000000000000, 0.9273348408774886309, 1.000000000000000000),
 ( 1.000000000000000000, 0.9264755133099957796, 1.000000000000000000),
 ( 1.000000000000000000, 0.9243017816395038277, 1.000000000000000000),
 ( 1.000000000000000000, 0.9233922826853561139, 1.000000000000000000),
 ( 1.000000000000000000, 0.9230541040372001182, 1.000000000000000000) ) ) 
 REPRESENTATION_ITEM ( '' )  SURFACE ( )  );
#9704=CARTESIAN_POINT ( 'NONE',  ( -198.0012400611979047, 14.15884001207450460, 49.19397081476446942 ) ) ;
#9705=CARTESIAN_POINT ( 'NONE',  ( 4.995406935893290878, 39.06748935135185263, 39.06748935135198764 ) ) ;
#9706=CARTESIAN_POINT ( 'NONE',  ( -105.3841228958018092, -6.698390573547676752, -20.33918053570303641 ) ) ;
#9707=CARTESIAN_POINT ( 'NONE',  ( 146.6084372240433993, 1.478241399363601114E-13, -34.62501878078305850 ) ) ;
#9708=CARTESIAN_POINT ( 'NONE',  ( -162.0762913951021176, 1.694272876828294194, 40.00000000000002132 ) ) ;
#9711=EDGE_CURVE ( 'NONE', #17072, #5580, #7736, .T. ) ;
#9713=CARTESIAN_POINT ( 'NONE',  ( 0.2972598230769957217, 1.502051041545559470E-13, -14.33493731733933352 ) ) ;
#9714=CARTESIAN_POINT ( 'NONE',  ( -198.0356074513804572, 1.247057299367198800E-13, -15.37879056873070560 ) ) ;
#9715=CARTESIAN_POINT ( 'NONE',  ( -200.0000000000000000, -45.34857661735436807, -20.90527768611926263 ) ) ;
#9716=CARTESIAN_POINT ( 'NONE',  ( 200.0000000000000000, -14.14213562373062949, -42.42640687119301646 ) ) ;
#9717=CARTESIAN_POINT ( 'NONE',  ( -238.4067589809705794, -40.96449427990185654, -40.00000000000002132 ) ) ;
#9719=CARTESIAN_POINT ( 'NONE',  ( -238.4067589809705794, -28.96627169325313389, -27.60227080167074831 ) ) ;
#9723=CARTESIAN_POINT ( 'NONE',  ( -77.84460141634585284, 19.81807444411913011, -9.302297467148907373 ) ) ;
#9724=CARTESIAN_POINT ( 'NONE',  ( 130.8568914410475372, -3.326198072800416995E-13, 34.05028731879788495 ) ) ;
#9725=CARTESIAN_POINT ( 'NONE',  ( 91.82158438592158234, 7.693928927950222250E-14, -17.20528682183300262 ) ) ;
#9726=CARTESIAN_POINT ( 'NONE',  ( 200.0000000000000000, -42.42640687119293119, 14.14213562373082134 ) ) ;
#9727=CARTESIAN_POINT ( 'NONE',  ( -208.1127848780265026, -10.60833733269537227, -10.60833733269551793 ) ) ;
#9728=CARTESIAN_POINT ( 'NONE',  ( -197.4153392275570411, -14.14666332906662660, -49.11379398047656508 ) ) ;
#9729=CARTESIAN_POINT ( 'NONE',  ( 14.38125909742181285, -10.73282306404727393, 10.73282306404716380 ) ) ;
#9731=CARTESIAN_POINT ( 'NONE',  ( -198.0356074513804572, 10.87444709761036066, -67.44298959253325165 ) ) ;
#9732=CARTESIAN_POINT ( 'NONE',  ( -91.56559293963836410, 16.03295912088714203, -16.03295912088699282 ) ) ;
#9733=CARTESIAN_POINT ( 'NONE',  ( -100.7734535825088500, 22.67402823373189946, -40.00000000000002132 ) ) ;
#9734=CARTESIAN_POINT ( 'NONE',  ( -105.4741150117367283, 19.77569912955882359, -7.943527260733686646 ) ) ;
#9735=CARTESIAN_POINT ( 'NONE',  ( 14.38125909742181285, -17.55144818341421598, -39.01709431150935359 ) ) ;
#9736=CARTESIAN_POINT ( 'NONE',  ( -199.9999999999999716, -49.28189405767602693, 14.17215463606940595 ) ) ;
#9737=ORIENTED_EDGE ( 'NONE', *, *, #10945, .F. ) ;
#9738=CARTESIAN_POINT ( 'NONE',  ( -30.26275506840324070, -40.00000000000001421, -1.694272468446678559 ) ) ;
#9739=CARTESIAN_POINT ( 'NONE',  ( 14.33519843538167571, -24.71012982060716823, 44.71104701565639772 ) ) ;
#9740=B_SPLINE_CURVE_WITH_KNOTS ( 'NONE', 3,
 ( #15353, #17857, #7744, #26008, #3509, #11879, #21862, #15856, #13482, #25734 ),
 .UNSPECIFIED., .F., .F.,
 ( 4, 2, 2, 2, 4 ),
 ( 0.7921542097164070428, 0.8508620842112317728, 0.8814014469398914198, 0.9119408096685510667, 0.9406682828396426554 ),
 .UNSPECIFIED. ) ;
#9741=CARTESIAN_POINT ( 'NONE',  ( -4.201409602820307398, 13.81669219312490249, 46.93439176590543127 ) ) ;
#9745=CARTESIAN_POINT ( 'NONE',  ( 0.2972598230769930017, 54.33493731733938148, -40.00000000000002132 ) ) ;
#9746=CARTESIAN_POINT ( 'NONE',  ( -194.4222169613592257, -48.65437996130108900, -14.07715596671970815 ) ) ;
#9747=CARTESIAN_POINT ( 'NONE',  ( 19.06497207195980792, 39.99999999999983658, 54.19242893257857929 ) ) ;
#9749=CARTESIAN_POINT ( 'NONE',  ( 200.0000000000000000, 7.347880794884121511E-14, 0.000000000000000000 ) ) ;
#9751=CARTESIAN_POINT ( 'NONE',  ( 163.1118516004056573, -2.556006622855449647E-13, 27.26290988616872824 ) ) ;
#9752=DIRECTION ( 'NONE',  ( 0.01051738792036862290, -0.3995761383050656090, -0.9166396752533372272 ) ) ;
#9753=CARTESIAN_POINT ( 'NONE',  ( -190.6136434985683934, 42.75828627302750107, 17.71106207812097111 ) ) ;
#9754=CARTESIAN_POINT ( 'NONE',  ( 3.774039766387189854, -18.47898247163652741, -44.61221010187593805 ) ) ;
#9755=CARTESIAN_POINT ( 'NONE',  ( 146.6084372240433709, -32.08495691632075619, 24.48358557860298035 ) ) ;
#9756=( BOUNDED_SURFACE ( )  B_SPLINE_SURFACE ( 3, 3, ( 
 ( #20235, #5, #2141, #25969, #3598, #24362, #16095, #20101, #26101, #6000, #22236, #13966, #14106, #18092, #1743, #18361, #3875, #24226, #5860, #10252, #17821, #6126, #14234, #11706, #7709, #15820, #6257, #19959, #140, #9982 ),
 ( #4011, #10118, #21828, #22374, #26242, #11977, #16362, #18219, #8117, #8244, #4150, #23948, #24496, #5725, #7977, #3736, #13829, #21962, #12110, #7838, #2015, #16233, #11839, #15961, #24086, #19827, #9851, #22101, #12244, #20367 ),
 ( #17954, #1613, #9717, #808, #10918, #22890, #12772, #19029, #8512, #20764, #409, #18626, #4540, #8649, #2534, #14624, #16630, #8914, #20899, #6381, #22761, #22630, #2677, #20498, #17023, #12637, #24625, #24891, #25159, #673 ),
 ( #24760, #6646, #14760, #6513, #4670, #10651, #20626, #14370, #18761, #16757, #544, #2807, #10378, #16895, #6780, #4280, #18489, #270, #22502, #12499, #12370, #10783, #8378, #8782, #18894, #25027, #14892, #23032, #4807, #2401 ),
 ( #12909, #2270, #21025, #16500, #14499, #4405, #10512, #1063, #19660, #6910, #13414, #11291, #23157, #19411, #13042, #25543, #23412, #21412, #17530, #9547, #7042, #11410, #1195, #17152, #7414, #15159, #1316, #3185, #23657, #25668 ),
 ( #15528, #5437, #9300, #25286, #23285, #13538, #4932, #17404, #23533, #21664, #17655, #13291, #7294, #21160, #3313, #2934, #15408, #5061, #13167, #5304, #21287, #11043, #3061, #15282, #19280, #21538, #19532, #938, #9169, #11164 ),
 ( #17283, #25416, #7166, #15027, #5189, #9423, #3437, #11536, #1447, #19153, #9047, #24187, #22336, #19926, #5829, #11806, #3701, #15920, #20068, #13931, #26066, #1709, #20331, #5961, #17788, #7804, #7674, #14071, #5563, #4111 ) ),
 .UNSPECIFIED., .T., .F., .F. ) 
 B_SPLINE_SURFACE_WITH_KNOTS ( ( 4, 3, 4 ),
 ( 4, 2, 2, 2, 2, 2, 2, 2, 2, 2, 2, 2, 2, 2, 4 ),
 ( 0.000000000000000000, 0.5000000000000000000, 1.000000000000000000 ),
 ( 0.000000000000000000, 0.1357259735107005372, 0.1651108541090157700, 0.1944957347073310028, 0.3598804999793158710, 0.3867117631979620773, 0.4135430264166082281, 0.5789277916885930964, 0.6062785021374117456, 0.6336292125862302838, 0.8508620842112317728, 0.8814014469398914198, 0.9119408096685510667, 0.9559704048342755334, 1.000000000000000000 ),
 .UNSPECIFIED. ) 
 GEOMETRIC_REPRESENTATION_ITEM ( )  RATIONAL_B_SPLINE_SURFACE ( (
 ( 1.000000000000000000, 1.000000000000000000, 1.000000000000000000, 1.000000000000000000, 1.000000000000000000, 1.000000000000000000, 1.000000000000000000, 1.000000000000000000, 1.000000000000000000, 1.000000000000000000, 1.000000000000000000, 1.000000000000000000, 1.000000000000000000, 1.000000000000000000, 1.000000000000000000, 1.000000000000000000, 1.000000000000000000, 1.000000000000000000, 1.000000000000000000, 1.000000000000000000, 1.000000000000000000, 1.000000000000000000, 1.000000000000000000, 1.000000000000000000, 1.000000000000000000, 1.000000000000000000, 1.000000000000000000, 1.000000000000000000, 1.000000000000000000, 1.000000000000000000),
 ( 0.3333333333333333703, 0.3333333333333333703, 0.3333333333333333703, 0.3333333333333333703, 0.3333333333333333703, 0.3333333333333333703, 0.3333333333333333703, 0.3333333333333333703, 0.3333333333333333703, 0.3333333333333333703, 0.3333333333333333703, 0.3333333333333333703, 0.3333333333333333703, 0.3333333333333333703, 0.3333333333333333703, 0.3333333333333333703, 0.3333333333333333703, 0.3333333333333333703, 0.3333333333333333703, 0.3333333333333333703, 0.3333333333333333703, 0.3333333333333333703, 0.3333333333333333703, 0.3333333333333333703, 0.3333333333333333703, 0.3333333333333333703, 0.3333333333333333703, 0.3333333333333333703, 0.3333333333333333703, 0.3333333333333333703),
 ( 0.3333333333333333703, 0.3333333333333333703, 0.3333333333333333703, 0.3333333333333333703, 0.3333333333333333703, 0.3333333333333333703, 0.3333333333333333703, 0.3333333333333333703, 0.3333333333333333703, 0.3333333333333333703, 0.3333333333333333703, 0.3333333333333333703, 0.3333333333333333703, 0.3333333333333333703, 0.3333333333333333703, 0.3333333333333333703, 0.3333333333333333703, 0.3333333333333333703, 0.3333333333333333703, 0.3333333333333333703, 0.3333333333333333703, 0.3333333333333333703, 0.3333333333333333703, 0.3333333333333333703, 0.3333333333333333703, 0.3333333333333333703, 0.3333333333333333703, 0.3333333333333333703, 0.3333333333333333703, 0.3333333333333333703),
 ( 1.000000000000000000, 1.000000000000000000, 1.000000000000000000, 1.000000000000000000, 1.000000000000000000, 1.000000000000000000, 1.000000000000000000, 1.000000000000000000, 1.000000000000000000, 1.000000000000000000, 1.000000000000000000, 1.000000000000000000, 1.000000000000000000, 1.000000000000000000, 1.000000000000000000, 1.000000000000000000, 1.000000000000000000, 1.000000000000000000, 1.000000000000000000, 1.000000000000000000, 1.000000000000000000, 1.000000000000000000, 1.000000000000000000, 1.000000000000000000, 1.000000000000000000, 1.000000000000000000, 1.000000000000000000, 1.000000000000000000, 1.000000000000000000, 1.000000000000000000),
 ( 0.3333333333333333703, 0.3333333333333333703, 0.3333333333333333703, 0.3333333333333333703, 0.3333333333333333703, 0.3333333333333333703, 0.3333333333333333703, 0.3333333333333333703, 0.3333333333333333703, 0.3333333333333333703, 0.3333333333333333703, 0.3333333333333333703, 0.3333333333333333703, 0.3333333333333333703, 0.3333333333333333703, 0.3333333333333333703, 0.3333333333333333703, 0.3333333333333333703, 0.3333333333333333703, 0.3333333333333333703, 0.3333333333333333703, 0.3333333333333333703, 0.3333333333333333703, 0.3333333333333333703, 0.3333333333333333703, 0.3333333333333333703, 0.3333333333333333703, 0.3333333333333333703, 0.3333333333333333703, 0.3333333333333333703),
 ( 0.3333333333333333703, 0.3333333333333333703, 0.3333333333333333703, 0.3333333333333333703, 0.3333333333333333703, 0.3333333333333333703, 0.3333333333333333703, 0.3333333333333333703, 0.3333333333333333703, 0.3333333333333333703, 0.3333333333333333703, 0.3333333333333333703, 0.3333333333333333703, 0.3333333333333333703, 0.3333333333333333703, 0.3333333333333333703, 0.3333333333333333703, 0.3333333333333333703, 0.3333333333333333703, 0.3333333333333333703, 0.3333333333333333703, 0.3333333333333333703, 0.3333333333333333703, 0.3333333333333333703, 0.3333333333333333703, 0.3333333333333333703, 0.3333333333333333703, 0.3333333333333333703, 0.3333333333333333703, 0.3333333333333333703),
 ( 1.000000000000000000, 1.000000000000000000, 1.000000000000000000, 1.000000000000000000, 1.000000000000000000, 1.000000000000000000, 1.000000000000000000, 1.000000000000000000, 1.000000000000000000, 1.000000000000000000, 1.000000000000000000, 1.000000000000000000, 1.000000000000000000, 1.000000000000000000, 1.000000000000000000, 1.000000000000000000, 1.000000000000000000, 1.000000000000000000, 1.000000000000000000, 1.000000000000000000, 1.000000000000000000, 1.000000000000000000, 1.000000000000000000, 1.000000000000000000, 1.000000000000000000, 1.000000000000000000, 1.000000000000000000, 1.000000000000000000, 1.000000000000000000, 1.000000000000000000) ) ) 
 REPRESENTATION_ITEM ( '' )  SURFACE ( )  );
#9757=CARTESIAN_POINT ( 'NONE',  ( -77.55640685876511498, -22.13135000837103661, -4.964495286674871776E-15 ) ) ;
#9758=CARTESIAN_POINT ( 'NONE',  ( -162.0762913951020892, -29.48230308784785692, 29.48230308784751230 ) ) ;
#9759=CARTESIAN_POINT ( 'NONE',  ( -198.0356074513804572, -39.99999999999990052, -15.37879056873112482 ) ) ;
#9760=CARTESIAN_POINT ( 'NONE',  ( 170.0000000000000000, -24.95097643316997704, 0.000000000000000000 ) ) ;
#9761=CARTESIAN_POINT ( 'NONE',  ( -135.8532207217289738, 6.472252184284096543, 6.472252184284234211 ) ) ;
#9762=CARTESIAN_POINT ( 'NONE',  ( 0.2972598230770130412, -54.33493731733936016, -2.449293598294708485E-15 ) ) ;
#9763=CARTESIAN_POINT ( 'NONE',  ( 91.82158438592159655, 12.16597498400028776, 44.40256751092339016 ) ) ;
#9764=CARTESIAN_POINT ( 'NONE',  ( 14.38125909742182884, -55.17850393972636169, -2.449293598294708485E-15 ) ) ;
#9765=CARTESIAN_POINT ( 'NONE',  ( 23.37394308801980713, -42.85717664514568526, -23.33966569535099822 ) ) ;
#9766=CARTESIAN_POINT ( 'NONE',  ( -114.7799951756084482, 22.11694418166576526, 1.588013269880939271 ) ) ;
#9767=CARTESIAN_POINT ( 'NONE',  ( 146.6084372240433709, -24.48358557860329299, 32.08495691632052882 ) ) ;
#9768=CARTESIAN_POINT ( 'NONE',  ( -135.8532207217289738, -9.153146818113595984, -40.00000000000002132 ) ) ;
#9771=CARTESIAN_POINT ( 'NONE',  ( 27.55177309529049268, -41.56868263114476747, 22.48880744267832199 ) ) ;
#9772=CARTESIAN_POINT ( 'NONE',  ( 125.5832160019861021, 11.61997419108361385, 28.05309928654009610 ) ) ;
#9773=CARTESIAN_POINT ( 'NONE',  ( 170.2234770963711128, 10.92277846919210660, -45.64576402573182889 ) ) ;
#9774=CARTESIAN_POINT ( 'NONE',  ( 163.1118516004056573, -39.99999999999990052, -27.26290988616886679 ) ) ;
#9775=CARTESIAN_POINT ( 'NONE',  ( 192.4448373802100889, -14.14213562375896061, 14.14213562375865330 ) ) ;
#9776=EDGE_CURVE ( 'NONE', #8569, #17668, #6744, .T. ) ;
#9777=CARTESIAN_POINT ( 'NONE',  ( 170.2234770963711128, -24.55285855007183926, 0.000000000000000000 ) ) ;
#9778=CARTESIAN_POINT ( 'NONE',  ( 0.2972598230769930572, 14.33493731733933352, 0.000000000000000000 ) ) ;
#9781=CARTESIAN_POINT ( 'NONE',  ( 170.2234770963711128, 39.20704971665372796, 17.36149277827039583 ) ) ;
#9782=CARTESIAN_POINT ( 'NONE',  ( 57.59792236341147031, 30.00663442387720181, -26.56190807104661289 ) ) ;
#9783=CARTESIAN_POINT ( 'NONE',  ( 14.38125909742181285, -10.73282306404727393, 10.73282306404716380 ) ) ;
#9784=CARTESIAN_POINT ( 'NONE',  ( -192.9588430854689989, 1.161019517985663313E-13, -14.46834944099969533 ) ) ;
#9785=CARTESIAN_POINT ( 'NONE',  ( -135.8532207217289738, -21.81201906317757633, -21.81201906317793515 ) ) ;
#9786=CARTESIAN_POINT ( 'NONE',  ( 130.8568914410475088, 52.36146031193427319, -4.207082182989173802 ) ) ;
#9787=CARTESIAN_POINT ( 'NONE',  ( 184.8905102610680444, -14.79361573936399665, 14.79361573936367158 ) ) ;
#9788=CARTESIAN_POINT ( 'NONE',  ( -30.26275506840324070, -27.08623969584554558, -29.48230279907826912 ) ) ;
#9789=CARTESIAN_POINT ( 'NONE',  ( -192.9588430854689989, -10.23066800230756890, 10.23066800230742501 ) ) ;
#9792=CARTESIAN_POINT ( 'NONE',  ( -105.3755690713226585, -39.99999999999996447, -21.75974354311664527 ) ) ;
#9793=CARTESIAN_POINT ( 'NONE',  ( 130.8568914410475372, -4.207082182992846420, 4.207082182992822439 ) ) ;
#9795=CARTESIAN_POINT ( 'NONE',  ( -213.1075012329537230, 53.71589010953660193, 40.00000000000002132 ) ) ;
#9797=CARTESIAN_POINT ( 'NONE',  ( 163.1118516004056573, 9.006482792074356425, -47.56205970284957374 ) ) ;
#9801=CARTESIAN_POINT ( 'NONE',  ( -100.7734535825088358, -22.67402823373193499, 0.000000000000000000 ) ) ;
#9803=CARTESIAN_POINT ( 'NONE',  ( -195.1686598214593289, -44.46432177479800174, 24.52826087131761668 ) ) ;
#9805=CARTESIAN_POINT ( 'NONE',  ( 9.349823541318809106, -18.59402391555502376, 44.88994471603710679 ) ) ;
#9808=B_SPLINE_CURVE_WITH_KNOTS ( 'NONE', 3,
 ( #10519, #10923, #14631, #22768, #22510, #12506 ),
 .UNSPECIFIED., .F., .F.,
 ( 4, 2, 4 ),
 ( -5.999999999808750012E-08, 0.04017169446089190188, 0.08034344892178379993 ),
 .UNSPECIFIED. ) ;
#9809=CARTESIAN_POINT ( 'NONE',  ( 16.38602454699985955, 14.09104119328187821, -48.74566733939354179 ) ) ;
#9812=CARTESIAN_POINT ( 'NONE',  ( -114.4364955367301775, -8.064892380834896457, 20.29001642039033371 ) ) ;
#9813=CARTESIAN_POINT ( 'NONE',  ( 184.8905102610680444, 13.49065550809826952, -13.49065550809790359 ) ) ;
#9814=CARTESIAN_POINT ( 'NONE',  ( 163.1118516004056573, -12.73709011382472589, 40.00000000000002132 ) ) ;
#9818=CARTESIAN_POINT ( 'NONE',  ( 98.29820294273291381, -18.47759065023123526, -7.653668647304108674 ) ) ;
#9819=CARTESIAN_POINT ( 'NONE',  ( 184.8905102610680444, 20.92133201514447549, 0.000000000000000000 ) ) ;
#9821=CARTESIAN_POINT ( 'NONE',  ( -105.3755690713226727, -21.75974354311652093, 0.000000000000000000 ) ) ;
#9822=CARTESIAN_POINT ( 'NONE',  ( -30.26275506840323359, 4.336144384597734078E-13, -41.69427246844629309 ) ) ;
#9823=CARTESIAN_POINT ( 'NONE',  ( 192.4448373802101173, -40.00000000000019185, 20.00000000003900524 ) ) ;
#9824=CARTESIAN_POINT ( 'NONE',  ( -208.1127848780264742, 17.67593391476678377, -38.89260858015718014 ) ) ;
#9827=CARTESIAN_POINT ( 'NONE',  ( -30.26275506840324070, -1.694272468446265112, 0.000000000000000000 ) ) ;
#9831=CARTESIAN_POINT ( 'NONE',  ( 0.2972598230770153171, -66.70487387989861361, 10.13633138497438324 ) ) ;
#9832=CARTESIAN_POINT ( 'NONE',  ( 23.13330272892113371, -43.07356808498585821, -17.84165608060053998 ) ) ;
#9833=VERTEX_POINT ( 'NONE', #11468 ) ;
#9834=CARTESIAN_POINT ( 'NONE',  ( -192.9588430854690273, 54.46834944098218756, -40.00000000000002132 ) ) ;
#9836=ORIENTED_EDGE ( 'NONE', *, *, #16711, .F. ) ;
#9840=CARTESIAN_POINT ( 'NONE',  ( 199.9999999999999432, 14.14213562373090838, 14.14213562373092437 ) ) ;
#9841=CARTESIAN_POINT ( 'NONE',  ( -188.4265466358331196, -47.03621809928752384, -13.83489705870362840 ) ) ;
#9842=CARTESIAN_POINT ( 'NONE',  ( -86.96347745069643054, -40.00000000000009948, 18.24025645688337960 ) ) ;
#9843=CARTESIAN_POINT ( 'NONE',  ( -213.1075012329537230, 13.71589010951907817, 40.00000000000002132 ) ) ;
#9847=CARTESIAN_POINT ( 'NONE',  ( 130.8568914410475372, 1.429239637432775288E-13, -34.05028731879788495 ) ) ;
#9848=CARTESIAN_POINT ( 'NONE',  ( -259.2033419157646676, -40.00000000000017053, 9.517827891722212996 ) ) ;
#9849=CARTESIAN_POINT ( 'NONE',  ( -110.1018001840479599, -14.72021915946409543, 13.84057942000516128 ) ) ;
#9850=CARTESIAN_POINT ( 'NONE',  ( -213.1075012329537230, -9.698598906438496314, 66.26714140136188291 ) ) ;
#9851=CARTESIAN_POINT ( 'NONE',  ( 170.2234770963711128, 24.55285855007190676, -40.00000000000002132 ) ) ;
#9852=CARTESIAN_POINT ( 'NONE',  ( -56.48582580120558561, -50.09629031063963112, -6.472252184284449150 ) ) ;
#9854=CARTESIAN_POINT ( 'NONE',  ( 22.40986519363269025, -47.15972762675173868, 13.85314893102521161 ) ) ;
#9855=CARTESIAN_POINT ( 'NONE',  ( -135.8532207217289738, 39.99999999999990763, 9.153146818113990335 ) ) ;
#9856=CARTESIAN_POINT ( 'NONE',  ( 19.06497207195981858, -40.00000000000007105, 14.19242893257826665 ) ) ;
#9857=CARTESIAN_POINT ( 'NONE',  ( 14.38125909742180397, 67.30136555895953165, 10.73282306403583242 ) ) ;
#9859=CARTESIAN_POINT ( 'NONE',  ( 192.4448373802101173, -14.14213562370342281, 42.42640687122062104 ) ) ;
#9860=CARTESIAN_POINT ( 'NONE',  ( -190.7346372395638241, -23.92885340725213439, -43.65255821760446509 ) ) ;
#9861=CARTESIAN_POINT ( 'NONE',  ( -213.1075012329537230, -9.698598906450557777, 9.698598906450415669 ) ) ;
#9862=ORIENTED_EDGE ( 'NONE', *, *, #16291, .T. ) ;
#9863=CARTESIAN_POINT ( 'NONE',  ( -91.56559293963834989, -16.03295912088728414, 16.03295912088688269 ) ) ;
#9864=CARTESIAN_POINT ( 'NONE',  ( -192.9588430854689989, -10.23066800230756890, 10.23066800230742501 ) ) ;
#9865=CARTESIAN_POINT ( 'NONE',  ( -213.1075012329537230, -13.71589010951915810, 0.000000000000000000 ) ) ;
#9867=CARTESIAN_POINT ( 'NONE',  ( -280.0000000000000568, -42.42640687119276066, -14.14213562373147148 ) ) ;
#9868=CARTESIAN_POINT ( 'NONE',  ( -82.30220482034381746, 7.441767004347251024, 18.74474319041271997 ) ) ;
#9871=CARTESIAN_POINT ( 'NONE',  ( 85.88498484994616433, -8.769905298562015616, -23.37206192994392140 ) ) ;
#9872=CARTESIAN_POINT ( 'NONE',  ( -8.720657192110643052, 13.49580954686805079, 45.36528685023045426 ) ) ;
#9873=VERTEX_POINT ( 'NONE', #1382 ) ;
#9875=CARTESIAN_POINT ( 'NONE',  ( 4.995406935893289102, 10.78321810388998081, 10.78321810389001811 ) ) ;
#9878=CARTESIAN_POINT ( 'NONE',  ( -88.37877758186448318, -19.92653024483028190, -8.575405934408012243 ) ) ;
#9881=CARTESIAN_POINT ( 'NONE',  ( 19.06497207195981147, 1.521599808664285085E-13, -14.19242893257840521 ) ) ;
#9882=FACE_OUTER_BOUND ( 'NONE', #6622, .T. ) ;
#9886=CARTESIAN_POINT ( 'NONE',  ( -151.7004365449059264, 13.46261988209483640, 32.50163950446889061 ) ) ;
#9887=CARTESIAN_POINT ( 'NONE',  ( 6.615221834219322083, -14.16446777330033768, -49.23097633541950557 ) ) ;
#9888=CARTESIAN_POINT ( 'NONE',  ( 151.7948205124836534, 23.49921654116056047, -33.06932595376338213 ) ) ;
#9890=CARTESIAN_POINT ( 'NONE',  ( -91.56559293963834989, -40.53558337403669753, -16.03295912088728770 ) ) ;
#9891=CARTESIAN_POINT ( 'NONE',  ( -86.96347745069644475, -2.438961472018186339E-13, 21.75974354311649961 ) ) ;
#9892=CARTESIAN_POINT ( 'NONE',  ( -238.4067589809705794, 0.6820004457912851592, -0.6820004457913123597 ) ) ;
#9893=CARTESIAN_POINT ( 'NONE',  ( -208.1127848780264742, 17.67593391476678377, -38.89260858015718014 ) ) ;
#9894=CARTESIAN_POINT ( 'NONE',  ( 57.59792236341148453, -37.56421063658185489, -2.449293598294708485E-15 ) ) ;
#9895=FACE_OUTER_BOUND ( 'NONE', #20949, .T. ) ;
#9896=CARTESIAN_POINT ( 'NONE',  ( -213.1075012329537230, -53.71589010950170717, 40.00000000000002132 ) ) ;
#9897=CARTESIAN_POINT ( 'NONE',  ( -102.4068193528148072, 20.44188272012841878, -8.088405365069068154 ) ) ;
#9898=CARTESIAN_POINT ( 'NONE',  ( 0.2972598230769883387, 40.00000000000017053, -14.33493731733891607 ) ) ;
#9899=CARTESIAN_POINT ( 'NONE',  ( -56.48582580120559982, 21.81201906317778594, -34.75652343174606074 ) ) ;
#9900=CARTESIAN_POINT ( 'NONE',  ( 0.2972598230769930572, 14.33493731733933352, 0.000000000000000000 ) ) ;
#9901=ORIENTED_EDGE ( 'NONE', *, *, #16818, .T. ) ;
#9902=CARTESIAN_POINT ( 'NONE',  ( 27.55177309528321317, -45.29548561697026088, 13.49150912998325325 ) ) ;
#9904=CARTESIAN_POINT ( 'NONE',  ( -259.2033419157646676, 21.55415060305839958, -35.01439189186541512 ) ) ;
#9905=CARTESIAN_POINT ( 'NONE',  ( -208.1127848780264742, -40.00000000000025580, 55.00245453014408525 ) ) ;
#9906=CARTESIAN_POINT ( 'NONE',  ( 0.2972598230769886718, 38.42060263243643448, 18.14793986248763957 ) ) ;
#9908=CARTESIAN_POINT ( 'NONE',  ( 57.59792236341147031, 37.56421063658187620, -40.00000000000002132 ) ) ;
#9912=CARTESIAN_POINT ( 'NONE',  ( 4.995406935893286438, 67.35176059880245703, -10.78321810387767066 ) ) ;
#9913=CARTESIAN_POINT ( 'NONE',  ( -198.0356074513804572, -67.44298959253333692, -10.87444709761016348 ) ) ;
#9914=CARTESIAN_POINT ( 'NONE',  ( -188.2995950289364941, -46.99046209955528042, 13.82811170417144453 ) ) ;
#9915=CARTESIAN_POINT ( 'NONE',  ( -77.67315633212002979, 18.60060890640625075, -11.80559230994880515 ) ) ;
#9916=CARTESIAN_POINT ( 'NONE',  ( 151.7948205124836250, -4.785054706301600902, -4.785054706301715477 ) ) ;
#9917=CARTESIAN_POINT ( 'NONE',  ( 57.59792236341148453, -26.56190807104663421, -26.56190807104710672 ) ) ;
#9919=CARTESIAN_POINT ( 'NONE',  ( 57.59792236341147031, -30.00663442387662627, -26.56190807104723461 ) ) ;
#9920=CARTESIAN_POINT ( 'NONE',  ( -280.0000000000000000, 14.14213562373098299, -14.14213562373088706 ) ) ;
#9923=CARTESIAN_POINT ( 'NONE',  ( 91.82158438592159655, -39.99999999999994316, -17.20528682183314118 ) ) ;
#9924=CARTESIAN_POINT ( 'NONE',  ( 184.8905102610680444, 43.07788698682572459, 13.49065550809829439 ) ) ;
#9925=CARTESIAN_POINT ( 'NONE',  ( -208.1127848780265026, -10.60833733269537227, -10.60833733269551793 ) ) ;
#9926=CARTESIAN_POINT ( 'NONE',  ( 9.006212071484325676, 49.32687279761466215, -14.17897189021863902 ) ) ;
#9927=CARTESIAN_POINT ( 'NONE',  ( 184.8905102610680444, -20.92133201514440799, 40.00000000000002132 ) ) ;
#9928=ORIENTED_EDGE ( 'NONE', *, *, #20307, .F. ) ;
#9930=CARTESIAN_POINT ( 'NONE',  ( -5.983078567328675490, 41.77006127201591568, 17.30172588002420753 ) ) ;
#9934=CARTESIAN_POINT ( 'NONE',  ( -189.0540043421004270, -43.34487664254536554, 17.95403576473164264 ) ) ;
#9936=CARTESIAN_POINT ( 'NONE',  ( 16.03312633940209153, -18.43342098164813336, 44.50221493480265877 ) ) ;
#9937=CARTESIAN_POINT ( 'NONE',  ( 22.75882399337413986, 17.88527043150909890, -43.17886244245817551 ) ) ;
#9940=LINE ( 'NONE', #22197, #10568 ) ;
#9942=CARTESIAN_POINT ( 'NONE',  ( -105.3755690713226585, 41.18208027870575449, 15.38646221621837107 ) ) ;
#9943=CARTESIAN_POINT ( 'NONE',  ( 130.8568914410475088, -5.949712681206671405, 40.00000000000002132 ) ) ;
#9944=CARTESIAN_POINT ( 'NONE',  ( -188.9001659262682722, 17.93767091109533496, -43.30536839095024959 ) ) ;
#9945=CARTESIAN_POINT ( 'NONE',  ( -30.26275506840325136, 29.48230279907760121, 27.08623969584625613 ) ) ;
#9948=CARTESIAN_POINT ( 'NONE',  ( -30.26275506840324425, -1.694272468446265334, -40.00000000000002132 ) ) ;
#9949=CARTESIAN_POINT ( 'NONE',  ( 199.9999999999999432, -20.00000000000006750, 0.000000000000000000 ) ) ;
#9950=CARTESIAN_POINT ( 'NONE',  ( 163.1118516004056573, 1.658263919738574066E-13, -12.73709011382475254 ) ) ;
#9951=CARTESIAN_POINT ( 'NONE',  ( 136.1360204305621266, 3.511608612530704665, 3.511608612530695339 ) ) ;
#9952=CARTESIAN_POINT ( 'NONE',  ( -91.56559293963834989, -2.543181659092656077E-13, 22.67402823373191723 ) ) ;
#9953=CARTESIAN_POINT ( 'NONE',  ( 91.82158438592158234, 12.16597498397756993, 12.16597498397776356 ) ) ;
#9954=EDGE_CURVE ( 'NONE', #15005, #6531, #8809, .T. ) ;
#9957=CARTESIAN_POINT ( 'NONE',  ( -238.4067589809705794, -27.60227080167069147, 28.96627169325319429 ) ) ;
#9958=CARTESIAN_POINT ( 'NONE',  ( 57.59792236341147031, 2.435789363418171760, 0.000000000000000000 ) ) ;
#9959=CARTESIAN_POINT ( 'NONE',  ( -88.38011429763034243, -8.298859915572245782, 20.03522015847540061 ) ) ;
#9960=SHAPE_DEFINITION_REPRESENTATION ( #2559, #15720 ) ;
#9961=ORIENTED_EDGE ( 'NONE', *, *, #23375, .T. ) ;
#9963=B_SPLINE_CURVE_WITH_KNOTS ( 'NONE', 3,
 ( #754, #13490, #13980, #6269, #17603, #1397 ),
 .UNSPECIFIED., .F., .F.,
 ( 4, 2, 4 ),
 ( 2.453269466693398698E-18, 0.004090000753319153470, 0.008180001506638303471 ),
 .UNSPECIFIED. ) ;
#9964=CARTESIAN_POINT ( 'NONE',  ( -238.4067589809705794, -57.25054294065807881, 0.6820004457338858517 ) ) ;
#9965=CARTESIAN_POINT ( 'NONE',  ( 22.89002945277386303, -43.14209108112270741, -17.87003923493590207 ) ) ;
#9967=CARTESIAN_POINT ( 'NONE',  ( 4.995406935893289102, 55.24977328856464709, -40.00000000000002132 ) ) ;
#9969=VERTEX_POINT ( 'NONE', #12402 ) ;
#9972=CARTESIAN_POINT ( 'NONE',  ( -135.8532207217289738, -6.472252184284190690, -6.472252184284188914 ) ) ;
#9973=CARTESIAN_POINT ( 'NONE',  ( -188.2507053403089969, -46.97353740712736681, -13.82466505297411352 ) ) ;
#9974=CARTESIAN_POINT ( 'NONE',  ( -198.0356074513804572, -2.321818583541004323E-13, 55.37879056873073580 ) ) ;
#9975=CARTESIAN_POINT ( 'NONE',  ( 151.7948205124836534, -33.23291073765550863, 40.00000000000002132 ) ) ;
#9978=CARTESIAN_POINT ( 'NONE',  ( -238.4067589809705794, -40.00000000000007105, 0.9644942799824426372 ) ) ;
#9979=CARTESIAN_POINT ( 'NONE',  ( 163.1118516004056573, -39.99999999999986500, -12.73709011382517353 ) ) ;
#9980=CARTESIAN_POINT ( 'NONE',  ( -105.2276882640349811, -13.16704209471193643, 17.02247659824342563 ) ) ;
#9981=CARTESIAN_POINT ( 'NONE',  ( 91.82158438592159655, -44.40256751092324095, -12.16597498400075139 ) ) ;
#9982=CARTESIAN_POINT ( 'NONE',  ( 199.9999999999999432, 20.00000000000013856, 0.000000000000000000 ) ) ;
#9983=CARTESIAN_POINT ( 'NONE',  ( 130.8568914410475088, -4.207082182989324792, -52.36146031193423056 ) ) ;
#9986=CARTESIAN_POINT ( 'NONE',  ( 184.8905102610680444, -1.851754852062639767E-13, 20.92133201514444352 ) ) ;
#9987=CARTESIAN_POINT ( 'NONE',  ( 4.995406935893290878, -5.232665749138292703E-14, 15.24977328854832592 ) ) ;
#9989=CARTESIAN_POINT ( 'NONE',  ( 0.2972598230769886718, 38.42060263243669027, -18.14793986248710667 ) ) ;
#9990=CARTESIAN_POINT ( 'NONE',  ( 130.8568914410475088, -4.207082182990058428, 52.36146031193416661 ) ) ;
#9991=CARTESIAN_POINT ( 'NONE',  ( -188.4702232936801920, -13.83721295434097698, -47.05182887786487100 ) ) ;
#9992=CARTESIAN_POINT ( 'NONE',  ( 160.7895100360958622, -2.688594056682756800E-13, 28.48799984206441138 ) ) ;
#9994=CARTESIAN_POINT ( 'NONE',  ( -238.4067589809705794, 0.6820004457912851592, -0.6820004457913123597 ) ) ;
#9996=CARTESIAN_POINT ( 'NONE',  ( 57.59792236341147031, 1.722363176415065089, -1.722363176415036445 ) ) ;
#9997=CARTESIAN_POINT ( 'NONE',  ( -135.8532207217289738, 9.153146818113546246, -0.000000000000000000 ) ) ;
#9998=CARTESIAN_POINT ( 'NONE',  ( 35.93739780938212647, 20.78453051354052761, 38.99308239399191933 ) ) ;
#9999=CARTESIAN_POINT ( 'NONE',  ( 91.82158438592158234, -40.45024623143936537, -16.11829626348475131 ) ) ;
#10000=DIRECTION ( 'NONE',  ( 0.9352143328345786655, 0.1355013631633526505, 0.3271292286568833751 ) ) ;
#10004=CARTESIAN_POINT ( 'NONE',  ( -105.2110227778625955, -16.13864963246017226, 14.20565731140640153 ) ) ;
#10005=CARTESIAN_POINT ( 'NONE',  ( -7.769366557096160975, 13.56374645827035330, 45.69637362128187164 ) ) ;
#10008=CARTESIAN_POINT ( 'NONE',  ( 192.4448373802100889, -20.00000000003938538, 0.000000000000000000 ) ) ;
#10010=CARTESIAN_POINT ( 'NONE',  ( -105.3178975793838532, 5.416379678185476720, 20.76461410732419921 ) ) ;
#10011=CARTESIAN_POINT ( 'NONE',  ( -213.1075012329537230, 9.698598906450410340, 9.698598906450483170 ) ) ;
#10012=CARTESIAN_POINT ( 'NONE',  ( -96.94475454972024409, -9.001119816611835134, -20.58449551011104361 ) ) ;
#10013=CARTESIAN_POINT ( 'NONE',  ( 146.6084372240433993, -3.357462877844280890E-13, 34.62501878078305850 ) ) ;
#10019=CARTESIAN_POINT ( 'NONE',  ( -4.082462733454481629, -23.44093842354198287, -42.99255347688251305 ) ) ;
#10020=CARTESIAN_POINT ( 'NONE',  ( -135.8532207217289738, -50.09629031063973770, 6.472252184283735943 ) ) ;
#10021=CARTESIAN_POINT ( 'NONE',  ( -114.5520604218033327, -9.956332160911816942, -19.58753817072744496 ) ) ;
#10022=CARTESIAN_POINT ( 'NONE',  ( 184.8905102610680444, -13.49065550809780412, -43.07788698682583828 ) ) ;
#10023=CARTESIAN_POINT ( 'NONE',  ( -192.9588430854689989, 1.161019517985663313E-13, -14.46834944099969533 ) ) ;
#10024=CARTESIAN_POINT ( 'NONE',  ( 0.2972598230769976091, -10.13633138497465147, -10.13633138497482733 ) ) ;
#10025=CARTESIAN_POINT ( 'NONE',  ( -192.9588430854690273, -54.46834944098226572, 40.00000000000002132 ) ) ;
#10026=AXIS2_PLACEMENT_3D ( 'NONE', #22793, #20795, #8947 ) ;
#10028=CARTESIAN_POINT ( 'NONE',  ( -100.7734535825088358, -17.32597176626813251, -2.449293598294708485E-15 ) ) ;
#10029=CARTESIAN_POINT ( 'NONE',  ( -105.2800168526293874, 11.81670533840901349, 17.89480874142644495 ) ) ;
#10030=ADVANCED_FACE ( 'NONE', ( #16260 ), #7723, .T. ) ;
#10031=CARTESIAN_POINT ( 'NONE',  ( 192.4448373802101173, 40.00000000000026290, -19.99999999996018474 ) ) ;
#10032=CARTESIAN_POINT ( 'NONE',  ( 130.8568914410475372, -24.07718906447222551, -24.07718906447233209 ) ) ;
#10033=CARTESIAN_POINT ( 'NONE',  ( 4.995406935893288214, 15.24977328854832770, 0.000000000000000000 ) ) ;
#10036=CARTESIAN_POINT ( 'NONE',  ( -238.4067589809705794, 0.9644942799825386714, 0.000000000000000000 ) ) ;
#10037=CLOSED_SHELL ( 'NONE', ( #1344, #18404, #14041, #4705, #5818, #4310, #8981, #1351, #1128, #23456, #24175, #6061, #11417, #9245, #3052, #23613, #15293, #19712, #3765, #22893, #2491, #16398, #18431, #10865, #22490, #17987, #5713, #1831, #20641, #4210, #21821, #9656, #3290, #14663, #22308, #20697, #13615, #5175, #9151, #3932, #2156, #10634, #6467, #22266, #19239, #5120, #4121, #14673, #19798, #22652, #14743, #5087, #22686, #17750, #18579, #7327, #16550, #359, #2490, #14428, #13938, #881, #639, #9140, #7053, #2080, #199, #14007, #21123, #1016, #25260, #4455, #10977, #11347, #12807, #356, #11728, #20968, #10784, #23090, #6719, #8294, #22159, #14531, #6197, #6953, #8247, #18916, #6568, #7658, #23762, #20128, #4450, #17907, #10782, #20189, #4691, #15568, #26326, #11416, #10030, #14285, #17751, #23445, #16723, #8681, #13472, #20535, #7575, #12885, #198, #6527, #7273, #16966, #23487, #17203, #1827, #25507 ) ) ;
#10038=CARTESIAN_POINT ( 'NONE',  ( 128.5824617753800965, 11.99766463964378360, 28.96492468983284851 ) ) ;
#10039=CARTESIAN_POINT ( 'NONE',  ( -162.0762913951020892, -1.777970010055771463E-13, 41.69427287682835015 ) ) ;
#10040=CARTESIAN_POINT ( 'NONE',  ( 170.2234770963711128, 10.92277846919147066, 45.64576402573197811 ) ) ;
#10045=CARTESIAN_POINT ( 'NONE',  ( -163.5815439468644854, -12.03526835479589430, -38.33196286469318181 ) ) ;
#10046=CARTESIAN_POINT ( 'NONE',  ( -109.1264249741457633, 13.72187187126429997, 33.12752917268171871 ) ) ;
#10049=CARTESIAN_POINT ( 'NONE',  ( -259.2033419157646676, 49.83842185052017015, 6.730120644404137487 ) ) ;
#10050=CARTESIAN_POINT ( 'NONE',  ( 199.9999999999999432, -14.14213562373073607, -14.14213562373102206 ) ) ;
#10051=CARTESIAN_POINT ( 'NONE',  ( -114.6112526615690115, 21.20804461678012132, 5.819739293988868134 ) ) ;
#10052=CARTESIAN_POINT ( 'NONE',  ( -77.79459117305557925, 19.55393134992732129, -9.938707241617530386 ) ) ;
#10053=CARTESIAN_POINT ( 'NONE',  ( -105.3755690713226585, -12.89780903124444578, 43.67073346367968156 ) ) ;
#10054=CARTESIAN_POINT ( 'NONE',  ( -87.10563802237744824, 13.14174799572376706, -16.99650074894995910 ) ) ;
#10055=CARTESIAN_POINT ( 'NONE',  ( -213.1075012329537230, 9.698598906450543566, -9.698598906450348167 ) ) ;
#10056=CARTESIAN_POINT ( 'NONE',  ( 170.2234770963711128, 17.36149277827004411, -17.36149277826983095 ) ) ;
#10058=EDGE_CURVE ( 'NONE', #13429, #23676, #8599, .T. ) ;
#10060=CARTESIAN_POINT ( 'NONE',  ( 170.2234770963711128, 1.169953928977015745E-13, -24.55285855007187124 ) ) ;
#10061=CARTESIAN_POINT ( 'NONE',  ( 0.2972598230769976091, -10.13633138497465147, -10.13633138497482733 ) ) ;
#10062=CARTESIAN_POINT ( 'NONE',  ( 21.25019396254074167, 43.56030393975865422, -18.04326867293220360 ) ) ;
#10063=CARTESIAN_POINT ( 'NONE',  ( -213.1075012329537230, 53.71589010950162191, -40.00000000000002132 ) ) ;
#10064=ORIENTED_EDGE ( 'NONE', *, *, #4931, .T. ) ;
#10065=CARTESIAN_POINT ( 'NONE',  ( -238.4067589809705794, 0.9644942799825386714, 0.000000000000000000 ) ) ;
#10067=CARTESIAN_POINT ( 'NONE',  ( -4.201409602816648992, -46.93439176590693052, 13.81669219312499486 ) ) ;
#10068=CARTESIAN_POINT ( 'NONE',  ( -208.1127848780264742, 15.00245453012665742, 40.00000000000002132 ) ) ;
#10069=VERTEX_POINT ( 'NONE', #18928 ) ;
#10070=CARTESIAN_POINT ( 'NONE',  ( -188.6013476421594817, -43.09288642756992971, 23.51433506917121008 ) ) ;
#10071=CIRCLE ( 'NONE', #21142, 14.99999999999999467 ) ;
#10073=CARTESIAN_POINT ( 'NONE',  ( -3.696864809816500230, -23.52297716615279555, 43.10456217110754551 ) ) ;
#10074=CARTESIAN_POINT ( 'NONE',  ( 23.54890483848213378, 13.78807129923295527, -46.74501720879577960 ) ) ;
#10077=CARTESIAN_POINT ( 'NONE',  ( -187.7699188115033735, -13.79076593538429130, 46.80708926513559476 ) ) ;
#10078=CARTESIAN_POINT ( 'NONE',  ( 151.7948205124836534, 33.06932595376333239, 23.49921654116065284 ) ) ;
#10079=CARTESIAN_POINT ( 'NONE',  ( -135.8532207217289738, 9.153146818113546246, -0.000000000000000000 ) ) ;
#10080=CARTESIAN_POINT ( 'NONE',  ( -190.0144721489061794, 23.79987203025343234, -43.47822244622717136 ) ) ;
#10081=CARTESIAN_POINT ( 'NONE',  ( -162.0762913951021176, 29.48230308784730980, 27.08623940707652622 ) ) ;
#10083=CARTESIAN_POINT ( 'NONE',  ( -208.1127848780264742, -55.00245453014425578, -40.00000000000002132 ) ) ;
#10084=CARTESIAN_POINT ( 'NONE',  ( -135.8532207217289738, 30.84685318188643066, 2.449293598294708485E-15 ) ) ;
#10085=CARTESIAN_POINT ( 'NONE',  ( -105.3755690713226585, -39.99999999999985079, -18.24025645688394448 ) ) ;
#10086=CARTESIAN_POINT ( 'NONE',  ( -135.8532207217289738, 50.09629031063965243, -6.472252184284084109 ) ) ;
#10087=CARTESIAN_POINT ( 'NONE',  ( 14.38125909742181108, 1.616281842095393922E-13, -15.17850393972633682 ) ) ;
#10088=CARTESIAN_POINT ( 'NONE',  ( 98.29820294273291381, -18.47759065023123526, -7.653668647304108674 ) ) ;
#10090=CARTESIAN_POINT ( 'NONE',  ( 192.4448373802101173, -42.42640687122073473, 14.14213562370301780 ) ) ;
#10091=B_SPLINE_CURVE_WITH_KNOTS ( 'NONE', 3,
 ( #22691, #2330, #20559, #6311, #336, #20294 ),
 .UNSPECIFIED., .F., .F.,
 ( 4, 2, 4 ),
 ( 1.142150420466554580E-15, 0.03937685942888059787, 0.07875371885776004388 ),
 .UNSPECIFIED. ) ;
#10092=CARTESIAN_POINT ( 'NONE',  ( -99.31267923333879821, -8.544756979511673123, 20.62886818714596160 ) ) ;
#10094=VERTEX_POINT ( 'NONE', #7075 ) ;
#10096=CARTESIAN_POINT ( 'NONE',  ( 200.0000000000000000, -42.42640687119269671, -14.14213562373124766 ) ) ;
#10097=CARTESIAN_POINT ( 'NONE',  ( 23.35928221536255833, -46.81377789283288848, -13.80178577956144181 ) ) ;
#10098=VERTEX_POINT ( 'NONE', #17181 ) ;
#10099=CARTESIAN_POINT ( 'NONE',  ( -259.2033419157646676, -9.517827891722680178, 0.000000000000000000 ) ) ;
#10100=CARTESIAN_POINT ( 'NONE',  ( -86.86493150571114086, -8.366608963953822808, -19.60045294882766598 ) ) ;
#10105=CARTESIAN_POINT ( 'NONE',  ( -100.7734535825088358, -16.03295912088706743, -16.03295912088710296 ) ) ;
#10106=EDGE_CURVE ( 'NONE', #25810, #1453, #8009, .T. ) ;
#10107=CARTESIAN_POINT ( 'NONE',  ( -129.2920262391662050, -25.26067940890114372, -10.46331600579726739 ) ) ;
#10108=CARTESIAN_POINT ( 'NONE',  ( -105.3755690713226585, -39.99999999999996447, -21.75974354311664527 ) ) ;
#10109=CARTESIAN_POINT ( 'NONE',  ( -30.26275506840324070, 1.694272468446254232, 0.000000000000000000 ) ) ;
#10113=CARTESIAN_POINT ( 'NONE',  ( -30.26275506840324070, -40.00000000000003553, 1.694272468446120117 ) ) ;
#10114=CARTESIAN_POINT ( 'NONE',  ( 184.8905102610680444, -39.99999999999991473, -20.92133201514458207 ) ) ;
#10115=CARTESIAN_POINT ( 'NONE',  ( 136.1360204305621551, -40.00000000000036238, 35.03383547441254109 ) ) ;
#10116=CARTESIAN_POINT ( 'NONE',  ( -213.1075012329537230, -8.703598725189323045E-14, 13.71589010951911902 ) ) ;
#10117=CARTESIAN_POINT ( 'NONE',  ( -30.26275506840322294, -57.76657404653985139, 1.198031551615709844 ) ) ;
#10118=CARTESIAN_POINT ( 'NONE',  ( -259.2033419157646676, 9.517827891722582478, -40.00000000000002132 ) ) ;
#10119=CARTESIAN_POINT ( 'NONE',  ( -280.0000000000000568, -42.42640687119285303, -14.14213562373118371 ) ) ;
#10122=CARTESIAN_POINT ( 'NONE',  ( -86.96347745069644475, -2.438961472018186339E-13, 21.75974354311649961 ) ) ;
#10123=CARTESIAN_POINT ( 'NONE',  ( -30.26275506840323359, -40.00000000000017053, 41.69427246844613677 ) ) ;
#10124=CARTESIAN_POINT ( 'NONE',  ( -208.1127848780264742, 67.17687982760683951, 10.60833733268317403 ) ) ;
#10125=CARTESIAN_POINT ( 'NONE',  ( -114.5468827412802710, 9.969911493407927594, 19.54080463289418290 ) ) ;
#10126=CARTESIAN_POINT ( 'NONE',  ( -189.1816166312681560, -17.96744819724773734, -43.37725711903312487 ) ) ;
#10127=CARTESIAN_POINT ( 'NONE',  ( 184.8905102610680444, 14.79361573936396113, -14.79361573936377461 ) ) ;
#10129=CARTESIAN_POINT ( 'NONE',  ( -86.96347745069644475, -43.67073346367964604, -12.89780903124457545 ) ) ;
#10131=CARTESIAN_POINT ( 'NONE',  ( -208.1127848780264742, -15.00245453012673202, -40.00000000000002132 ) ) ;
#10133=CARTESIAN_POINT ( 'NONE',  ( 192.4448373802101173, -14.14213562375826605, -42.42640687116518450 ) ) ;
#10134=CARTESIAN_POINT ( 'NONE',  ( -77.62874474886946530, 3.805079090663308516, 21.73921449504242531 ) ) ;
#10137=CARTESIAN_POINT ( 'NONE',  ( 12.01361959687196190, -24.84115733209533516, 44.88892880200814517 ) ) ;
#10138=CARTESIAN_POINT ( 'NONE',  ( -2.557884977174613716, 23.77085849409060003, 43.43882039325016109 ) ) ;
#10139=ORIENTED_EDGE ( 'NONE', *, *, #1162, .T. ) ;
#10142=CARTESIAN_POINT ( 'NONE',  ( 151.7948205124836250, -33.23291073765550863, 0.000000000000000000 ) ) ;
#10145=CARTESIAN_POINT ( 'NONE',  ( -100.7734535825088358, -16.03295912088706743, -16.03295912088710296 ) ) ;
#10147=B_SPLINE_CURVE_WITH_KNOTS ( 'NONE', 3,
 ( #19823, #17817, #25829, #1609, #20324, #8205 ),
 .UNSPECIFIED., .F., .F.,
 ( 4, 2, 4 ),
 ( 0.3689590070116581799, 0.3867117631979620773, 0.4044645193949216733 ),
 .UNSPECIFIED. ) ;
#10149=CARTESIAN_POINT ( 'NONE',  ( -99.31364972215654063, -8.933506367378383217, -20.48028939132497328 ) ) ;
#10150=( BOUNDED_CURVE ( )  B_SPLINE_CURVE ( 3, ( #21951, #7441, #17429, #17681, #17553, #21817, #19304 ),
 .UNSPECIFIED., .F., .F. ) 
 B_SPLINE_CURVE_WITH_KNOTS ( ( 4, 3, 4 ),
 ( 0.007486030685209696563, 0.02316748376737270271, 0.03884893684953900223 ),
 .UNSPECIFIED. ) 
 CURVE ( )  GEOMETRIC_REPRESENTATION_ITEM ( )  RATIONAL_B_SPLINE_CURVE ( ( 0.5852718452494432011, 0.6660804010233991601, 0.8043231192735847968, 1.000000000000000000, 0.8043231192735437185, 0.6660804010233410954, 0.5852718452493922419 ) ) 
 REPRESENTATION_ITEM ( '' )  );
#10151=CARTESIAN_POINT ( 'NONE',  ( 0.2972598230769883387, 40.00000000000017053, -14.33493731733891607 ) ) ;
#10152=CARTESIAN_POINT ( 'NONE',  ( 98.29820294267473457, 1.310413973322231751, -20.00000000000522959 ) ) ;
#10156=CARTESIAN_POINT ( 'NONE',  ( -186.5449016017332440, 41.81559155949143758, 17.32058514259380289 ) ) ;
#10157=CARTESIAN_POINT ( 'NONE',  ( 9.006212071498026717, -24.85331907610667912, -44.90541342374617528 ) ) ;
#10158=CARTESIAN_POINT ( 'NONE',  ( 192.4448373802100889, -14.14213562370293431, -14.14213562370322030 ) ) ;
#10159=CARTESIAN_POINT ( 'NONE',  ( -105.2054292635175585, 5.571723593410010660E-14, -21.49321519473983955 ) ) ;
#10160=CARTESIAN_POINT ( 'NONE',  ( 0.2972598230770153171, -66.70487387989861361, 10.13633138497438324 ) ) ;
#10162=CARTESIAN_POINT ( 'NONE',  ( -198.0356074513804572, -10.87444709759714634, -10.87444709759729911 ) ) ;
#10163=CARTESIAN_POINT ( 'NONE',  ( -238.4067589809705794, -0.9644942799826263791, 40.00000000000002132 ) ) ;
#10164=CARTESIAN_POINT ( 'NONE',  ( -198.0356074513804572, 10.87444709759730088, -10.87444709759707173 ) ) ;
#10165=CARTESIAN_POINT ( 'NONE',  ( 200.0000000000000000, -19.99999999999988631, -40.00000000000002132 ) ) ;
#10166=CARTESIAN_POINT ( 'NONE',  ( -114.4364955367320107, 8.644468109212716911, 20.04994829327460337 ) ) ;
#10167=CARTESIAN_POINT ( 'NONE',  ( 170.2234770963711128, 39.99999999999980105, 24.55285855007229401 ) ) ;
#10168=CARTESIAN_POINT ( 'NONE',  ( 130.8568914410475088, 4.207082182989741348, -52.36146031193420924 ) ) ;
#10169=CARTESIAN_POINT ( 'NONE',  ( -208.1127848780264742, 15.00245453012665742, -40.00000000000002132 ) ) ;
#10170=ORIENTED_EDGE ( 'NONE', *, *, #26073, .T. ) ;
#10171=ORIENTED_EDGE ( 'NONE', *, *, #11409, .T. ) ;
#10172=CARTESIAN_POINT ( 'NONE',  ( -280.0000000000000000, -20.00000000000006750, 0.000000000000000000 ) ) ;
#10174=CARTESIAN_POINT ( 'NONE',  ( -97.72675010090193837, -8.185591577777252326, -20.89622088363372399 ) ) ;
#10175=CARTESIAN_POINT ( 'NONE',  ( -259.2033419157646676, -1.564921101325656229E-13, 30.48217210827739621 ) ) ;
#10176=CARTESIAN_POINT ( 'NONE',  ( -105.3755690713226727, 12.89780903124418998, -12.89780903124389155 ) ) ;
#10177=CARTESIAN_POINT ( 'NONE',  ( -213.1075012329537230, 13.71589010951907994, 0.000000000000000000 ) ) ;
#10178=CARTESIAN_POINT ( 'NONE',  ( 184.8905102610680444, -20.92133201514440799, 0.000000000000000000 ) ) ;
#10179=DIRECTION ( 'NONE',  ( -1.000000000000000000, 1.018913292508929218E-14, 0.000000000000000000 ) ) ;
#10182=CARTESIAN_POINT ( 'NONE',  ( 0.2972598230769907257, 66.70487387989869887, -10.13633138497392494 ) ) ;
#10183=CARTESIAN_POINT ( 'NONE',  ( -162.0762913951021176, -29.48230308784793152, 27.08623940707591515 ) ) ;
#10185=CARTESIAN_POINT ( 'NONE',  ( -86.96347745069644475, -2.438961472018186339E-13, 21.75974354311649961 ) ) ;
#10186=CARTESIAN_POINT ( 'NONE',  ( -198.0356074513804572, -39.15871834505931304, 17.40982414986437377 ) ) ;
#10187=CARTESIAN_POINT ( 'NONE',  ( 19.06497207195980792, 10.03556273973447155, -10.03556273973422286 ) ) ;
#10188=CARTESIAN_POINT ( 'NONE',  ( 136.1360204305621266, -24.77266263493151044, 24.77266263493093135 ) ) ;
#10189=CARTESIAN_POINT ( 'NONE',  ( -105.3755690713226585, -12.89780903124383471, -43.67073346367985920 ) ) ;
#10193=CARTESIAN_POINT ( 'NONE',  ( 14.38125909742181818, -1.924622159709266762E-13, 55.17850393972636880 ) ) ;
#10195=CARTESIAN_POINT ( 'NONE',  ( 22.57783252600447454, 43.22748647439907899, -17.90541116499352015 ) ) ;
#10196=CARTESIAN_POINT ( 'NONE',  ( 192.4448373802101173, 19.99999999996065014, -40.00000000000002132 ) ) ;
#10198=CARTESIAN_POINT ( 'NONE',  ( -56.48582580120559271, -6.472252184284187138, -6.472252184284199572 ) ) ;
#10199=B_SPLINE_CURVE_WITH_KNOTS ( 'NONE', 3,
 ( #1583, #24057, #17926, #21933, #5693, #13798, #20202, #18061 ),
 .UNSPECIFIED., .F., .F.,
 ( 4, 2, 2, 4 ),
 ( -5.298247996646543873E-05, 0.001923793760049340336, 0.003900570000065146144, 0.007854122480096750389 ),
 .UNSPECIFIED. ) ;
#10200=CARTESIAN_POINT ( 'NONE',  ( -5.152948516943984814, -42.67688069069014745, 23.23217004669189123 ) ) ;
#10202=CARTESIAN_POINT ( 'NONE',  ( -238.4067589809705794, 40.96449427998256709, 2.449293598294708485E-15 ) ) ;
#10203=ORIENTED_EDGE ( 'NONE', *, *, #388, .F. ) ;
#10206=CARTESIAN_POINT ( 'NONE',  ( 22.37977766478752883, -13.85469381972563241, 47.17011059970548104 ) ) ;
#10208=CARTESIAN_POINT ( 'NONE',  ( -3.838270362648607659, 17.89317813950102831, -43.19795333834863982 ) ) ;
#10212=CARTESIAN_POINT ( 'NONE',  ( 19.06497207195981147, -4.605042221739098431E-14, 14.19242893257840521 ) ) ;
#10213=CARTESIAN_POINT ( 'NONE',  ( -30.26275506840323715, 29.48230279907829754, -29.48230279907758344 ) ) ;
#10215=CARTESIAN_POINT ( 'NONE',  ( -188.3120606736016214, 23.45204117844427572, -43.00889065702882874 ) ) ;
#10216=CARTESIAN_POINT ( 'NONE',  ( -280.0000000000000568, 14.14213562373038968, 42.42640687119305198 ) ) ;
#10218=CARTESIAN_POINT ( 'NONE',  ( -105.3755690713226727, -18.24025645688354302, -2.449293598294708485E-15 ) ) ;
#10219=CARTESIAN_POINT ( 'NONE',  ( -238.4067589809705794, 40.96449428006337001, -40.00000000000002132 ) ) ;
#10220=CARTESIAN_POINT ( 'NONE',  ( 184.8905102610680444, -39.99999999999978684, -19.07866798485600768 ) ) ;
#10221=CARTESIAN_POINT ( 'NONE',  ( -56.48582580120559982, -6.472252184284282173, 50.09629031063965243 ) ) ;
#10223=CARTESIAN_POINT ( 'NONE',  ( -56.48582580120558561, 6.472252184284607246, -50.09629031063960269 ) ) ;
#10224=EDGE_LOOP ( 'NONE', ( #15900, #15458, #19615, #7345, #13183, #125, #7996 ) ) ;
#10225=CARTESIAN_POINT ( 'NONE',  ( -56.48582580120559271, -6.472252184284187138, -6.472252184284199572 ) ) ;
#10226=CARTESIAN_POINT ( 'NONE',  ( -103.9663809734695405, 8.026122151187262688, 20.15238534352856803 ) ) ;
#10227=EDGE_LOOP ( 'NONE', ( #23795, #14393, #15586, #21944, #11309 ) ) ;
#10228=VERTEX_POINT ( 'NONE', #15057 ) ;
#10229=CARTESIAN_POINT ( 'NONE',  ( -238.4067589809705794, -28.96627169325313389, -27.60227080167074831 ) ) ;
#10230=CARTESIAN_POINT ( 'NONE',  ( 21.80484139881942696, -43.42703366220392525, -17.98806631651325816 ) ) ;
#10231=VERTEX_POINT ( 'NONE', #8683 ) ;
#10232=CARTESIAN_POINT ( 'NONE',  ( -105.3755690713226727, -21.75974354311652093, 0.000000000000000000 ) ) ;
#10233=CARTESIAN_POINT ( 'NONE',  ( -86.95456283525173546, -9.640367918722454021, -19.12038226852981992 ) ) ;
#10235=B_SPLINE_CURVE_WITH_KNOTS ( 'NONE', 3,
 ( #17555, #15683, #21436, #21562, #11191, #23808, #11563, #13195, #17683, #15309, #25825, #21690 ),
 .UNSPECIFIED., .F., .F.,
 ( 4, 2, 2, 2, 2, 4 ),
 ( -5.998499568646490758E-08, 0.003531500499830293825, 0.007063060984656273529, 0.01412618195430823814, 0.02118930292396020362, 0.02825242389361216910 ),
 .UNSPECIFIED. ) ;
#10238=CARTESIAN_POINT ( 'NONE',  ( -91.56559293963834989, 12.25131212657490209, -44.31723036834897300 ) ) ;
#10239=CARTESIAN_POINT ( 'NONE',  ( -144.0562696875023789, -31.27040355047325093, -10.50947022297233246 ) ) ;
#10240=CARTESIAN_POINT ( 'NONE',  ( 200.0000000000000000, -39.99999999999991473, -20.00000000000024514 ) ) ;
#10241=CARTESIAN_POINT ( 'NONE',  ( 170.2234770963711128, -24.55285855007183926, 0.000000000000000000 ) ) ;
#10246=CARTESIAN_POINT ( 'NONE',  ( -135.8532207217289738, -40.00000000000001421, -9.153146818113709671 ) ) ;
#10247=CARTESIAN_POINT ( 'NONE',  ( -198.0356074513804572, -2.321818583541004323E-13, 55.37879056873073580 ) ) ;
#10249=CARTESIAN_POINT ( 'NONE',  ( -86.96347745069645896, 40.00000000000008527, -21.75974354311636461 ) ) ;
#10250=CARTESIAN_POINT ( 'NONE',  ( 0.2972598230769983307, -14.33493731733933352, 0.000000000000000000 ) ) ;
#10251=CARTESIAN_POINT ( 'NONE',  ( 184.8905102610680444, -41.77492675555986779, -14.79361573936407304 ) ) ;
#10252=CARTESIAN_POINT ( 'NONE',  ( 57.59792236341147031, 2.435789363418171760, 0.000000000000000000 ) ) ;
#10253=CARTESIAN_POINT ( 'NONE',  ( -91.56559293963834989, 16.03295912088683650, 40.53558337403684675 ) ) ;
#10255=CARTESIAN_POINT ( 'NONE',  ( 14.32711937312301487, -49.08922911798406830, 14.14294248749828498 ) ) ;
#10256=CARTESIAN_POINT ( 'NONE',  ( -105.3755690713226727, 1.741486606973311632E-13, -18.24025645688352881 ) ) ;
#10257=CARTESIAN_POINT ( 'NONE',  ( 146.6084372240433993, 5.715592784339989804E-15, 5.374981219216972583 ) ) ;
#10258=CARTESIAN_POINT ( 'NONE',  ( 163.1118516004056573, 37.29075403953160617, -19.27778845539222985 ) ) ;
#10259=CARTESIAN_POINT ( 'NONE',  ( 170.2234770963711128, -10.92277846919235529, 45.64576402573175073 ) ) ;
#10260=CARTESIAN_POINT ( 'NONE',  ( -188.9266751785335146, -17.94050871568824235, -43.31221945728833589 ) ) ;
#10261=CARTESIAN_POINT ( 'NONE',  ( 0.2972598230770027716, -38.42060263243656237, -18.14793986248737667 ) ) ;
#10262=ORIENTED_EDGE ( 'NONE', *, *, #3297, .T. ) ;
#10263=CARTESIAN_POINT ( 'NONE',  ( -259.2033419157646676, -35.01439189186523748, -21.55415060305881170 ) ) ;
#10265=CARTESIAN_POINT ( 'NONE',  ( 91.82158438592158234, 17.20528682183301683, 0.000000000000000000 ) ) ;
#10266=CARTESIAN_POINT ( 'NONE',  ( 73.43374839994166337, 12.96823619005579964, 26.88865971589134318 ) ) ;
#10267=CARTESIAN_POINT ( 'NONE',  ( 184.8905102610680444, -14.79361573936399665, 14.79361573936367158 ) ) ;
#10269=ORIENTED_EDGE ( 'NONE', *, *, #18324, .F. ) ;
#10273=CARTESIAN_POINT ( 'NONE',  ( 21.98945382326331810, -23.63684424402667261, 43.25809532770878008 ) ) ;
#10274=CARTESIAN_POINT ( 'NONE',  ( 5.823571940223595256, 24.75780943189298355, 44.77584346942381188 ) ) ;
#10275=ORIENTED_EDGE ( 'NONE', *, *, #18243, .T. ) ;
#10280=CARTESIAN_POINT ( 'NONE',  ( 4.995406935893289102, 10.78321810388998081, 10.78321810389001811 ) ) ;
#10281=CARTESIAN_POINT ( 'NONE',  ( 23.37394308801976806, 42.85717664514618264, -23.33966569535049373 ) ) ;
#10282=CARTESIAN_POINT ( 'NONE',  ( 192.4448373802101173, 40.00000000000026290, -19.99999999996018474 ) ) ;
#10284=CARTESIAN_POINT ( 'NONE',  ( -138.9613198120178765, 29.42718893709621142, -10.11110880661601996 ) ) ;
#10288=CARTESIAN_POINT ( 'NONE',  ( -121.8425418803964817, 9.420907392434369143, 22.74408238734170595 ) ) ;
#10289=CARTESIAN_POINT ( 'NONE',  ( 16.10036699873721489, -24.53427828609593675, -44.47262139758191779 ) ) ;
#10290=CARTESIAN_POINT ( 'NONE',  ( -135.8532207217289738, -21.81201906317757633, -21.81201906317793515 ) ) ;
#10292=CARTESIAN_POINT ( 'NONE',  ( -105.2054292634647936, 1.359558446572939561, -21.49321519475378750 ) ) ;
#10293=CARTESIAN_POINT ( 'NONE',  ( -192.9588430854690273, -66.79921049724377724, 10.23066800231950069 ) ) ;
#10295=CARTESIAN_POINT ( 'NONE',  ( 170.2234770963711128, 24.55285855007190321, 0.000000000000000000 ) ) ;
#10296=CARTESIAN_POINT ( 'NONE',  ( 136.1360204305621551, -4.966164525587043244, 40.00000000000002132 ) ) ;
#10299=CARTESIAN_POINT ( 'NONE',  ( 0.2972598230770130412, -54.33493731733936016, -2.449293598294708485E-15 ) ) ;
#10300=CARTESIAN_POINT ( 'NONE',  ( -105.3366978519447059, 10.59928388867598237, 18.59727947899841993 ) ) ;
#10301=CARTESIAN_POINT ( 'NONE',  ( -198.0356074513804572, 40.00000000000056843, -55.37879056871282302 ) ) ;
#10302=EDGE_CURVE ( 'NONE', #11184, #14253, #2566, .T. ) ;
#10303=CARTESIAN_POINT ( 'NONE',  ( -135.8532207217289738, 21.81201906317777883, -34.75652343174605363 ) ) ;
#10305=CARTESIAN_POINT ( 'NONE',  ( -56.48582580120559271, -9.153146818113595984, 0.000000000000000000 ) ) ;
#10308=CARTESIAN_POINT ( 'NONE',  ( -162.0762913951021176, 1.694272876828294194, 40.00000000000002132 ) ) ;
#10310=CARTESIAN_POINT ( 'NONE',  ( 170.0000000000000000, -21.59613885783082665, -12.70659020859102739 ) ) ;
#10311=CARTESIAN_POINT ( 'NONE',  ( -162.0762913951021176, 57.76657433523994456, -1.198031840315424867 ) ) ;
#10312=CARTESIAN_POINT ( 'NONE',  ( 199.9999999999999432, -20.00000000000006750, 0.000000000000000000 ) ) ;
#10313=CARTESIAN_POINT ( 'NONE',  ( 170.2234770963711128, -24.55285855007183926, 0.000000000000000000 ) ) ;
#10317=CARTESIAN_POINT ( 'NONE',  ( 14.38125909742181108, 39.01709431150961649, -39.01709431150867147 ) ) ;
#10318=CARTESIAN_POINT ( 'NONE',  ( 192.4448373802101173, -42.42640687116510634, 14.14213562375845257 ) ) ;
#10320=CARTESIAN_POINT ( 'NONE',  ( -208.1127848780264742, 40.00000000000014211, -15.00245453012627728 ) ) ;
#10321=CARTESIAN_POINT ( 'NONE',  ( 200.0000000000000000, -42.42640687119290988, 14.14213562373064903 ) ) ;
#10322=CARTESIAN_POINT ( 'NONE',  ( -87.13361725327074225, 15.19799821270847850, -15.19799821270833284 ) ) ;
#10323=CARTESIAN_POINT ( 'NONE',  ( 146.6084372240433993, -24.48358557860319706, -24.48358557860330720 ) ) ;
#10324=CARTESIAN_POINT ( 'NONE',  ( 4.995406935893297984, -39.06748935135182421, -17.50105314357212549 ) ) ;
#10327=CARTESIAN_POINT ( 'NONE',  ( -208.1127848780264742, 39.99999999999979394, 55.00245453010936103 ) ) ;
#10329=CARTESIAN_POINT ( 'NONE',  ( 23.26364522860089323, 46.84987168986916117, -13.80713620122723917 ) ) ;
#10330=CARTESIAN_POINT ( 'NONE',  ( -192.9588430854690273, 14.46834944099966336, -40.00000000000002132 ) ) ;
#10331=CARTESIAN_POINT ( 'NONE',  ( 98.29820294267527458, 2.689882573189819553E-13, -20.00000000000500222 ) ) ;
#10332=CARTESIAN_POINT ( 'NONE',  ( -3.494657986427672114, -43.29048295385651812, 17.93150516116827120 ) ) ;
#10333=CARTESIAN_POINT ( 'NONE',  ( -259.2033419157646676, 30.48217210827734647, 2.449293598294708485E-15 ) ) ;
#10336=CARTESIAN_POINT ( 'NONE',  ( -77.55640685876518603, 15.64922766773203122, 15.64922766773211471 ) ) ;
#10337=CARTESIAN_POINT ( 'NONE',  ( -4.660840668352994598, -13.78427145221255934, 46.77528141313064225 ) ) ;
#10338=CARTESIAN_POINT ( 'NONE',  ( 2.332272417556594313, 24.49123061636224463, -44.41409500754982531 ) ) ;
#10340=CARTESIAN_POINT ( 'NONE',  ( -259.2033419157646676, -1.473088368616265084E-13, 9.517827891722632216 ) ) ;
#10342=CARTESIAN_POINT ( 'NONE',  ( -187.3037411061906425, -23.25513534570069041, 42.71163782367113271 ) ) ;
#10343=CARTESIAN_POINT ( 'NONE',  ( -238.4067589809705794, -27.60227080167029001, -28.96627169325357798 ) ) ;
#10344=CARTESIAN_POINT ( 'NONE',  ( 136.1360204305621266, 35.03383547441298873, 0.000000000000000000 ) ) ;
#10345=CARTESIAN_POINT ( 'NONE',  ( -194.4222169613859421, 14.07715596672279545, -48.65437996130461329 ) ) ;
#10346=CARTESIAN_POINT ( 'NONE',  ( 136.1360204305621551, 3.511608612530062512, 53.05693388239318864 ) ) ;
#10347=CARTESIAN_POINT ( 'NONE',  ( 163.1118516004056573, 9.006482792073693844, 47.56205970284970164 ) ) ;
#10348=CARTESIAN_POINT ( 'NONE',  ( -192.9588430854690273, -54.46834944098226572, 40.00000000000002132 ) ) ;
#10349=CARTESIAN_POINT ( 'NONE',  ( -135.8532207217289738, 30.84685318188643421, 40.00000000000002132 ) ) ;
#10350=CARTESIAN_POINT ( 'NONE',  ( 192.4448373802101173, -40.00000000000019185, 20.00000000003900524 ) ) ;
#10351=CARTESIAN_POINT ( 'NONE',  ( 146.6084372240433993, 3.800685668858676980, 3.800685668858667210 ) ) ;
#10352=CARTESIAN_POINT ( 'NONE',  ( -97.73806390045244541, 20.71810467719082283, -8.581719943944259299 ) ) ;
#10353=CARTESIAN_POINT ( 'NONE',  ( 4.995406935893305977, -39.06748935135157552, -39.06748935135225764 ) ) ;
#10354=ORIENTED_EDGE ( 'NONE', *, *, #15991, .F. ) ;
#10355=CARTESIAN_POINT ( 'NONE',  ( 14.38125909742180752, 10.73282306404720465, 10.73282306404724018 ) ) ;
#10359=CARTESIAN_POINT ( 'NONE',  ( 14.38125909742181996, -10.73282306403606157, 67.30136555895948902 ) ) ;
#10360=CARTESIAN_POINT ( 'NONE',  ( 6.202588567996038194, -49.19971320597203146, -14.15973318135109871 ) ) ;
#10362=CARTESIAN_POINT ( 'NONE',  ( 4.990270234119186021, -49.14367003637712372, -14.15117691407198741 ) ) ;
#10364=ORIENTED_EDGE ( 'NONE', *, *, #4933, .F. ) ;
#10366=DIRECTION ( 'NONE',  ( 0.3301743741175477975, 0.9439199556509468847, 0.000000000000000000 ) ) ;
#10367=CARTESIAN_POINT ( 'NONE',  ( 163.1118516004056573, 9.006482792074356425, -47.56205970284957374 ) ) ;
#10368=CARTESIAN_POINT ( 'NONE',  ( -189.1816166312713960, -43.37725711903439674, -17.96744819724840880 ) ) ;
#10369=B_SPLINE_CURVE_WITH_KNOTS ( 'NONE', 3,
 ( #7626, #17872, #26023, #13750, #3935, #17610 ),
 .UNSPECIFIED., .F., .F.,
 ( 4, 2, 4 ),
 ( -5.998621906354538341E-08, 0.03938016914544736902, 0.07876039827711379948 ),
 .UNSPECIFIED. ) ;
#10370=CARTESIAN_POINT ( 'NONE',  ( 163.1118516004056573, -40.00000000000003553, 12.73709011382460687 ) ) ;
#10371=CARTESIAN_POINT ( 'NONE',  ( 192.4448373802100889, 19.99999999996064304, 2.449293598294708485E-15 ) ) ;
#10374=CARTESIAN_POINT ( 'NONE',  ( -208.1127848780264742, -40.00000000000011369, 15.00245453012655439 ) ) ;
#10375=CARTESIAN_POINT ( 'NONE',  ( -259.2033419157646676, 39.99999999999987210, 30.48217210827754542 ) ) ;
#10376=CARTESIAN_POINT ( 'NONE',  ( -192.9588430854690273, 39.99999999999992895, 14.46834944099983922 ) ) ;
#10377=CARTESIAN_POINT ( 'NONE',  ( 19.06497207195981503, -14.19242893257840166, 0.000000000000000000 ) ) ;
#10378=CARTESIAN_POINT ( 'NONE',  ( -86.96347745069644475, -18.24025645688354302, -2.449293598294708485E-15 ) ) ;
#10379=EDGE_CURVE ( 'NONE', #4560, #7864, #4662, .T. ) ;
#10380=CARTESIAN_POINT ( 'NONE',  ( 199.9999999999999432, -14.14213562373093680, 14.14213562373082311 ) ) ;
#10381=CARTESIAN_POINT ( 'NONE',  ( 159.7744820660625180, -10.75261058663746816, -25.95909830917691608 ) ) ;
#10382=CARTESIAN_POINT ( 'NONE',  ( 23.37394308801977871, -46.80823611210205115, 13.80096434448272724 ) ) ;
#10383=CARTESIAN_POINT ( 'NONE',  ( 91.82158438592156813, 40.00000000000027711, -22.79471317813428044 ) ) ;
#10384=CARTESIAN_POINT ( 'NONE',  ( -30.26275506840323359, -1.535832457777009877E-13, 41.69427246844629309 ) ) ;
#10385=CARTESIAN_POINT ( 'NONE',  ( -259.2033419157646676, 49.83842185052027673, -6.730120644403441155 ) ) ;
#10388=CARTESIAN_POINT ( 'NONE',  ( 151.7948205124836534, -33.06932595376343897, -23.49921654116042902 ) ) ;
#10390=CARTESIAN_POINT ( 'NONE',  ( -192.9588430854689989, 10.23066800230756712, -10.23066800230735396 ) ) ;
#10391=CARTESIAN_POINT ( 'NONE',  ( 141.7948666911895259, 30.38861427224637879, -12.58737617328896086 ) ) ;
#10392=CARTESIAN_POINT ( 'NONE',  ( -162.0762913951020892, -41.69427287672991866, -40.00000000000002132 ) ) ;
#10393=CARTESIAN_POINT ( 'NONE',  ( -114.7756899093962062, 16.59394837944376988, -14.65087933325889225 ) ) ;
#10397=CARTESIAN_POINT ( 'NONE',  ( -83.21262154144254453, 33.12752917118434226, -13.72187187061452107 ) ) ;
#10398=CARTESIAN_POINT ( 'NONE',  ( 9.028290303185817933, 18.59346688787791635, 44.88859993222893507 ) ) ;
#10401=PRODUCT ( 'Stator', 'Stator', '', ( #20079 ) ) ;
#10402=CARTESIAN_POINT ( 'NONE',  ( 170.2234770963711128, -24.55285855007184281, -40.00000000000002132 ) ) ;
#10404=CARTESIAN_POINT ( 'NONE',  ( -105.4741150117389594, 7.943527260764311926, 19.77569912954495024 ) ) ;
#10405=CARTESIAN_POINT ( 'NONE',  ( -135.8532207217289738, 50.09629031063965243, -6.472252184284084109 ) ) ;
#10407=CARTESIAN_POINT ( 'NONE',  ( -103.9650464693342826, -8.298274097555776052, -20.03380587592332773 ) ) ;
#10408=CARTESIAN_POINT ( 'NONE',  ( 146.6084372240433993, 8.568076647504290689E-14, -5.374981219216972583 ) ) ;
#10409=CARTESIAN_POINT ( 'NONE',  ( -198.0356074513804572, 40.00000000000014921, -15.37879056873028816 ) ) ;
#10411=SPHERICAL_SURFACE ( 'NONE', #25140, 15.00000000000000000 ) ;
#10413=CARTESIAN_POINT ( 'NONE',  ( -189.1815713358150788, 17.96744347545610410, 43.37724571961807385 ) ) ;
#10414=CARTESIAN_POINT ( 'NONE',  ( -100.7734535825088500, -12.25131212657524316, 44.31723036834888774 ) ) ;
#10415=CARTESIAN_POINT ( 'NONE',  ( -114.4364955367314991, -8.644468109207263495, -20.04994829327655737 ) ) ;
#10416=CARTESIAN_POINT ( 'NONE',  ( 4.995406935893287326, 17.50105314357170627, 39.06748935135200895 ) ) ;
#10417=CARTESIAN_POINT ( 'NONE',  ( -77.78697283798739193, 6.810146944752746734, 20.89074004980727395 ) ) ;
#10419=CARTESIAN_POINT ( 'NONE',  ( 192.4448373802101173, 42.42640687122089815, -14.14213562370272470 ) ) ;
#10421=CARTESIAN_POINT ( 'NONE',  ( 14.38125909742181285, -15.17850393972633505, 40.00000000000002132 ) ) ;
#10422=CARTESIAN_POINT ( 'NONE',  ( -91.56559293963834989, -16.03295912088728414, 16.03295912088688269 ) ) ;
#10423=CARTESIAN_POINT ( 'NONE',  ( -198.0356074513804572, -15.37879056873074290, 40.00000000000002132 ) ) ;
#10424=CARTESIAN_POINT ( 'NONE',  ( -110.0947816603262908, 15.91249765680895045, 12.43490089449757185 ) ) ;
#10425=CARTESIAN_POINT ( 'NONE',  ( -280.0000000000000568, 40.00000000000017764, -19.99999999999959144 ) ) ;
#10426=CARTESIAN_POINT ( 'NONE',  ( -208.1127848780264742, 38.89260858015732936, -17.67593391476642140 ) ) ;
#10427=CARTESIAN_POINT ( 'NONE',  ( 135.5356265174576436, -12.51227922893921196, 30.20731421070332345 ) ) ;
#10428=B_SPLINE_CURVE_WITH_KNOTS ( 'NONE', 3,
 ( #663, #16886, #4798, #21653, #17395, #25534 ),
 .UNSPECIFIED., .F., .F.,
 ( 4, 2, 4 ),
 ( 0.000000000000000000, 0.004519108751124900972, 0.009038217502249801943 ),
 .UNSPECIFIED. ) ;
#10430=ORIENTED_EDGE ( 'NONE', *, *, #16051, .T. ) ;
#10431=ORIENTED_EDGE ( 'NONE', *, *, #20307, .T. ) ;
#10432=CARTESIAN_POINT ( 'NONE',  ( -198.0356074513804572, 15.37879056873066830, 40.00000000000002132 ) ) ;
#10436=CARTESIAN_POINT ( 'NONE',  ( 136.1360204305621551, 31.79587985999232558, 24.77266263493161702 ) ) ;
#10437=CARTESIAN_POINT ( 'NONE',  ( -105.2958943010001605, -20.90688085069862723, -4.721182065470063804 ) ) ;
#10439=CARTESIAN_POINT ( 'NONE',  ( -200.0000000000000000, -55.16984130227027094, 4.865628651907646152 ) ) ;
#10440=CARTESIAN_POINT ( 'NONE',  ( -86.86493150571111244, 7.943527260496201947, -19.77569912839169319 ) ) ;
#10447=CARTESIAN_POINT ( 'NONE',  ( -198.0356074513804572, 10.87444709759730088, -10.87444709759707173 ) ) ;
#10448=CARTESIAN_POINT ( 'NONE',  ( 19.06497207195981858, -38.31983398719641087, 18.24870850772724040 ) ) ;
#10450=CARTESIAN_POINT ( 'NONE',  ( 199.9999999999999432, -1.727494763561684666E-13, 20.00000000000010303 ) ) ;
#10451=CARTESIAN_POINT ( 'NONE',  ( -162.0762913951020607, -57.76657433537922515, -1.198031840455874963 ) ) ;
#10452=CARTESIAN_POINT ( 'NONE',  ( 1.564252679174723770, 14.06374044400962120, 48.56509332159242831 ) ) ;
#10453=CARTESIAN_POINT ( 'NONE',  ( 130.8568914410475372, -24.07718906447255947, 24.07718906447199458 ) ) ;
#10454=CARTESIAN_POINT ( 'NONE',  ( -86.96347745069643054, -41.18208027870589660, -15.38646221621809040 ) ) ;
#10457=CARTESIAN_POINT ( 'NONE',  ( -86.96347745069645896, 39.99999999999994316, 18.24025645688366737 ) ) ;
#10460=CARTESIAN_POINT ( 'NONE',  ( 25.62979979002535202, 45.99287499161375337, -13.63460241473574897 ) ) ;
#10461=CARTESIAN_POINT ( 'NONE',  ( 199.9999999999999432, 19.99999999999996092, 2.449293598294708485E-15 ) ) ;
#10462=CARTESIAN_POINT ( 'NONE',  ( -213.1075012329537230, 9.698598906450410340, 9.698598906450483170 ) ) ;
#10463=CARTESIAN_POINT ( 'NONE',  ( -4.039451493210483690, -23.44932283416618191, -43.00522595894033628 ) ) ;
#10464=( BOUNDED_CURVE ( )  B_SPLINE_CURVE ( 3, ( #5463, #25828, #1221, #9325 ),
 .UNSPECIFIED., .F., .F. ) 
 B_SPLINE_CURVE_WITH_KNOTS ( ( 4, 4 ),
 ( 0.007858036080414859334, 0.01577215542394082640 ),
 .UNSPECIFIED. ) 
 CURVE ( )  GEOMETRIC_REPRESENTATION_ITEM ( )  RATIONAL_B_SPLINE_CURVE ( ( 0.5857864376268567819, 0.5560595459730498513, 0.5340584217468483663, 0.5197830649482524379 ) ) 
 REPRESENTATION_ITEM ( '' )  );
#10465=CARTESIAN_POINT ( 'NONE',  ( -3.615356597027800767, -43.25798660799100759, 17.91804473398356023 ) ) ;
#10466=CARTESIAN_POINT ( 'NONE',  ( 146.6084372240433709, -34.62501878078303008, 40.00000000000002132 ) ) ;
#10468=ORIENTED_EDGE ( 'NONE', *, *, #25887, .F. ) ;
#10469=CARTESIAN_POINT ( 'NONE',  ( 14.33519843538172189, 24.71012982060745955, -44.71104701565624140 ) ) ;
#10470=CARTESIAN_POINT ( 'NONE',  ( 14.38125909742180752, 10.73282306404720465, 10.73282306404724018 ) ) ;
#10471=CARTESIAN_POINT ( 'NONE',  ( -7.726389047727614034, -17.45517700520998972, 42.14052505957891981 ) ) ;
#10472=CARTESIAN_POINT ( 'NONE',  ( -0.6848998192527971929, 24.09453515735949480, -43.87669161505412774 ) ) ;
#10477=CARTESIAN_POINT ( 'NONE',  ( -189.6939645179850515, -18.01965094556746649, 43.50328570201445189 ) ) ;
#10478=CARTESIAN_POINT ( 'NONE',  ( -192.9588430854690273, -18.05360324515400094, -38.51493924976961836 ) ) ;
#10479=CARTESIAN_POINT ( 'NONE',  ( -87.13361725327072804, -21.49321519333431141, -3.542586001259484843E-15 ) ) ;
#10480=CARTESIAN_POINT ( 'NONE',  ( -197.4153392276936358, 24.72549520225541286, -44.73189834455630631 ) ) ;
#10481=CARTESIAN_POINT ( 'NONE',  ( 170.2234770963711128, 10.92277846919147066, 45.64576402573197811 ) ) ;
#10482=CARTESIAN_POINT ( 'NONE',  ( 91.82158438592158234, -12.16597498397778843, 12.16597498397750954 ) ) ;
#10483=CARTESIAN_POINT ( 'NONE',  ( 0.2972598230770129857, -54.33493731733936016, -40.00000000000002132 ) ) ;
#10484=CARTESIAN_POINT ( 'NONE',  ( 19.06497207195980792, 54.19242893257843718, 2.449293598294708485E-15 ) ) ;
#10485=CARTESIAN_POINT ( 'NONE',  ( 57.59792236341147031, -1.493297263419786540E-14, 2.435789363418160658 ) ) ;
#10486=CARTESIAN_POINT ( 'NONE',  ( -86.96347745069644475, 12.89780903124401057, 12.89780903124407629 ) ) ;
#10488=CARTESIAN_POINT ( 'NONE',  ( -88.37877758187934774, 19.92653024472395273, -8.575405934686655129 ) ) ;
#10489=CARTESIAN_POINT ( 'NONE',  ( -208.1127848780264742, -10.60833733270725787, -67.17687982763172272 ) ) ;
#10490=CARTESIAN_POINT ( 'NONE',  ( 19.06497207195980792, 18.24870850772737185, 38.31983398719634692 ) ) ;
#10491=ORIENTED_EDGE ( 'NONE', *, *, #10586, .T. ) ;
#10492=CARTESIAN_POINT ( 'NONE',  ( -192.9588430854689989, 10.23066800230742679, 10.23066800230749607 ) ) ;
#10493=CARTESIAN_POINT ( 'NONE',  ( -86.86493150570990451, 8.366608963953497735, 19.60045294882744216 ) ) ;
#10494=CARTESIAN_POINT ( 'NONE',  ( 163.1118516004056573, 19.27778845539212327, 37.29075403953164169 ) ) ;
#10495=CARTESIAN_POINT ( 'NONE',  ( 20.16956056503174466, -47.86583268169049177, -13.95858718338156734 ) ) ;
#10502=CARTESIAN_POINT ( 'NONE',  ( -188.9524938556191955, -47.22059665006131013, -13.86227398173359759 ) ) ;
#10504=CARTESIAN_POINT ( 'NONE',  ( -30.26275506840323359, -1.535832457777009877E-13, 41.69427246844629309 ) ) ;
#10505=CARTESIAN_POINT ( 'NONE',  ( -30.26275506840324425, 41.69427246844628598, -40.00000000000002132 ) ) ;
#10508=CARTESIAN_POINT ( 'NONE',  ( -213.1075012329537230, -2.291445344039133686E-13, 53.71589010951915100 ) ) ;
#10509=CARTESIAN_POINT ( 'NONE',  ( 0.2972598230769956662, 39.99999999999983658, 54.33493731733950938 ) ) ;
#10511=CARTESIAN_POINT ( 'NONE',  ( -30.26275506840324070, -1.694272468446265112, 0.000000000000000000 ) ) ;
#10512=CARTESIAN_POINT ( 'NONE',  ( -192.9588430854690273, -54.46834944098226572, 40.00000000000002132 ) ) ;
#10513=CARTESIAN_POINT ( 'NONE',  ( -30.26275506840323359, -1.198031551616339341, 57.76657404653985139 ) ) ;
#10514=CARTESIAN_POINT ( 'NONE',  ( 169.9999999999999716, -9.369682556672181306, -22.62041470344887273 ) ) ;
#10516=CARTESIAN_POINT ( 'NONE',  ( 130.8568914410475088, 40.00000000000011369, -5.949712681206269949 ) ) ;
#10517=CARTESIAN_POINT ( 'NONE',  ( -192.9588430854690273, 39.99999999999980105, 54.46834944098235809 ) ) ;
#10519=CARTESIAN_POINT ( 'NONE',  ( 23.37394308801977871, -23.33966569535098046, 42.85717664514577763 ) ) ;
#10520=CARTESIAN_POINT ( 'NONE',  ( 23.37394308801977161, 13.80096434448334186, -46.80823611210181667 ) ) ;
#10521=CARTESIAN_POINT ( 'NONE',  ( -198.0356074513804288, -39.15871834505936278, 39.15871834505892224 ) ) ;
#10523=CARTESIAN_POINT ( 'NONE',  ( -5.152948516936860734, 46.60473671797380746, -13.74948675458147740 ) ) ;
#10524=CARTESIAN_POINT ( 'NONE',  ( 110.0479209278586126, 22.74092928740055441, -9.419601331808626909 ) ) ;
#10525=CARTESIAN_POINT ( 'NONE',  ( -208.1127848780264742, -55.00245453014425578, -40.00000000000002132 ) ) ;
#10526=CARTESIAN_POINT ( 'NONE',  ( 169.9999999999999716, -9.369682556672181306, -22.62041470344887273 ) ) ;
#10532=CARTESIAN_POINT ( 'NONE',  ( -103.9650464692780218, 8.298274099701076878, -20.03380587474480379 ) ) ;
#10533=CARTESIAN_POINT ( 'NONE',  ( 16.10036699856469156, 24.53427828609990513, 44.47262139759975241 ) ) ;
#10534=B_SPLINE_CURVE_WITH_KNOTS ( 'NONE', 3,
 ( #12761, #14487, #20886, #10906, #22880, #8502, #22749, #14881, #6368, #4917, #24749, #16489 ),
 .UNSPECIFIED., .F., .F.,
 ( 4, 2, 2, 2, 2, 4 ),
 ( -5.998499568707339487E-08, 0.003531500499830289921, 0.007063060984656267458, 0.01412618195430823294, 0.02118930292396019321, 0.02825242389361215523 ),
 .UNSPECIFIED. ) ;
#10535=ORIENTED_EDGE ( 'NONE', *, *, #12719, .F. ) ;
#10537=CARTESIAN_POINT ( 'NONE',  ( -198.0356074513804572, 10.87444709758468875, 67.44298959250869530 ) ) ;
#10540=CARTESIAN_POINT ( 'NONE',  ( -208.1127848780265026, 10.60833733269537049, 10.60833733269544510 ) ) ;
#10541=CARTESIAN_POINT ( 'NONE',  ( 163.1118516004056573, 37.29075403953160617, -19.27778845539222985 ) ) ;
#10545=CARTESIAN_POINT ( 'NONE',  ( 19.06497207195980792, 40.00000000000059686, -54.19242893257802507 ) ) ;
#10546=CARTESIAN_POINT ( 'NONE',  ( -280.0000000000000568, 40.00000000000017764, -19.99999999999959144 ) ) ;
#10550=CARTESIAN_POINT ( 'NONE',  ( -188.2506440019886327, 23.43978047293197164, 42.99080317017340747 ) ) ;
#10551=CARTESIAN_POINT ( 'NONE',  ( -135.8532207217289738, 6.472252184284096543, 6.472252184284234211 ) ) ;
#10552=CARTESIAN_POINT ( 'NONE',  ( -105.3844635032202461, 6.703103239450354245, -20.33704783843148434 ) ) ;
#10553=CARTESIAN_POINT ( 'NONE',  ( -213.1075012329537230, -9.698598906438496314, 66.26714140136188291 ) ) ;
#10554=CARTESIAN_POINT ( 'NONE',  ( -77.55640685876510076, 0.6996548653659642181, 22.13135000837105082 ) ) ;
#10555=CARTESIAN_POINT ( 'NONE',  ( -91.56559293963836410, 44.31723036834908669, -12.25131212657445801 ) ) ;
#10556=CARTESIAN_POINT ( 'NONE',  ( -200.0000000000000568, 46.38610861938607144, -18.14877749763654080 ) ) ;
#10557=CARTESIAN_POINT ( 'NONE',  ( 136.1360204305621266, 35.03383547441298873, 0.000000000000000000 ) ) ;
#10558=CARTESIAN_POINT ( 'NONE',  ( 200.0000000000000000, 14.14213562373041455, 42.42640687119311593 ) ) ;
#10559=CARTESIAN_POINT ( 'NONE',  ( -192.9588430854689989, -14.46834944099973086, 0.000000000000000000 ) ) ;
#10561=CARTESIAN_POINT ( 'NONE',  ( -30.26275506840323359, 4.336144384597734078E-13, -41.69427246844629309 ) ) ;
#10563=CARTESIAN_POINT ( 'NONE',  ( 167.0466155511619775, -9.710058186602013919, 23.44215416552578901 ) ) ;
#10564=EDGE_LOOP ( 'NONE', ( #13065, #4415, #10662, #21240 ) ) ;
#10565=ORIENTED_EDGE ( 'NONE', *, *, #1189, .F. ) ;
#10566=CARTESIAN_POINT ( 'NONE',  ( 163.1118516004056573, -27.26290988616869626, 0.000000000000000000 ) ) ;
#10568=VECTOR ( 'NONE', #18182, 1000.000000000000000 ) ;
#10569=( BOUNDED_SURFACE ( )  B_SPLINE_SURFACE ( 3, 3, ( 
 ( #9920, #1552, #21513, #3285, #23631, #17761, #9789, #15892, #24020, #11917, #20167, #8450, #18163, #16033, #12441, #14308, #24158, #16569, #2215, #14570, #1949, #22700, #4083, #12577, #18432, #6071, #10056, #24566, #16169, #6195 ),
 ( #14042, #20569, #5935, #18293, #4475, #22176, #4220, #20707, #18699, #10189, #79, #2342, #12184, #20305, #6321, #22442, #10324, #14442, #22306, #24700, #14173, #8189, #12047, #2473, #7915, #208, #3950, #12310, #8317, #18567 ),
 ( #10583, #24304, #16305, #26309, #8052, #346, #2082, #24429, #20437, #16440, #22571, #4349, #10454, #6455, #18836, #14705, #882, #4613, #23357, #8992, #25228, #20969, #12709, #615, #14833, #23229, #11234, #15226, #13239, #18971 ),
 ( #20837, #22838, #6852, #2612, #24832, #17222, #10725, #1008, #8721, #8589, #5007, #14969, #16700, #9111, #21102, #7115, #16839, #5134, #22965, #21364, #10990, #24972, #6721, #17096, #4745, #3131, #2749, #6981, #12851, #6585 ),
 ( #751, #10853, #16967, #483, #25103, #8855, #23104, #4876, #12979, #19099, #2882, #15096, #13112, #21233, #3006, #11114, #19228, #25361, #17352, #5256, #9763, #11614, #7751, #17476, #26014, #25488, #11751, #19736, #15862, #23991 ),
 ( #17600, #5771, #7237, #9246, #23482, #11480, #15358, #13879, #19872, #13358, #22012, #5382, #19608, #1523, #1141, #9631, #23603, #21480, #1654, #13742, #1262, #3255, #17732, #17863, #3645, #1394, #25873, #15732, #11359, #13487 ),
 ( #3783, #19352, #7617, #7364, #23858, #19476, #9495, #21608, #9366, #15602, #3382, #25618, #15476, #25741, #13610, #7491, #23727, #5508, #21738, #3514, #5635, #21868, #12023, #2189, #321, #4193, #20143, #6297, #24541, #5906 ) ),
 .UNSPECIFIED., .T., .F., .F. ) 
 B_SPLINE_SURFACE_WITH_KNOTS ( ( 4, 3, 4 ),
 ( 4, 2, 2, 2, 2, 2, 2, 2, 2, 2, 2, 2, 2, 2, 4 ),
 ( 0.000000000000000000, 0.5000000000000000000, 1.000000000000000000 ),
 ( 0.000000000000000000, 0.1357259735107005372, 0.1651108541090157700, 0.1944957347073310028, 0.3598804999793158710, 0.3867117631979620773, 0.4135430264166082281, 0.5789277916885930964, 0.6062785021374117456, 0.6336292125862302838, 0.8508620842112317728, 0.8814014469398914198, 0.9119408096685510667, 0.9559704048342755334, 1.000000000000000000 ),
 .UNSPECIFIED. ) 
 GEOMETRIC_REPRESENTATION_ITEM ( )  RATIONAL_B_SPLINE_SURFACE ( (
 ( 1.000000000000000000, 1.000000000000000000, 1.000000000000000000, 1.000000000000000000, 1.000000000000000000, 1.000000000000000000, 1.000000000000000000, 1.000000000000000000, 1.000000000000000000, 1.000000000000000000, 1.000000000000000000, 1.000000000000000000, 1.000000000000000000, 1.000000000000000000, 1.000000000000000000, 1.000000000000000000, 1.000000000000000000, 1.000000000000000000, 1.000000000000000000, 1.000000000000000000, 1.000000000000000000, 1.000000000000000000, 1.000000000000000000, 1.000000000000000000, 1.000000000000000000, 1.000000000000000000, 1.000000000000000000, 1.000000000000000000, 1.000000000000000000, 1.000000000000000000),
 ( 0.3333333333333333703, 0.3333333333333333703, 0.3333333333333333703, 0.3333333333333333703, 0.3333333333333333703, 0.3333333333333333703, 0.3333333333333333703, 0.3333333333333333703, 0.3333333333333333703, 0.3333333333333333703, 0.3333333333333333703, 0.3333333333333333703, 0.3333333333333333703, 0.3333333333333333703, 0.3333333333333333703, 0.3333333333333333703, 0.3333333333333333703, 0.3333333333333333703, 0.3333333333333333703, 0.3333333333333333703, 0.3333333333333333703, 0.3333333333333333703, 0.3333333333333333703, 0.3333333333333333703, 0.3333333333333333703, 0.3333333333333333703, 0.3333333333333333703, 0.3333333333333333703, 0.3333333333333333703, 0.3333333333333333703),
 ( 0.3333333333333333703, 0.3333333333333333703, 0.3333333333333333703, 0.3333333333333333703, 0.3333333333333333703, 0.3333333333333333703, 0.3333333333333333703, 0.3333333333333333703, 0.3333333333333333703, 0.3333333333333333703, 0.3333333333333333703, 0.3333333333333333703, 0.3333333333333333703, 0.3333333333333333703, 0.3333333333333333703, 0.3333333333333333703, 0.3333333333333333703, 0.3333333333333333703, 0.3333333333333333703, 0.3333333333333333703, 0.3333333333333333703, 0.3333333333333333703, 0.3333333333333333703, 0.3333333333333333703, 0.3333333333333333703, 0.3333333333333333703, 0.3333333333333333703, 0.3333333333333333703, 0.3333333333333333703, 0.3333333333333333703),
 ( 1.000000000000000000, 1.000000000000000000, 1.000000000000000000, 1.000000000000000000, 1.000000000000000000, 1.000000000000000000, 1.000000000000000000, 1.000000000000000000, 1.000000000000000000, 1.000000000000000000, 1.000000000000000000, 1.000000000000000000, 1.000000000000000000, 1.000000000000000000, 1.000000000000000000, 1.000000000000000000, 1.000000000000000000, 1.000000000000000000, 1.000000000000000000, 1.000000000000000000, 1.000000000000000000, 1.000000000000000000, 1.000000000000000000, 1.000000000000000000, 1.000000000000000000, 1.000000000000000000, 1.000000000000000000, 1.000000000000000000, 1.000000000000000000, 1.000000000000000000),
 ( 0.3333333333333333703, 0.3333333333333333703, 0.3333333333333333703, 0.3333333333333333703, 0.3333333333333333703, 0.3333333333333333703, 0.3333333333333333703, 0.3333333333333333703, 0.3333333333333333703, 0.3333333333333333703, 0.3333333333333333703, 0.3333333333333333703, 0.3333333333333333703, 0.3333333333333333703, 0.3333333333333333703, 0.3333333333333333703, 0.3333333333333333703, 0.3333333333333333703, 0.3333333333333333703, 0.3333333333333333703, 0.3333333333333333703, 0.3333333333333333703, 0.3333333333333333703, 0.3333333333333333703, 0.3333333333333333703, 0.3333333333333333703, 0.3333333333333333703, 0.3333333333333333703, 0.3333333333333333703, 0.3333333333333333703),
 ( 0.3333333333333333703, 0.3333333333333333703, 0.3333333333333333703, 0.3333333333333333703, 0.3333333333333333703, 0.3333333333333333703, 0.3333333333333333703, 0.3333333333333333703, 0.3333333333333333703, 0.3333333333333333703, 0.3333333333333333703, 0.3333333333333333703, 0.3333333333333333703, 0.3333333333333333703, 0.3333333333333333703, 0.3333333333333333703, 0.3333333333333333703, 0.3333333333333333703, 0.3333333333333333703, 0.3333333333333333703, 0.3333333333333333703, 0.3333333333333333703, 0.3333333333333333703, 0.3333333333333333703, 0.3333333333333333703, 0.3333333333333333703, 0.3333333333333333703, 0.3333333333333333703, 0.3333333333333333703, 0.3333333333333333703),
 ( 1.000000000000000000, 1.000000000000000000, 1.000000000000000000, 1.000000000000000000, 1.000000000000000000, 1.000000000000000000, 1.000000000000000000, 1.000000000000000000, 1.000000000000000000, 1.000000000000000000, 1.000000000000000000, 1.000000000000000000, 1.000000000000000000, 1.000000000000000000, 1.000000000000000000, 1.000000000000000000, 1.000000000000000000, 1.000000000000000000, 1.000000000000000000, 1.000000000000000000, 1.000000000000000000, 1.000000000000000000, 1.000000000000000000, 1.000000000000000000, 1.000000000000000000, 1.000000000000000000, 1.000000000000000000, 1.000000000000000000, 1.000000000000000000, 1.000000000000000000) ) ) 
 REPRESENTATION_ITEM ( '' )  SURFACE ( )  );
#10570=CARTESIAN_POINT ( 'NONE',  ( 91.82158438592158234, 16.11829626346161604, -16.11829626346121103 ) ) ;
#10571=CARTESIAN_POINT ( 'NONE',  ( -110.1017491837608446, -20.19444236859277098, -1.278135197240527043 ) ) ;
#10572=CARTESIAN_POINT ( 'NONE',  ( -199.9999999999999147, -53.44529986889379103, 10.02640517461957614 ) ) ;
#10576=CARTESIAN_POINT ( 'NONE',  ( -91.56559293963834989, -44.31723036834885932, -12.25131212657538171 ) ) ;
#10577=CARTESIAN_POINT ( 'NONE',  ( -208.1127848780265026, -10.60833733269537227, -10.60833733269551793 ) ) ;
#10578=CARTESIAN_POINT ( 'NONE',  ( -114.7792487060331865, 22.11287803872790647, 1.644740498667294881 ) ) ;
#10579=CARTESIAN_POINT ( 'NONE',  ( 146.6084372240433709, 40.00000000000010658, -5.374981219216549810 ) ) ;
#10580=CARTESIAN_POINT ( 'NONE',  ( -94.58366989427227622, -8.190486896679354700, 20.91926462023902999 ) ) ;
#10581=CARTESIAN_POINT ( 'NONE',  ( 170.2234770963711128, 24.55285855007190321, 0.000000000000000000 ) ) ;
#10582=CARTESIAN_POINT ( 'NONE',  ( -56.48582580120559271, -6.472252184284187138, -6.472252184284199572 ) ) ;
#10583=CARTESIAN_POINT ( 'NONE',  ( -280.0000000000000568, -42.42640687119285303, -14.14213562373118371 ) ) ;
#10584=CARTESIAN_POINT ( 'NONE',  ( -100.7734535825088500, 22.67402823373189591, -0.000000000000000000 ) ) ;
#10585=CIRCLE ( 'NONE', #19088, 15.00000000000000000 ) ;
#10586=EDGE_CURVE ( 'NONE', #9969, #11726, #10464, .T. ) ;
#10588=CARTESIAN_POINT ( 'NONE',  ( -30.26275506840324425, 39.99999999999987210, 41.69427246844643520 ) ) ;
#10590=CARTESIAN_POINT ( 'NONE',  ( 22.76403192593601688, 43.17745271018617359, -17.88468650128181991 ) ) ;
#10591=CARTESIAN_POINT ( 'NONE',  ( -100.7734535825088500, -22.67402823373193499, -40.00000000000002132 ) ) ;
#10592=CARTESIAN_POINT ( 'NONE',  ( -105.3755690713226585, -43.67073346367983788, 12.89780903124397149 ) ) ;
#10593=CARTESIAN_POINT ( 'NONE',  ( -100.7734535825088500, 17.32597176626808988, 40.00000000000002132 ) ) ;
#10594=AXIS2_PLACEMENT_3D ( 'NONE', #23196, #15199, #17190 ) ;
#10596=CARTESIAN_POINT ( 'NONE',  ( -4.558244102846490620, -42.85231560262746342, 23.34817229226001345 ) ) ;
#10597=CARTESIAN_POINT ( 'NONE',  ( 170.2234770963711128, 15.44714144992818738, 40.00000000000002132 ) ) ;
#10600=CARTESIAN_POINT ( 'NONE',  ( -190.1760961843813789, -47.67020129257696937, -13.92889018389476874 ) ) ;
#10601=CARTESIAN_POINT ( 'NONE',  ( -100.7734535825088358, -16.03295912088706743, -16.03295912088710296 ) ) ;
#10602=CARTESIAN_POINT ( 'NONE',  ( -5.379830816902669177, -13.73345071524718897, 46.52611083736134390 ) ) ;
#10603=CARTESIAN_POINT ( 'NONE',  ( -4.660840668352909333, 23.32816686155626584, -42.82207049670912369 ) ) ;
#10605=CARTESIAN_POINT ( 'NONE',  ( -30.26275506840324070, 1.198031551616030033, -1.198031551616006496 ) ) ;
#10606=CARTESIAN_POINT ( 'NONE',  ( -82.30220482034327745, 7.441767004318980305, -18.74474319042418458 ) ) ;
#10607=CARTESIAN_POINT ( 'NONE',  ( -65.65555754753494000, -24.04429191298299884, -11.16466304451123825 ) ) ;
#10608=CARTESIAN_POINT ( 'NONE',  ( -190.0144721487978643, -23.79987203025130071, 43.47822244619790411 ) ) ;
#10609=FACE_OUTER_BOUND ( 'NONE', #16517, .T. ) ;
#10611=CARTESIAN_POINT ( 'NONE',  ( 163.1118516004056573, -19.27778845539181063, -37.29075403953176959 ) ) ;
#10613=CARTESIAN_POINT ( 'NONE',  ( -199.0730705747853051, 18.57195860668882048, -44.83667434815284736 ) ) ;
#10614=CARTESIAN_POINT ( 'NONE',  ( 170.2234770963711128, 10.92277846919216522, -10.92277846919186501 ) ) ;
#10615=CARTESIAN_POINT ( 'NONE',  ( 130.8568914410475372, -24.07718906447255947, 24.07718906447199458 ) ) ;
#10616=CARTESIAN_POINT ( 'NONE',  ( -198.0356074513804288, -55.37879056873077133, -2.449293598294708485E-15 ) ) ;
#10617=CARTESIAN_POINT ( 'NONE',  ( 170.2234770963711128, 15.44714144992819094, 2.449293598294708485E-15 ) ) ;
#10618=CARTESIAN_POINT ( 'NONE',  ( -280.0000000000000568, -40.00000000000028422, 19.99999999999959499 ) ) ;
#10619=CARTESIAN_POINT ( 'NONE',  ( -135.8532207217289738, 21.81201906317777883, -34.75652343174605363 ) ) ;
#10621=( BOUNDED_SURFACE ( )  B_SPLINE_SURFACE ( 3, 3, ( 
 ( #5027, #25249, #23252, #15689, #13702, #9329, #21323, #11442, #19690, #1225, #5596, #15564, #5467, #11198, #23689, #7577, #13321, #23320, #15437, #17316, #3096, #13570, #7450, #17561, #23564, #25699, #17439, #21696, #21568, #21441 ),
 ( #9584, #23814, #7080, #3341, #3216, #21827, #25448, #3597, #19438, #19826, #25577, #7323, #11705, #19564, #5096, #5339, #13449, #1356, #9455, #7200, #1612, #3472, #1478, #11571, #17689, #19312, #13201, #11322, #25832, #9716 ),
 ( #1095, #9205, #15315, #25321, #15193, #23441, #5217, #4279, #17820, #24361, #22235, #7708, #4010, #23946, #10117, #7976, #5999, #24495, #2140, #8116, #9981, #11976, #16094, #18090, #1742, #12109, #25968, #10251, #18360, #139 ),
 ( #7836, #12369, #18218, #8243, #16361, #26241, #16232, #14233, #5724, #3874, #3735, #22373, #4149, #24225, #11838, #6256, #15960, #14105, #13828, #14369, #20497, #15819, #21961, #22500, #2640, #4, #6125, #24085, #20100, #20234 ),
 ( #1878, #2013, #19958, #9850, #17953, #12242, #20366, #26100, #5859, #13965, #22100, #21129, #13260, #9266, #18859, #21256, #14859, #13380, #15123, #21383, #23381, #10748, #904, #24994, #6875, #22993, #17247, #25513, #17374, #3155 ),
 ( #19252, #3028, #9016, #11136, #2904, #1032, #7003, #14991, #15251, #9132, #7260, #25384, #11257, #5275, #7136, #19375, #640, #4769, #12874, #23501, #1163, #16990, #17121, #2772, #6747, #21507, #11012, #25252, #5155, #10882 ),
 ( #15378, #19122, #8744, #16862, #23254, #20990, #18996, #8879, #5030, #773, #25125, #23126, #4898, #13007, #13137, #5930, #21890, #9783, #1414, #15623, #1545, #3666, #7384, #26169, #11775, #25765, #23746, #11911, #17885, #7910 ) ),
 .UNSPECIFIED., .T., .F., .F. ) 
 B_SPLINE_SURFACE_WITH_KNOTS ( ( 4, 3, 4 ),
 ( 4, 2, 2, 2, 2, 2, 2, 2, 2, 2, 2, 2, 2, 2, 4 ),
 ( 0.000000000000000000, 0.5000000000000000000, 1.000000000000000000 ),
 ( 0.000000000000000000, 0.1357259735107005372, 0.1651108541090157700, 0.1944957347073310028, 0.3598804999793158710, 0.3867117631979620773, 0.4135430264166082281, 0.5789277916885930964, 0.6062785021374117456, 0.6336292125862302838, 0.8508620842112317728, 0.8814014469398914198, 0.9119408096685510667, 0.9559704048342755334, 1.000000000000000000 ),
 .UNSPECIFIED. ) 
 GEOMETRIC_REPRESENTATION_ITEM ( )  RATIONAL_B_SPLINE_SURFACE ( (
 ( 1.000000000000000000, 1.000000000000000000, 1.000000000000000000, 1.000000000000000000, 1.000000000000000000, 1.000000000000000000, 1.000000000000000000, 1.000000000000000000, 1.000000000000000000, 1.000000000000000000, 1.000000000000000000, 1.000000000000000000, 1.000000000000000000, 1.000000000000000000, 1.000000000000000000, 1.000000000000000000, 1.000000000000000000, 1.000000000000000000, 1.000000000000000000, 1.000000000000000000, 1.000000000000000000, 1.000000000000000000, 1.000000000000000000, 1.000000000000000000, 1.000000000000000000, 1.000000000000000000, 1.000000000000000000, 1.000000000000000000, 1.000000000000000000, 1.000000000000000000),
 ( 0.3333333333333333703, 0.3333333333333333703, 0.3333333333333333703, 0.3333333333333333703, 0.3333333333333333703, 0.3333333333333333703, 0.3333333333333333703, 0.3333333333333333703, 0.3333333333333333703, 0.3333333333333333703, 0.3333333333333333703, 0.3333333333333333703, 0.3333333333333333703, 0.3333333333333333703, 0.3333333333333333703, 0.3333333333333333703, 0.3333333333333333703, 0.3333333333333333703, 0.3333333333333333703, 0.3333333333333333703, 0.3333333333333333703, 0.3333333333333333703, 0.3333333333333333703, 0.3333333333333333703, 0.3333333333333333703, 0.3333333333333333703, 0.3333333333333333703, 0.3333333333333333703, 0.3333333333333333703, 0.3333333333333333703),
 ( 0.3333333333333333703, 0.3333333333333333703, 0.3333333333333333703, 0.3333333333333333703, 0.3333333333333333703, 0.3333333333333333703, 0.3333333333333333703, 0.3333333333333333703, 0.3333333333333333703, 0.3333333333333333703, 0.3333333333333333703, 0.3333333333333333703, 0.3333333333333333703, 0.3333333333333333703, 0.3333333333333333703, 0.3333333333333333703, 0.3333333333333333703, 0.3333333333333333703, 0.3333333333333333703, 0.3333333333333333703, 0.3333333333333333703, 0.3333333333333333703, 0.3333333333333333703, 0.3333333333333333703, 0.3333333333333333703, 0.3333333333333333703, 0.3333333333333333703, 0.3333333333333333703, 0.3333333333333333703, 0.3333333333333333703),
 ( 1.000000000000000000, 1.000000000000000000, 1.000000000000000000, 1.000000000000000000, 1.000000000000000000, 1.000000000000000000, 1.000000000000000000, 1.000000000000000000, 1.000000000000000000, 1.000000000000000000, 1.000000000000000000, 1.000000000000000000, 1.000000000000000000, 1.000000000000000000, 1.000000000000000000, 1.000000000000000000, 1.000000000000000000, 1.000000000000000000, 1.000000000000000000, 1.000000000000000000, 1.000000000000000000, 1.000000000000000000, 1.000000000000000000, 1.000000000000000000, 1.000000000000000000, 1.000000000000000000, 1.000000000000000000, 1.000000000000000000, 1.000000000000000000, 1.000000000000000000),
 ( 0.3333333333333333703, 0.3333333333333333703, 0.3333333333333333703, 0.3333333333333333703, 0.3333333333333333703, 0.3333333333333333703, 0.3333333333333333703, 0.3333333333333333703, 0.3333333333333333703, 0.3333333333333333703, 0.3333333333333333703, 0.3333333333333333703, 0.3333333333333333703, 0.3333333333333333703, 0.3333333333333333703, 0.3333333333333333703, 0.3333333333333333703, 0.3333333333333333703, 0.3333333333333333703, 0.3333333333333333703, 0.3333333333333333703, 0.3333333333333333703, 0.3333333333333333703, 0.3333333333333333703, 0.3333333333333333703, 0.3333333333333333703, 0.3333333333333333703, 0.3333333333333333703, 0.3333333333333333703, 0.3333333333333333703),
 ( 0.3333333333333333703, 0.3333333333333333703, 0.3333333333333333703, 0.3333333333333333703, 0.3333333333333333703, 0.3333333333333333703, 0.3333333333333333703, 0.3333333333333333703, 0.3333333333333333703, 0.3333333333333333703, 0.3333333333333333703, 0.3333333333333333703, 0.3333333333333333703, 0.3333333333333333703, 0.3333333333333333703, 0.3333333333333333703, 0.3333333333333333703, 0.3333333333333333703, 0.3333333333333333703, 0.3333333333333333703, 0.3333333333333333703, 0.3333333333333333703, 0.3333333333333333703, 0.3333333333333333703, 0.3333333333333333703, 0.3333333333333333703, 0.3333333333333333703, 0.3333333333333333703, 0.3333333333333333703, 0.3333333333333333703),
 ( 1.000000000000000000, 1.000000000000000000, 1.000000000000000000, 1.000000000000000000, 1.000000000000000000, 1.000000000000000000, 1.000000000000000000, 1.000000000000000000, 1.000000000000000000, 1.000000000000000000, 1.000000000000000000, 1.000000000000000000, 1.000000000000000000, 1.000000000000000000, 1.000000000000000000, 1.000000000000000000, 1.000000000000000000, 1.000000000000000000, 1.000000000000000000, 1.000000000000000000, 1.000000000000000000, 1.000000000000000000, 1.000000000000000000, 1.000000000000000000, 1.000000000000000000, 1.000000000000000000, 1.000000000000000000, 1.000000000000000000, 1.000000000000000000, 1.000000000000000000) ) ) 
 REPRESENTATION_ITEM ( '' )  SURFACE ( )  );
#10622=CARTESIAN_POINT ( 'NONE',  ( 98.29850319112431123, -7.044854747019780206, 18.72964005471164128 ) ) ;
#10624=CARTESIAN_POINT ( 'NONE',  ( 146.6084372240433709, 24.48358557860356655, -32.08495691632035118 ) ) ;
#10626=CARTESIAN_POINT ( 'NONE',  ( -114.4944481313176823, -7.435744517473530379, 20.59122811151904031 ) ) ;
#10627=ORIENTED_EDGE ( 'NONE', *, *, #21919, .F. ) ;
#10628=CARTESIAN_POINT ( 'NONE',  ( -280.0000000000000568, 42.42640687119285303, -14.14213562373088351 ) ) ;
#10631=CARTESIAN_POINT ( 'NONE',  ( 57.59792236341148453, -26.56190807104700369, 26.56190807104673723 ) ) ;
#10632=CARTESIAN_POINT ( 'NONE',  ( 11.59303701482569338, -44.86219070952746790, -18.58252782965046279 ) ) ;
#10634=ADVANCED_FACE ( 'NONE', ( #11318 ), #22363, .T. ) ;
#10635=EDGE_LOOP ( 'NONE', ( #988, #18785, #18471, #9063 ) ) ;
#10636=CARTESIAN_POINT ( 'NONE',  ( 14.38125909742180752, 15.17850393972634038, 0.000000000000000000 ) ) ;
#10641=CARTESIAN_POINT ( 'NONE',  ( -114.7756899093957799, -22.09342955265395858, 1.373957298914630032 ) ) ;
#10642=CARTESIAN_POINT ( 'NONE',  ( -91.56559293963834989, 17.32597176626809343, 2.449293598294708485E-15 ) ) ;
#10645=CARTESIAN_POINT ( 'NONE',  ( -30.26275506840322294, -57.76657404653985139, -1.198031551616531853 ) ) ;
#10646=CARTESIAN_POINT ( 'NONE',  ( 146.6084372240433993, 5.715592784339989804E-15, 5.374981219216972583 ) ) ;
#10647=CARTESIAN_POINT ( 'NONE',  ( 57.59792236341147031, 39.99999999999990763, 37.56421063658199699 ) ) ;
#10650=CARTESIAN_POINT ( 'NONE',  ( -198.0356074513804572, -10.87444709759729911, 10.87444709759714812 ) ) ;
#10651=CARTESIAN_POINT ( 'NONE',  ( -198.0356074513804288, -55.37879056873077133, -2.449293598294708485E-15 ) ) ;
#10652=CARTESIAN_POINT ( 'NONE',  ( -100.7734535825088358, -12.25131212657493052, 12.25131212657478130 ) ) ;
#10653=CARTESIAN_POINT ( 'NONE',  ( -162.0762913951020892, -1.202636532414034422E-14, -1.694272876828323948 ) ) ;
#10655=CARTESIAN_POINT ( 'NONE',  ( -105.2055636156081277, 14.22328983909173061, -16.17146666062084037 ) ) ;
#10656=CARTESIAN_POINT ( 'NONE',  ( 163.1118516004056573, 40.00000000000017764, -12.73709011382432976 ) ) ;
#10657=CARTESIAN_POINT ( 'NONE',  ( -198.0356074513804572, -40.00000000000025580, 55.37879056871310013 ) ) ;
#10658=CARTESIAN_POINT ( 'NONE',  ( 130.8568914410475372, -24.07718906447222551, -24.07718906447233209 ) ) ;
#10661=CARTESIAN_POINT ( 'NONE',  ( -135.8532207217289738, -50.09629031063965243, -6.472252184284438492 ) ) ;
#10662=ORIENTED_EDGE ( 'NONE', *, *, #11501, .F. ) ;
#10663=CARTESIAN_POINT ( 'NONE',  ( -196.0240701155047702, 24.63338802315957565, -44.60678452943314198 ) ) ;
#10665=CARTESIAN_POINT ( 'NONE',  ( 146.6084372240433709, 34.62501878078307982, -40.00000000000002132 ) ) ;
#10666=CARTESIAN_POINT ( 'NONE',  ( -114.7827960788991959, 16.12461489703415651, -15.17504536826869987 ) ) ;
#10667=CARTESIAN_POINT ( 'NONE',  ( -135.8532207217289738, -6.472252184284280396, 6.472252184284099208 ) ) ;
#10669=ORIENTED_EDGE ( 'NONE', *, *, #3298, .T. ) ;
#10671=CARTESIAN_POINT ( 'NONE',  ( 127.8236149080042310, 11.91256696755868205, -28.75948073575747443 ) ) ;
#10672=CARTESIAN_POINT ( 'NONE',  ( 8.209392600923674621, 14.17653494426514804, 49.31072049264779622 ) ) ;
#10674=ORIENTED_EDGE ( 'NONE', *, *, #22495, .T. ) ;
#10675=CARTESIAN_POINT ( 'NONE',  ( 57.59792236341147031, -30.00663442387700641, 26.56190807104681895 ) ) ;
#10677=CARTESIAN_POINT ( 'NONE',  ( -114.7538884076128340, -2.777513412055030884, 21.97380054627827306 ) ) ;
#10678=CARTESIAN_POINT ( 'NONE',  ( 184.8905102610680444, -43.07788698682576722, 13.49065550809799063 ) ) ;
#10679=CIRCLE ( 'NONE', #14057, 14.99999999999999822 ) ;
#10682=CARTESIAN_POINT ( 'NONE',  ( 184.8905102610680444, 40.00000000000013500, -20.92133201514430141 ) ) ;
#10683=SPHERICAL_SURFACE ( 'NONE', #16017, 15.00000000000000000 ) ;
#10685=CARTESIAN_POINT ( 'NONE',  ( 184.8905102610680444, 40.00000000000025580, -19.07866798485515503 ) ) ;
#10686=CARTESIAN_POINT ( 'NONE',  ( 19.06497207195979726, 40.00000000000017053, -14.19242893257798599 ) ) ;
#10690=CARTESIAN_POINT ( 'NONE',  ( -188.4701769959791022, 23.48627020870861770, 43.05504096897863064 ) ) ;
#10691=CARTESIAN_POINT ( 'NONE',  ( 136.1360204305621266, 24.77266263493104148, 24.77266263493145004 ) ) ;
#10692=CARTESIAN_POINT ( 'NONE',  ( -77.90255099906769942, -20.04994828523962269, 8.644468104261498809 ) ) ;
#10693=CARTESIAN_POINT ( 'NONE',  ( 192.4448373802100889, -14.14213562370313682, 14.14213562370301958 ) ) ;
#10696=CARTESIAN_POINT ( 'NONE',  ( -198.0356074513804288, -39.15871834505882276, -39.15871834505946936 ) ) ;
#10698=CARTESIAN_POINT ( 'NONE',  ( 163.1118516004056573, 27.26290988616876021, 40.00000000000002132 ) ) ;
#10699=CARTESIAN_POINT ( 'NONE',  ( 184.8905102610680444, 13.49065550809757497, 43.07788698682593065 ) ) ;
#10701=CARTESIAN_POINT ( 'NONE',  ( -135.8532207217289738, 9.153146818113546246, -0.000000000000000000 ) ) ;
#10704=CARTESIAN_POINT ( 'NONE',  ( -238.4067589809705794, -39.99999999999963762, -40.96449428006383187 ) ) ;
#10706=CARTESIAN_POINT ( 'NONE',  ( 133.2080217031555094, -12.38638889282761291, 29.90338805389101751 ) ) ;
#10709=VERTEX_POINT ( 'NONE', #24453 ) ;
#10710=CARTESIAN_POINT ( 'NONE',  ( 0.2972598230769930017, 54.33493731733936016, 40.00000000000002132 ) ) ;
#10711=AXIS2_PLACEMENT_3D ( 'NONE', #24483, #7825, #4267 ) ;
#10712=CARTESIAN_POINT ( 'NONE',  ( -110.0574180500383079, -19.22461201380497187, 6.256710540534125009 ) ) ;
#10713=B_SPLINE_CURVE_WITH_KNOTS ( 'NONE', 3,
 ( #12036, #4465, #22294, #22690, #22431, #26298, #14559, #12561, #20155, #20694, #8038, #2461 ),
 .UNSPECIFIED., .F., .F.,
 ( 4, 2, 2, 2, 2, 4 ),
 ( 2.797157557069881010E-17, 0.005971652981263739571, 0.008957479471895556447, 0.01045039271721150131, 0.01119684933986943645, 0.01194330596252737159 ),
 .UNSPECIFIED. ) ;
#10714=CARTESIAN_POINT ( 'NONE',  ( 116.7964245048383702, -19.78678521258524725, -19.78678521258533607 ) ) ;
#10717=CARTESIAN_POINT ( 'NONE',  ( -105.3841230195789791, 6.698392286129924322, -20.33917976067976596 ) ) ;
#10718=CARTESIAN_POINT ( 'NONE',  ( 184.8905102610680444, -43.07788698682556827, -13.49065550809859104 ) ) ;
#10719=CARTESIAN_POINT ( 'NONE',  ( -259.2033419157646676, 6.730120644403426944, 6.730120644403592145 ) ) ;
#10720=CARTESIAN_POINT ( 'NONE',  ( -114.5516905194150183, -19.58901826161396187, -9.952133121982182473 ) ) ;
#10721=CARTESIAN_POINT ( 'NONE',  ( -105.3755690713226585, 40.00000000000019185, -18.24025645688310249 ) ) ;
#10722=CARTESIAN_POINT ( 'NONE',  ( 170.2234770963711128, -10.92277846919235529, 45.64576402573175073 ) ) ;
#10723=CARTESIAN_POINT ( 'NONE',  ( -1.258540240222673523, 13.96099832920788764, 47.88180740053026341 ) ) ;
#10725=CARTESIAN_POINT ( 'NONE',  ( -192.9588430854689705, -38.51493924976963967, 38.51493924976919914 ) ) ;
#10728=CARTESIAN_POINT ( 'NONE',  ( -259.2033419157646676, -1.438356298054549103E-14, -9.517827891722632216 ) ) ;
#10730=CARTESIAN_POINT ( 'NONE',  ( 67.67011021033935947, 29.29769665555166469, -12.13550330100044583 ) ) ;
#10731=CARTESIAN_POINT ( 'NONE',  ( 136.1360204305621266, -35.03383547441293899, 0.000000000000000000 ) ) ;
#10732=CARTESIAN_POINT ( 'NONE',  ( 130.8568914410475088, -52.36146031193419503, 4.207082182989537955 ) ) ;
#10733=CARTESIAN_POINT ( 'NONE',  ( 19.06497207195980792, 14.19242893257840876, 0.000000000000000000 ) ) ;
#10735=CARTESIAN_POINT ( 'NONE',  ( -3.993758944536592193, -47.00698038897011344, 13.83056263162088051 ) ) ;
#10736=CARTESIAN_POINT ( 'NONE',  ( -213.1075012329537230, 53.71589010951910836, 2.449293598294708485E-15 ) ) ;
#10738=CARTESIAN_POINT ( 'NONE',  ( 23.37394308801977871, -23.33966569535037294, -42.85717664514612579 ) ) ;
#10739=CARTESIAN_POINT ( 'NONE',  ( 57.59792236341147031, -1.722363176415032004, -1.722363176415048880 ) ) ;
#10740=CARTESIAN_POINT ( 'NONE',  ( -4.081455915266636758, -17.86600351372037565, 43.13234798823257421 ) ) ;
#10741=CARTESIAN_POINT ( 'NONE',  ( -5.379830816903563573, 13.73345071525145045, -46.52611083735715169 ) ) ;
#10743=CARTESIAN_POINT ( 'NONE',  ( 4.995406935893289102, 10.78321810389013002, -10.78321810388986712 ) ) ;
#10745=CARTESIAN_POINT ( 'NONE',  ( 170.0000000000000000, -30.00000000000001421, 3.673940397442065489E-15 ) ) ;
#10746=CARTESIAN_POINT ( 'NONE',  ( -188.2507053402891586, -23.43979243030692317, 42.99082124348444722 ) ) ;
#10747=CARTESIAN_POINT ( 'NONE',  ( 57.59792236341147031, 1.722363176415040886, 1.722363176415060426 ) ) ;
#10748=CARTESIAN_POINT ( 'NONE',  ( 130.8568914410475088, 24.07718906446891793, 32.49135343045489321 ) ) ;
#10749=CARTESIAN_POINT ( 'NONE',  ( -86.96347745069644475, -43.67073346367964604, -12.89780903124457545 ) ) ;
#10750=CARTESIAN_POINT ( 'NONE',  ( 130.8568914410475372, 24.07718906447210472, 24.07718906447249907 ) ) ;
#10751=CARTESIAN_POINT ( 'NONE',  ( -105.3755690713226727, 15.38646221621771737, 15.38646221621800514 ) ) ;
#10752=CARTESIAN_POINT ( 'NONE',  ( -259.2033419157646676, -6.730120644402966867, -49.83842185052038332 ) ) ;
#10753=CARTESIAN_POINT ( 'NONE',  ( 4.995406935893283773, 39.06748935135171052, 17.50105314357239195 ) ) ;
#10754=CARTESIAN_POINT ( 'NONE',  ( -56.48582580120558561, -30.84685318188645908, 40.00000000000002132 ) ) ;
#10755=CARTESIAN_POINT ( 'NONE',  ( -30.26275506840324070, 1.694272468446254232, 0.000000000000000000 ) ) ;
#10756=CARTESIAN_POINT ( 'NONE',  ( 57.59792236341147031, 54.84617931850881689, -1.722363176414946073 ) ) ;
#10758=CARTESIAN_POINT ( 'NONE',  ( -238.4067589809705794, -0.6820004457337348613, -57.25054294065803617 ) ) ;
#10759=CARTESIAN_POINT ( 'NONE',  ( -174.2681662549567818, 39.26785901271982482, -16.26527976844781520 ) ) ;
#10761=CARTESIAN_POINT ( 'NONE',  ( 151.7948205124836250, 4.785054706301690608, 4.785054706301682614 ) ) ;
#10762=CARTESIAN_POINT ( 'NONE',  ( -192.1167141818824291, -14.00295881688914790, -48.16218163818186326 ) ) ;
#10763=CARTESIAN_POINT ( 'NONE',  ( -280.0000000000000000, -14.14213562373108779, 14.14213562373088529 ) ) ;
#10764=CARTESIAN_POINT ( 'NONE',  ( 13.28449813601724827, -49.16593779331688552, -14.15462405555096304 ) ) ;
#10766=CARTESIAN_POINT ( 'NONE',  ( -86.86493150571114086, -19.77569912839162569, 7.943527260496431985 ) ) ;
#10767=CARTESIAN_POINT ( 'NONE',  ( -77.58456283179702950, -13.58505704039792050, -17.49511081174808069 ) ) ;
#10770=EDGE_CURVE ( 'NONE', #21913, #14253, #9940, .T. ) ;
#10771=CARTESIAN_POINT ( 'NONE',  ( 14.38125909742180752, 55.17850393972636880, 2.449293598294708485E-15 ) ) ;
#10774=CARTESIAN_POINT ( 'NONE',  ( -192.9588430854690273, -66.79921049721887982, -10.23066800229569040 ) ) ;
#10775=CARTESIAN_POINT ( 'NONE',  ( -213.1075012329537230, 39.99999999999979394, 53.71589010950180665 ) ) ;
#10776=CARTESIAN_POINT ( 'NONE',  ( -259.2033419157646676, -1.438356298054549103E-14, -9.517827891722632216 ) ) ;
#10777=( BOUNDED_SURFACE ( )  B_SPLINE_SURFACE ( 3, 2, ( 
 ( #15491, #11373, #20267 ),
 ( #2046, #14138, #23620 ),
 ( #5401, #17984, #22269 ),
 ( #13866, #3769, #3912 ),
 ( #5271, #4044, #19993 ),
 ( #15996, #13375, #8013 ) ),
 .UNSPECIFIED., .F., .F., .F. ) 
 B_SPLINE_SURFACE_WITH_KNOTS ( ( 4, 2, 4 ),
 ( 3, 3 ),
 ( 0.04143173980255905609, 0.04845742520045778767, 0.05548311059835652620 ),
 ( 0.000000000000000000, 1.000000000000000000 ),
 .UNSPECIFIED. ) 
 GEOMETRIC_REPRESENTATION_ITEM ( )  RATIONAL_B_SPLINE_SURFACE ( (
 ( 1.000000000000000000, 0.9541700779530454257, 1.000000000000000000),
 ( 1.000000000000000000, 0.9520119910812291364, 1.000000000000000000),
 ( 1.000000000000000000, 0.9503148373211529609, 1.000000000000000000),
 ( 1.000000000000000000, 0.9480088447022436693, 1.000000000000000000),
 ( 1.000000000000000000, 0.9474362535696445597, 1.000000000000000000),
 ( 1.000000000000000000, 0.9474350314971539122, 1.000000000000000000) ) ) 
 REPRESENTATION_ITEM ( '' )  SURFACE ( )  );
#10779=CARTESIAN_POINT ( 'NONE',  ( -56.48582580120557850, -30.84685318188645198, -2.449293598294708485E-15 ) ) ;
#10780=CARTESIAN_POINT ( 'NONE',  ( 22.66553228237846795, -17.89571368754641867, -43.20407469282425694 ) ) ;
#10781=CARTESIAN_POINT ( 'NONE',  ( 163.1118516004056573, 19.27778845538780317, -19.27778845538757224 ) ) ;
#10782=ADVANCED_FACE ( 'NONE', ( #13788 ), #15779, .T. ) ;
#10783=CARTESIAN_POINT ( 'NONE',  ( 130.8568914410475372, -5.949712681206667853, -2.449293598294708485E-15 ) ) ;
#10784=ADVANCED_FACE ( 'NONE', ( #26059 ), #17903, .T. ) ;
#10785=CARTESIAN_POINT ( 'NONE',  ( 0.2972598230770048811, -10.13633138497510089, 66.70487387989852834 ) ) ;
#10786=CARTESIAN_POINT ( 'NONE',  ( 137.0939645874030361, -12.56330697291244824, -30.33050608226196232 ) ) ;
#10787=CARTESIAN_POINT ( 'NONE',  ( -105.4741150117382205, 19.60045294982718644, -8.366608964594128395 ) ) ;
#10788=CARTESIAN_POINT ( 'NONE',  ( 200.0000000000000000, 40.00000000000026290, -19.99999999999950617 ) ) ;
#10789=CARTESIAN_POINT ( 'NONE',  ( 19.06497207195980792, 39.99999999999983658, 54.19242893257857929 ) ) ;
#10793=CARTESIAN_POINT ( 'NONE',  ( 170.2234770963711128, -39.20704971665379190, -17.36149277827012938 ) ) ;
#10795=CARTESIAN_POINT ( 'NONE',  ( -87.11162894489415010, 17.01505826596463322, -13.17695786912958589 ) ) ;
#10796=CARTESIAN_POINT ( 'NONE',  ( -188.7701102708081748, 23.55033952083685023, -43.14144101424751199 ) ) ;
#10798=CARTESIAN_POINT ( 'NONE',  ( -86.96347745069643054, -18.24025645688353947, -40.00000000000002132 ) ) ;
#10801=EDGE_LOOP ( 'NONE', ( #597, #17454, #25006, #2290 ) ) ;
#10804=SPHERICAL_SURFACE ( 'NONE', #12820, 15.00000000000000000 ) ;
#10805=CARTESIAN_POINT ( 'NONE',  ( 23.40652632867838179, 13.79856377312528082, 46.79646383233881579 ) ) ;
#10807=VERTEX_POINT ( 'NONE', #9014 ) ;
#10808=CARTESIAN_POINT ( 'NONE',  ( 19.06497207195980792, 10.03556273973433299, 10.03556273973436319 ) ) ;
#10810=CARTESIAN_POINT ( 'NONE',  ( -114.6297772183134782, -5.474609583110028765, 21.30737554389971677 ) ) ;
#10811=CARTESIAN_POINT ( 'NONE',  ( 146.6084372240433993, -24.48358557860319706, -24.48358557860330720 ) ) ;
#10812=CARTESIAN_POINT ( 'NONE',  ( -213.1075012329537230, 9.698598906450410340, 9.698598906450483170 ) ) ;
#10813=CARTESIAN_POINT ( 'NONE',  ( -56.48582580120560692, 40.00000000000004263, -9.153146818113443217 ) ) ;
#10815=CARTESIAN_POINT ( 'NONE',  ( -199.9999999999999147, 4.865628651907465851, 55.16984130227024252 ) ) ;
#10816=CARTESIAN_POINT ( 'NONE',  ( 130.8568914410475088, 40.00000000000011369, -5.949712681206269949 ) ) ;
#10817=CARTESIAN_POINT ( 'NONE',  ( 4.995406935893290878, 1.606505379428369110E-13, -15.24977328854832592 ) ) ;
#10818=CARTESIAN_POINT ( 'NONE',  ( -82.26772520252667675, 17.52690089560000430, 10.09596362476956877 ) ) ;
#10821=CARTESIAN_POINT ( 'NONE',  ( -188.4265004370316205, 13.83489460444899244, 47.03620155434649064 ) ) ;
#10822=CARTESIAN_POINT ( 'NONE',  ( -208.1127848780264742, -38.89260858015753541, 17.67593391476614784 ) ) ;
#10824=CARTESIAN_POINT ( 'NONE',  ( -100.7734535825088500, 16.03295912088683295, 40.53558337403684675 ) ) ;
#10825=CARTESIAN_POINT ( 'NONE',  ( -82.30220482034332008, -7.992411108785072216, 18.51665893431356480 ) ) ;
#10826=CARTESIAN_POINT ( 'NONE',  ( 151.7948205124835681, 51.78348778862544322, -4.785054706298002891 ) ) ;
#10828=DIRECTION ( 'NONE',  ( -0.01051738777841067576, 0.9166396752739927045, -0.3995761382614180235 ) ) ;
#10829=CARTESIAN_POINT ( 'NONE',  ( 0.2972598230769938343, 10.13633138497486286, -10.13633138497461594 ) ) ;
#10830=CARTESIAN_POINT ( 'NONE',  ( 151.7948205124836534, -6.767089262349006873, 40.00000000000002132 ) ) ;
#10832=ORIENTED_EDGE ( 'NONE', *, *, #22495, .F. ) ;
#10833=CARTESIAN_POINT ( 'NONE',  ( -105.3755690713226585, -39.99999999999985079, -18.24025645688394448 ) ) ;
#10835=CARTESIAN_POINT ( 'NONE',  ( 141.7948666911894975, -12.58737617328932323, 30.38861427224615852 ) ) ;
#10837=ORIENTED_EDGE ( 'NONE', *, *, #25724, .T. ) ;
#10839=CARTESIAN_POINT ( 'NONE',  ( -30.26275506840324425, 41.69427246844627177, 40.00000000000002132 ) ) ;
#10840=CARTESIAN_POINT ( 'NONE',  ( -103.9663809733125959, -19.92521373380484917, -8.574562932411120997 ) ) ;
#10841=CARTESIAN_POINT ( 'NONE',  ( -110.0791661673351598, -19.70411816747342826, -4.394837301270150043 ) ) ;
#10846=CARTESIAN_POINT ( 'NONE',  ( 130.8568914410475088, -52.36146031193413108, -4.207082182990267150 ) ) ;
#10847=CARTESIAN_POINT ( 'NONE',  ( 57.59792236341147031, 1.722363176415040886, 1.722363176415060426 ) ) ;
#10848=FACE_OUTER_BOUND ( 'NONE', #3389, .T. ) ;
#10849=CARTESIAN_POINT ( 'NONE',  ( -91.56559293963836410, 40.00000000000019185, -17.32597176626768487 ) ) ;
#10850=CARTESIAN_POINT ( 'NONE',  ( -135.8532207217289738, 6.472252184284096543, 6.472252184284234211 ) ) ;
#10851=CARTESIAN_POINT ( 'NONE',  ( 23.09931156284630305, 13.81622350327232240, 46.91113948292954205 ) ) ;
#10852=CARTESIAN_POINT ( 'NONE',  ( 151.7948205124836534, -23.49921654116027980, 33.06932595376354556 ) ) ;
#10853=CARTESIAN_POINT ( 'NONE',  ( -259.2033419157646676, 6.730120644403214669, 49.83842185052034068 ) ) ;
#10856=CARTESIAN_POINT ( 'NONE',  ( 184.8905102610680444, 40.00000000000013500, -20.92133201514430141 ) ) ;
#10857=CARTESIAN_POINT ( 'NONE',  ( -86.96347745069644475, -21.75974354311651737, 0.000000000000000000 ) ) ;
#10858=CARTESIAN_POINT ( 'NONE',  ( -192.9588430854690273, 10.23066800231970319, 66.79921049724369198 ) ) ;
#10859=CARTESIAN_POINT ( 'NONE',  ( 192.4448373802101173, -20.00000000003938538, 40.00000000000002132 ) ) ;
#10861=CARTESIAN_POINT ( 'NONE',  ( 15.76057515053193647, -44.53539632573529872, 18.44716516375831716 ) ) ;
#10862=AXIS2_PLACEMENT_3D ( 'NONE', #13473, #23714, #11466 ) ;
#10864=CARTESIAN_POINT ( 'NONE',  ( 199.9999999999999432, 19.99999999999996092, 2.449293598294708485E-15 ) ) ;
#10865=ADVANCED_FACE ( 'NONE', ( #15121 ), #10621, .T. ) ;
#10866=ORIENTED_EDGE ( 'NONE', *, *, #14445, .F. ) ;
#10868=B_SPLINE_CURVE_WITH_KNOTS ( 'NONE', 3,
 ( #12355, #5849, #23934, #14092, #24073, #17943, #20221, #13955 ),
 .UNSPECIFIED., .F., .F.,
 ( 4, 2, 2, 4 ),
 ( 0.008467075098540726916, 0.01051709959615203076, 0.01256712409376333460, 0.01666717308898594402 ),
 .UNSPECIFIED. ) ;
#10869=CARTESIAN_POINT ( 'NONE',  ( 19.06497207195980792, 10.03556273973433299, 10.03556273973436319 ) ) ;
#10870=CARTESIAN_POINT ( 'NONE',  ( -62.62756078637954005, -10.52198127419510598, 25.40230989532181383 ) ) ;
#10872=EDGE_CURVE ( 'NONE', #23760, #13429, #20197, .T. ) ;
#10873=CARTESIAN_POINT ( 'NONE',  ( 14.38125909742180752, 10.73282306404720465, 10.73282306404724018 ) ) ;
#10874=CARTESIAN_POINT ( 'NONE',  ( 5.009865950673480839, -14.14399394884917527, -49.09576456953148949 ) ) ;
#10876=CARTESIAN_POINT ( 'NONE',  ( 57.59792236341147031, -1.722363176415055985, 1.722363176415024677 ) ) ;
#10877=CARTESIAN_POINT ( 'NONE',  ( -82.23866954408245533, -20.16514221457112299, 1.261533135312056242 ) ) ;
#10878=CARTESIAN_POINT ( 'NONE',  ( 130.8568914410475372, -34.05028731879786363, 0.000000000000000000 ) ) ;
#10879=CARTESIAN_POINT ( 'NONE',  ( -194.4222169614009204, -14.07715596671739533, 48.65437996131331744 ) ) ;
#10880=CARTESIAN_POINT ( 'NONE',  ( 19.06497207195981147, -10.03556273973425483, -10.03556273973443247 ) ) ;
#10882=CARTESIAN_POINT ( 'NONE',  ( 200.0000000000000000, 42.42640687119290988, 14.14213562373111976 ) ) ;
#10883=CARTESIAN_POINT ( 'NONE',  ( -238.4067589809705794, 0.6820004457912851592, -0.6820004457913123597 ) ) ;
#10886=CIRCLE ( 'NONE', #4954, 15.00000000000000178 ) ;
#10887=CARTESIAN_POINT ( 'NONE',  ( -192.9588430854690273, 18.05360324515473280, -38.51493924976924177 ) ) ;
#10888=CARTESIAN_POINT ( 'NONE',  ( -259.2033419157646676, 21.55415060305860209, -21.55415060305812602 ) ) ;
#10889=CARTESIAN_POINT ( 'NONE',  ( -100.7734535825088358, 12.25131212657497848, -12.25131212657469604 ) ) ;
#10890=CARTESIAN_POINT ( 'NONE',  ( -208.1127848780265026, -15.00245453012673202, 0.000000000000000000 ) ) ;
#10891=CARTESIAN_POINT ( 'NONE',  ( 170.2234770963711128, 15.44714144992819627, -40.00000000000002132 ) ) ;
#10892=CARTESIAN_POINT ( 'NONE',  ( 151.7948205124836534, 33.06932595376365924, -23.49921654116018743 ) ) ;
#10894=CARTESIAN_POINT ( 'NONE',  ( -56.48582580120559982, -21.81201906317804173, 34.75652343174591152 ) ) ;
#10895=CARTESIAN_POINT ( 'NONE',  ( -187.8778500559049007, 43.02985669703468830, -17.82355023088518564 ) ) ;
#10896=EDGE_LOOP ( 'NONE', ( #12988, #22449, #23055, #3622 ) ) ;
#10898=CARTESIAN_POINT ( 'NONE',  ( -208.1127848780265026, 38.89260858015724409, 38.89260858015741462 ) ) ;
#10899=CARTESIAN_POINT ( 'NONE',  ( -65.65550967526378656, 24.89650881518296188, -9.107276986623963566 ) ) ;
#10900=CARTESIAN_POINT ( 'NONE',  ( -135.8532207217289738, 6.472252184283881604, 50.09629031063969506 ) ) ;
#10901=CARTESIAN_POINT ( 'NONE',  ( 17.91733029159629709, -48.44632265251725300, -14.04577174277931384 ) ) ;
#10902=ORIENTED_EDGE ( 'NONE', *, *, #9390, .F. ) ;
#10903=CARTESIAN_POINT ( 'NONE',  ( -185.5190358317587709, -42.39054933780622036, 17.55874045219087165 ) ) ;
#10904=CARTESIAN_POINT ( 'NONE',  ( -105.2054292635175585, -15.19799821370228621, -15.19799821370231818 ) ) ;
#10906=CARTESIAN_POINT ( 'NONE',  ( 18.90082769090739134, 14.00978943384327735, -48.20711988125814429 ) ) ;
#10907=CARTESIAN_POINT ( 'NONE',  ( -100.7734535825088500, 17.32597176626809699, -40.00000000000002132 ) ) ;
#10911=CARTESIAN_POINT ( 'NONE',  ( 170.2234770963711128, -10.92277846919235529, 45.64576402573175073 ) ) ;
#10912=CARTESIAN_POINT ( 'NONE',  ( -100.7734535825088500, -40.00000000000009948, 17.32597176626796909 ) ) ;
#10913=CARTESIAN_POINT ( 'NONE',  ( -192.9588430854690273, 39.99999999999992895, 14.46834944099983922 ) ) ;
#10915=CARTESIAN_POINT ( 'NONE',  ( 136.1360204305621551, -4.966164525587036138, -40.00000000000002132 ) ) ;
#10916=CARTESIAN_POINT ( 'NONE',  ( 22.76403192593580016, -17.88468650128144333, -43.17745271018603859 ) ) ;
#10917=CARTESIAN_POINT ( 'NONE',  ( 91.82158438592158234, 12.16597498397773869, -12.16597498397759303 ) ) ;
#10918=CARTESIAN_POINT ( 'NONE',  ( -208.1127848780264742, -55.00245453014425578, -40.00000000000002132 ) ) ;
#10919=CARTESIAN_POINT ( 'NONE',  ( -105.3755690713226727, 15.38646221621793231, -15.38646221621779020 ) ) ;
#10920=CARTESIAN_POINT ( 'NONE',  ( 144.1620285550791039, -12.51613133675853895, -30.21661402164560073 ) ) ;
#10921=CARTESIAN_POINT ( 'NONE',  ( -198.0356074513804572, -39.99999999999990052, -15.37879056873112482 ) ) ;
#10922=CARTESIAN_POINT ( 'NONE',  ( 91.82158438592158234, -12.16597498397761967, -12.16597498397768007 ) ) ;
#10923=CARTESIAN_POINT ( 'NONE',  ( 35.93765801217426059, -20.78447758813318202, 38.99300236454103441 ) ) ;
#10924=CARTESIAN_POINT ( 'NONE',  ( 98.29820294273281434, -7.653668647304240125, 18.47759065023114644 ) ) ;
#10925=B_SPLINE_CURVE_WITH_KNOTS ( 'NONE', 3,
 ( #3612, #3232, #19452, #25848, #23828, #11723 ),
 .UNSPECIFIED., .F., .F.,
 ( 4, 2, 4 ),
 ( -5.998621905802982250E-08, 0.03938016914544736902, 0.07876039827711379948 ),
 .UNSPECIFIED. ) ;
#10926=CARTESIAN_POINT ( 'NONE',  ( -280.0000000000000568, 14.14213562373067745, 42.42640687119295251 ) ) ;
#10928=CARTESIAN_POINT ( 'NONE',  ( -77.67292258764865664, -4.800060567486668539, -21.50168463689548659 ) ) ;
#10929=CARTESIAN_POINT ( 'NONE',  ( -7.233308327732243193, 42.27575367455148125, -17.51119053152626037 ) ) ;
#10931=CARTESIAN_POINT ( 'NONE',  ( 14.38125909742181285, -15.17850393972633505, -40.00000000000002132 ) ) ;
#10932=EDGE_CURVE ( 'NONE', #19642, #9531, #11604, .T. ) ;
#10933=CARTESIAN_POINT ( 'NONE',  ( -114.4944481313177675, 9.302331659127901275, -19.81806240209493808 ) ) ;
#10934=CARTESIAN_POINT ( 'NONE',  ( -188.6889827002346465, 43.11787295909656592, -23.53286111060870311 ) ) ;
#10936=EDGE_LOOP ( 'NONE', ( #13341, #10902, #25558, #4953, #20351, #14119 ) ) ;
#10938=CARTESIAN_POINT ( 'NONE',  ( -86.86493150571126876, 8.366608963954069722, -19.60045294882757005 ) ) ;
#10942=CARTESIAN_POINT ( 'NONE',  ( 130.8568914410475372, -24.07718906447222551, -24.07718906447233209 ) ) ;
#10945=EDGE_CURVE ( 'NONE', #17137, #23643, #368, .T. ) ;
#10946=CARTESIAN_POINT ( 'NONE',  ( 136.1360204305621266, -24.77266263493116583, -24.77266263493127951 ) ) ;
#10948=CARTESIAN_POINT ( 'NONE',  ( -162.0762913951020892, 1.198031840385716418, 1.198031840385750169 ) ) ;
#10949=CARTESIAN_POINT ( 'NONE',  ( 4.995406935893292655, 39.99999999999982947, 55.24977328856478209 ) ) ;
#10951=CARTESIAN_POINT ( 'NONE',  ( -199.9999999999999432, -2.318131689465268957E-13, 55.16984130226961724 ) ) ;
#10952=CARTESIAN_POINT ( 'NONE',  ( -213.1075012329537230, -39.99999999999948841, -53.71589010950208376 ) ) ;
#10953=CARTESIAN_POINT ( 'NONE',  ( 136.1360204305621551, 39.99999999999968026, 35.03383547441337953 ) ) ;
#10954=DIRECTION ( 'NONE',  ( 1.000000000000000000, 1.836970198721025990E-16, 0.000000000000000000 ) ) ;
#10957=CARTESIAN_POINT ( 'NONE',  ( -238.4067589809705794, -0.6820004457913680929, 0.6820004457913170226 ) ) ;
#10958=CARTESIAN_POINT ( 'NONE',  ( 199.9999999999999432, 14.14213562373093680, 14.14213562373114641 ) ) ;
#10960=CARTESIAN_POINT ( 'NONE',  ( 130.8568914410475372, -4.207082182992846420, 4.207082182992822439 ) ) ;
#10961=CARTESIAN_POINT ( 'NONE',  ( -77.70933353445910541, -18.93828009115086886, 11.19441472888376410 ) ) ;
#10962=CARTESIAN_POINT ( 'NONE',  ( -105.3755690713226585, 43.67073346367988051, -12.89780903124366418 ) ) ;
#10963=CARTESIAN_POINT ( 'NONE',  ( -200.0000000000000000, 45.36622447512545619, -20.93268228684340571 ) ) ;
#10964=CARTESIAN_POINT ( 'NONE',  ( -91.56559293963836410, 22.67402823373189946, -0.000000000000000000 ) ) ;
#10966=CARTESIAN_POINT ( 'NONE',  ( -100.7734535825088500, 40.53558337403654832, 16.03295912088756481 ) ) ;
#10967=CARTESIAN_POINT ( 'NONE',  ( 200.0000000000000000, -19.99999999999989342, 40.00000000000002132 ) ) ;
#10970=CARTESIAN_POINT ( 'NONE',  ( -198.0356074513804572, -39.99999999999990052, -15.37879056873112482 ) ) ;
#10972=CARTESIAN_POINT ( 'NONE',  ( 125.5832160019859600, -11.61997419108413609, 28.05309928653982965 ) ) ;
#10974=VERTEX_POINT ( 'NONE', #9914 ) ;
#10976=CARTESIAN_POINT ( 'NONE',  ( -198.0356074513804572, 55.37879056871320671, 40.00000000000002132 ) ) ;
#10977=ADVANCED_FACE ( 'NONE', ( #5528 ), #3308, .T. ) ;
#10980=CARTESIAN_POINT ( 'NONE',  ( -199.9999999999998010, 49.28189405767604114, -14.17215463606931358 ) ) ;
#10981=CARTESIAN_POINT ( 'NONE',  ( -105.3755690713226727, 5.661656051307470077E-14, -21.75974354311649961 ) ) ;
#10984=CARTESIAN_POINT ( 'NONE',  ( 170.2234770963711128, -17.36149277826940462, -39.20704971665412586 ) ) ;
#10985=CARTESIAN_POINT ( 'NONE',  ( 4.995406935893293543, -10.78321810388990265, -10.78321810389009272 ) ) ;
#10986=DIRECTION ( 'NONE',  ( 0.000000000000000000, 1.000000000000000000, 0.000000000000000000 ) ) ;
#10987=CARTESIAN_POINT ( 'NONE',  ( -192.9588430854689989, 5.375290060580374156E-13, -54.46834944099972375 ) ) ;
#10989=CARTESIAN_POINT ( 'NONE',  ( 19.06497207195981503, -14.19242893257840166, 0.000000000000000000 ) ) ;
#10990=CARTESIAN_POINT ( 'NONE',  ( 91.82158438592159655, -16.11829626346147393, 16.11829626346132116 ) ) ;
#10993=CARTESIAN_POINT ( 'NONE',  ( 4.995406935893290878, -5.232665749138292703E-14, 15.24977328854832592 ) ) ;
#10995=CARTESIAN_POINT ( 'NONE',  ( 14.38125909742181463, 10.73282306405862485, 67.30136555898259587 ) ) ;
#10996=CARTESIAN_POINT ( 'NONE',  ( -91.56559293963834989, 17.32597176626808988, 40.00000000000002132 ) ) ;
#10997=EDGE_LOOP ( 'NONE', ( #2868, #23768, #25564, #16342, #13854 ) ) ;
#10998=CARTESIAN_POINT ( 'NONE',  ( 16.10036699868849652, -48.79524671500755773, 14.09853761973996988 ) ) ;
#10999=CARTESIAN_POINT ( 'NONE',  ( -213.1075012329537230, 53.71589010950162191, -40.00000000000002132 ) ) ;
#11001=CARTESIAN_POINT ( 'NONE',  ( -259.2033419157646676, 21.55415060305830366, 21.55415060305842800 ) ) ;
#11002=CARTESIAN_POINT ( 'NONE',  ( 57.59792236341147031, 1.908507979671054758E-14, -2.435789363418160658 ) ) ;
#11003=CARTESIAN_POINT ( 'NONE',  ( -86.95085644346978881, 20.31668269185783871, -6.657466348996070593 ) ) ;
#11004=CARTESIAN_POINT ( 'NONE',  ( -39.58644176656166991, 13.59899295360881588, -32.83087322320439938 ) ) ;
#11006=CARTESIAN_POINT ( 'NONE',  ( -259.2033419157646676, 49.83842185052017015, 6.730120644404137487 ) ) ;
#11007=CARTESIAN_POINT ( 'NONE',  ( -77.55640685867214756, -22.13135000840951250, 0.6928334182904269944 ) ) ;
#11010=CARTESIAN_POINT ( 'NONE',  ( -198.9233928134752034, -14.16707757975546045, 49.24835219440009126 ) ) ;
#11011=CARTESIAN_POINT ( 'NONE',  ( 184.8905102610680444, -1.851754852062639767E-13, 20.92133201514444352 ) ) ;
#11012=CARTESIAN_POINT ( 'NONE',  ( 170.2234770963711128, 45.64576402573181468, 10.92277846919223627 ) ) ;
#11015=CARTESIAN_POINT ( 'NONE',  ( -198.0356074513804572, 17.40982414986501325, -39.15871834505897198 ) ) ;
#11016=CARTESIAN_POINT ( 'NONE',  ( -91.56559293963834989, 40.53558337403654832, 16.03295912088756481 ) ) ;
#11017=CARTESIAN_POINT ( 'NONE',  ( 136.1360204305621551, 31.79587985999232558, 24.77266263493161702 ) ) ;
#11018=CARTESIAN_POINT ( 'NONE',  ( 130.8568914410475088, 5.949712681206719367, -40.00000000000002132 ) ) ;
#11019=CARTESIAN_POINT ( 'NONE',  ( -208.1127848780264742, 38.89260858015732936, -17.67593391476642140 ) ) ;
#11021=CARTESIAN_POINT ( 'NONE',  ( 4.995406935893312195, -67.35176059882525124, -10.78321810390210445 ) ) ;
#11022=SPHERICAL_SURFACE ( 'NONE', #53, 15.00000000000000000 ) ;
#11024=CARTESIAN_POINT ( 'NONE',  ( -238.4067589809705794, 0.6820004457340470561, 57.25054294065803617 ) ) ;
#11026=CARTESIAN_POINT ( 'NONE',  ( -135.8532207217289738, 34.75652343174594705, 21.81201906317792449 ) ) ;
#11027=CARTESIAN_POINT ( 'NONE',  ( 98.29820294273291381, -18.47759065023123526, -7.653668647304108674 ) ) ;
#11029=CARTESIAN_POINT ( 'NONE',  ( -188.2870673237550818, -46.98612534495526205, 13.82722856953792068 ) ) ;
#11032=CARTESIAN_POINT ( 'NONE',  ( 190.0000000000000000, 7.164183775012018789E-14, 0.000000000000000000 ) ) ;
#11033=CARTESIAN_POINT ( 'NONE',  ( -280.0000000000000568, -20.00000000000006750, -40.00000000000002132 ) ) ;
#11036=CARTESIAN_POINT ( 'NONE',  ( -208.1127848780265026, -10.60833733269537227, -10.60833733269551793 ) ) ;
#11037=CARTESIAN_POINT ( 'NONE',  ( -162.0762913951020892, -1.777970010055771463E-13, 41.69427287682835015 ) ) ;
#11038=CARTESIAN_POINT ( 'NONE',  ( -30.26275506840324070, -1.147469862568086380E-14, 1.694272468446259783 ) ) ;
#11039=CARTESIAN_POINT ( 'NONE',  ( 0.4289713102705600689, 48.32239598606162900, -14.02712011273571946 ) ) ;
#11040=CARTESIAN_POINT ( 'NONE',  ( 14.38125909742182884, -55.17850393974264733, -40.00000000000002132 ) ) ;
#11041=CARTESIAN_POINT ( 'NONE',  ( 27.00968939605884245, -17.38581019152039531, -41.97305875718011237 ) ) ;
#11043=CARTESIAN_POINT ( 'NONE',  ( 130.8568914410475088, 34.05028731879790627, 40.00000000000002132 ) ) ;
#11044=CARTESIAN_POINT ( 'NONE',  ( -280.0000000000000000, 14.14213562373098299, -14.14213562373088706 ) ) ;
#11045=CARTESIAN_POINT ( 'NONE',  ( 4.995406935893283773, 40.00000000000017764, -15.24977328854790848 ) ) ;
#11046=CARTESIAN_POINT ( 'NONE',  ( -105.2276882639850015, 13.16704209471405029, -17.02247659825660975 ) ) ;
#11047=CARTESIAN_POINT ( 'NONE',  ( -56.48582580120558561, -40.00000000000012790, 9.153146818113166105 ) ) ;
#11048=CARTESIAN_POINT ( 'NONE',  ( -86.96347745069644475, -15.38646221621786125, -15.38646221621789856 ) ) ;
#11049=CARTESIAN_POINT ( 'NONE',  ( 153.3016677565462942, -28.42263824612669154, -11.77304223996991261 ) ) ;
#11051=CARTESIAN_POINT ( 'NONE',  ( -280.0000000000000568, 42.42640687119274645, 14.14213562373118194 ) ) ;
#11053=CARTESIAN_POINT ( 'NONE',  ( -87.13361725327074225, 16.16366093422423589, -14.23233549119255059 ) ) ;
#11054=CARTESIAN_POINT ( 'NONE',  ( -70.33906594826318326, 22.79894061131100003, -9.443630412774925986 ) ) ;
#11056=CARTESIAN_POINT ( 'NONE',  ( 0.2972598230769983307, -14.33493731733933352, 40.00000000000002132 ) ) ;
#11059=CARTESIAN_POINT ( 'NONE',  ( -190.7345856381643898, 47.78725959878585172, -13.94676320010617054 ) ) ;
#11063=CARTESIAN_POINT ( 'NONE',  ( 73.43468099484969969, -26.88834960806366681, -12.96803874020853797 ) ) ;
#11064=CARTESIAN_POINT ( 'NONE',  ( -199.9999999999998579, 44.86878812508723513, -24.82633483071237634 ) ) ;
#11068=CARTESIAN_POINT ( 'NONE',  ( -30.26275506840324070, 1.198031551615912571, 57.76657404653985139 ) ) ;
#11070=CARTESIAN_POINT ( 'NONE',  ( -91.56559293963836410, 40.00000000000008527, -22.67402823373177867 ) ) ;
#11071=CARTESIAN_POINT ( 'NONE',  ( -200.0000000000000568, -46.84854965773187985, 17.28402242884639151 ) ) ;
#11074=CARTESIAN_POINT ( 'NONE',  ( 14.38125909742182529, -39.99999999999944578, -55.17850393971050238 ) ) ;
#11075=CARTESIAN_POINT ( 'NONE',  ( 192.4448373802100889, 2.472897170449861688E-13, -19.99999999996060751 ) ) ;
#11076=CARTESIAN_POINT ( 'NONE',  ( -114.5514240060904001, -19.59008466214005750, 9.949107728608549195 ) ) ;
#11078=CARTESIAN_POINT ( 'NONE',  ( -30.26275506840324070, -1.147469862568086380E-14, 1.694272468446259783 ) ) ;
#11079=CARTESIAN_POINT ( 'NONE',  ( 151.7948205124836250, 23.49921654116361225, -23.49921654116333514 ) ) ;
#11080=CARTESIAN_POINT ( 'NONE',  ( -89.92902785008678279, 8.088236460649781634, 20.44110050034142745 ) ) ;
#11081=CARTESIAN_POINT ( 'NONE',  ( -99.29480781227293562, 8.934325994365014623, 20.48155342677144475 ) ) ;
#11082=FACE_BOUND ( 'NONE', #3490, .T. ) ;
#11083=CARTESIAN_POINT ( 'NONE',  ( 14.38125909742182529, -39.01709431150879936, -39.01709431150948859 ) ) ;
#11084=CARTESIAN_POINT ( 'NONE',  ( -129.2303573021169143, -9.309001178959640299, -25.82247248365550263 ) ) ;
#11085=CARTESIAN_POINT ( 'NONE',  ( -1.821043593238330205, 23.89737153267520142, 43.61003463695173821 ) ) ;
#11087=CARTESIAN_POINT ( 'NONE',  ( 57.59792236341147031, -1.722363176415055985, 1.722363176415024677 ) ) ;
#11088=CARTESIAN_POINT ( 'NONE',  ( 151.7948205124836250, 33.23291073765556547, 0.000000000000000000 ) ) ;
#11091=CARTESIAN_POINT ( 'NONE',  ( -135.8532207217289738, -40.00000000000014211, 9.153146818113153671 ) ) ;
#11095=EDGE_LOOP ( 'NONE', ( #3790, #4422, #4300, #20257 ) ) ;
#11097=CARTESIAN_POINT ( 'NONE',  ( -280.0000000000000568, 19.99999999999996447, -40.00000000000002132 ) ) ;
#11098=B_SPLINE_CURVE_WITH_KNOTS ( 'NONE', 3,
 ( #843, #8687, #13079, #2847, #19061, #16666 ),
 .UNSPECIFIED., .F., .F.,
 ( 4, 2, 4 ),
 ( 0.000000000000000000, 0.004089961189160419563, 0.008179922378320839127 ),
 .UNSPECIFIED. ) ;
#11100=CARTESIAN_POINT ( 'NONE',  ( -77.67292258764859980, -18.59814239105924827, 11.80983163630759414 ) ) ;
#11101=CARTESIAN_POINT ( 'NONE',  ( 184.8905102610680444, 1.070102760522089011E-13, -20.92133201514444352 ) ) ;
#11104=EDGE_CURVE ( 'NONE', #3577, #19812, #20778, .T. ) ;
#11106=CARTESIAN_POINT ( 'NONE',  ( -70.35386311798177417, -8.707385185642063874, -23.12931224674694164 ) ) ;
#11107=CARTESIAN_POINT ( 'NONE',  ( 91.82158438592158234, 12.16597498397756993, 12.16597498397776356 ) ) ;
#11108=FACE_OUTER_BOUND ( 'NONE', #9697, .T. ) ;
#11109=CARTESIAN_POINT ( 'NONE',  ( -259.2033419157646676, 2.741182173978444749E-13, -30.48217210827739621 ) ) ;
#11110=CARTESIAN_POINT ( 'NONE',  ( 91.82158438592158234, 12.16597498397756993, 12.16597498397776356 ) ) ;
#11111=CARTESIAN_POINT ( 'NONE',  ( 130.8568914410475088, 34.05028731879790627, -40.00000000000002132 ) ) ;
#11114=CARTESIAN_POINT ( 'NONE',  ( 0.2972598230770048811, -10.13633138497510089, 66.70487387989852834 ) ) ;
#11115=CARTESIAN_POINT ( 'NONE',  ( -280.0000000000000000, 19.99999999999996092, -0.000000000000000000 ) ) ;
#11117=CARTESIAN_POINT ( 'NONE',  ( -135.8532207217289738, 7.002209520526292428E-15, -9.153146818113572891 ) ) ;
#11119=CARTESIAN_POINT ( 'NONE',  ( 136.1360204305621266, -24.77266263493116583, -24.77266263493127951 ) ) ;
#11120=CARTESIAN_POINT ( 'NONE',  ( 57.59792236341147031, -2.435789363418150444, 0.000000000000000000 ) ) ;
#11121=B_SPLINE_CURVE_WITH_KNOTS ( 'NONE', 3,
 ( #19177, #5322, #9066, #25306, #15301, #23305, #13187, #3084, #1082, #5846 ),
 .UNSPECIFIED., .F., .F.,
 ( 4, 2, 2, 2, 4 ),
 ( 0.7921542097163948304, 0.8508620842112317728, 0.8814014469398914198, 0.9119408096685510667, 0.9406682828395580565 ),
 .UNSPECIFIED. ) ;
#11123=CARTESIAN_POINT ( 'NONE',  ( 21.80824205439684249, -43.30754100652733740, 23.67346680103123191 ) ) ;
#11125=CARTESIAN_POINT ( 'NONE',  ( 57.59792236341147031, -2.435789363418150000, -40.00000000000002132 ) ) ;
#11126=CARTESIAN_POINT ( 'NONE',  ( -105.2110227778628939, 16.13864963247413442, -14.20565731138971088 ) ) ;
#11127=CARTESIAN_POINT ( 'NONE',  ( -259.2033419157646676, -6.730120644403667640, 49.83842185052029805 ) ) ;
#11128=CARTESIAN_POINT ( 'NONE',  ( 146.6084372240433993, 1.478241399363601114E-13, -34.62501878078305850 ) ) ;
#11129=CARTESIAN_POINT ( 'NONE',  ( -87.00601149411200197, 20.66743745453288739, 5.745309048958548992 ) ) ;
#11132=CARTESIAN_POINT ( 'NONE',  ( -213.1075012329537230, 9.698598906450543566, -9.698598906450348167 ) ) ;
#11133=CARTESIAN_POINT ( 'NONE',  ( -82.23729782345287731, -1.277530580954402861, -20.19443213282674776 ) ) ;
#11134=CARTESIAN_POINT ( 'NONE',  ( -213.1075012329537230, 9.698598906450543566, -9.698598906450348167 ) ) ;
#11136=CARTESIAN_POINT ( 'NONE',  ( -213.1075012329537230, 18.58567234101121102, 37.98287015391247223 ) ) ;
#11137=CARTESIAN_POINT ( 'NONE',  ( 91.82158438592158234, -12.16597498397778843, 12.16597498397750954 ) ) ;
#11138=CARTESIAN_POINT ( 'NONE',  ( -280.0000000000000000, 14.14213562373078581, 14.14213562373108424 ) ) ;
#11140=CARTESIAN_POINT ( 'NONE',  ( 163.1118516004056573, 19.27778845538753316, 19.27778845538783870 ) ) ;
#11141=CARTESIAN_POINT ( 'NONE',  ( 136.1360204305621551, 31.79587985999232558, 24.77266263493161702 ) ) ;
#11142=CARTESIAN_POINT ( 'NONE',  ( -192.9588430854689989, 38.51493924976983152, -38.51493924976893624 ) ) ;
#11143=CARTESIAN_POINT ( 'NONE',  ( -56.48582580120559982, 30.84685318188643777, -40.00000000000002132 ) ) ;
#11144=CARTESIAN_POINT ( 'NONE',  ( 170.2234770963711128, 10.92277846919210660, -45.64576402573182889 ) ) ;
#11146=CARTESIAN_POINT ( 'NONE',  ( -56.48582580120558561, -50.09629031063971638, 6.472252184283745713 ) ) ;
#11149=CARTESIAN_POINT ( 'NONE',  ( 91.82158438592158234, 16.11829626346139577, 16.11829626346143840 ) ) ;
#11150=CARTESIAN_POINT ( 'NONE',  ( 170.0000000000001421, 9.369682556672135121, 22.62041470344889760 ) ) ;
#11151=CARTESIAN_POINT ( 'NONE',  ( -47.45115950045780551, -29.80449331803366775, -14.84795788642767356 ) ) ;
#11153=CARTESIAN_POINT ( 'NONE',  ( -121.8281105901183849, -23.07023229738023673, 8.694016233238142988 ) ) ;
#11155=CARTESIAN_POINT ( 'NONE',  ( 23.36927571439207796, -23.34061495561071808, 42.85861222363632805 ) ) ;
#11156=CARTESIAN_POINT ( 'NONE',  ( 98.29820294267314296, 18.47759065023127079, 7.653668647304075812 ) ) ;
#11158=CARTESIAN_POINT ( 'NONE',  ( -100.7734535825088500, -12.25131212657524316, 44.31723036834888774 ) ) ;
#11159=CARTESIAN_POINT ( 'NONE',  ( -213.1075012329537230, -8.703598725189323045E-14, 13.71589010951911902 ) ) ;
#11160=CARTESIAN_POINT ( 'NONE',  ( 190.0000000000001137, 30.00000000000007461, 0.000000000000000000 ) ) ;
#11161=CARTESIAN_POINT ( 'NONE',  ( 136.1360204305621266, 35.03383547441298163, -40.00000000000002132 ) ) ;
#11162=CARTESIAN_POINT ( 'NONE',  ( 23.37583784646148644, -13.80085822090975434, -46.80752016581924835 ) ) ;
#11164=CARTESIAN_POINT ( 'NONE',  ( 200.0000000000000000, 20.00000000000013856, 40.00000000000002132 ) ) ;
#11165=CARTESIAN_POINT ( 'NONE',  ( 19.06497207195980792, 18.24870850772737185, 38.31983398719634692 ) ) ;
#11166=CARTESIAN_POINT ( 'NONE',  ( 184.8905102610680444, 39.99999999999983658, 20.92133201514485563 ) ) ;
#11168=CARTESIAN_POINT ( 'NONE',  ( -105.3755690713226585, -39.99999999999985079, -18.24025645688394448 ) ) ;
#11170=CARTESIAN_POINT ( 'NONE',  ( 133.2072010122031713, -29.90326689760170709, -12.38633870824907568 ) ) ;
#11172=CARTESIAN_POINT ( 'NONE',  ( -213.1075012329537230, -9.698598906438496314, 66.26714140136188291 ) ) ;
#11174=CARTESIAN_POINT ( 'NONE',  ( -77.55672185583993894, -1.410533997352584334, -22.12963403628582171 ) ) ;
#11175=CARTESIAN_POINT ( 'NONE',  ( 8.273828130719147467, 44.87796109790431842, -18.58906013839431282 ) ) ;
#11176=CARTESIAN_POINT ( 'NONE',  ( -162.0762913951021176, -1.694272876828353702, 40.00000000000002132 ) ) ;
#11177=CARTESIAN_POINT ( 'NONE',  ( -138.9613198120158302, -29.42718893709543337, 10.11110880661598443 ) ) ;
#11182=CARTESIAN_POINT ( 'NONE',  ( -97.72675010090424053, -20.56394680065914926, 8.987772175319408419 ) ) ;
#11183=CARTESIAN_POINT ( 'NONE',  ( -93.02511667906942705, 8.169918093965671702, -20.82219708225684940 ) ) ;
#11184=VERTEX_POINT ( 'NONE', #16435 ) ;
#11188=CARTESIAN_POINT ( 'NONE',  ( 170.2234770963711128, -17.36149277826985937, -17.36149277826995174 ) ) ;
#11189=DIRECTION ( 'NONE',  ( 1.000000000000000000, 0.000000000000000000, 0.000000000000000000 ) ) ;
#11190=CARTESIAN_POINT ( 'NONE',  ( 163.1118516004056573, 40.00000000000014921, -27.26290988616858968 ) ) ;
#11191=CARTESIAN_POINT ( 'NONE',  ( 17.76569288431004878, -14.04863394049465519, 48.46476365406687137 ) ) ;
#11195=CARTESIAN_POINT ( 'NONE',  ( -162.0762913951021176, -40.00000000000003553, -1.694272876828743168 ) ) ;
#11196=CARTESIAN_POINT ( 'NONE',  ( 151.7948205124836534, 40.00000000000012079, -6.767089262348609857 ) ) ;
#11198=CARTESIAN_POINT ( 'NONE',  ( -56.48582580120559271, 6.472252184284211118, -6.472252184284153387 ) ) ;
#11200=CARTESIAN_POINT ( 'NONE',  ( -198.0356074513804572, -10.87444709759729911, 10.87444709759714812 ) ) ;
#11202=EDGE_CURVE ( 'NONE', #17668, #8569, #2521, .T. ) ;
#11205=CARTESIAN_POINT ( 'NONE',  ( -77.59243545049976376, -13.54949188064048116, 17.47199274922497381 ) ) ;
#11206=CARTESIAN_POINT ( 'NONE',  ( 184.8905102610680444, -41.77492675556007384, 14.79361573936348684 ) ) ;
#11207=CARTESIAN_POINT ( 'NONE',  ( -151.7004448983857117, -13.46262099565286796, -32.50164219297025170 ) ) ;
#11208=CARTESIAN_POINT ( 'NONE',  ( 7.340276910564533352, 24.82763627182876931, 44.87059041559387396 ) ) ;
#11209=EDGE_LOOP ( 'NONE', ( #8255, #20603, #7101, #26084, #23341, #6798, #10275, #19776, #3652, #14485 ) ) ;
#11210=CARTESIAN_POINT ( 'NONE',  ( -86.96347745069644475, -15.38646221621738164, -41.18208027870615240 ) ) ;
#11215=CARTESIAN_POINT ( 'NONE',  ( -91.56559293963834989, -2.543181659092656077E-13, 22.67402823373191723 ) ) ;
#11217=CARTESIAN_POINT ( 'NONE',  ( 14.32711916788068152, -44.71189734681519923, 24.71075626504589096 ) ) ;
#11219=VERTEX_POINT ( 'NONE', #6580 ) ;
#11220=CARTESIAN_POINT ( 'NONE',  ( 57.59792236341147031, 37.56421063658187620, 2.449293598294708485E-15 ) ) ;
#11221=UNCERTAINTY_MEASURE_WITH_UNIT (LENGTH_MEASURE( 1.000000000000000082E-05 ), #25985, 'distance_accuracy_value', 'NONE');
#11222=CARTESIAN_POINT ( 'NONE',  ( -91.56559293963836410, 16.03295912088714203, -16.03295912088699282 ) ) ;
#11223=CARTESIAN_POINT ( 'NONE',  ( 184.8905102610680444, 39.99999999999999289, 19.07866798485573057 ) ) ;
#11224=CARTESIAN_POINT ( 'NONE',  ( -77.70896657118075268, -18.93513500903290137, 11.20032855622331702 ) ) ;
#11225=CARTESIAN_POINT ( 'NONE',  ( -238.4067589809705794, -40.00000000000007105, 0.9644942799824426372 ) ) ;
#11227=DIRECTION ( 'NONE',  ( 0.9698969544100555229, 0.09318942523065473771, -0.2249791742612613499 ) ) ;
#11228=CARTESIAN_POINT ( 'NONE',  ( -8.197988474444986906, -17.40147972965361589, -42.01088836873536536 ) ) ;
#11229=CARTESIAN_POINT ( 'NONE',  ( 136.1360204305621266, 24.77266263493104148, 24.77266263493145004 ) ) ;
#11230=CARTESIAN_POINT ( 'NONE',  ( -105.2272256531326207, -17.01582848540546777, -13.17790690984702984 ) ) ;
#11231=CARTESIAN_POINT ( 'NONE',  ( 184.8905102610680444, -39.99999999999978684, -19.07866798485600768 ) ) ;
#11233=CARTESIAN_POINT ( 'NONE',  ( 136.1360204305621551, -4.966164525587036138, -40.00000000000002132 ) ) ;
#11234=CARTESIAN_POINT ( 'NONE',  ( 170.2234770963711128, -39.20704971665379190, -17.36149277827012938 ) ) ;
#11235=CARTESIAN_POINT ( 'NONE',  ( -56.48582580120559982, 9.153146818113574668, -40.00000000000002132 ) ) ;
#11236=CARTESIAN_POINT ( 'NONE',  ( 23.30631261066300297, -42.87793822514719011, -23.35506702544013180 ) ) ;
#11237=CARTESIAN_POINT ( 'NONE',  ( -105.3755690713226727, 5.661656051307470077E-14, -21.75974354311649961 ) ) ;
#11238=CARTESIAN_POINT ( 'NONE',  ( 170.0000000000000000, 1.183443619805854272E-13, -24.95097643317000546 ) ) ;
#11239=CARTESIAN_POINT ( 'NONE',  ( -198.0356074513804572, 67.44298959253333692, 10.87444709760969452 ) ) ;
#11240=CARTESIAN_POINT ( 'NONE',  ( -192.9588430854689989, 54.46834944099968823, 2.449293598294708485E-15 ) ) ;
#11241=ORIENTED_EDGE ( 'NONE', *, *, #20205, .T. ) ;
#11242=EDGE_CURVE ( 'NONE', #10069, #1078, #21222, .T. ) ;
#11243=CARTESIAN_POINT ( 'NONE',  ( -3.417371742523301670, -43.31092608455668369, 17.93997298316205047 ) ) ;
#11244=DIRECTION ( 'NONE',  ( -1.850371707708594760E-15, 0.9166903767334100284, -0.3995982397413169185 ) ) ;
#11245=EDGE_CURVE ( 'NONE', #18786, #12394, #2446, .T. ) ;
#11246=CARTESIAN_POINT ( 'NONE',  ( 163.1118516004056573, -19.27778845539233998, 37.29075403953149959 ) ) ;
#11247=CARTESIAN_POINT ( 'NONE',  ( -105.3755690713226727, 5.661656051307470077E-14, -21.75974354311649961 ) ) ;
#11248=CARTESIAN_POINT ( 'NONE',  ( -87.06808288329423817, 21.06763942722659877, 4.035072084556908578 ) ) ;
#11250=CARTESIAN_POINT ( 'NONE',  ( -4.039451493210483690, -13.82811171175408127, -46.99046209229819482 ) ) ;
#11254=CARTESIAN_POINT ( 'NONE',  ( 0.2972598230769938343, 10.13633138497486286, -10.13633138497461594 ) ) ;
#11255=CARTESIAN_POINT ( 'NONE',  ( -30.26275506840323359, -1.198031551615522439, -57.76657404653986561 ) ) ;
#11257=CARTESIAN_POINT ( 'NONE',  ( -86.96347745069645896, 43.67073346367970288, 12.89780903124427702 ) ) ;
#11259=CARTESIAN_POINT ( 'NONE',  ( -208.1127848780264742, -38.89260858015704514, -38.89260858015768463 ) ) ;
#11260=CARTESIAN_POINT ( 'NONE',  ( -135.8532207217289738, 6.472252184284583265, -50.09629031063960980 ) ) ;
#11261=CARTESIAN_POINT ( 'NONE',  ( -100.7734535825088500, -44.31723036834885932, -12.25131212657538171 ) ) ;
#11262=CARTESIAN_POINT ( 'NONE',  ( 192.4448373802100889, 14.14213562370330379, -14.14213562370292365 ) ) ;
#11263=CARTESIAN_POINT ( 'NONE',  ( 57.59792236341147031, -2.435789363418150000, -40.00000000000002132 ) ) ;
#11264=CARTESIAN_POINT ( 'NONE',  ( 151.7948205124836250, -23.49921654116339553, -23.49921654116350211 ) ) ;
#11267=CARTESIAN_POINT ( 'NONE',  ( 199.9999999999999432, -14.14213562373073607, -14.14213562373102206 ) ) ;
#11269=CARTESIAN_POINT ( 'NONE',  ( -188.2956751479547393, 43.00407324591997593, -23.44846780264088437 ) ) ;
#11271=CARTESIAN_POINT ( 'NONE',  ( -105.3755690713226585, 41.18208027870598187, -15.38646221621779731 ) ) ;
#11273=CARTESIAN_POINT ( 'NONE',  ( 16.10036699856384956, 14.09853761972935615, 48.79524671503644129 ) ) ;
#11274=CARTESIAN_POINT ( 'NONE',  ( -87.02142894580126153, -20.76642173392621515, 5.408203463872810701 ) ) ;
#11276=CARTESIAN_POINT ( 'NONE',  ( -105.2349941599195802, 17.04272630156315316, 13.08094329434171144 ) ) ;
#11279=CARTESIAN_POINT ( 'NONE',  ( 22.50777602749776207, -17.91321921095823910, 43.24633676486227785 ) ) ;
#11281=CARTESIAN_POINT ( 'NONE',  ( 27.79909650596783877, 22.43832426418754267, -41.49206490659992141 ) ) ;
#11285=CARTESIAN_POINT ( 'NONE',  ( 19.06497207195979726, 39.99999999999997158, 14.19242893257854554 ) ) ;
#11286=CARTESIAN_POINT ( 'NONE',  ( 163.1118516004056573, 1.251511021549353291E-13, -27.26290988616872824 ) ) ;
#11287=CARTESIAN_POINT ( 'NONE',  ( -199.9999999999999716, -16.05666331275163117, -47.66874763508944568 ) ) ;
#11288=CARTESIAN_POINT ( 'NONE',  ( -105.3755690713226585, -18.24025645688353947, -40.00000000000002132 ) ) ;
#11289=CARTESIAN_POINT ( 'NONE',  ( 20.69615274310995190, -23.88537831998747052, -43.59383154590273790 ) ) ;
#11290=FACE_OUTER_BOUND ( 'NONE', #6333, .T. ) ;
#11291=CARTESIAN_POINT ( 'NONE',  ( -91.56559293963834989, -17.32597176626812896, 40.00000000000002132 ) ) ;
#11293=CARTESIAN_POINT ( 'NONE',  ( -213.1075012329537230, -13.71589010951915810, 0.000000000000000000 ) ) ;
#11295=CARTESIAN_POINT ( 'NONE',  ( 163.1118516004056573, 39.99999999999976552, 27.26290988616914746 ) ) ;
#11296=CARTESIAN_POINT ( 'NONE',  ( 4.995406935893297984, -39.99999999999986500, -15.24977328854874870 ) ) ;
#11298=CARTESIAN_POINT ( 'NONE',  ( 127.8226996004795950, -28.75922372236458813, -11.91246050912548071 ) ) ;
#11299=EDGE_LOOP ( 'NONE', ( #22745, #23294, #14784, #9282 ) ) ;
#11301=CARTESIAN_POINT ( 'NONE',  ( -4.004886986945064287, 43.01537795656800256, -23.45685150724343870 ) ) ;
#11302=CARTESIAN_POINT ( 'NONE',  ( -280.0000000000000568, -20.00000000000007105, 40.00000000000002132 ) ) ;
#11303=CARTESIAN_POINT ( 'NONE',  ( -199.0731274799843504, 44.83667511838923048, -18.57195892570682361 ) ) ;
#11306=CARTESIAN_POINT ( 'NONE',  ( -99.29480781227283614, -20.48155342677143409, 8.934325994365179824 ) ) ;
#11307=CARTESIAN_POINT ( 'NONE',  ( 90.71511022951216319, -21.46756116403335568, -8.335579107441619229 ) ) ;
#11308=EDGE_LOOP ( 'NONE', ( #1372, #18952, #15075, #19174 ) ) ;
#11309=ORIENTED_EDGE ( 'NONE', *, *, #7502, .F. ) ;
#11310=( BOUNDED_CURVE ( )  B_SPLINE_CURVE ( 3, ( #25893, #23743, #17243, #5152 ),
 .UNSPECIFIED., .F., .F. ) 
 B_SPLINE_CURVE_WITH_KNOTS ( ( 4, 4 ),
 ( 0.01388163287021919670, 0.02359082919309990825 ),
 .UNSPECIFIED. ) 
 CURVE ( )  GEOMETRIC_REPRESENTATION_ITEM ( )  RATIONAL_B_SPLINE_CURVE ( ( 1.000000000000000000, 0.8672072324489000783, 0.7608653435686208999, 0.6809743333591623538 ) ) 
 REPRESENTATION_ITEM ( '' )  );
#11312=CARTESIAN_POINT ( 'NONE',  ( -109.1264249741452232, 13.72187187126506558, -33.12752917268247188 ) ) ;
#11314=CARTESIAN_POINT ( 'NONE',  ( 184.8905102610680444, 13.49065550809807945, 13.49065550809809544 ) ) ;
#11316=CARTESIAN_POINT ( 'NONE',  ( 4.995406935893290878, -5.232665749138292703E-14, 15.24977328854832592 ) ) ;
#11317=CARTESIAN_POINT ( 'NONE',  ( -200.0000000000000284, -45.36622447512538514, 20.93268228684354426 ) ) ;
#11318=FACE_OUTER_BOUND ( 'NONE', #15939, .T. ) ;
#11319=CARTESIAN_POINT ( 'NONE',  ( -105.3755690713226585, -40.00000000000027711, 21.75974354311608749 ) ) ;
#11320=CARTESIAN_POINT ( 'NONE',  ( 0.2972598230770030492, 5.716321584140269555E-13, -54.33493731733936016 ) ) ;
#11321=CARTESIAN_POINT ( 'NONE',  ( -105.3178975793387337, -18.51275824393216496, 10.85284064411901817 ) ) ;
#11322=CARTESIAN_POINT ( 'NONE',  ( 184.8905102610680444, -13.49065550809780412, -43.07788698682583828 ) ) ;
#11323=CARTESIAN_POINT ( 'NONE',  ( 170.2234770963711128, 1.169953928977015745E-13, -24.55285855007187124 ) ) ;
#11325=CARTESIAN_POINT ( 'NONE',  ( 127.8236149080040889, 28.75948073575744601, 11.91256696755863054 ) ) ;
#11326=CARTESIAN_POINT ( 'NONE',  ( 98.29820294271928560, -10.07205412907102549, -17.47586258463233477 ) ) ;
#11327=CARTESIAN_POINT ( 'NONE',  ( -56.48582580120559271, 6.472252184284211118, -6.472252184284153387 ) ) ;
#11328=CARTESIAN_POINT ( 'NONE',  ( -77.55658273871470954, -16.64052652070192195, 14.65657382809084552 ) ) ;
#11329=CARTESIAN_POINT ( 'NONE',  ( -56.48582580120559982, -34.75652343174615311, 21.81201906317766870 ) ) ;
#11330=CARTESIAN_POINT ( 'NONE',  ( -86.96347745069645896, -12.89780903124443689, 43.67073346367968156 ) ) ;
#11334=CARTESIAN_POINT ( 'NONE',  ( -162.0762913951020892, 29.48230308784799902, -29.48230308784730980 ) ) ;
#11339=CARTESIAN_POINT ( 'NONE',  ( -208.1127848780265026, 1.189126717069624012E-13, -15.00245453012669472 ) ) ;
#11341=CARTESIAN_POINT ( 'NONE',  ( 0.4289717129526404160, -44.08776571100848685, 24.25042218720266618 ) ) ;
#11343=ORIENTED_EDGE ( 'NONE', *, *, #8923, .T. ) ;
#11344=CARTESIAN_POINT ( 'NONE',  ( -200.4318156386405576, -49.29858106685330910, -14.17468120671522236 ) ) ;
#11345=CARTESIAN_POINT ( 'NONE',  ( -198.0356074513804572, 39.99999999999979394, 55.37879056874835726 ) ) ;
#11347=ADVANCED_FACE ( 'NONE', ( #9241 ), #2462, .T. ) ;
#11352=CARTESIAN_POINT ( 'NONE',  ( -70.35386311679275195, -10.19784240597756941, -22.51194465199612438 ) ) ;
#11353=CARTESIAN_POINT ( 'NONE',  ( -208.1127848780264742, 17.67593391476678377, -38.89260858015718014 ) ) ;
#11354=CARTESIAN_POINT ( 'NONE',  ( -77.61444910505873906, -21.81614215778263244, 3.470426107494282597 ) ) ;
#11355=CARTESIAN_POINT ( 'NONE',  ( -280.0000000000000568, -39.99999999999987210, -20.00000000000043343 ) ) ;
#11356=CARTESIAN_POINT ( 'NONE',  ( 48.46159092537987334, -37.63079858261907873, -11.89574569450916286 ) ) ;
#11357=CARTESIAN_POINT ( 'NONE',  ( -162.0762913951020892, -1.694272876828353702, 0.000000000000000000 ) ) ;
#11358=CARTESIAN_POINT ( 'NONE',  ( 151.7948205124835681, 33.23291073765556547, -40.00000000000002132 ) ) ;
#11359=CARTESIAN_POINT ( 'NONE',  ( 192.4448373802101173, 42.42640687122070631, 14.14213562370331623 ) ) ;
#11360=CARTESIAN_POINT ( 'NONE',  ( -208.1127848780264742, -15.00245453012673202, -40.00000000000002132 ) ) ;
#11361=CARTESIAN_POINT ( 'NONE',  ( -4.039451493210478361, -43.00522595893993838, -23.44932283416681429 ) ) ;
#11363=CARTESIAN_POINT ( 'NONE',  ( -280.0000000000000000, -2.609240458947769655E-13, 20.00000000000001421 ) ) ;
#11364=CARTESIAN_POINT ( 'NONE',  ( 146.6084372240433709, 32.08495691632064961, -24.48358557860320417 ) ) ;
#11365=CARTESIAN_POINT ( 'NONE',  ( -91.56559293963834989, 17.32597176626809343, 2.449293598294708485E-15 ) ) ;
#11367=CARTESIAN_POINT ( 'NONE',  ( 22.75856136761861492, -43.17893233522182328, 17.88529938203894787 ) ) ;
#11368=CARTESIAN_POINT ( 'NONE',  ( -86.95488169845611992, -9.644899311047964829, 19.11867441905828002 ) ) ;
#11369=CARTESIAN_POINT ( 'NONE',  ( -105.3755690713226727, 12.89780903124400879, 12.89780903124407452 ) ) ;
#11370=CARTESIAN_POINT ( 'NONE',  ( -86.83718372825752851, 19.60232422073417879, 8.316105076740864632 ) ) ;
#11371=CARTESIAN_POINT ( 'NONE',  ( -5.296937277117006460, 17.72975434250563254, -42.80341339123120292 ) ) ;
#11373=CARTESIAN_POINT ( 'NONE',  ( -82.30220482034327745, -18.74474319042430892, -7.441767004318710299 ) ) ;
#11374=CARTESIAN_POINT ( 'NONE',  ( -77.90255099906775627, -8.064892378658402805, -20.29001641120661148 ) ) ;
#11375=CARTESIAN_POINT ( 'NONE',  ( 91.82158438592158234, -12.16597498397778843, 12.16597498397750954 ) ) ;
#11376=CARTESIAN_POINT ( 'NONE',  ( 192.4448373802101173, 42.42640687122089815, -14.14213562370272470 ) ) ;
#11377=CARTESIAN_POINT ( 'NONE',  ( -114.6419057268807791, 21.37096723866840975, -5.444467006605387738 ) ) ;
#11379=CARTESIAN_POINT ( 'NONE',  ( -238.4067589809705794, -0.6820004457337348613, -57.25054294065803617 ) ) ;
#11380=CARTESIAN_POINT ( 'NONE',  ( 14.38125909742181996, -10.73282306405815234, -67.30136555898266693 ) ) ;
#11381=CARTESIAN_POINT ( 'NONE',  ( 14.38125909742181463, 10.73282306403652875, -67.30136555895941797 ) ) ;
#11382=CARTESIAN_POINT ( 'NONE',  ( 14.38125909742180397, 67.30136555898270956, -10.73282306405792319 ) ) ;
#11383=CARTESIAN_POINT ( 'NONE',  ( 0.2972598230769930572, 14.33493731733933352, 0.000000000000000000 ) ) ;
#11385=CARTESIAN_POINT ( 'NONE',  ( 19.06497207195981147, -4.605042221739098431E-14, 14.19242893257840521 ) ) ;
#11386=CARTESIAN_POINT ( 'NONE',  ( 163.1118516004056573, -37.29075403953166301, 19.27778845539196695 ) ) ;
#11387=CARTESIAN_POINT ( 'NONE',  ( -192.9588430854690273, 14.46834944099966336, 40.00000000000002132 ) ) ;
#11389=CARTESIAN_POINT ( 'NONE',  ( -100.7734535825088500, 40.53558337403677569, -16.03295912088699993 ) ) ;
#11390=CARTESIAN_POINT ( 'NONE',  ( -89.92902785008715227, -20.44110050034142745, -8.088236460650017889 ) ) ;
#11391=CARTESIAN_POINT ( 'NONE',  ( -28.75808802591297209, -12.03522322449749637, -38.33175228464058648 ) ) ;
#11392=CARTESIAN_POINT ( 'NONE',  ( -4.660840668352969729, -46.77528141313101173, -13.78427145221207262 ) ) ;
#11394=CARTESIAN_POINT ( 'NONE',  ( -188.2956751479547108, -43.00407324591987646, 23.44846780264116859 ) ) ;
#11396=CARTESIAN_POINT ( 'NONE',  ( 98.29820294267315717, -7.653668647304115780, 18.47759065023121039 ) ) ;
#11398=CARTESIAN_POINT ( 'NONE',  ( 170.0000000000000000, -12.70659020859111088, 21.59613885783081955 ) ) ;
#11400=( BOUNDED_SURFACE ( )  B_SPLINE_SURFACE ( 3, 2, ( 
 ( #13803, #5448, #16071 ),
 ( #26347, #5698, #15799 ),
 ( #21938, #1719, #18195 ),
 ( #24200, #11816, #24062 ),
 ( #19935, #10092, #11678 ),
 ( #19670, #5972, #8088 ),
 ( #7555, #20208, #16208 ),
 ( #11953, #19803, #7685 ),
 ( #20078, #15667, #13549 ),
 ( #1856, #23923, #23793 ),
 ( #1590, #9959, #21678 ),
 ( #22212, #21802, #14081 ) ),
 .UNSPECIFIED., .F., .F., .F. ) 
 B_SPLINE_SURFACE_WITH_KNOTS ( ( 4, 2, 2, 2, 2, 4 ),
 ( 3, 3 ),
 ( 0.006022589392325213183, 0.01254516766564344951, 0.01580645680230256811, 0.01906774593896168671, 0.02559032421227992043, 0.03211290248559815763 ),
 ( 0.000000000000000000, 1.000000000000000000 ),
 .UNSPECIFIED. ) 
 GEOMETRIC_REPRESENTATION_ITEM ( )  RATIONAL_B_SPLINE_SURFACE ( (
 ( 1.000000000000000000, 0.9998834880171258988, 1.000000000000000000),
 ( 1.000000000000000000, 0.9998139205012247510, 1.000000000000000000),
 ( 1.000000000000000000, 0.9997315632444677691, 1.000000000000000000),
 ( 1.000000000000000000, 0.9996405464946958030, 1.000000000000000000),
 ( 1.000000000000000000, 0.9996155081776925133, 1.000000000000000000),
 ( 1.000000000000000000, 0.9995814087511105672, 1.000000000000000000),
 ( 1.000000000000000000, 0.9995724100939918921, 1.000000000000000000),
 ( 1.000000000000000000, 0.9995726760936894939, 1.000000000000000000),
 ( 1.000000000000000000, 0.9996103361816741639, 1.000000000000000000),
 ( 1.000000000000000000, 0.9997312749796802844, 1.000000000000000000),
 ( 1.000000000000000000, 0.9998135910914284219, 1.000000000000000000),
 ( 1.000000000000000000, 0.9998834880173383954, 1.000000000000000000) ) ) 
 REPRESENTATION_ITEM ( '' )  SURFACE ( )  );
#11402=CARTESIAN_POINT ( 'NONE',  ( 200.0000000000000000, 39.99999999999999289, 20.00000000000007105 ) ) ;
#11403=CARTESIAN_POINT ( 'NONE',  ( 170.2234770963711128, 1.169953928977015745E-13, -24.55285855007187124 ) ) ;
#11405=CARTESIAN_POINT ( 'NONE',  ( 12.01676479903289874, 49.30523874212545365, -14.17570730777195998 ) ) ;
#11406=CARTESIAN_POINT ( 'NONE',  ( -30.26275506840323004, -41.69427246844629309, 40.00000000000002132 ) ) ;
#11407=CARTESIAN_POINT ( 'NONE',  ( -151.4802930568858415, 11.09498731357607504, -33.96623840857670729 ) ) ;
#11409=EDGE_CURVE ( 'NONE', #12267, #6802, #6576, .T. ) ;
#11410=CARTESIAN_POINT ( 'NONE',  ( 130.8568914410475088, -5.949712681206671405, 40.00000000000002132 ) ) ;
#11411=CARTESIAN_POINT ( 'NONE',  ( -208.1127848780265026, -10.60833733269551971, 10.60833733269537049 ) ) ;
#11412=CARTESIAN_POINT ( 'NONE',  ( 57.59792236341147031, -2.435789363418150444, 0.000000000000000000 ) ) ;
#11413=CARTESIAN_POINT ( 'NONE',  ( -198.0356074513804572, 40.00000000000014921, -15.37879056873028816 ) ) ;
#11414=CARTESIAN_POINT ( 'NONE',  ( 57.59792236341148453, -40.00000000000003553, 2.435789363417741438 ) ) ;
#11415=CARTESIAN_POINT ( 'NONE',  ( -16.41594856550787895, -39.35878123526666172, 21.03672846785433137 ) ) ;
#11416=ADVANCED_FACE ( 'NONE', ( #10848 ), #4740, .T. ) ;
#11417=ADVANCED_FACE ( 'NONE', ( #11108 ), #22960, .T. ) ;
#11420=CARTESIAN_POINT ( 'NONE',  ( -3.675706741948014500, 43.24173023805430205, -17.91131112508040601 ) ) ;
#11421=CARTESIAN_POINT ( 'NONE',  ( -259.2033419157646676, -30.48217210827744950, 40.00000000000002132 ) ) ;
#11422=CARTESIAN_POINT ( 'NONE',  ( -114.6379801953803650, 5.502459769868860207, -21.35001481053563666 ) ) ;
#11432=CARTESIAN_POINT ( 'NONE',  ( -126.6834156230595454, 11.16464796290217087, -24.04426801068344588 ) ) ;
#11433=CARTESIAN_POINT ( 'NONE',  ( 136.1360204305621551, 31.79587985999267374, -24.77266263493117293 ) ) ;
#11434=CARTESIAN_POINT ( 'NONE',  ( -121.8281150758585341, -22.46071699780029363, -10.16552079116060803 ) ) ;
#11435=CARTESIAN_POINT ( 'NONE',  ( -30.26275506840324070, -1.147469862568086380E-14, 1.694272468446259783 ) ) ;
#11436=CARTESIAN_POINT ( 'NONE',  ( -105.3174402647060361, -10.86264740497938242, -18.50711184654230479 ) ) ;
#11439=CARTESIAN_POINT ( 'NONE',  ( -105.3755690713226585, -39.99999999999985079, -18.24025645688394448 ) ) ;
#11440=CARTESIAN_POINT ( 'NONE',  ( 163.1118516004056573, 40.00000000000017764, -12.73709011382432976 ) ) ;
#11441=CARTESIAN_POINT ( 'NONE',  ( -110.0822598093819522, -11.09289860105409353, 16.86905266169973316 ) ) ;
#11442=CARTESIAN_POINT ( 'NONE',  ( -162.0762913951020892, -1.198031840385783919, 1.198031840385741731 ) ) ;
#11443=CARTESIAN_POINT ( 'NONE',  ( 146.6084372240433709, 40.00000000000017053, -34.62501878078291639 ) ) ;
#11444=CARTESIAN_POINT ( 'NONE',  ( 199.9999999999999432, 14.14213562373113398, -14.14213562373094923 ) ) ;
#11446=CARTESIAN_POINT ( 'NONE',  ( -77.90255099906853786, 8.644468104252323926, -20.04994828524279882 ) ) ;
#11447=CARTESIAN_POINT ( 'NONE',  ( -280.0000000000000000, 14.14213562373098299, -14.14213562373088706 ) ) ;
#11448=CARTESIAN_POINT ( 'NONE',  ( -259.2033419157646676, -1.438356298054549103E-14, -9.517827891722632216 ) ) ;
#11449=CARTESIAN_POINT ( 'NONE',  ( -280.0000000000000568, -14.14213562373108601, 42.42640687119285303 ) ) ;
#11450=CARTESIAN_POINT ( 'NONE',  ( -135.8532207217289738, -50.09629031063973770, 6.472252184283735943 ) ) ;
#11451=CARTESIAN_POINT ( 'NONE',  ( -144.1957134277073465, -12.48102206811670811, -30.13185274890651399 ) ) ;
#11453=VERTEX_POINT ( 'NONE', #9490 ) ;
#11454=CARTESIAN_POINT ( 'NONE',  ( 151.7948205124836250, 4.785054706301759886, -4.785054706301612448 ) ) ;
#11459=CARTESIAN_POINT ( 'NONE',  ( 192.4448373802100889, -1.741373372144848397E-13, 20.00000000003942091 ) ) ;
#11461=CARTESIAN_POINT ( 'NONE',  ( -62.72988123315806064, 10.50767649796025616, 25.36777511002372876 ) ) ;
#11463=EDGE_LOOP ( 'NONE', ( #2512, #683, #18170, #10535, #5319, #9836 ) ) ;
#11464=CARTESIAN_POINT ( 'NONE',  ( 0.2972598230769976091, -10.13633138497479180, 10.13633138497468522 ) ) ;
#11465=CARTESIAN_POINT ( 'NONE',  ( 91.82158438592156813, 39.99999999999995737, 22.79471317813484887 ) ) ;
#11466=DIRECTION ( 'NONE',  ( 0.000000000000000000, -0.9307566067258455922, 0.3656393565197673112 ) ) ;
#11467=CIRCLE ( 'NONE', #9354, 14.99999999999999822 ) ;
#11468=CARTESIAN_POINT ( 'NONE',  ( -200.0000000000001421, -14.17215463606902404, -49.28189405767602693 ) ) ;
#11469=CARTESIAN_POINT ( 'NONE',  ( -280.0000000000000000, -1.237140859393462838E-13, 20.00000000000001421 ) ) ;
#11471=CARTESIAN_POINT ( 'NONE',  ( 91.82158438592158234, 7.693928927950222250E-14, -17.20528682183300262 ) ) ;
#11473=CARTESIAN_POINT ( 'NONE',  ( -5.787027468458424195, -17.67457596682273291, -42.67020100828553808 ) ) ;
#11474=CARTESIAN_POINT ( 'NONE',  ( 184.8905102610680444, 43.07788698682591644, -13.49065550809769221 ) ) ;
#11475=CARTESIAN_POINT ( 'NONE',  ( -77.90255099906769942, -20.29001641120661859, 8.064892378658379712 ) ) ;
#11476=CARTESIAN_POINT ( 'NONE',  ( -135.8532207217289738, -39.99999999999972289, -30.84685318188688541 ) ) ;
#11477=CARTESIAN_POINT ( 'NONE',  ( 85.88525995977231275, -23.37195345543618430, -8.769880559910854245 ) ) ;
#11478=CARTESIAN_POINT ( 'NONE',  ( 184.8905102610680444, -19.07866798485554938, 40.00000000000002132 ) ) ;
#11479=CARTESIAN_POINT ( 'NONE',  ( -208.1127848780264742, -55.00245453014425578, -40.00000000000002132 ) ) ;
#11480=CARTESIAN_POINT ( 'NONE',  ( -198.0356074513804572, 17.40982414986446969, 39.15871834505921356 ) ) ;
#11481=CARTESIAN_POINT ( 'NONE',  ( 14.38125909742181285, -15.17850393972633505, -40.00000000000002132 ) ) ;
#11482=CARTESIAN_POINT ( 'NONE',  ( -1.815588850254795217, -43.60036197523984924, -23.89016120430183676 ) ) ;
#11483=CARTESIAN_POINT ( 'NONE',  ( -83.21262154144233136, 13.72187187059966895, -33.12752917119015450 ) ) ;
#11484=CARTESIAN_POINT ( 'NONE',  ( -192.9588430854689989, 1.161019517985663313E-13, -14.46834944099969533 ) ) ;
#11485=CARTESIAN_POINT ( 'NONE',  ( 184.8905102610680444, -14.79361573936389540, 41.77492675555996016 ) ) ;
#11486=CARTESIAN_POINT ( 'NONE',  ( -280.0000000000000568, 19.99999999999996447, -40.00000000000002132 ) ) ;
#11487=ORIENTED_EDGE ( 'NONE', *, *, #1162, .F. ) ;
#11488=CARTESIAN_POINT ( 'NONE',  ( 23.42154907652887630, -46.79103593565392316, 13.79745687233760876 ) ) ;
#11489=SPHERICAL_SURFACE ( 'NONE', #22332, 15.00000000000000000 ) ;
#11490=CARTESIAN_POINT ( 'NONE',  ( -105.3755690713226585, -15.38646221621796251, 41.18208027870593924 ) ) ;
#11491=CARTESIAN_POINT ( 'NONE',  ( 0.2972598230769957217, -4.999556039334937811E-14, 14.33493731733933352 ) ) ;
#11493=FACE_OUTER_BOUND ( 'NONE', #19677, .T. ) ;
#11494=B_SPLINE_CURVE_WITH_KNOTS ( 'NONE', 3,
 ( #21307, #5082, #17172, #11063, #7065, #13431 ),
 .UNSPECIFIED., .F., .F.,
 ( 4, 2, 4 ),
 ( -6.000000002287634284E-08, 0.04017169446089188106, 0.08034344892178377218 ),
 .UNSPECIFIED. ) ;
#11495=CARTESIAN_POINT ( 'NONE',  ( 91.82158438592158234, 22.79471317813472453, -40.00000000000002132 ) ) ;
#11498=CARTESIAN_POINT ( 'NONE',  ( -114.4098922876147384, 20.15198150140922451, 8.347224046571190215 ) ) ;
#11501=EDGE_CURVE ( 'NONE', #9531, #1858, #20543, .T. ) ;
#11502=CARTESIAN_POINT ( 'NONE',  ( -77.90255099906772784, 8.064892378658852223, -20.29001641120641608 ) ) ;
#11503=CARTESIAN_POINT ( 'NONE',  ( 170.0000000000000000, -24.95097643316997704, 0.000000000000000000 ) ) ;
#11504=CARTESIAN_POINT ( 'NONE',  ( -192.9588430854690273, -10.23066800231931239, -66.79921049724377724 ) ) ;
#11505=CARTESIAN_POINT ( 'NONE',  ( -105.2050109279299761, 21.49594509020261413, -0.1304588126430248907 ) ) ;
#11506=CARTESIAN_POINT ( 'NONE',  ( -77.78761611110736851, 9.949180589398501695, -19.59005896965153326 ) ) ;
#11507=CARTESIAN_POINT ( 'NONE',  ( 0.2972598230770048811, -10.13633138497415942, -66.70487387989865624 ) ) ;
#11508=CARTESIAN_POINT ( 'NONE',  ( -198.0356074513804572, -10.87444709758429262, -67.44298959250878056 ) ) ;
#11509=CARTESIAN_POINT ( 'NONE',  ( -198.0356074513804572, 10.87444709759730088, -10.87444709759707173 ) ) ;
#11510=CARTESIAN_POINT ( 'NONE',  ( -162.0762913951020892, 1.198031840385732849, -1.198031840385733515 ) ) ;
#11511=CARTESIAN_POINT ( 'NONE',  ( -105.2940237833718982, -11.46076537570947451, 18.12284447398040754 ) ) ;
#11513=CARTESIAN_POINT ( 'NONE',  ( -100.7734535825088500, -40.00000000000009948, 17.32597176626796909 ) ) ;
#11514=CARTESIAN_POINT ( 'NONE',  ( -56.48582580120559271, 6.472252184284121412, 6.472252184284244869 ) ) ;
#11515=CIRCLE ( 'NONE', #12838, 15.00000000000000000 ) ;
#11516=CARTESIAN_POINT ( 'NONE',  ( 151.7948205124836534, -33.23291073765550863, 40.00000000000002132 ) ) ;
#11518=CARTESIAN_POINT ( 'NONE',  ( 184.8905102610680444, 13.49065550809817715, -43.07788698682574591 ) ) ;
#11519=CARTESIAN_POINT ( 'NONE',  ( -19.45810057983592500, 38.38097177479090760, 15.89791904617739249 ) ) ;
#11520=CARTESIAN_POINT ( 'NONE',  ( 83.06440094989142153, 9.006081069517801296, 24.44702070087263834 ) ) ;
#11521=CARTESIAN_POINT ( 'NONE',  ( -4.121597284766468583, -46.96202426942434727, -13.82232031191962562 ) ) ;
#11522=VERTEX_POINT ( 'NONE', #23985 ) ;
#11523=CARTESIAN_POINT ( 'NONE',  ( -197.4154352060510575, -44.73190714601606288, 24.72550168626919742 ) ) ;
#11525=CARTESIAN_POINT ( 'NONE',  ( 23.25494099740784293, -17.82744980609922791, 43.03927110441377124 ) ) ;
#11526=CARTESIAN_POINT ( 'NONE',  ( 98.29820294269173075, 19.99999999998819433, -2.308575297063409524E-13 ) ) ;
#11528=CONICAL_SURFACE ( 'NONE', #20061, 60.00000000000000000, 0.7853981633974447263 ) ;
#11529=CARTESIAN_POINT ( 'NONE',  ( -87.08627934007971305, 21.18514689813062191, 3.496387290698740102 ) ) ;
#11530=CARTESIAN_POINT ( 'NONE',  ( 91.82158438592156813, 39.99999999999995737, 22.79471317813484887 ) ) ;
#11531=CARTESIAN_POINT ( 'NONE',  ( -87.13361725325452767, -1.359581015579222063, 21.49321519332998065 ) ) ;
#11532=CARTESIAN_POINT ( 'NONE',  ( 1.564252679174713778, 48.56509332159259884, -14.06374044400957501 ) ) ;
#11533=CARTESIAN_POINT ( 'NONE',  ( 130.8568914410475088, 34.05028731879790627, 40.00000000000002132 ) ) ;
#11536=CARTESIAN_POINT ( 'NONE',  ( -162.0762913951020892, -1.694272876828353702, 0.000000000000000000 ) ) ;
#11537=CARTESIAN_POINT ( 'NONE',  ( 163.1118516004056573, 27.26290988616876021, -40.00000000000002132 ) ) ;
#11538=CARTESIAN_POINT ( 'NONE',  ( -86.96347745069644475, -21.75974354311651737, 0.000000000000000000 ) ) ;
#11539=CARTESIAN_POINT ( 'NONE',  ( -280.0000000000000568, 40.00000000000017764, -19.99999999999959144 ) ) ;
#11540=CARTESIAN_POINT ( 'NONE',  ( -56.48582580120559271, -1.062504017861011783E-13, 9.153146818113587102 ) ) ;
#11541=CARTESIAN_POINT ( 'NONE',  ( 113.0017353590611293, -23.76250624610700513, -9.842752363112978742 ) ) ;
#11543=CARTESIAN_POINT ( 'NONE',  ( -4.039451493210481026, -46.99046209229813797, 13.82811171175447917 ) ) ;
#11544=CARTESIAN_POINT ( 'NONE',  ( -3.449394506061540966, 43.30266483527620380, -17.93655106166781366 ) ) ;
#11545=CARTESIAN_POINT ( 'NONE',  ( 170.2234770963711128, -15.44714144992812876, -2.449293598294708485E-15 ) ) ;
#11546=CARTESIAN_POINT ( 'NONE',  ( -114.4364955367328491, -20.29001642038857156, 8.064892380842218600 ) ) ;
#11554=ORIENTED_EDGE ( 'NONE', *, *, #18389, .F. ) ;
#11555=EDGE_CURVE ( 'NONE', #13654, #8031, #9740, .T. ) ;
#11559=CARTESIAN_POINT ( 'NONE',  ( -30.26275506840325136, 57.76657404653985139, 1.198031551616126178 ) ) ;
#11562=CARTESIAN_POINT ( 'NONE',  ( 14.38125909742181108, -5.035366881890652543E-14, 15.17850393972633682 ) ) ;
#11563=CARTESIAN_POINT ( 'NONE',  ( 12.01361943528961262, -14.17591515420103754, 49.30661675909298935 ) ) ;
#11565=EDGE_CURVE ( 'NONE', #11184, #23643, #5249, .T. ) ;
#11568=CARTESIAN_POINT ( 'NONE',  ( 4.995406935893290878, 1.606505379428369110E-13, -15.24977328854832592 ) ) ;
#11569=CARTESIAN_POINT ( 'NONE',  ( -280.0000000000000568, -39.99999999999987210, -20.00000000000043343 ) ) ;
#11570=CARTESIAN_POINT ( 'NONE',  ( -114.6659165474107311, -11.80608088190434302, 18.60032035379251170 ) ) ;
#11571=CARTESIAN_POINT ( 'NONE',  ( 146.6084372240433709, -3.800685668858344801, -52.76785682606520567 ) ) ;
#11572=CARTESIAN_POINT ( 'NONE',  ( -280.0000000000000000, 1.839446121267387017E-14, -20.00000000000001421 ) ) ;
#11573=CARTESIAN_POINT ( 'NONE',  ( 14.38125909742181818, -39.01709431150904095, -17.55144818341490165 ) ) ;
#11574=CARTESIAN_POINT ( 'NONE',  ( 144.1620285550791323, 30.21661402164551191, 12.51613133675876810 ) ) ;
#11575=CARTESIAN_POINT ( 'NONE',  ( -4.039451493210481026, -46.99046209229813797, 13.82811171175447917 ) ) ;
#11576=CARTESIAN_POINT ( 'NONE',  ( -208.1127848780265026, -10.60833733269551971, 10.60833733269537049 ) ) ;
#11577=CARTESIAN_POINT ( 'NONE',  ( -86.96347745069643054, -39.99999999999995737, -21.75974354311664527 ) ) ;
#11578=CARTESIAN_POINT ( 'NONE',  ( -280.0000000000000000, 14.14213562373088351, 14.14213562373098654 ) ) ;
#11579=CARTESIAN_POINT ( 'NONE',  ( 130.8568914410475372, -4.207082182992785135, -4.207082182992884611 ) ) ;
#11580=CARTESIAN_POINT ( 'NONE',  ( -166.3490736461069446, -19.13702016934220040, -36.43932733823757530 ) ) ;
#11581=CARTESIAN_POINT ( 'NONE',  ( -77.58504658027047185, 13.57343625279989219, 17.50303174137573592 ) ) ;
#11583=CARTESIAN_POINT ( 'NONE',  ( 151.7948205124836534, 33.06932595376333239, 23.49921654116065284 ) ) ;
#11584=CARTESIAN_POINT ( 'NONE',  ( 184.8905102610680444, 20.92133201514447549, 0.000000000000000000 ) ) ;
#11586=CARTESIAN_POINT ( 'NONE',  ( -102.2610585947572872, 22.27377874548541925, -0.000000000000000000 ) ) ;
#11587=VERTEX_POINT ( 'NONE', #17595 ) ;
#11588=CARTESIAN_POINT ( 'NONE',  ( -213.1075012329537230, 1.045191102001431893E-13, -13.71589010951911902 ) ) ;
#11590=CARTESIAN_POINT ( 'NONE',  ( 18.89824403360313099, -43.99464769172834622, 24.18164459663369925 ) ) ;
#11591=EDGE_LOOP ( 'NONE', ( #21044, #9089, #4623, #2731 ) ) ;
#11595=CARTESIAN_POINT ( 'NONE',  ( 136.1360204305621551, 4.966164525587093870, -40.00000000000002132 ) ) ;
#11596=CARTESIAN_POINT ( 'NONE',  ( -213.1075012329537230, -37.98287015391232302, -18.58567234101164800 ) ) ;
#11597=CARTESIAN_POINT ( 'NONE',  ( 200.0000000000000000, 39.99999999999999289, 20.00000000000007105 ) ) ;
#11600=CARTESIAN_POINT ( 'NONE',  ( 0.2972598230769957217, 1.502051041545559470E-13, -14.33493731733933352 ) ) ;
#11601=CARTESIAN_POINT ( 'NONE',  ( -105.3755690713226727, -8.549198663894545631E-14, 18.24025645688352881 ) ) ;
#11603=CARTESIAN_POINT ( 'NONE',  ( -238.4067589809705794, -4.716212492215116094E-14, 0.9644942799825824142 ) ) ;
#11604=B_SPLINE_CURVE_WITH_KNOTS ( 'NONE', 3,
 ( #9650, #1283, #17621, #7771, #3533, #15752 ),
 .UNSPECIFIED., .F., .F.,
 ( 4, 2, 4 ),
 ( 0.0003134778200527471104, 0.004479062015275551457, 0.008644646210498357214 ),
 .UNSPECIFIED. ) ;
#11606=CARTESIAN_POINT ( 'NONE',  ( -7.769366557094651959, -13.56374645826313063, -45.69637362128903391 ) ) ;
#11607=CARTESIAN_POINT ( 'NONE',  ( -100.7734535825088500, 44.31723036834907958, -12.25131212657445801 ) ) ;
#11608=( BOUNDED_SURFACE ( )  B_SPLINE_SURFACE ( 3, 3, ( 
 ( #7982, #11448, #26247, #11982, #21702, #20106, #3479, #3603, #25840, #11712, #13575, #3741, #1883, #5730, #19697, #17568, #9987, #19832, #3348, #13972, #9725, #17827, #1618, #25974, #23820, #26106, #18098, #9461, #13455, #7714 ),
 ( #15825, #22106, #25705, #19571, #3882, #23955, #16100, #7456, #24232, #9590, #21574, #13834, #11577, #15571, #11846, #21969, #19967, #1748, #9856, #1485, #1362, #23695, #17959, #7844, #5602, #15966, #5475, #13709, #24091, #5866 ),
 ( #17695, #7584, #15696, #21834, #14504, #10657, #8250, #16636, #8518, #24368, #275, #16367, #8654, #20372, #10123, #12644, #4016, #24765, #24630, #22766, #24501, #22508, #18366, #6518, #12116, #18631, #14113, #146, #6131, #14375 ),
 ( #16762, #6262, #4286, #6388, #22241, #22635, #14629, #12250, #12375, #18224, #18766, #6005, #8383, #20240, #10384, #16505, #4546, #20769, #12504, #2147, #4410, #11, #20503, #10257, #8122, #2275, #18495, #14239, #550, #2021 ),
 ( #20632, #2539, #16239, #2407, #22379, #4155, #10517, #414, #4675, #6651, #14766, #22896, #24896, #12777, #2682, #18899, #20904, #678, #10789, #8787, #19598, #4008, #25730, #21599, #14367, #9486, #24493, #16230, #2011, #6254 ),
 ( #8114, #24359, #6123, #22498, #25864, #4277, #10376, #12107, #13477, #1385, #137, #14231, #10249, #8376, #3370, #5499, #8241, #5997, #14103, #18487, #3505, #13599, #24223, #22232, #23718, #20232, #15723, #19727, #22371, #1514 ),
 ( #16359, #17590, #11603, #10116, #268, #2, #21729, #18216, #4147, #20364, #12240, #2138, #18358, #12367, #20495, #9619, #2268, #17723, #23594, #5372, #11471, #7480, #15593, #7608, #4537, #20624, #16498, #804, #19149, #2531 ) ),
 .UNSPECIFIED., .T., .F., .F. ) 
 B_SPLINE_SURFACE_WITH_KNOTS ( ( 4, 3, 4 ),
 ( 4, 2, 2, 2, 2, 2, 2, 2, 2, 2, 2, 2, 2, 2, 4 ),
 ( 0.000000000000000000, 0.5000000000000000000, 1.000000000000000000 ),
 ( 0.000000000000000000, 0.1357259735107005372, 0.1651108541090157700, 0.1944957347073310028, 0.3598804999793158710, 0.3867117631979620773, 0.4135430264166082281, 0.5789277916885930964, 0.6062785021374117456, 0.6336292125862302838, 0.8508620842112317728, 0.8814014469398914198, 0.9119408096685510667, 0.9559704048342755334, 1.000000000000000000 ),
 .UNSPECIFIED. ) 
 GEOMETRIC_REPRESENTATION_ITEM ( )  RATIONAL_B_SPLINE_SURFACE ( (
 ( 1.000000000000000000, 1.000000000000000000, 1.000000000000000000, 1.000000000000000000, 1.000000000000000000, 1.000000000000000000, 1.000000000000000000, 1.000000000000000000, 1.000000000000000000, 1.000000000000000000, 1.000000000000000000, 1.000000000000000000, 1.000000000000000000, 1.000000000000000000, 1.000000000000000000, 1.000000000000000000, 1.000000000000000000, 1.000000000000000000, 1.000000000000000000, 1.000000000000000000, 1.000000000000000000, 1.000000000000000000, 1.000000000000000000, 1.000000000000000000, 1.000000000000000000, 1.000000000000000000, 1.000000000000000000, 1.000000000000000000, 1.000000000000000000, 1.000000000000000000),
 ( 0.3333333333333333703, 0.3333333333333333703, 0.3333333333333333703, 0.3333333333333333703, 0.3333333333333333703, 0.3333333333333333703, 0.3333333333333333703, 0.3333333333333333703, 0.3333333333333333703, 0.3333333333333333703, 0.3333333333333333703, 0.3333333333333333703, 0.3333333333333333703, 0.3333333333333333703, 0.3333333333333333703, 0.3333333333333333703, 0.3333333333333333703, 0.3333333333333333703, 0.3333333333333333703, 0.3333333333333333703, 0.3333333333333333703, 0.3333333333333333703, 0.3333333333333333703, 0.3333333333333333703, 0.3333333333333333703, 0.3333333333333333703, 0.3333333333333333703, 0.3333333333333333703, 0.3333333333333333703, 0.3333333333333333703),
 ( 0.3333333333333333703, 0.3333333333333333703, 0.3333333333333333703, 0.3333333333333333703, 0.3333333333333333703, 0.3333333333333333703, 0.3333333333333333703, 0.3333333333333333703, 0.3333333333333333703, 0.3333333333333333703, 0.3333333333333333703, 0.3333333333333333703, 0.3333333333333333703, 0.3333333333333333703, 0.3333333333333333703, 0.3333333333333333703, 0.3333333333333333703, 0.3333333333333333703, 0.3333333333333333703, 0.3333333333333333703, 0.3333333333333333703, 0.3333333333333333703, 0.3333333333333333703, 0.3333333333333333703, 0.3333333333333333703, 0.3333333333333333703, 0.3333333333333333703, 0.3333333333333333703, 0.3333333333333333703, 0.3333333333333333703),
 ( 1.000000000000000000, 1.000000000000000000, 1.000000000000000000, 1.000000000000000000, 1.000000000000000000, 1.000000000000000000, 1.000000000000000000, 1.000000000000000000, 1.000000000000000000, 1.000000000000000000, 1.000000000000000000, 1.000000000000000000, 1.000000000000000000, 1.000000000000000000, 1.000000000000000000, 1.000000000000000000, 1.000000000000000000, 1.000000000000000000, 1.000000000000000000, 1.000000000000000000, 1.000000000000000000, 1.000000000000000000, 1.000000000000000000, 1.000000000000000000, 1.000000000000000000, 1.000000000000000000, 1.000000000000000000, 1.000000000000000000, 1.000000000000000000, 1.000000000000000000),
 ( 0.3333333333333333703, 0.3333333333333333703, 0.3333333333333333703, 0.3333333333333333703, 0.3333333333333333703, 0.3333333333333333703, 0.3333333333333333703, 0.3333333333333333703, 0.3333333333333333703, 0.3333333333333333703, 0.3333333333333333703, 0.3333333333333333703, 0.3333333333333333703, 0.3333333333333333703, 0.3333333333333333703, 0.3333333333333333703, 0.3333333333333333703, 0.3333333333333333703, 0.3333333333333333703, 0.3333333333333333703, 0.3333333333333333703, 0.3333333333333333703, 0.3333333333333333703, 0.3333333333333333703, 0.3333333333333333703, 0.3333333333333333703, 0.3333333333333333703, 0.3333333333333333703, 0.3333333333333333703, 0.3333333333333333703),
 ( 0.3333333333333333703, 0.3333333333333333703, 0.3333333333333333703, 0.3333333333333333703, 0.3333333333333333703, 0.3333333333333333703, 0.3333333333333333703, 0.3333333333333333703, 0.3333333333333333703, 0.3333333333333333703, 0.3333333333333333703, 0.3333333333333333703, 0.3333333333333333703, 0.3333333333333333703, 0.3333333333333333703, 0.3333333333333333703, 0.3333333333333333703, 0.3333333333333333703, 0.3333333333333333703, 0.3333333333333333703, 0.3333333333333333703, 0.3333333333333333703, 0.3333333333333333703, 0.3333333333333333703, 0.3333333333333333703, 0.3333333333333333703, 0.3333333333333333703, 0.3333333333333333703, 0.3333333333333333703, 0.3333333333333333703),
 ( 1.000000000000000000, 1.000000000000000000, 1.000000000000000000, 1.000000000000000000, 1.000000000000000000, 1.000000000000000000, 1.000000000000000000, 1.000000000000000000, 1.000000000000000000, 1.000000000000000000, 1.000000000000000000, 1.000000000000000000, 1.000000000000000000, 1.000000000000000000, 1.000000000000000000, 1.000000000000000000, 1.000000000000000000, 1.000000000000000000, 1.000000000000000000, 1.000000000000000000, 1.000000000000000000, 1.000000000000000000, 1.000000000000000000, 1.000000000000000000, 1.000000000000000000, 1.000000000000000000, 1.000000000000000000, 1.000000000000000000, 1.000000000000000000, 1.000000000000000000) ) ) 
 REPRESENTATION_ITEM ( '' )  SURFACE ( )  );
#11610=CARTESIAN_POINT ( 'NONE',  ( -208.1127848780265026, 1.189126717069624012E-13, -15.00245453012669472 ) ) ;
#11612=CARTESIAN_POINT ( 'NONE',  ( 14.38125909742181285, -15.17850393972633505, 0.000000000000000000 ) ) ;
#11613=CARTESIAN_POINT ( 'NONE',  ( -135.8532207217289454, -30.84685318188648750, -40.00000000000002132 ) ) ;
#11614=CARTESIAN_POINT ( 'NONE',  ( 130.8568914410475088, 24.07718906446891793, 32.49135343045489321 ) ) ;
#11615=CARTESIAN_POINT ( 'NONE',  ( -238.4067589809705794, -40.96449427990185654, -40.00000000000002132 ) ) ;
#11616=CARTESIAN_POINT ( 'NONE',  ( -114.5247514186166313, 19.74212785478623999, 9.597443935963386963 ) ) ;
#11617=CARTESIAN_POINT ( 'NONE',  ( -135.8532207217289738, -1.208299557080134822E-13, 9.153146818113572891 ) ) ;
#11618=CARTESIAN_POINT ( 'NONE',  ( -56.48582580120559271, 21.81201906317768291, 21.81201906317777173 ) ) ;
#11619=CARTESIAN_POINT ( 'NONE',  ( -30.26275506840324070, 41.69427246844628598, 2.449293598294708485E-15 ) ) ;
#11621=CARTESIAN_POINT ( 'NONE',  ( 23.64688638900299722, -42.77321027809698961, 23.28414885118088762 ) ) ;
#11624=CARTESIAN_POINT ( 'NONE',  ( -100.7734535825088500, 12.25131212657490209, -44.31723036834897300 ) ) ;
#11625=CARTESIAN_POINT ( 'NONE',  ( 200.0000000000000000, -40.00000000000005684, 19.99999999999978328 ) ) ;
#11626=CARTESIAN_POINT ( 'NONE',  ( 192.4448373802101173, 14.14213562370261279, 42.42640687122091236 ) ) ;
#11627=CARTESIAN_POINT ( 'NONE',  ( 57.59792236341147031, -2.435789363418150000, -40.00000000000002132 ) ) ;
#11630=CARTESIAN_POINT ( 'NONE',  ( -77.56349232229743507, 1.384135235510518758, -22.09269011744814648 ) ) ;
#11631=CARTESIAN_POINT ( 'NONE',  ( 91.82158438592158234, 16.11829626348378142, 40.45024623143977749 ) ) ;
#11632=CARTESIAN_POINT ( 'NONE',  ( 0.2972598230770048811, -10.13633138497415942, -66.70487387989865624 ) ) ;
#11633=CARTESIAN_POINT ( 'NONE',  ( -105.3824009378448494, 20.34996249420144565, -6.674565453639575985 ) ) ;
#11634=CARTESIAN_POINT ( 'NONE',  ( -82.23866184891308251, 13.36787606754487534, -15.15017645651541045 ) ) ;
#11635=CARTESIAN_POINT ( 'NONE',  ( -192.9588430854690273, -10.23066800231931239, -66.79921049724377724 ) ) ;
#11636=CARTESIAN_POINT ( 'NONE',  ( 170.2234770963711128, 17.36149277827028925, -39.20704971665377059 ) ) ;
#11637=CARTESIAN_POINT ( 'NONE',  ( -192.9588430854690273, -18.05360324515400094, -38.51493924976961836 ) ) ;
#11638=CARTESIAN_POINT ( 'NONE',  ( -238.4067589809705794, 0.6820004457912851592, -0.6820004457913123597 ) ) ;
#11639=CARTESIAN_POINT ( 'NONE',  ( 163.1118516004056573, -27.26290988616869626, 0.000000000000000000 ) ) ;
#11640=CARTESIAN_POINT ( 'NONE',  ( 136.1360204305621266, -24.77266263493116583, -24.77266263493127951 ) ) ;
#11642=CARTESIAN_POINT ( 'NONE',  ( -86.96347745069643054, -40.00000000000009948, 18.24025645688337960 ) ) ;
#11643=CARTESIAN_POINT ( 'NONE',  ( 146.6084372240433993, -3.800685668858652999, 3.800685668858636568 ) ) ;
#11644=CARTESIAN_POINT ( 'NONE',  ( 136.1360204305621266, 24.77266263493104148, 24.77266263493145004 ) ) ;
#11645=CARTESIAN_POINT ( 'NONE',  ( -135.8532207217289738, 30.84685318188643421, 40.00000000000002132 ) ) ;
#11647=EDGE_CURVE ( 'NONE', #13223, #9531, #10585, .T. ) ;
#11648=CARTESIAN_POINT ( 'NONE',  ( 4.995406935893287326, 67.35176059882533650, 10.78321810390163549 ) ) ;
#11650=CARTESIAN_POINT ( 'NONE',  ( 60.14720761598680099, 15.75494750870317517, 31.22869220294058934 ) ) ;
#11651=CARTESIAN_POINT ( 'NONE',  ( -100.7734535825088500, -22.67402823373193499, 40.00000000000002132 ) ) ;
#11653=CARTESIAN_POINT ( 'NONE',  ( -195.1686598215339075, -48.78512304066069305, 14.09692385499214673 ) ) ;
#11655=CARTESIAN_POINT ( 'NONE',  ( -0.1993645193002740457, -18.24262160098860264, 44.04158448240443846 ) ) ;
#11656=EDGE_CURVE ( 'NONE', #1634, #15141, #21471, .T. ) ;
#11657=EDGE_CURVE ( 'NONE', #15674, #8800, #3702, .T. ) ;
#11658=CARTESIAN_POINT ( 'NONE',  ( 25.31597067608072393, 17.58652183054798357, -42.45761951827109471 ) ) ;
#11661=CARTESIAN_POINT ( 'NONE',  ( -88.39148973765163930, -19.92926839984433229, -8.577159256668494436 ) ) ;
#11662=CARTESIAN_POINT ( 'NONE',  ( -238.4067589809705794, 39.99999999999997158, 0.9644942799827220803 ) ) ;
#11664=CARTESIAN_POINT ( 'NONE',  ( 8.517493190815718762, 49.32792454093251422, -14.17913040910384126 ) ) ;
#11665=CARTESIAN_POINT ( 'NONE',  ( -259.2033419157646676, -30.48217210827744950, 40.00000000000002132 ) ) ;
#11666=CARTESIAN_POINT ( 'NONE',  ( -187.3037411061767727, 23.25513534570619356, -42.71163782366665629 ) ) ;
#11667=CARTESIAN_POINT ( 'NONE',  ( 169.9999999999999716, 22.62041470344888339, -9.369682556672254137 ) ) ;
#11668=CARTESIAN_POINT ( 'NONE',  ( 98.29820294267349823, -16.98253775143801292, -10.58389073156956961 ) ) ;
#11669=CARTESIAN_POINT ( 'NONE',  ( -280.0000000000000568, 19.99999999999996092, -40.00000000000002132 ) ) ;
#11670=CARTESIAN_POINT ( 'NONE',  ( -135.8532207217289738, -9.153146818113595984, 40.00000000000002132 ) ) ;
#11671=CARTESIAN_POINT ( 'NONE',  ( 91.82158438592159655, -39.99999999999976552, -22.79471317813512599 ) ) ;
#11672=CARTESIAN_POINT ( 'NONE',  ( 199.9999999999999432, -1.727494763561684666E-13, 20.00000000000010303 ) ) ;
#11673=CARTESIAN_POINT ( 'NONE',  ( -198.0356074513804572, -10.87444709759714634, -10.87444709759729911 ) ) ;
#11676=CARTESIAN_POINT ( 'NONE',  ( 184.8905102610680444, 20.92133201514447194, 40.00000000000002132 ) ) ;
#11678=CARTESIAN_POINT ( 'NONE',  ( -99.31364972218659659, -8.933506367414295823, 20.48028939130929160 ) ) ;
#11680=ORIENTED_EDGE ( 'NONE', *, *, #13374, .T. ) ;
#11682=CARTESIAN_POINT ( 'NONE',  ( 98.29820294267528880, -14.14213562373450017, -14.14213562373441668 ) ) ;
#11683=CARTESIAN_POINT ( 'NONE',  ( 20.91285618069844077, -43.54130497318310233, -23.84652503052226535 ) ) ;
#11684=ORIENTED_EDGE ( 'NONE', *, *, #3297, .F. ) ;
#11685=CARTESIAN_POINT ( 'NONE',  ( 19.06497207195980792, 54.19242893257844429, -40.00000000000002132 ) ) ;
#11686=CARTESIAN_POINT ( 'NONE',  ( -105.4732637872244112, -19.68494377761390268, 8.153770687239109805 ) ) ;
#11689=STYLED_ITEM('',(#26409),#8606);
#11690=CONICAL_SURFACE ( 'NONE', #17632, 60.00000000000000000, 0.7853981633974447263 ) ;
#11691=CARTESIAN_POINT ( 'NONE',  ( -190.1935165880706222, 13.92226094463962127, 47.62328200654616950 ) ) ;
#11692=CARTESIAN_POINT ( 'NONE',  ( -86.96347745069644475, 12.89780903124401057, 12.89780903124407629 ) ) ;
#11694=CARTESIAN_POINT ( 'NONE',  ( 91.82158438592158234, 7.693928927950222250E-14, -17.20528682183300262 ) ) ;
#11696=CARTESIAN_POINT ( 'NONE',  ( -105.2054292635175585, -2.444554031225951202E-13, 21.49321519473985020 ) ) ;
#11701=CARTESIAN_POINT ( 'NONE',  ( 136.1360204305621266, -3.419521671106983309E-13, 35.03383547441296741 ) ) ;
#11703=CARTESIAN_POINT ( 'NONE',  ( 91.82158438592159655, -40.00000000000017764, 17.20528682183258340 ) ) ;
#11704=CARTESIAN_POINT ( 'NONE',  ( -110.1017491837281597, -13.37584907588316518, 15.18340520632177260 ) ) ;
#11705=CARTESIAN_POINT ( 'NONE',  ( -86.96347745069645896, -12.89780903124382938, -43.67073346367985920 ) ) ;
#11706=CARTESIAN_POINT ( 'NONE',  ( 146.6084372240433993, 34.62501878078308692, 0.000000000000000000 ) ) ;
#11707=CARTESIAN_POINT ( 'NONE',  ( -162.0762913951020892, -57.76657433524000851, 1.198031840315820329 ) ) ;
#11710=CARTESIAN_POINT ( 'NONE',  ( -3.486753633152337439, -47.18604396268657553, 13.85715877881439262 ) ) ;
#11711=CARTESIAN_POINT ( 'NONE',  ( -162.0762913951021176, 40.00000000000001421, -1.694272876827905394 ) ) ;
#11712=CARTESIAN_POINT ( 'NONE',  ( -105.3755690713226727, 5.661656051307470077E-14, -21.75974354311649961 ) ) ;
#11713=CARTESIAN_POINT ( 'NONE',  ( 4.995406935893294431, -17.50105314357198694, 39.06748935135188816 ) ) ;
#11715=CARTESIAN_POINT ( 'NONE',  ( 136.1360204305621266, 24.77266263493104148, 24.77266263493145004 ) ) ;
#11716=CARTESIAN_POINT ( 'NONE',  ( -195.1685814578710279, -14.09692187701076982, -48.78510996053330473 ) ) ;
#11717=CARTESIAN_POINT ( 'NONE',  ( -86.96347745069645896, -12.89780903124382938, -43.67073346367985920 ) ) ;
#11719=CARTESIAN_POINT ( 'NONE',  ( -280.0000000000000000, 14.14213562373108246, -14.14213562373078581 ) ) ;
#11723=CARTESIAN_POINT ( 'NONE',  ( -77.90255099906767100, 8.064892378658102601, -20.29001641120677846 ) ) ;
#11724=CARTESIAN_POINT ( 'NONE',  ( -105.3755690713226585, -43.67073346367964604, -12.89780903124457545 ) ) ;
#11726=VERTEX_POINT ( 'NONE', #17727 ) ;
#11727=CARTESIAN_POINT ( 'NONE',  ( 170.2234770963711128, -2.259079968736224833E-13, 24.55285855007187124 ) ) ;
#11728=ADVANCED_FACE ( 'NONE', ( #21603 ), #19464, .T. ) ;
#11730=CARTESIAN_POINT ( 'NONE',  ( -3.675706741950853118, 17.91131112508025680, 43.24173023805306570 ) ) ;
#11732=ORIENTED_EDGE ( 'NONE', *, *, #16051, .F. ) ;
#11733=CARTESIAN_POINT ( 'NONE',  ( -213.1075012329537230, 13.71589010951907817, -40.00000000000002132 ) ) ;
#11734=CARTESIAN_POINT ( 'NONE',  ( 91.82158438592158234, 12.16597498397773869, -12.16597498397759303 ) ) ;
#11735=CARTESIAN_POINT ( 'NONE',  ( -105.3755690713226585, 39.99999999999993605, 18.24025645688366737 ) ) ;
#11736=CARTESIAN_POINT ( 'NONE',  ( -114.5520593196445418, -19.58754258080286093, -9.956319649466946586 ) ) ;
#11738=CARTESIAN_POINT ( 'NONE',  ( 23.37394308801978937, 23.33966569535129310, -42.85717664514559999 ) ) ;
#11741=CARTESIAN_POINT ( 'NONE',  ( 6.011245401487375517, -18.54985650213898651, -44.78331514753573828 ) ) ;
#11742=CARTESIAN_POINT ( 'NONE',  ( -56.48582580120559982, 34.75652343174628101, -21.81201906317743067 ) ) ;
#11744=EDGE_CURVE ( 'NONE', #10228, #1453, #9403, .T. ) ;
#11745=CARTESIAN_POINT ( 'NONE',  ( -397.9898987322331436, -69.99999999999998579, 8.572527594031463526E-15 ) ) ;
#11746=CARTESIAN_POINT ( 'NONE',  ( 4.995406935893310418, -67.35176059880237176, 10.78321810387813429 ) ) ;
#11747=CARTESIAN_POINT ( 'NONE',  ( 57.59792236341148453, -40.00000000000003553, 2.435789363417741438 ) ) ;
#11750=CARTESIAN_POINT ( 'NONE',  ( 130.8568914410475088, -5.949712681206671405, 40.00000000000002132 ) ) ;
#11751=CARTESIAN_POINT ( 'NONE',  ( 170.2234770963711128, 17.36149277826973503, 39.20704971665401217 ) ) ;
#11752=CARTESIAN_POINT ( 'NONE',  ( -105.3755690713226727, -18.24025645688354302, -2.449293598294708485E-15 ) ) ;
#11753=CARTESIAN_POINT ( 'NONE',  ( -105.3175882261754310, 5.408274864382292435, 20.76660717853357951 ) ) ;
#11755=EDGE_CURVE ( 'NONE', #22554, #23676, #3371, .T. ) ;
#11756=CARTESIAN_POINT ( 'NONE',  ( 136.1360204305621266, 3.511608612530704665, 3.511608612530695339 ) ) ;
#11758=CARTESIAN_POINT ( 'NONE',  ( 14.38125909742180752, 55.17850393971008316, -40.00000000000002132 ) ) ;
#11759=ORIENTED_EDGE ( 'NONE', *, *, #14441, .T. ) ;
#11761=CARTESIAN_POINT ( 'NONE',  ( -200.0000000000000000, -44.88127304974053544, -30.70179486994611295 ) ) ;
#11762=AXIS2_PLACEMENT_3D ( 'NONE', #20827, #4602, #8578 ) ;
#11763=CARTESIAN_POINT ( 'NONE',  ( 163.1118516004056573, 9.006482792074356425, -47.56205970284957374 ) ) ;
#11764=CARTESIAN_POINT ( 'NONE',  ( 170.2234770963711128, -2.511315425431857630E-14, 15.44714144992816074 ) ) ;
#11766=CARTESIAN_POINT ( 'NONE',  ( 170.2234770963711128, -2.259079968736224833E-13, 24.55285855007187124 ) ) ;
#11768=CARTESIAN_POINT ( 'NONE',  ( -86.96347745069644475, -21.75974354311651737, 0.000000000000000000 ) ) ;
#11769=CARTESIAN_POINT ( 'NONE',  ( -87.13361725327072804, 5.903697393916396424E-14, -21.49321519333428299 ) ) ;
#11772=CARTESIAN_POINT ( 'NONE',  ( 4.995406935893290878, 39.06748935135239265, -39.06748935135144762 ) ) ;
#11773=CARTESIAN_POINT ( 'NONE',  ( 0.2972598230769923355, 18.14793986248751168, -38.42060263243650553 ) ) ;
#11774=B_SPLINE_CURVE_WITH_KNOTS ( 'NONE', 3,
 ( #5115, #25598, #19456, #15212, #3493, #17457 ),
 .UNSPECIFIED., .F., .F.,
 ( 4, 2, 4 ),
 ( -5.998621905801447002E-08, 0.03937827992696037865, 0.07875661984013980488 ),
 .UNSPECIFIED. ) ;
#11775=CARTESIAN_POINT ( 'NONE',  ( 151.7948205124836250, 23.49921654116361225, -23.49921654116333514 ) ) ;
#11776=CARTESIAN_POINT ( 'NONE',  ( -77.72936527555063435, 19.09948130765502938, -10.88227939677040013 ) ) ;
#11777=CARTESIAN_POINT ( 'NONE',  ( 146.6084372240433709, 24.48358557860356655, -32.08495691632035118 ) ) ;
#11778=CARTESIAN_POINT ( 'NONE',  ( -91.56559293963834989, 16.03295912088740849, -40.53558337403661938 ) ) ;
#11779=CARTESIAN_POINT ( 'NONE',  ( 0.2972598230770011618, 10.13633138497555919, -66.70487387989845729 ) ) ;
#11780=CARTESIAN_POINT ( 'NONE',  ( 19.06497207195981858, 10.03556273973516078, -66.60410523465806421 ) ) ;
#11781=CARTESIAN_POINT ( 'NONE',  ( 151.7948205124836250, -33.23291073765550863, 0.000000000000000000 ) ) ;
#11782=CARTESIAN_POINT ( 'NONE',  ( 98.29820294269173075, 19.99999999998819433, -2.308575297063409524E-13 ) ) ;
#11784=CARTESIAN_POINT ( 'NONE',  ( 192.4448373802100889, 1.051811698935164031E-13, -20.00000000003942091 ) ) ;
#11785=CARTESIAN_POINT ( 'NONE',  ( 57.59792236341148453, 1.722363176414758668, 54.84617931850880268 ) ) ;
#11787=CARTESIAN_POINT ( 'NONE',  ( 91.82158438592158234, -17.20528682183298486, 40.00000000000002132 ) ) ;
#11788=ORIENTED_EDGE ( 'NONE', *, *, #4630, .T. ) ;
#11789=CARTESIAN_POINT ( 'NONE',  ( 146.6084372240433709, 3.800685668858776900, -52.76785682606518435 ) ) ;
#11791=CARTESIAN_POINT ( 'NONE',  ( -188.2995950289364373, 13.82811170417132196, 46.99046209955516673 ) ) ;
#11793=CARTESIAN_POINT ( 'NONE',  ( -91.56559293963834989, -22.67402823373193499, 0.000000000000000000 ) ) ;
#11795=CARTESIAN_POINT ( 'NONE',  ( -188.4265004370326722, -47.03620155434649064, 13.83489460444966923 ) ) ;
#11797=CARTESIAN_POINT ( 'NONE',  ( 8.556015491674958895, -24.84887822174851024, 44.89939803569725285 ) ) ;
#11798=CARTESIAN_POINT ( 'NONE',  ( 23.48902902575126106, 23.31625887490740823, -42.82177761400715355 ) ) ;
#11801=CARTESIAN_POINT ( 'NONE',  ( 151.7948205124836250, 1.439163438361279259E-13, -33.23291073765553705 ) ) ;
#11802=CARTESIAN_POINT ( 'NONE',  ( -135.8532207217289738, -6.472252184283586729, -50.09629031063973770 ) ) ;
#11803=CARTESIAN_POINT ( 'NONE',  ( 19.06497207195980792, -14.19242893257839988, 40.00000000000002132 ) ) ;
#11804=CARTESIAN_POINT ( 'NONE',  ( -121.8425463771063164, 9.420908039661981093, -22.74408395512567793 ) ) ;
#11806=CARTESIAN_POINT ( 'NONE',  ( 0.2972598230769983307, -14.33493731733933352, 0.000000000000000000 ) ) ;
#11807=CARTESIAN_POINT ( 'NONE',  ( -213.1075012329537230, -13.71589010951915810, -40.00000000000002132 ) ) ;
#11808=CARTESIAN_POINT ( 'NONE',  ( -198.0356074513804572, 15.37879056873067007, 0.000000000000000000 ) ) ;
#11809=CARTESIAN_POINT ( 'NONE',  ( 151.7948205124836534, -39.99999999999992184, -6.767089262349454515 ) ) ;
#11810=CARTESIAN_POINT ( 'NONE',  ( -208.1127848780265026, 1.189126717069624012E-13, -15.00245453012669472 ) ) ;
#11811=CARTESIAN_POINT ( 'NONE',  ( 163.1118516004056573, 19.27778845538753316, 19.27778845538783870 ) ) ;
#11812=VERTEX_POINT ( 'NONE', #8019 ) ;
#11813=CARTESIAN_POINT ( 'NONE',  ( -53.37769371738608726, 27.95780717557945039, -13.65853730965343260 ) ) ;
#11814=CARTESIAN_POINT ( 'NONE',  ( -198.0356074513804572, 10.87444709759714989, 10.87444709759722450 ) ) ;
#11815=EDGE_CURVE ( 'NONE', #13176, #4726, #7916, .T. ) ;
#11816=CARTESIAN_POINT ( 'NONE',  ( -100.0957100001397748, -8.517115559226354549, 20.56213589532580954 ) ) ;
#11820=CARTESIAN_POINT ( 'NONE',  ( 14.38125909742181818, -39.01709431150904095, -17.55144818341490165 ) ) ;
#11821=CARTESIAN_POINT ( 'NONE',  ( 27.26078259668992843, -41.90087417143951853, -17.35591035705024510 ) ) ;
#11823=CARTESIAN_POINT ( 'NONE',  ( -213.1075012329537230, 13.71589010951907817, -40.00000000000002132 ) ) ;
#11824=CARTESIAN_POINT ( 'NONE',  ( -102.4309680866104202, -20.43798635336410285, 8.087567261735790325 ) ) ;
#11828=CARTESIAN_POINT ( 'NONE',  ( 170.0000000000133014, 17.64300463311800016, 17.64300463311827016 ) ) ;
#11829=CARTESIAN_POINT ( 'NONE',  ( 192.4448373802100889, 14.14213562370310662, 14.14213562370312438 ) ) ;
#11830=CARTESIAN_POINT ( 'NONE',  ( -188.2652746676668869, -46.97858116095166281, -13.82569223135941883 ) ) ;
#11831=CARTESIAN_POINT ( 'NONE',  ( 184.8905102610680444, 1.070102760522089011E-13, -20.92133201514444352 ) ) ;
#11832=CARTESIAN_POINT ( 'NONE',  ( 192.4448373802101173, -20.00000000003938538, 40.00000000000002132 ) ) ;
#11835=CARTESIAN_POINT ( 'NONE',  ( -86.96347745069644475, 5.999880687339585546E-14, -21.75974354311649961 ) ) ;
#11836=CARTESIAN_POINT ( 'NONE',  ( -105.3755690713226585, -40.00000000000027711, 21.75974354311608749 ) ) ;
#11837=CARTESIAN_POINT ( 'NONE',  ( 170.0000000000000000, -3.062538285712981700, -24.95097643317001612 ) ) ;
#11838=CARTESIAN_POINT ( 'NONE',  ( -30.26275506840322649, -29.48230279907810925, 29.48230279907778950 ) ) ;
#11839=CARTESIAN_POINT ( 'NONE',  ( 136.1360204305621266, 35.03383547441298163, -40.00000000000002132 ) ) ;
#11840=CARTESIAN_POINT ( 'NONE',  ( -86.96347745069643054, -41.18208027870589660, -15.38646221621809040 ) ) ;
#11841=CARTESIAN_POINT ( 'NONE',  ( 200.0000000000000000, -40.00000000000000711, 4.898587196589418548E-15 ) ) ;
#11842=AXIS2_PLACEMENT_3D ( 'NONE', #22695, #8583, #16694 ) ;
#11843=( BOUNDED_CURVE ( )  B_SPLINE_CURVE ( 3, ( #5356, #13463, #21583, #20512 ),
 .UNSPECIFIED., .F., .F. ) 
 B_SPLINE_CURVE_WITH_KNOTS ( ( 4, 4 ),
 ( 0.004183487405659313055, 0.01388163287021778290 ),
 .UNSPECIFIED. ) 
 CURVE ( )  GEOMETRIC_REPRESENTATION_ITEM ( )  RATIONAL_B_SPLINE_CURVE ( ( 0.6809743333591573577, 0.7608653435686164590, 0.8672072324488973027, 1.000000000000000000 ) ) 
 REPRESENTATION_ITEM ( '' )  );
#11844=CARTESIAN_POINT ( 'NONE',  ( 5.009865950673486168, -49.09576456953146817, 14.14399394884959804 ) ) ;
#11845=CARTESIAN_POINT ( 'NONE',  ( 136.1360204305621266, 24.77266263493104148, 24.77266263493145004 ) ) ;
#11846=CARTESIAN_POINT ( 'NONE',  ( -30.26275506840324070, -40.00000000000003553, 1.694272468446120117 ) ) ;
#11847=CARTESIAN_POINT ( 'NONE',  ( 151.7948205124836534, 33.06932595376365924, -23.49921654116018743 ) ) ;
#11848=CARTESIAN_POINT ( 'NONE',  ( -114.6854600082618276, 12.16985185534088920, 18.38493165714585231 ) ) ;
#11849=CARTESIAN_POINT ( 'NONE',  ( -189.1288815661498006, -13.87115472123443283, -47.28031329127929183 ) ) ;
#11853=CARTESIAN_POINT ( 'NONE',  ( 91.82158438592158234, -40.45024623143936537, -16.11829626348475131 ) ) ;
#11854=CARTESIAN_POINT ( 'NONE',  ( 184.8905102610680444, 14.79361573936396113, -14.79361573936377461 ) ) ;
#11855=CARTESIAN_POINT ( 'NONE',  ( -259.2033419157646676, 9.517827891722582478, -40.00000000000002132 ) ) ;
#11857=CARTESIAN_POINT ( 'NONE',  ( 184.8905102610680444, -43.07788698682556827, -13.49065550809859104 ) ) ;
#11858=CARTESIAN_POINT ( 'NONE',  ( -87.13361725327072804, 21.49321519333427233, -1.448021113139547951E-30 ) ) ;
#11861=CARTESIAN_POINT ( 'NONE',  ( 35.93702930655396699, -12.87541766444613778, -42.26928858172315273 ) ) ;
#11862=CARTESIAN_POINT ( 'NONE',  ( -3.449394506063832466, 17.93655106166724522, 43.30266483527507404 ) ) ;
#11865=CARTESIAN_POINT ( 'NONE',  ( -56.48582580120559271, -9.153146818113595984, 0.000000000000000000 ) ) ;
#11867=CARTESIAN_POINT ( 'NONE',  ( -77.90255099906769942, -8.644468104261466834, -20.04994828523962980 ) ) ;
#11868=CARTESIAN_POINT ( 'NONE',  ( -94.58360650941212100, -20.91945674511385533, -8.190527749482289011 ) ) ;
#11869=DIRECTION ( 'NONE',  ( 1.000000000000000000, 1.836970198721030181E-16, 0.000000000000000000 ) ) ;
#11871=CARTESIAN_POINT ( 'NONE',  ( -30.26275506840324070, 1.218738420030236455E-14, -1.694272468446259783 ) ) ;
#11876=CARTESIAN_POINT ( 'NONE',  ( -114.4364955367310586, 8.064892380842531239, 20.29001642038765141 ) ) ;
#11877=CARTESIAN_POINT ( 'NONE',  ( -3.449394506061945531, -17.93655106166727720, -43.30266483527577037 ) ) ;
#11878=CARTESIAN_POINT ( 'NONE',  ( -162.0762913951020607, -57.76657433537922515, -1.198031840455874963 ) ) ;
#11879=CARTESIAN_POINT ( 'NONE',  ( 146.6084372240433993, -24.48358557860353457, 24.48358557860296258 ) ) ;
#11880=CARTESIAN_POINT ( 'NONE',  ( -91.56559293963834989, -12.25131212657492874, 12.25131212657477953 ) ) ;
#11881=CARTESIAN_POINT ( 'NONE',  ( -56.48582580120558561, -40.00000000000012790, 9.153146818113166105 ) ) ;
#11882=FACE_OUTER_BOUND ( 'NONE', #9305, .T. ) ;
#11883=CARTESIAN_POINT ( 'NONE',  ( 199.9999999999999432, 14.14213562373093680, 14.14213562373114641 ) ) ;
#11884=CARTESIAN_POINT ( 'NONE',  ( -30.26275506840322649, -41.69427246844630019, -2.449293598294708485E-15 ) ) ;
#11886=CARTESIAN_POINT ( 'NONE',  ( 57.59792236341148453, -37.56421063658185489, -2.449293598294708485E-15 ) ) ;
#11887=CARTESIAN_POINT ( 'NONE',  ( -114.7852463542949124, 14.79002490267117054, 16.52851182054974188 ) ) ;
#11889=CARTESIAN_POINT ( 'NONE',  ( -114.7284988330193443, 21.83722598071101828, -3.361565411871531683 ) ) ;
#11890=CARTESIAN_POINT ( 'NONE',  ( -208.1127848780265026, 10.60833733269537049, 10.60833733269544510 ) ) ;
#11891=CARTESIAN_POINT ( 'NONE',  ( -259.2033419157646676, -9.517827891722680178, -40.00000000000002132 ) ) ;
#11892=VERTEX_POINT ( 'NONE', #14144 ) ;
#11894=CARTESIAN_POINT ( 'NONE',  ( 37.15749683985864493, -38.58455518503008363, 20.52531616262464098 ) ) ;
#11895=CARTESIAN_POINT ( 'NONE',  ( 98.29820294272414571, 7.653668647302724892, 18.47759065022804137 ) ) ;
#11896=EDGE_CURVE ( 'NONE', #20612, #23081, #15872, .T. ) ;
#11897=CARTESIAN_POINT ( 'NONE',  ( 14.38125909742180397, 67.30136555895953165, 10.73282306403583242 ) ) ;
#11898=CARTESIAN_POINT ( 'NONE',  ( 136.1360204305621551, -40.00000000000001421, 4.966164525586921563 ) ) ;
#11899=CARTESIAN_POINT ( 'NONE',  ( 184.8905102610680444, -14.79361573936399665, 14.79361573936367158 ) ) ;
#11901=CARTESIAN_POINT ( 'NONE',  ( -213.1075012329537230, 13.71589010951907817, 40.00000000000002132 ) ) ;
#11902=CARTESIAN_POINT ( 'NONE',  ( 19.06497207195980792, 54.19242893257844429, -40.00000000000002132 ) ) ;
#11908=CARTESIAN_POINT ( 'NONE',  ( -238.4067589809705794, 57.25054294065799354, -0.6820004457334954973 ) ) ;
#11909=CARTESIAN_POINT ( 'NONE',  ( -238.4067589809705794, -28.96627169325352469, 27.60227080167035041 ) ) ;
#11911=CARTESIAN_POINT ( 'NONE',  ( 184.8905102610680444, 14.79361573936396113, -14.79361573936377461 ) ) ;
#11912=CARTESIAN_POINT ( 'NONE',  ( -82.24297220888476545, 15.98176361809532331, -12.40742895870143059 ) ) ;
#11913=CARTESIAN_POINT ( 'NONE',  ( 130.8568914410475088, -4.207082182990058428, 52.36146031193416661 ) ) ;
#11914=CARTESIAN_POINT ( 'NONE',  ( 192.4448373802100889, -14.14213562370293431, -14.14213562370322030 ) ) ;
#11916=CARTESIAN_POINT ( 'NONE',  ( 57.59792236341147031, -1.722363176414363206, -54.84617931850881689 ) ) ;
#11917=CARTESIAN_POINT ( 'NONE',  ( -105.3755690713226727, 15.38646221621793231, -15.38646221621779020 ) ) ;
#11920=CARTESIAN_POINT ( 'NONE',  ( -192.9588430854690273, -40.00000000000024158, 54.46834944101708231 ) ) ;
#11921=CARTESIAN_POINT ( 'NONE',  ( -213.1075012329537230, -9.698598906450557777, 9.698598906450415669 ) ) ;
#11922=CARTESIAN_POINT ( 'NONE',  ( -105.3755690713226585, -21.75974354311652448, 40.00000000000002132 ) ) ;
#11924=CARTESIAN_POINT ( 'NONE',  ( 19.06497207195980792, 10.03556273973433299, 10.03556273973436319 ) ) ;
#11925=CARTESIAN_POINT ( 'NONE',  ( -4.119579890815007417, 42.21781124616257586, 17.48718999186797873 ) ) ;
#11926=CARTESIAN_POINT ( 'NONE',  ( 67.79414719530582545, 10.30785037361446044, 30.31905270965464538 ) ) ;
#11927=CARTESIAN_POINT ( 'NONE',  ( -135.8532207217289738, -9.153146818113595984, 0.000000000000000000 ) ) ;
#11929=CARTESIAN_POINT ( 'NONE',  ( -198.9234529670461598, -49.24835336344875714, 14.16707775654302459 ) ) ;
#11931=CARTESIAN_POINT ( 'NONE',  ( 2.692156443725823411, -18.42752958146757436, 44.48799183655690825 ) ) ;
#11932=CARTESIAN_POINT ( 'NONE',  ( 13.28449813596364848, 24.75673736218053023, -44.77439867187970179 ) ) ;
#11934=AXIS2_PLACEMENT_3D ( 'NONE', #7500, #23869, #14025 ) ;
#11935=CARTESIAN_POINT ( 'NONE',  ( 140.2235668266257278, -30.42137084504314615, 12.60094438999813704 ) ) ;
#11936=CARTESIAN_POINT ( 'NONE',  ( 146.6084372240433993, 1.478241399363601114E-13, -34.62501878078305850 ) ) ;
#11937=CARTESIAN_POINT ( 'NONE',  ( 192.4448373802101173, 42.42640687116487896, 14.14213562375934075 ) ) ;
#11938=CARTESIAN_POINT ( 'NONE',  ( 91.82158438592159655, -22.79471317813468900, 40.00000000000002132 ) ) ;
#11939=CIRCLE ( 'NONE', #493, 60.00000000000011369 ) ;
#11940=CARTESIAN_POINT ( 'NONE',  ( -188.3392995398626510, 13.83024151208869235, -47.00482667599663955 ) ) ;
#11941=CARTESIAN_POINT ( 'NONE',  ( -259.2033419157646676, -6.730120644403663199, 6.730120644403451813 ) ) ;
#11942=CARTESIAN_POINT ( 'NONE',  ( 98.29820294267410929, -15.89413956777455539, -12.20973600806684622 ) ) ;
#11943=CARTESIAN_POINT ( 'NONE',  ( -91.56559293963836410, 22.67402823373190301, -40.00000000000002132 ) ) ;
#11944=AXIS2_PLACEMENT_3D ( 'NONE', #17185, #24797, #6549 ) ;
#11945=CARTESIAN_POINT ( 'NONE',  ( -208.1127848780264742, 15.00245453012665742, 40.00000000000002132 ) ) ;
#11946=CARTESIAN_POINT ( 'NONE',  ( 91.82158438592158234, 2.580785920671402147E-13, -22.79471317813470321 ) ) ;
#11947=CARTESIAN_POINT ( 'NONE',  ( 19.06497207195981147, 38.31983398719620482, 38.31983398719633271 ) ) ;
#11948=CARTESIAN_POINT ( 'NONE',  ( 146.6084372240433993, -3.357462877844280890E-13, 34.62501878078305850 ) ) ;
#11949=CARTESIAN_POINT ( 'NONE',  ( 91.82158438592156813, 40.45024623143973486, -16.11829626348390931 ) ) ;
#11953=CARTESIAN_POINT ( 'NONE',  ( -94.58360650944290171, -8.190527749669946900, 20.91945674502963826 ) ) ;
#11957=CARTESIAN_POINT ( 'NONE',  ( -192.9588430854690273, -66.79921049724377724, 10.23066800231950069 ) ) ;
#11958=CARTESIAN_POINT ( 'NONE',  ( 27.79909650602947835, -41.49206490658383473, -22.43832426412121350 ) ) ;
#11960=CARTESIAN_POINT ( 'NONE',  ( 136.1360204305621551, -35.03383547441293899, -40.00000000000002132 ) ) ;
#11961=CARTESIAN_POINT ( 'NONE',  ( -4.039451493210490796, -23.44932283416679297, 43.00522595894000943 ) ) ;
#11964=AXIS2_PLACEMENT_3D ( 'NONE', #128, #22089, #10366 ) ;
#11966=CARTESIAN_POINT ( 'NONE',  ( -105.3755690713226585, 12.89780903124410472, -43.67073346367977393 ) ) ;
#11967=CARTESIAN_POINT ( 'NONE',  ( -151.4802930569763362, -31.86309827676129558, -16.17241674347988578 ) ) ;
#11968=CARTESIAN_POINT ( 'NONE',  ( 4.995406935893297984, -40.00000000000007816, 15.24977328854818914 ) ) ;
#11969=CARTESIAN_POINT ( 'NONE',  ( -100.7734535825088500, -22.67402823373193499, 40.00000000000002132 ) ) ;
#11972=CARTESIAN_POINT ( 'NONE',  ( 163.1118516004056573, -39.99999999999990052, -27.26290988616886679 ) ) ;
#11973=CARTESIAN_POINT ( 'NONE',  ( -56.48582580120558561, -40.00000000000012790, 9.153146818113166105 ) ) ;
#11975=CARTESIAN_POINT ( 'NONE',  ( -199.9999999999998863, -44.86878812508856385, -24.82633483071075986 ) ) ;
#11976=CARTESIAN_POINT ( 'NONE',  ( 130.8568914410475088, -32.49135343045460900, -24.07718906446924478 ) ) ;
#11977=CARTESIAN_POINT ( 'NONE',  ( -198.0356074513804572, -15.37879056873074290, -40.00000000000002132 ) ) ;
#11978=CARTESIAN_POINT ( 'NONE',  ( 192.4448373802101173, -42.42640687116490028, -14.14213562375904942 ) ) ;
#11981=CARTESIAN_POINT ( 'NONE',  ( 170.0000000000133014, 17.64300463311800016, 17.64300463311827016 ) ) ;
#11982=CARTESIAN_POINT ( 'NONE',  ( -213.1075012329537230, -8.703598725189323045E-14, 13.71589010951911902 ) ) ;
#11983=CARTESIAN_POINT ( 'NONE',  ( -86.96347745069644475, 12.89780903124410472, -43.67073346367977393 ) ) ;
#11986=CARTESIAN_POINT ( 'NONE',  ( -188.4702232936901396, -23.48628015403117431, -43.05505437950768766 ) ) ;
#11988=ORIENTED_EDGE ( 'NONE', *, *, #3013, .T. ) ;
#11989=CARTESIAN_POINT ( 'NONE',  ( 200.0000000000000000, -14.14213562373046784, -42.42640687119298804 ) ) ;
#11990=CARTESIAN_POINT ( 'NONE',  ( -77.92915424793434909, 20.15198149301296482, 8.347224043097730473 ) ) ;
#11991=CARTESIAN_POINT ( 'NONE',  ( -162.0762913951020892, -1.198031840385783919, 1.198031840385741731 ) ) ;
#11992=FACE_OUTER_BOUND ( 'NONE', #23429, .T. ) ;
#11993=CARTESIAN_POINT ( 'NONE',  ( 85.88462074443611982, 10.32536233759628708, 22.72792765570313023 ) ) ;
#11994=CARTESIAN_POINT ( 'NONE',  ( 151.7948205124836534, -51.78348778862529400, -4.785054706299085581 ) ) ;
#11995=CARTESIAN_POINT ( 'NONE',  ( 85.88462074442188054, -22.72792765587123398, 10.32536233720564667 ) ) ;
#11996=ORIENTED_EDGE ( 'NONE', *, *, #9622, .T. ) ;
#12000=CARTESIAN_POINT ( 'NONE',  ( -4.260882601032770722, 13.81249720866915709, 46.91379881627262449 ) ) ;
#12003=CARTESIAN_POINT ( 'NONE',  ( 14.38125909742180752, 10.73282306404720465, 10.73282306404724018 ) ) ;
#12005=CARTESIAN_POINT ( 'NONE',  ( -110.1017833366170748, 9.974944988646792322E-14, -20.19517362627950874 ) ) ;
#12007=DIRECTION ( 'NONE',  ( -0.01051738777842040756, -0.3995761382618722712, -0.9166396752737944187 ) ) ;
#12008=CARTESIAN_POINT ( 'NONE',  ( 22.27781863259630768, 43.19367102554032556, -23.58928354771935076 ) ) ;
#12009=EDGE_CURVE ( 'NONE', #22947, #151, #475, .T. ) ;
#12010=CARTESIAN_POINT ( 'NONE',  ( 35.93765736440253278, 20.78447772034747842, -38.99300256376233875 ) ) ;
#12013=CARTESIAN_POINT ( 'NONE',  ( -53.37686176745753386, -13.65870576116508239, 27.95807077219537717 ) ) ;
#12015=CARTESIAN_POINT ( 'NONE',  ( -163.7067538432321783, 35.82971521589534092, 14.84115397836969485 ) ) ;
#12016=CARTESIAN_POINT ( 'NONE',  ( -4.558244102846352064, -13.79151199599447963, -46.81081390833299594 ) ) ;
#12017=CARTESIAN_POINT ( 'NONE',  ( -30.26275506840322294, -57.76657404653985139, -1.198031551616531853 ) ) ;
#12018=CARTESIAN_POINT ( 'NONE',  ( -105.3174728402264151, 5.408230752242470629, -20.76733781320130490 ) ) ;
#12019=CARTESIAN_POINT ( 'NONE',  ( -100.7734535825088358, -12.25131212657493052, 12.25131212657478130 ) ) ;
#12020=CARTESIAN_POINT ( 'NONE',  ( -238.4067589809705794, -40.00000000000005684, -0.9644942799830014124 ) ) ;
#12022=CARTESIAN_POINT ( 'NONE',  ( 184.8905102610680444, -19.07866798485554938, 40.00000000000002132 ) ) ;
#12023=CARTESIAN_POINT ( 'NONE',  ( 136.1360204305621266, 24.77266263493138965, -24.77266263493110188 ) ) ;
#12024=CARTESIAN_POINT ( 'NONE',  ( -91.56559293963834989, -17.32597176626812896, 40.00000000000002132 ) ) ;
#12025=CARTESIAN_POINT ( 'NONE',  ( -110.0996815860078328, 15.29816958059242538, 13.19859759219660766 ) ) ;
#12026=CARTESIAN_POINT ( 'NONE',  ( 57.59792236341147031, 40.00000000000042633, -37.56421063658144277 ) ) ;
#12027=CARTESIAN_POINT ( 'NONE',  ( -192.9588430854690273, 38.51493924976939098, -18.05360324515436687 ) ) ;
#12028=CARTESIAN_POINT ( 'NONE',  ( -105.3755690713226585, -21.75974354311652448, -40.00000000000002132 ) ) ;
#12029=ORIENTED_EDGE ( 'NONE', *, *, #13374, .F. ) ;
#12030=CARTESIAN_POINT ( 'NONE',  ( -259.2033419157646676, -9.517827891722680178, 40.00000000000002132 ) ) ;
#12032=CARTESIAN_POINT ( 'NONE',  ( -192.9588430854690273, 66.79921049721887982, 10.23066800229522677 ) ) ;
#12033=CARTESIAN_POINT ( 'NONE',  ( -198.0356074513804572, -2.321818583541004323E-13, 55.37879056873073580 ) ) ;
#12034=CARTESIAN_POINT ( 'NONE',  ( 163.1118516004056573, 9.006482792073693844, 47.56205970284970164 ) ) ;
#12035=CARTESIAN_POINT ( 'NONE',  ( 184.8905102610680444, -1.851754852062639767E-13, 20.92133201514444352 ) ) ;
#12036=CARTESIAN_POINT ( 'NONE',  ( -199.9999999999998863, -44.86878812508856385, -24.82633483071075986 ) ) ;
#12037=CARTESIAN_POINT ( 'NONE',  ( -138.9613193423055861, -27.95779829447855747, -13.65853114841838334 ) ) ;
#12040=CARTESIAN_POINT ( 'NONE',  ( 130.8568914410475372, 4.207082182992923691, -4.207082182992794017 ) ) ;
#12041=CARTESIAN_POINT ( 'NONE',  ( -213.1075012329537230, -66.26714140136188291, -9.698598906438677503 ) ) ;
#12042=CARTESIAN_POINT ( 'NONE',  ( -105.3382940165702166, 20.63437339945704352, 5.722104500121528048 ) ) ;
#12043=CARTESIAN_POINT ( 'NONE',  ( -208.1127848780265026, 1.189126717069624012E-13, -15.00245453012669472 ) ) ;
#12044=CARTESIAN_POINT ( 'NONE',  ( -56.48582580120558561, -50.09629031063971638, 6.472252184283745713 ) ) ;
#12046=CARTESIAN_POINT ( 'NONE',  ( -259.2033419157646676, -6.730120644403663199, 6.730120644403451813 ) ) ;
#12047=CARTESIAN_POINT ( 'NONE',  ( 136.1360204305621266, -3.511608612530379592, -53.05693388239318153 ) ) ;
#12049=EDGE_CURVE ( 'NONE', #2955, #17072, #51, .T. ) ;
#12051=CARTESIAN_POINT ( 'NONE',  ( 91.82158438592158234, 7.693928927950222250E-14, -17.20528682183300262 ) ) ;
#12052=CARTESIAN_POINT ( 'NONE',  ( -213.1075012329537230, -9.698598906450422774, -9.698598906450550672 ) ) ;
#12053=CARTESIAN_POINT ( 'NONE',  ( 9.006212071497149196, 44.90541342374627476, -24.85331907610142821 ) ) ;
#12054=CARTESIAN_POINT ( 'NONE',  ( -259.2033419157646676, 30.48217210827735713, -40.00000000000002132 ) ) ;
#12056=CARTESIAN_POINT ( 'NONE',  ( 12.01676469546555559, -24.84032989753396237, -44.88780742856565809 ) ) ;
#12057=EDGE_CURVE ( 'NONE', #16316, #7090, #25110, .T. ) ;
#12058=CARTESIAN_POINT ( 'NONE',  ( 23.10131000537883850, 42.18277622344346867, 17.47267801029965284 ) ) ;
#12061=CARTESIAN_POINT ( 'NONE',  ( 146.6084372240433993, -34.62501878078303008, 0.000000000000000000 ) ) ;
#12063=ORIENTED_EDGE ( 'NONE', *, *, #24937, .F. ) ;
#12064=CARTESIAN_POINT ( 'NONE',  ( -188.6889827002227094, -47.12918603174894372, 13.84869468767960576 ) ) ;
#12066=CARTESIAN_POINT ( 'NONE',  ( 3.869409319520470625, -24.63759630011287172, 44.61273074174902575 ) ) ;
#12067=CARTESIAN_POINT ( 'NONE',  ( 23.13330272892167727, 17.84165608060106223, -43.07356808498627032 ) ) ;
#12070=CARTESIAN_POINT ( 'NONE',  ( -187.3037411062135504, -13.75782484034011510, 46.64555264107092825 ) ) ;
#12071=CARTESIAN_POINT ( 'NONE',  ( 91.82158438592158234, 44.40256751092319121, 12.16597498400105515 ) ) ;
#12072=CARTESIAN_POINT ( 'NONE',  ( -238.4067589809705794, -0.9644942799826262680, 0.000000000000000000 ) ) ;
#12073=CARTESIAN_POINT ( 'NONE',  ( -188.2507053402893860, 23.43979243030716830, -42.99082124348435485 ) ) ;
#12074=CARTESIAN_POINT ( 'NONE',  ( 57.59792236341147031, -1.722363176415055985, 1.722363176415024677 ) ) ;
#12076=CARTESIAN_POINT ( 'NONE',  ( -86.96347745069645896, 21.75974354311648895, -40.00000000000002132 ) ) ;
#12077=CARTESIAN_POINT ( 'NONE',  ( 184.8905102610680444, 19.07866798485562043, 2.449293598294708485E-15 ) ) ;
#12078=CARTESIAN_POINT ( 'NONE',  ( -198.0356074513804572, 5.461327841961909642E-13, -55.37879056873073580 ) ) ;
#12079=CARTESIAN_POINT ( 'NONE',  ( -105.3755690713226727, 12.89780903124400879, 12.89780903124407452 ) ) ;
#12080=CARTESIAN_POINT ( 'NONE',  ( 200.0000000000000000, -40.00000000000019185, 19.99999999999968381 ) ) ;
#12082=CARTESIAN_POINT ( 'NONE',  ( -91.56559293963836410, 44.31723036834908669, -12.25131212657445801 ) ) ;
#12083=B_SPLINE_CURVE_WITH_KNOTS ( 'NONE', 3,
 ( #2095, #10600, #22455, #18712, #496, #8603 ),
 .UNSPECIFIED., .F., .F.,
 ( 4, 2, 4 ),
 ( -5.998616629415296830E-08, 0.005995031700373161000, 0.01199012338691261489 ),
 .UNSPECIFIED. ) ;
#12084=ORIENTED_EDGE ( 'NONE', *, *, #9630, .F. ) ;
#12085=CARTESIAN_POINT ( 'NONE',  ( 136.1360204305621266, -24.77266263493116583, -24.77266263493127951 ) ) ;
#12090=CARTESIAN_POINT ( 'NONE',  ( 192.4448373802101173, -42.42640687116490028, -14.14213562375904942 ) ) ;
#12091=CARTESIAN_POINT ( 'NONE',  ( 23.25494099740648934, -43.03927110441365755, -17.82744980610230456 ) ) ;
#12093=ORIENTED_EDGE ( 'NONE', *, *, #13669, .F. ) ;
#12094=CARTESIAN_POINT ( 'NONE',  ( 91.82158438592158234, 22.79471317813472453, -40.00000000000002132 ) ) ;
#12098=CARTESIAN_POINT ( 'NONE',  ( 136.1360204305621551, 3.511608612530801032, -53.05693388239316022 ) ) ;
#12099=CARTESIAN_POINT ( 'NONE',  ( -187.7699188114776234, -46.80708926512986778, -13.79076593537901552 ) ) ;
#12100=CARTESIAN_POINT ( 'NONE',  ( 184.8905102610680444, -39.99999999999991473, -20.92133201514458207 ) ) ;
#12101=CARTESIAN_POINT ( 'NONE',  ( -192.9588430854690273, 14.46834944099966336, 40.00000000000002132 ) ) ;
#12104=CARTESIAN_POINT ( 'NONE',  ( 4.995406935893290878, -5.232665749138292703E-14, 15.24977328854832592 ) ) ;
#12105=CARTESIAN_POINT ( 'NONE',  ( 4.995406935893298872, -1.944352046434030652E-13, 55.24977328854835434 ) ) ;
#12106=CARTESIAN_POINT ( 'NONE',  ( 192.4448373802101173, -40.00000000000019185, 20.00000000003900524 ) ) ;
#12107=CARTESIAN_POINT ( 'NONE',  ( -162.0762913951021176, 39.99999999999998579, 1.694272876828463614 ) ) ;
#12108=CARTESIAN_POINT ( 'NONE',  ( -238.4067589809705794, -0.9644942799826262680, 0.000000000000000000 ) ) ;
#12109=CARTESIAN_POINT ( 'NONE',  ( 163.1118516004056573, -37.29075403953139300, -19.27778845539249630 ) ) ;
#12110=CARTESIAN_POINT ( 'NONE',  ( 19.06497207195980792, -14.19242893257839988, -40.00000000000002132 ) ) ;
#12111=CARTESIAN_POINT ( 'NONE',  ( -135.8532207217289738, -50.09629031063965243, -6.472252184284438492 ) ) ;
#12113=B_SPLINE_CURVE_WITH_KNOTS ( 'NONE', 3,
 ( #22075, #26075, #5444, #13677, #13422, #11543 ),
 .UNSPECIFIED., .F., .F.,
 ( 4, 2, 4 ),
 ( 1.430489624538199204E-17, 0.03937634048170810669, 0.07875268096341619950 ),
 .UNSPECIFIED. ) ;
#12115=CARTESIAN_POINT ( 'NONE',  ( -105.3755690713226727, -2.472783935621397949E-13, 21.75974354311649961 ) ) ;
#12116=CARTESIAN_POINT ( 'NONE',  ( 151.7948205124836534, -40.00000000000001421, 6.767089262348889633 ) ) ;
#12117=CARTESIAN_POINT ( 'NONE',  ( 146.6084372240433993, 3.800685668858676980, 3.800685668858667210 ) ) ;
#12118=CARTESIAN_POINT ( 'NONE',  ( -114.6692722883742164, 11.86629262262099083, 18.56554616133607993 ) ) ;
#12119=CARTESIAN_POINT ( 'NONE',  ( -188.2871287166142338, -13.82723289751134743, -46.98614659774170121 ) ) ;
#12120=CARTESIAN_POINT ( 'NONE',  ( -280.0000000000000000, 14.14213562373098299, -14.14213562373088706 ) ) ;
#12121=VERTEX_POINT ( 'NONE', #21200 ) ;
#12122=CARTESIAN_POINT ( 'NONE',  ( 136.1360204305621551, -24.77266263493081766, -31.79587985999290112 ) ) ;
#12124=CARTESIAN_POINT ( 'NONE',  ( 199.9999999999999432, 20.00000000000013856, 0.000000000000000000 ) ) ;
#12125=CARTESIAN_POINT ( 'NONE',  ( 136.1360204305621551, -24.77266263493081766, -31.79587985999290112 ) ) ;
#12126=B_SPLINE_CURVE_WITH_KNOTS ( 'NONE', 3,
 ( #17852, #24257, #6158, #14267, #5893, #14137, #10152, #26002 ),
 .UNSPECIFIED., .F., .F.,
 ( 4, 2, 2, 4 ),
 ( -5.298247996675143094E-05, 0.001923793760056806803, 0.003900570000080365307, 0.007854122480127481015 ),
 .UNSPECIFIED. ) ;
#12127=CARTESIAN_POINT ( 'NONE',  ( -82.26531528649849179, 5.040628272941656718, 19.58553546192279882 ) ) ;
#12129=ORIENTED_EDGE ( 'NONE', *, *, #25739, .T. ) ;
#12133=CARTESIAN_POINT ( 'NONE',  ( -8.197988474478083987, 17.40147972966425627, 42.01088836873465482 ) ) ;
#12136=CARTESIAN_POINT ( 'NONE',  ( 19.06497207195980792, 14.19242893257840876, 0.000000000000000000 ) ) ;
#12138=CARTESIAN_POINT ( 'NONE',  ( -110.0738147261103848, -5.034922404819302422, -19.58739231805851588 ) ) ;
#12140=CARTESIAN_POINT ( 'NONE',  ( 12.01676469546554493, 44.88780742856572203, -24.84032989753405474 ) ) ;
#12141=CARTESIAN_POINT ( 'NONE',  ( -56.48582580120560692, 39.99999999999991473, 9.153146818114004546 ) ) ;
#12143=AXIS2_PLACEMENT_3D ( 'NONE', #437, #6027, #4177 ) ;
#12149=CARTESIAN_POINT ( 'NONE',  ( 3.468680970034179634, -14.11592159092460719, -48.91035688726502428 ) ) ;
#12150=CARTESIAN_POINT ( 'NONE',  ( 14.38125909742182529, -39.01709431150879936, -39.01709431150948859 ) ) ;
#12151=CARTESIAN_POINT ( 'NONE',  ( -110.0738128639248288, 5.035098269363941448, -19.58735130876181785 ) ) ;
#12152=CARTESIAN_POINT ( 'NONE',  ( 4.995406935893297984, -39.06748935135182421, -17.50105314357212549 ) ) ;
#12153=CARTESIAN_POINT ( 'NONE',  ( -162.0762913951020892, -1.202636532414034422E-14, -1.694272876828323948 ) ) ;
#12154=CARTESIAN_POINT ( 'NONE',  ( 4.995406935893293543, -10.78321810388990265, -10.78321810389009272 ) ) ;
#12155=CARTESIAN_POINT ( 'NONE',  ( -280.0000000000000568, 19.99999999999996092, 40.00000000000002132 ) ) ;
#12158=CARTESIAN_POINT ( 'NONE',  ( 163.1118516004056573, -12.73709011382472234, -2.449293598294708485E-15 ) ) ;
#12159=CARTESIAN_POINT ( 'NONE',  ( -114.6701221307682914, 11.88156715851604339, 18.55671387348713353 ) ) ;
#12160=CARTESIAN_POINT ( 'NONE',  ( 200.0000000000000000, 40.00000000000026290, -19.99999999999950617 ) ) ;
#12161=CARTESIAN_POINT ( 'NONE',  ( 170.2234770963711128, 39.20704971665398375, -17.36149277826984871 ) ) ;
#12162=CARTESIAN_POINT ( 'NONE',  ( 136.1360204305621266, -35.03383547441293899, 0.000000000000000000 ) ) ;
#12164=EDGE_CURVE ( 'NONE', #525, #10974, #5706, .T. ) ;
#12165=VERTEX_POINT ( 'NONE', #20807 ) ;
#12166=CARTESIAN_POINT ( 'NONE',  ( 184.8905102610680444, -20.92133201514440799, 40.00000000000002132 ) ) ;
#12170=CARTESIAN_POINT ( 'NONE',  ( 151.7948205124836534, -39.99999999999987921, -33.23291073765567916 ) ) ;
#12171=CARTESIAN_POINT ( 'NONE',  ( 170.2234770963711128, 39.20704971665372796, 17.36149277827039583 ) ) ;
#12172=CARTESIAN_POINT ( 'NONE',  ( 184.8905102610680444, -20.92133201514440799, 0.000000000000000000 ) ) ;
#12174=CARTESIAN_POINT ( 'NONE',  ( -87.02146317964809441, 5.408180612257909914, -20.76663852858110815 ) ) ;
#12177=CARTESIAN_POINT ( 'NONE',  ( 199.9999999999999432, 14.14213562373110911, -14.14213562373072364 ) ) ;
#12178=CARTESIAN_POINT ( 'NONE',  ( -198.0356074513804572, -39.15871834505931304, 17.40982414986437377 ) ) ;
#12179=CARTESIAN_POINT ( 'NONE',  ( -105.3073921447119261, 20.83275309902035843, 5.041689060256491217 ) ) ;
#12180=CARTESIAN_POINT ( 'NONE',  ( -82.29192131161018153, 18.26745044306171550, -8.580784324595091661 ) ) ;
#12181=CARTESIAN_POINT ( 'NONE',  ( 199.9999999999999432, -14.14213562373073607, -14.14213562373102206 ) ) ;
#12182=CARTESIAN_POINT ( 'NONE',  ( 136.1360204305621266, -24.77266263493151044, 24.77266263493093135 ) ) ;
#12183=CARTESIAN_POINT ( 'NONE',  ( 14.38125909742180752, 10.73282306404720465, 10.73282306404724018 ) ) ;
#12184=CARTESIAN_POINT ( 'NONE',  ( -86.96347745069645896, -12.89780903124382938, -43.67073346367985920 ) ) ;
#12187=CARTESIAN_POINT ( 'NONE',  ( -213.1075012329537230, 39.99999999999979394, 53.71589010950180665 ) ) ;
#12189=CARTESIAN_POINT ( 'NONE',  ( 22.89778847645106907, 43.13990468001224343, -17.86913359794376532 ) ) ;
#12190=CARTESIAN_POINT ( 'NONE',  ( -238.4067589809705794, 0.9644942799825385604, -40.00000000000002132 ) ) ;
#12191=ORIENTED_EDGE ( 'NONE', *, *, #6239, .F. ) ;
#12192=CARTESIAN_POINT ( 'NONE',  ( 0.4289717129526320338, -24.25042218720239262, -44.08776571100859343 ) ) ;
#12194=CARTESIAN_POINT ( 'NONE',  ( -8.720657192108198785, -45.36528685022982899, 13.49580954686996925 ) ) ;
#12195=CARTESIAN_POINT ( 'NONE',  ( -162.0762913951021176, 1.694272876828294194, 40.00000000000002132 ) ) ;
#12196=ORIENTED_EDGE ( 'NONE', *, *, #3372, .F. ) ;
#12197=CARTESIAN_POINT ( 'NONE',  ( 21.15138808362603839, 23.80076113581877806, -43.47948264999411805 ) ) ;
#12199=CARTESIAN_POINT ( 'NONE',  ( 4.155455573144507753, -18.49472242009463230, 44.65020969902027304 ) ) ;
#12201=CARTESIAN_POINT ( 'NONE',  ( 20.38198589867913668, 18.12553405621813596, -43.75891014376608013 ) ) ;
#12203=CARTESIAN_POINT ( 'NONE',  ( 19.06497207195981147, 1.521599808664285085E-13, -14.19242893257840521 ) ) ;
#12204=CARTESIAN_POINT ( 'NONE',  ( 156.1979191798868385, -27.38417834433187892, 11.34289806466571982 ) ) ;
#12205=CARTESIAN_POINT ( 'NONE',  ( 170.2234770963711128, 1.169953928977015745E-13, -24.55285855007187124 ) ) ;
#12206=CARTESIAN_POINT ( 'NONE',  ( -135.8532207217289738, 50.09629031063956006, 6.472252184284782217 ) ) ;
#12207=CARTESIAN_POINT ( 'NONE',  ( -105.2054292635175869, 15.19799821370233062, -15.19799821370219206 ) ) ;
#12208=CARTESIAN_POINT ( 'NONE',  ( -188.2652746676487254, 23.44263257803753575, -42.99511404081827948 ) ) ;
#12209=CARTESIAN_POINT ( 'NONE',  ( -100.7734535825088500, 12.25131212657428748, 44.31723036834913643 ) ) ;
#12210=CARTESIAN_POINT ( 'NONE',  ( 136.1360204305621551, -4.966164525587036138, -40.00000000000002132 ) ) ;
#12211=CARTESIAN_POINT ( 'NONE',  ( -86.96347745069644475, 18.24025645688350750, 40.00000000000002132 ) ) ;
#12212=CARTESIAN_POINT ( 'NONE',  ( -135.8532207217289738, 3.005970985514575011E-13, -30.84685318188645553 ) ) ;
#12213=CARTESIAN_POINT ( 'NONE',  ( -30.26275506840325136, 57.76657404653985139, 1.198031551616126178 ) ) ;
#12214=CARTESIAN_POINT ( 'NONE',  ( -102.4309680865773373, 20.17061239842026765, -8.733065089982426699 ) ) ;
#12215=CARTESIAN_POINT ( 'NONE',  ( 163.1118516004056573, -9.006482792069506971, -9.006482792069697041 ) ) ;
#12216=VERTEX_POINT ( 'NONE', #10692 ) ;
#12217=CARTESIAN_POINT ( 'NONE',  ( 199.9999999999999432, -14.14213562373096345, -14.14213562373104871 ) ) ;
#12218=CARTESIAN_POINT ( 'NONE',  ( -102.4309680865808616, 8.087567261658067608, 20.43798635340267111 ) ) ;
#12220=ORIENTED_EDGE ( 'NONE', *, *, #11815, .F. ) ;
#12221=VERTEX_POINT ( 'NONE', #8691 ) ;
#12222=CARTESIAN_POINT ( 'NONE',  ( -100.7734535825088500, -12.25131212657462498, -44.31723036834905827 ) ) ;
#12223=CARTESIAN_POINT ( 'NONE',  ( 23.36927571439211704, -42.85861222363623568, -23.34061495561072519 ) ) ;
#12224=ORIENTED_EDGE ( 'NONE', *, *, #2653, .F. ) ;
#12225=CARTESIAN_POINT ( 'NONE',  ( -56.48582580120559982, -9.153146818113595984, -40.00000000000002132 ) ) ;
#12226=CARTESIAN_POINT ( 'NONE',  ( -83.21262154144231715, 13.72187187063211233, 33.12752917117668972 ) ) ;
#12227=ORIENTED_EDGE ( 'NONE', *, *, #16108, .F. ) ;
#12229=FACE_OUTER_BOUND ( 'NONE', #6958, .T. ) ;
#12230=CARTESIAN_POINT ( 'NONE',  ( -198.0356074513804572, 39.15871834505912119, -17.40982414986464377 ) ) ;
#12231=CARTESIAN_POINT ( 'NONE',  ( -188.3066136396865318, -43.00728998844432738, -23.45085387054221115 ) ) ;
#12233=CARTESIAN_POINT ( 'NONE',  ( -259.2033419157646676, -40.00000000000017764, 30.48217210827725054 ) ) ;
#12234=CARTESIAN_POINT ( 'NONE',  ( -208.1127848780264742, 55.00245453014418473, 40.00000000000002132 ) ) ;
#12238=CARTESIAN_POINT ( 'NONE',  ( 130.8568914410475088, -39.99999999999988631, -34.05028731879802706 ) ) ;
#12239=CARTESIAN_POINT ( 'NONE',  ( 163.1118516004056573, -39.99999999999990052, -27.26290988616886679 ) ) ;
#12240=CARTESIAN_POINT ( 'NONE',  ( -100.7734535825088358, 6.065416334915073333E-14, -22.67402823373191723 ) ) ;
#12241=CARTESIAN_POINT ( 'NONE',  ( -162.0762913951020892, -1.694272876828353702, 0.000000000000000000 ) ) ;
#12242=CARTESIAN_POINT ( 'NONE',  ( -198.0356074513804572, -10.87444709760996986, 67.44298959253333692 ) ) ;
#12244=CARTESIAN_POINT ( 'NONE',  ( 192.4448373802101173, 20.00000000003945644, -40.00000000000002132 ) ) ;
#12246=CARTESIAN_POINT ( 'NONE',  ( -86.96347745069644475, -12.89780903124413491, 12.89780903124398037 ) ) ;
#12249=CARTESIAN_POINT ( 'NONE',  ( 4.995406935893283773, 40.00000000000017764, -15.24977328854790848 ) ) ;
#12250=CARTESIAN_POINT ( 'NONE',  ( -162.0762913951020892, -1.777970010055771463E-13, 41.69427287682835015 ) ) ;
#12251=CARTESIAN_POINT ( 'NONE',  ( -135.8532207217289738, 50.09629031063965243, -6.472252184284084109 ) ) ;
#12252=CARTESIAN_POINT ( 'NONE',  ( 19.06497207195981147, -10.03556273973425483, -10.03556273973443247 ) ) ;
#12253=CARTESIAN_POINT ( 'NONE',  ( -188.2957210513887674, -23.44847782072339371, -43.00408675155699001 ) ) ;
#12254=CARTESIAN_POINT ( 'NONE',  ( -208.1127848780265026, -10.60833733269551971, 10.60833733269537049 ) ) ;
#12256=CARTESIAN_POINT ( 'NONE',  ( -105.3755690713226585, -43.67073346367964604, -12.89780903124457545 ) ) ;
#12258=CARTESIAN_POINT ( 'NONE',  ( -238.4067589809705794, -0.9644942799826262680, 0.000000000000000000 ) ) ;
#12259=CARTESIAN_POINT ( 'NONE',  ( 19.06497207195980792, -18.24870850772710540, -38.31983398719647482 ) ) ;
#12261=VERTEX_POINT ( 'NONE', #9209 ) ;
#12264=CARTESIAN_POINT ( 'NONE',  ( 20.59039453120230334, -23.90179120638647703, 43.61606461192731388 ) ) ;
#12265=CARTESIAN_POINT ( 'NONE',  ( 3.468680970031514210, 24.60338114559333889, 44.56630890487709706 ) ) ;
#12267=VERTEX_POINT ( 'NONE', #17443 ) ;
#12268=CARTESIAN_POINT ( 'NONE',  ( 163.1118516004056573, -27.26290988616869626, -40.00000000000002132 ) ) ;
#12270=CARTESIAN_POINT ( 'NONE',  ( -105.4741150117381636, -7.943527260753955765, -19.77569912954965758 ) ) ;
#12271=CARTESIAN_POINT ( 'NONE',  ( 0.2972598230769938343, 10.13633138497472252, 10.13633138497475628 ) ) ;
#12272=CARTESIAN_POINT ( 'NONE',  ( 0.4289717129525671413, 44.08776571100865027, -24.25042218720249920 ) ) ;
#12273=CARTESIAN_POINT ( 'NONE',  ( -280.0000000000000000, 1.605030083646939673E-13, -20.00000000000001421 ) ) ;
#12275=( BOUNDED_SURFACE ( )  B_SPLINE_SURFACE ( 3, 3, ( 
 ( #19894, #22172, #3946, #5658, #12043, #20163, #9784, #18159, #26305, #17756, #24299, #6067, #10185, #4079, #19757, #20301, #2078, #75, #5529, #13635, #1546, #7638, #4741, #22438, #16834, #16695, #14829, #8446, #14566, #10450 ),
 ( #14304, #2211, #16565, #12437, #10320, #24425, #8717, #748, #18563, #24695, #24828, #6191, #6581, #2336, #18427, #6715, #18830, #6317, #204, #14700, #22961, #24968, #6450, #22832, #20833, #24562, #22696, #4609, #20964, #8852 ),
 ( #12705, #4215, #2608, #342, #8313, #12848, #610, #14437, #16436, #10721, #2745, #10849, #4471, #18968, #12305, #20432, #12570, #18695, #20703, #22566, #4345, #20565, #2469, #10579, #479, #8584, #1258, #3377, #14966, #21099 ),
 ( #9242, #11109, #1005, #17472, #2879, #17349, #10987, #13483, #25485, #15354, #19225, #19096, #17093, #8989, #16962, #7234, #877, #5004, #23599, #12976, #3251, #25225, #6978, #23354, #15092, #23101, #7359, #23226, #25614, #23478 ),
 ( #11355, #25357, #1138, #5250, #13354, #15470, #9108, #5378, #11476, #5131, #6849, #13109, #19471, #21476, #9362, #1390, #4872, #21230, #21604, #7112, #15223, #19604, #3003, #17218, #13236, #21359, #3128, #11231, #19349, #25100 ),
 ( #1519, #13875, #12020, #5504, #15728, #9759, #20276, #13605, #3640, #14011, #3778, #5903, #22008, #11881, #20001, #1918, #20140, #25869, #26010, #11747, #7746, #22278, #7487, #25735, #21734, #1650, #26282, #19865, #15858, #21864 ),
 ( #15598, #3510, #17859, #23853, #11610, #9491, #10023, #12153, #23987, #5766, #1787, #17596, #9891, #13738, #19732, #18133, #3921, #17729, #9625, #17994, #8021, #16137, #26140, #7884, #22140, #23723, #16005, #24131, #24267, #6041 ) ),
 .UNSPECIFIED., .T., .F., .F. ) 
 B_SPLINE_SURFACE_WITH_KNOTS ( ( 4, 3, 4 ),
 ( 4, 2, 2, 2, 2, 2, 2, 2, 2, 2, 2, 2, 2, 2, 4 ),
 ( 0.000000000000000000, 0.5000000000000000000, 1.000000000000000000 ),
 ( 0.000000000000000000, 0.1357259735107005372, 0.1651108541090157700, 0.1944957347073310028, 0.3598804999793158710, 0.3867117631979620773, 0.4135430264166082281, 0.5789277916885930964, 0.6062785021374117456, 0.6336292125862302838, 0.8508620842112317728, 0.8814014469398914198, 0.9119408096685510667, 0.9559704048342755334, 1.000000000000000000 ),
 .UNSPECIFIED. ) 
 GEOMETRIC_REPRESENTATION_ITEM ( )  RATIONAL_B_SPLINE_SURFACE ( (
 ( 1.000000000000000000, 1.000000000000000000, 1.000000000000000000, 1.000000000000000000, 1.000000000000000000, 1.000000000000000000, 1.000000000000000000, 1.000000000000000000, 1.000000000000000000, 1.000000000000000000, 1.000000000000000000, 1.000000000000000000, 1.000000000000000000, 1.000000000000000000, 1.000000000000000000, 1.000000000000000000, 1.000000000000000000, 1.000000000000000000, 1.000000000000000000, 1.000000000000000000, 1.000000000000000000, 1.000000000000000000, 1.000000000000000000, 1.000000000000000000, 1.000000000000000000, 1.000000000000000000, 1.000000000000000000, 1.000000000000000000, 1.000000000000000000, 1.000000000000000000),
 ( 0.3333333333333333703, 0.3333333333333333703, 0.3333333333333333703, 0.3333333333333333703, 0.3333333333333333703, 0.3333333333333333703, 0.3333333333333333703, 0.3333333333333333703, 0.3333333333333333703, 0.3333333333333333703, 0.3333333333333333703, 0.3333333333333333703, 0.3333333333333333703, 0.3333333333333333703, 0.3333333333333333703, 0.3333333333333333703, 0.3333333333333333703, 0.3333333333333333703, 0.3333333333333333703, 0.3333333333333333703, 0.3333333333333333703, 0.3333333333333333703, 0.3333333333333333703, 0.3333333333333333703, 0.3333333333333333703, 0.3333333333333333703, 0.3333333333333333703, 0.3333333333333333703, 0.3333333333333333703, 0.3333333333333333703),
 ( 0.3333333333333333703, 0.3333333333333333703, 0.3333333333333333703, 0.3333333333333333703, 0.3333333333333333703, 0.3333333333333333703, 0.3333333333333333703, 0.3333333333333333703, 0.3333333333333333703, 0.3333333333333333703, 0.3333333333333333703, 0.3333333333333333703, 0.3333333333333333703, 0.3333333333333333703, 0.3333333333333333703, 0.3333333333333333703, 0.3333333333333333703, 0.3333333333333333703, 0.3333333333333333703, 0.3333333333333333703, 0.3333333333333333703, 0.3333333333333333703, 0.3333333333333333703, 0.3333333333333333703, 0.3333333333333333703, 0.3333333333333333703, 0.3333333333333333703, 0.3333333333333333703, 0.3333333333333333703, 0.3333333333333333703),
 ( 1.000000000000000000, 1.000000000000000000, 1.000000000000000000, 1.000000000000000000, 1.000000000000000000, 1.000000000000000000, 1.000000000000000000, 1.000000000000000000, 1.000000000000000000, 1.000000000000000000, 1.000000000000000000, 1.000000000000000000, 1.000000000000000000, 1.000000000000000000, 1.000000000000000000, 1.000000000000000000, 1.000000000000000000, 1.000000000000000000, 1.000000000000000000, 1.000000000000000000, 1.000000000000000000, 1.000000000000000000, 1.000000000000000000, 1.000000000000000000, 1.000000000000000000, 1.000000000000000000, 1.000000000000000000, 1.000000000000000000, 1.000000000000000000, 1.000000000000000000),
 ( 0.3333333333333333703, 0.3333333333333333703, 0.3333333333333333703, 0.3333333333333333703, 0.3333333333333333703, 0.3333333333333333703, 0.3333333333333333703, 0.3333333333333333703, 0.3333333333333333703, 0.3333333333333333703, 0.3333333333333333703, 0.3333333333333333703, 0.3333333333333333703, 0.3333333333333333703, 0.3333333333333333703, 0.3333333333333333703, 0.3333333333333333703, 0.3333333333333333703, 0.3333333333333333703, 0.3333333333333333703, 0.3333333333333333703, 0.3333333333333333703, 0.3333333333333333703, 0.3333333333333333703, 0.3333333333333333703, 0.3333333333333333703, 0.3333333333333333703, 0.3333333333333333703, 0.3333333333333333703, 0.3333333333333333703),
 ( 0.3333333333333333703, 0.3333333333333333703, 0.3333333333333333703, 0.3333333333333333703, 0.3333333333333333703, 0.3333333333333333703, 0.3333333333333333703, 0.3333333333333333703, 0.3333333333333333703, 0.3333333333333333703, 0.3333333333333333703, 0.3333333333333333703, 0.3333333333333333703, 0.3333333333333333703, 0.3333333333333333703, 0.3333333333333333703, 0.3333333333333333703, 0.3333333333333333703, 0.3333333333333333703, 0.3333333333333333703, 0.3333333333333333703, 0.3333333333333333703, 0.3333333333333333703, 0.3333333333333333703, 0.3333333333333333703, 0.3333333333333333703, 0.3333333333333333703, 0.3333333333333333703, 0.3333333333333333703, 0.3333333333333333703),
 ( 1.000000000000000000, 1.000000000000000000, 1.000000000000000000, 1.000000000000000000, 1.000000000000000000, 1.000000000000000000, 1.000000000000000000, 1.000000000000000000, 1.000000000000000000, 1.000000000000000000, 1.000000000000000000, 1.000000000000000000, 1.000000000000000000, 1.000000000000000000, 1.000000000000000000, 1.000000000000000000, 1.000000000000000000, 1.000000000000000000, 1.000000000000000000, 1.000000000000000000, 1.000000000000000000, 1.000000000000000000, 1.000000000000000000, 1.000000000000000000, 1.000000000000000000, 1.000000000000000000, 1.000000000000000000, 1.000000000000000000, 1.000000000000000000, 1.000000000000000000) ) ) 
 REPRESENTATION_ITEM ( '' )  SURFACE ( )  );
#12279=CARTESIAN_POINT ( 'NONE',  ( -114.4098922876147384, 20.15198150140922451, 8.347224046571190215 ) ) ;
#12280=CARTESIAN_POINT ( 'NONE',  ( -1.087763065926164341, -24.03018639663240918, -43.78960619332526960 ) ) ;
#12281=CARTESIAN_POINT ( 'NONE',  ( 19.06497207195982568, -38.31983398719592770, -38.31983398719660272 ) ) ;
#12282=CARTESIAN_POINT ( 'NONE',  ( -114.4364955367319396, 8.064892380839246755, -20.29001642038913644 ) ) ;
#12283=CARTESIAN_POINT ( 'NONE',  ( 163.1118516004056573, -9.006482792073960297, -47.56205970284963769 ) ) ;
#12284=CARTESIAN_POINT ( 'NONE',  ( 184.8905102610680444, 20.92133201514447549, 0.000000000000000000 ) ) ;
#12285=CARTESIAN_POINT ( 'NONE',  ( -105.3755690713226727, -18.24025645688354302, -2.449293598294708485E-15 ) ) ;
#12286=CARTESIAN_POINT ( 'NONE',  ( 130.8568914410475372, 24.07718906447243867, -24.07718906447216156 ) ) ;
#12287=CARTESIAN_POINT ( 'NONE',  ( 4.995406935893309530, -55.24977328856464709, 40.00000000000002132 ) ) ;
#12288=CARTESIAN_POINT ( 'NONE',  ( -100.0753760173604405, 20.72827493166397161, -8.149786832858799457 ) ) ;
#12289=CARTESIAN_POINT ( 'NONE',  ( -105.3755690713226585, 39.99999999999977263, 21.75974354311691883 ) ) ;
#12290=CARTESIAN_POINT ( 'NONE',  ( -162.0762913951021176, 29.48230308784768638, -27.08623940707612121 ) ) ;
#12291=CARTESIAN_POINT ( 'NONE',  ( 184.8905102610680444, -20.92133201514440799, -40.00000000000002132 ) ) ;
#12295=CARTESIAN_POINT ( 'NONE',  ( -93.02511667906878756, -8.169918093965518935, -20.82219708225685295 ) ) ;
#12296=CARTESIAN_POINT ( 'NONE',  ( 184.8905102610680444, 41.77492675555983936, 14.79361573936436081 ) ) ;
#12302=CARTESIAN_POINT ( 'NONE',  ( 192.4448373802100889, 14.14213562370330379, -14.14213562370292365 ) ) ;
#12303=CARTESIAN_POINT ( 'NONE',  ( -30.26275506840324070, -29.48230279907817675, 27.08623969584564151 ) ) ;
#12304=CARTESIAN_POINT ( 'NONE',  ( -110.0763310915540529, 19.64189236472208933, 4.694460244226943857 ) ) ;
#12305=CARTESIAN_POINT ( 'NONE',  ( -30.26275506840324425, 40.00000000000044764, -41.69427246844585255 ) ) ;
#12306=CARTESIAN_POINT ( 'NONE',  ( -86.96347745069643054, -41.18208027870611687, 15.38646221621750954 ) ) ;
#12309=CARTESIAN_POINT ( 'NONE',  ( -100.7734535825088500, -44.31723036834903695, 12.25131212657476709 ) ) ;
#12310=CARTESIAN_POINT ( 'NONE',  ( 184.8905102610680444, -13.49065550809780412, -43.07788698682583828 ) ) ;
#12314=CARTESIAN_POINT ( 'NONE',  ( -100.7734535825088358, -8.145438380286941744E-14, 17.32597176626811120 ) ) ;
#12316=CARTESIAN_POINT ( 'NONE',  ( 23.49666234703815704, 42.81942870555077008, -23.31470603676260467 ) ) ;
#12317=CARTESIAN_POINT ( 'NONE',  ( 151.7948205124836250, 6.767089262349059275, 2.449293598294708485E-15 ) ) ;
#12318=CARTESIAN_POINT ( 'NONE',  ( -30.26275506840324070, 1.694272468446254232, 0.000000000000000000 ) ) ;
#12319=( BOUNDED_SURFACE ( )  B_SPLINE_SURFACE ( 3, 3, ( 
 ( #25894, #5273, #23878, #11134, #17618, #15493, #9129, #23623, #17244, #3401, #1280, #25636, #9388, #3530, #1543, #11254, #5403, #15621, #3277, #5525, #11375, #19627, #15750, #17495, #25382, #7134, #5655, #13378, #13760, #19249 ),
 ( #15376, #23499, #21887, #21505, #13503, #19496, #1160, #1412, #21625, #9648, #15247, #9513, #25763, #7513, #23744, #23378, #9264, #13632, #5153, #21757, #11631, #19753, #13258, #21381, #7258, #3153, #19373, #17371, #14434, #16433 ),
 ( #19891, #10049, #11908, #15884, #20429, #1809, #3943, #17883, #14301, #24559, #1676, #7769, #18423, #6314, #22299, #10182, #9912, #16026, #1941, #18018, #72, #24010, #201, #26167, #18286, #16298, #9781, #8309, #18155, #24422 ),
 ( #14035, #6187, #2208, #22031, #20031, #26302, #3664, #22435, #26032, #7907, #5790, #20160, #13898, #24151, #3804, #8181, #11772, #10317, #4212, #5928, #22169, #12040, #8045, #16161, #24296, #6064, #14166, #4075, #12302, #12177 ),
 ( #20298, #2075, #18560, #25097, #14963, #12434, #339, #8443, #8984, #12973, #2466, #20830, #16562, #24825, #17090, #745, #8849, #16830, #16959, #25222, #4606, #4737, #20700, #6975, #21096, #22693, #10984, #16692, #22563, #22829 ),
 ( #2605, #24692, #6578, #4342, #6845, #23098, #24965, #12702, #6447, #607, #20961, #10576, #19094, #874, #4869, #14563, #2876, #4469, #2742, #12566, #8714, #10846, #476, #8581, #20562, #14697, #6712, #10718, #18691, #12845 ),
 ( #18827, #14826, #22958, #2333, #18965, #10447, #13106, #25611, #25866, #3507, #9239, #15595, #23720, #21227, #19222, #5001, #17469, #7231, #23596, #23351, #17346, #17725, #21473, #3248, #2999, #19346, #1002, #15089, #13234, #23475 ) ),
 .UNSPECIFIED., .T., .F., .F. ) 
 B_SPLINE_SURFACE_WITH_KNOTS ( ( 4, 3, 4 ),
 ( 4, 2, 2, 2, 2, 2, 2, 2, 2, 2, 2, 2, 2, 2, 4 ),
 ( 0.000000000000000000, 0.5000000000000000000, 1.000000000000000000 ),
 ( 0.000000000000000000, 0.1357259735107005372, 0.1651108541090157700, 0.1944957347073310028, 0.3598804999793158710, 0.3867117631979620773, 0.4135430264166082281, 0.5789277916885930964, 0.6062785021374117456, 0.6336292125862302838, 0.8508620842112317728, 0.8814014469398914198, 0.9119408096685510667, 0.9559704048342755334, 1.000000000000000000 ),
 .UNSPECIFIED. ) 
 GEOMETRIC_REPRESENTATION_ITEM ( )  RATIONAL_B_SPLINE_SURFACE ( (
 ( 1.000000000000000000, 1.000000000000000000, 1.000000000000000000, 1.000000000000000000, 1.000000000000000000, 1.000000000000000000, 1.000000000000000000, 1.000000000000000000, 1.000000000000000000, 1.000000000000000000, 1.000000000000000000, 1.000000000000000000, 1.000000000000000000, 1.000000000000000000, 1.000000000000000000, 1.000000000000000000, 1.000000000000000000, 1.000000000000000000, 1.000000000000000000, 1.000000000000000000, 1.000000000000000000, 1.000000000000000000, 1.000000000000000000, 1.000000000000000000, 1.000000000000000000, 1.000000000000000000, 1.000000000000000000, 1.000000000000000000, 1.000000000000000000, 1.000000000000000000),
 ( 0.3333333333333333703, 0.3333333333333333703, 0.3333333333333333703, 0.3333333333333333703, 0.3333333333333333703, 0.3333333333333333703, 0.3333333333333333703, 0.3333333333333333703, 0.3333333333333333703, 0.3333333333333333703, 0.3333333333333333703, 0.3333333333333333703, 0.3333333333333333703, 0.3333333333333333703, 0.3333333333333333703, 0.3333333333333333703, 0.3333333333333333703, 0.3333333333333333703, 0.3333333333333333703, 0.3333333333333333703, 0.3333333333333333703, 0.3333333333333333703, 0.3333333333333333703, 0.3333333333333333703, 0.3333333333333333703, 0.3333333333333333703, 0.3333333333333333703, 0.3333333333333333703, 0.3333333333333333703, 0.3333333333333333703),
 ( 0.3333333333333333703, 0.3333333333333333703, 0.3333333333333333703, 0.3333333333333333703, 0.3333333333333333703, 0.3333333333333333703, 0.3333333333333333703, 0.3333333333333333703, 0.3333333333333333703, 0.3333333333333333703, 0.3333333333333333703, 0.3333333333333333703, 0.3333333333333333703, 0.3333333333333333703, 0.3333333333333333703, 0.3333333333333333703, 0.3333333333333333703, 0.3333333333333333703, 0.3333333333333333703, 0.3333333333333333703, 0.3333333333333333703, 0.3333333333333333703, 0.3333333333333333703, 0.3333333333333333703, 0.3333333333333333703, 0.3333333333333333703, 0.3333333333333333703, 0.3333333333333333703, 0.3333333333333333703, 0.3333333333333333703),
 ( 1.000000000000000000, 1.000000000000000000, 1.000000000000000000, 1.000000000000000000, 1.000000000000000000, 1.000000000000000000, 1.000000000000000000, 1.000000000000000000, 1.000000000000000000, 1.000000000000000000, 1.000000000000000000, 1.000000000000000000, 1.000000000000000000, 1.000000000000000000, 1.000000000000000000, 1.000000000000000000, 1.000000000000000000, 1.000000000000000000, 1.000000000000000000, 1.000000000000000000, 1.000000000000000000, 1.000000000000000000, 1.000000000000000000, 1.000000000000000000, 1.000000000000000000, 1.000000000000000000, 1.000000000000000000, 1.000000000000000000, 1.000000000000000000, 1.000000000000000000),
 ( 0.3333333333333333703, 0.3333333333333333703, 0.3333333333333333703, 0.3333333333333333703, 0.3333333333333333703, 0.3333333333333333703, 0.3333333333333333703, 0.3333333333333333703, 0.3333333333333333703, 0.3333333333333333703, 0.3333333333333333703, 0.3333333333333333703, 0.3333333333333333703, 0.3333333333333333703, 0.3333333333333333703, 0.3333333333333333703, 0.3333333333333333703, 0.3333333333333333703, 0.3333333333333333703, 0.3333333333333333703, 0.3333333333333333703, 0.3333333333333333703, 0.3333333333333333703, 0.3333333333333333703, 0.3333333333333333703, 0.3333333333333333703, 0.3333333333333333703, 0.3333333333333333703, 0.3333333333333333703, 0.3333333333333333703),
 ( 0.3333333333333333703, 0.3333333333333333703, 0.3333333333333333703, 0.3333333333333333703, 0.3333333333333333703, 0.3333333333333333703, 0.3333333333333333703, 0.3333333333333333703, 0.3333333333333333703, 0.3333333333333333703, 0.3333333333333333703, 0.3333333333333333703, 0.3333333333333333703, 0.3333333333333333703, 0.3333333333333333703, 0.3333333333333333703, 0.3333333333333333703, 0.3333333333333333703, 0.3333333333333333703, 0.3333333333333333703, 0.3333333333333333703, 0.3333333333333333703, 0.3333333333333333703, 0.3333333333333333703, 0.3333333333333333703, 0.3333333333333333703, 0.3333333333333333703, 0.3333333333333333703, 0.3333333333333333703, 0.3333333333333333703),
 ( 1.000000000000000000, 1.000000000000000000, 1.000000000000000000, 1.000000000000000000, 1.000000000000000000, 1.000000000000000000, 1.000000000000000000, 1.000000000000000000, 1.000000000000000000, 1.000000000000000000, 1.000000000000000000, 1.000000000000000000, 1.000000000000000000, 1.000000000000000000, 1.000000000000000000, 1.000000000000000000, 1.000000000000000000, 1.000000000000000000, 1.000000000000000000, 1.000000000000000000, 1.000000000000000000, 1.000000000000000000, 1.000000000000000000, 1.000000000000000000, 1.000000000000000000, 1.000000000000000000, 1.000000000000000000, 1.000000000000000000, 1.000000000000000000, 1.000000000000000000) ) ) 
 REPRESENTATION_ITEM ( '' )  SURFACE ( )  );
#12320=CARTESIAN_POINT ( 'NONE',  ( -5.866564133084711585, -42.46617576965135044, 23.09290806363820892 ) ) ;
#12321=CARTESIAN_POINT ( 'NONE',  ( -91.56559293963834989, 17.32597176626809343, 2.449293598294708485E-15 ) ) ;
#12323=CARTESIAN_POINT ( 'NONE',  ( 1.564570055219367761, 24.39611894128515956, -44.28524390194891680 ) ) ;
#12324=CARTESIAN_POINT ( 'NONE',  ( 19.06497207195980792, -18.24870850772763475, 38.31983398719622613 ) ) ;
#12325=CARTESIAN_POINT ( 'NONE',  ( -24.53392603772963554, -19.42583462381907822, 36.88304647106062362 ) ) ;
#12326=EDGE_CURVE ( 'NONE', #15177, #4560, #18388, .T. ) ;
#12328=CARTESIAN_POINT ( 'NONE',  ( -3.966425590329084372, 23.46521855348175478, -43.02666064534172818 ) ) ;
#12331=CARTESIAN_POINT ( 'NONE',  ( 98.29820294269173075, 19.99999999998819433, -2.308575297063409524E-13 ) ) ;
#12332=CARTESIAN_POINT ( 'NONE',  ( -173.7925586253262793, -12.78856870757000763, 41.93433064647447139 ) ) ;
#12333=CARTESIAN_POINT ( 'NONE',  ( -192.9588430854690273, 10.23066800229588758, -66.79921049721882298 ) ) ;
#12334=CARTESIAN_POINT ( 'NONE',  ( 4.995406935893293543, -15.24977328854832592, 0.000000000000000000 ) ) ;
#12335=CARTESIAN_POINT ( 'NONE',  ( -190.7346372395231811, 23.92885340723965726, -43.65255821759343036 ) ) ;
#12336=CARTESIAN_POINT ( 'NONE',  ( -259.2033419157646676, 21.55415060305790931, 35.01439189186571355 ) ) ;
#12337=CARTESIAN_POINT ( 'NONE',  ( -238.4067589809705794, 28.96627169325285678, 27.60227080167094726 ) ) ;
#12338=CARTESIAN_POINT ( 'NONE',  ( -30.26275506840323004, -41.69427246844629309, 40.00000000000002132 ) ) ;
#12339=CARTESIAN_POINT ( 'NONE',  ( -56.48582580120559982, 30.84685318188643421, 40.00000000000002132 ) ) ;
#12340=CARTESIAN_POINT ( 'NONE',  ( -56.48582580120559271, -1.062504017861011783E-13, 9.153146818113587102 ) ) ;
#12341=CARTESIAN_POINT ( 'NONE',  ( 57.59792236341147031, 26.56190807104684382, 26.56190807104692553 ) ) ;
#12342=CARTESIAN_POINT ( 'NONE',  ( -103.9650464695150021, 20.03380587595252393, -8.298274099110376056 ) ) ;
#12343=CARTESIAN_POINT ( 'NONE',  ( 200.0000000000000000, 42.42640687119310172, -14.14213562373052646 ) ) ;
#12344=ORIENTED_EDGE ( 'NONE', *, *, #3474, .T. ) ;
#12345=CARTESIAN_POINT ( 'NONE',  ( 19.06497207195980792, -18.24870850772763475, 38.31983398719622613 ) ) ;
#12346=CARTESIAN_POINT ( 'NONE',  ( -105.4741150117389026, 7.943527260749601027, 19.77569912955131315 ) ) ;
#12348=CARTESIAN_POINT ( 'NONE',  ( 14.38125909742183062, -67.30136555898262429, 10.73282306405838682 ) ) ;
#12349=CARTESIAN_POINT ( 'NONE',  ( 6.202588567992542323, -44.80189419270367779, -24.77700748805923681 ) ) ;
#12351=CARTESIAN_POINT ( 'NONE',  ( 22.27434459959404478, -47.22399357554351695, -13.86259002508720073 ) ) ;
#12352=CARTESIAN_POINT ( 'NONE',  ( -87.13361725306405958, -14.23663034390084725, -16.15936608143848474 ) ) ;
#12355=CARTESIAN_POINT ( 'NONE',  ( -105.2054292635175585, 21.49321519473984665, 5.610018989487960791E-28 ) ) ;
#12356=CARTESIAN_POINT ( 'NONE',  ( 136.1360204305621266, -24.77266263493116583, -24.77266263493127951 ) ) ;
#12357=CARTESIAN_POINT ( 'NONE',  ( -173.7925586252841015, -38.69493321942316300, -20.60916591006939669 ) ) ;
#12358=CARTESIAN_POINT ( 'NONE',  ( -91.56559293963834989, -40.00000000000009948, 17.32597176626796553 ) ) ;
#12359=CARTESIAN_POINT ( 'NONE',  ( -238.4067589809705794, 40.96449427990177128, 40.00000000000002132 ) ) ;
#12364=CARTESIAN_POINT ( 'NONE',  ( 14.38125909742181108, -5.035366881890652543E-14, 15.17850393972633682 ) ) ;
#12365=CARTESIAN_POINT ( 'NONE',  ( 91.82158438592159655, -40.00000000000008527, 22.79471317813456110 ) ) ;
#12366=AXIS2_PLACEMENT_3D ( 'NONE', #7832, #9324, #868 ) ;
#12367=CARTESIAN_POINT ( 'NONE',  ( -56.48582580120559271, 2.158176344243877536E-14, -9.153146818113587102 ) ) ;
#12368=CARTESIAN_POINT ( 'NONE',  ( -135.8532207217289738, 9.153146818113546246, -0.000000000000000000 ) ) ;
#12369=CARTESIAN_POINT ( 'NONE',  ( -259.2033419157646676, -21.55415060305854524, 21.55415060305827524 ) ) ;
#12370=CARTESIAN_POINT ( 'NONE',  ( 91.82158438592159655, -22.79471317813468545, -2.449293598294708485E-15 ) ) ;
#12371=CARTESIAN_POINT ( 'NONE',  ( -259.2033419157646676, 35.01439189186528722, 21.55415060305857011 ) ) ;
#12372=CARTESIAN_POINT ( 'NONE',  ( 132.4338126186516149, -12.33615677966328938, -29.78211700502419390 ) ) ;
#12374=CARTESIAN_POINT ( 'NONE',  ( 19.06497207195981858, 5.735870351258996432E-13, -54.19242893257843008 ) ) ;
#12375=CARTESIAN_POINT ( 'NONE',  ( -135.8532207217289738, -1.351063376314938213E-13, 30.84685318188645553 ) ) ;
#12376=CARTESIAN_POINT ( 'NONE',  ( -91.56559293963834989, 12.25131212657490209, -44.31723036834897300 ) ) ;
#12379=CARTESIAN_POINT ( 'NONE',  ( 200.0000000000000000, -14.14213562373062949, -42.42640687119301646 ) ) ;
#12381=CARTESIAN_POINT ( 'NONE',  ( 146.6084372240433709, -24.48358557860284179, -32.08495691632087699 ) ) ;
#12383=CARTESIAN_POINT ( 'NONE',  ( -238.4067589809705510, -40.96449427998265946, -2.449293598294708485E-15 ) ) ;
#12388=VERTEX_POINT ( 'NONE', #15441 ) ;
#12393=CARTESIAN_POINT ( 'NONE',  ( 22.17571259162583175, 13.86510691866999778, 47.24006242885730700 ) ) ;
#12394=VERTEX_POINT ( 'NONE', #7454 ) ;
#12395=EDGE_LOOP ( 'NONE', ( #7015, #16373, #463, #3621 ) ) ;
#12396=CARTESIAN_POINT ( 'NONE',  ( 170.2234770963711128, -24.55285855007183926, 0.000000000000000000 ) ) ;
#12398=CARTESIAN_POINT ( 'NONE',  ( -77.70104068030501310, -11.20636163163649535, -18.98731336402689962 ) ) ;
#12400=EDGE_CURVE ( 'NONE', #12121, #16316, #4326, .T. ) ;
#12401=CARTESIAN_POINT ( 'NONE',  ( -135.8532207217289738, -6.472252184284190690, -6.472252184284188914 ) ) ;
#12402=CARTESIAN_POINT ( 'NONE',  ( 98.29820294273055481, 14.14213562373424971, 14.14213562373465294 ) ) ;
#12403=CARTESIAN_POINT ( 'NONE',  ( 136.1360204305621266, 7.947488714877270288E-14, -4.966164525587064560 ) ) ;
#12404=CARTESIAN_POINT ( 'NONE',  ( -208.1127848780265026, 1.189126717069624012E-13, -15.00245453012669472 ) ) ;
#12408=CARTESIAN_POINT ( 'NONE',  ( -188.9001212172966291, 17.93766612258000848, 43.30535683045329165 ) ) ;
#12409=CARTESIAN_POINT ( 'NONE',  ( -56.48582580120558561, -21.81201906317755146, -21.81201906317792449 ) ) ;
#12410=CARTESIAN_POINT ( 'NONE',  ( -200.0000000000000000, 14.89048929005512001, 48.59548038928821967 ) ) ;
#12411=CARTESIAN_POINT ( 'NONE',  ( 146.6084372240433709, 24.48358557860311180, 32.08495691632071356 ) ) ;
#12412=CARTESIAN_POINT ( 'NONE',  ( 23.37394308801978582, -46.80823611210187352, -13.80096434448294396 ) ) ;
#12413=CARTESIAN_POINT ( 'NONE',  ( -105.3755690713226585, 15.38646221621820764, -41.18208027870583265 ) ) ;
#12415=CARTESIAN_POINT ( 'NONE',  ( -86.96347745069645896, 21.75974354311648895, 40.00000000000002132 ) ) ;
#12416=CARTESIAN_POINT ( 'NONE',  ( -100.7734535825088358, -16.03295912088728770, 16.03295912088687913 ) ) ;
#12417=CARTESIAN_POINT ( 'NONE',  ( 136.1360204305621551, -4.966164525587043244, 40.00000000000002132 ) ) ;
#12419=CARTESIAN_POINT ( 'NONE',  ( 192.4448373802101173, 39.99999999999985079, 20.00000000003984013 ) ) ;
#12420=CARTESIAN_POINT ( 'NONE',  ( 14.38125909742180220, 39.01709431150916885, -17.55144818341463164 ) ) ;
#12421=CARTESIAN_POINT ( 'NONE',  ( 184.8905102610680444, -20.92133201514440799, 0.000000000000000000 ) ) ;
#12422=ORIENTED_EDGE ( 'NONE', *, *, #20621, .F. ) ;
#12424=FACE_OUTER_BOUND ( 'NONE', #22816, .T. ) ;
#12425=EDGE_CURVE ( 'NONE', #6406, #14842, #3163, .T. ) ;
#12427=( BOUNDED_SURFACE ( )  B_SPLINE_SURFACE ( 3, 2, ( 
 ( #10100, #14355, #124 ),
 ( #10233, #4655, #4525 ),
 ( #22616, #2386, #24610 ),
 ( #18611, #6766, #10767 ),
 ( #12352, #20611, #12623 ),
 ( #23018, #14483, #4392 ) ),
 .UNSPECIFIED., .F., .F., .F. ) 
 B_SPLINE_SURFACE_WITH_KNOTS ( ( 4, 2, 4 ),
 ( 3, 3 ),
 ( 0.04143179630788233064, 0.04845754690455064684, 0.05548329750121896997 ),
 ( 0.000000000000000000, 1.000000000000000000 ),
 .UNSPECIFIED. ) 
 GEOMETRIC_REPRESENTATION_ITEM ( )  RATIONAL_B_SPLINE_SURFACE ( (
 ( 1.000000000000000000, 0.9541700779530457588, 1.000000000000000000),
 ( 1.000000000000000000, 0.9520119187990010445, 1.000000000000000000),
 ( 1.000000000000000000, 0.9503150779442263163, 1.000000000000000000),
 ( 1.000000000000000000, 0.9480088369839682061, 1.000000000000000000),
 ( 1.000000000000000000, 0.9474362540968070956, 1.000000000000000000),
 ( 1.000000000000000000, 0.9474350314971540232, 1.000000000000000000) ) ) 
 REPRESENTATION_ITEM ( '' )  SURFACE ( )  );
#12428=CARTESIAN_POINT ( 'NONE',  ( -238.4067589809705794, 57.25054294065799354, -0.6820004457334954973 ) ) ;
#12429=CARTESIAN_POINT ( 'NONE',  ( -110.0368417077419707, -18.74474319002903755, -7.441767003006645176 ) ) ;
#12431=CARTESIAN_POINT ( 'NONE',  ( -87.08883615166497805, 3.401706263181337508, -21.20174225584124272 ) ) ;
#12434=CARTESIAN_POINT ( 'NONE',  ( -198.0356074513804572, 10.87444709761036066, -67.44298959253325165 ) ) ;
#12435=CARTESIAN_POINT ( 'NONE',  ( 151.7948205124836534, -33.06932595376376582, 23.49921654115996006 ) ) ;
#12437=CARTESIAN_POINT ( 'NONE',  ( -213.1075012329537230, 40.00000000000012790, -13.71589010951869980 ) ) ;
#12438=CARTESIAN_POINT ( 'NONE',  ( 57.59792236341148453, -26.56190807104663421, -26.56190807104710672 ) ) ;
#12439=CARTESIAN_POINT ( 'NONE',  ( 14.32711937312299000, 14.14294248749819793, 49.08922911798401145 ) ) ;
#12440=CARTESIAN_POINT ( 'NONE',  ( -126.6834156231698927, -11.16464796295173123, -24.04426801070755459 ) ) ;
#12441=CARTESIAN_POINT ( 'NONE',  ( -30.26275506840324070, -1.198031551616032919, 1.198031551616014712 ) ) ;
#12444=CARTESIAN_POINT ( 'NONE',  ( 146.6084372240433709, 40.00000000000003553, 5.374981219217116468 ) ) ;
#12445=B_SPLINE_CURVE_WITH_KNOTS ( 'NONE', 3,
 ( #19165, #4817, #12920, #21036, #15170, #23420, #7173, #11174, #2819, #16768, #10928, #8660, #19039, #818, #7055, #17034 ),
 .UNSPECIFIED., .F., .F.,
 ( 4, 2, 2, 2, 2, 2, 2, 4 ),
 ( 0.0003132551799524981831, 0.004485156913506553947, 0.006571107780283581314, 0.008657058647060608680, 0.01282896038061466341, 0.01387193581400317753, 0.01491491124739169165, 0.01700086211416872509 ),
 .UNSPECIFIED. ) ;
#12447=CARTESIAN_POINT ( 'NONE',  ( 22.31419732599935557, 43.29699898481473497, -17.93420418956763029 ) ) ;
#12448=CARTESIAN_POINT ( 'NONE',  ( 146.6084372240433993, 5.374981219216999229, 2.449293598294708485E-15 ) ) ;
#12450=CARTESIAN_POINT ( 'NONE',  ( 130.8568914410475372, -24.07718906447222551, -24.07718906447233209 ) ) ;
#12451=CARTESIAN_POINT ( 'NONE',  ( -4.037857402784122307, -46.99101396955040144, 13.82822410908682720 ) ) ;
#12452=CARTESIAN_POINT ( 'NONE',  ( 14.38125909742180752, 55.17850393972636880, 2.449293598294708485E-15 ) ) ;
#12453=EDGE_LOOP ( 'NONE', ( #24436, #13212, #5310, #3361 ) ) ;
#12454=B_SPLINE_CURVE_WITH_KNOTS ( 'NONE', 3,
 ( #10336, #498, #20849, #18583, #362, #8868 ),
 .UNSPECIFIED., .F., .F.,
 ( 4, 2, 4 ),
 ( 0.000000000000000000, 0.004324493460679611212, 0.008648986921359222424 ),
 .UNSPECIFIED. ) ;
#12455=CARTESIAN_POINT ( 'NONE',  ( -280.0000000000000568, -42.42640687119295251, 14.14213562373088351 ) ) ;
#12456=CARTESIAN_POINT ( 'NONE',  ( -5.859158571327203191, -13.69949429424866949, 46.35984297723813086 ) ) ;
#12457=CARTESIAN_POINT ( 'NONE',  ( -4.121597284766315816, 13.82232031192010702, -46.96202426942429753 ) ) ;
#12459=CARTESIAN_POINT ( 'NONE',  ( -238.4067589809705794, -3.369206980223063916E-14, -0.9644942799825824142 ) ) ;
#12461=CARTESIAN_POINT ( 'NONE',  ( -188.8384220655403851, -17.93083973458498193, 43.28887647197261401 ) ) ;
#12462=CARTESIAN_POINT ( 'NONE',  ( -208.1127848780265026, 10.60833733269551615, -10.60833733269529766 ) ) ;
#12463=CARTESIAN_POINT ( 'NONE',  ( -259.2033419157646676, 9.517827891722584255, -0.000000000000000000 ) ) ;
#12464=CARTESIAN_POINT ( 'NONE',  ( -188.9524938555910296, 23.58789616778520326, -43.19211203807366672 ) ) ;
#12465=CARTESIAN_POINT ( 'NONE',  ( 163.1118516004056573, 9.006482792073693844, 47.56205970284970164 ) ) ;
#12466=CARTESIAN_POINT ( 'NONE',  ( 91.82158438592158234, 16.11829626348378142, 40.45024623143977749 ) ) ;
#12467=EDGE_CURVE ( 'NONE', #2889, #22287, #2871, .T. ) ;
#12468=CARTESIAN_POINT ( 'NONE',  ( 184.8905102610680444, -19.07866798485553872, -40.00000000000002132 ) ) ;
#12469=CARTESIAN_POINT ( 'NONE',  ( 184.8905102610680444, 19.07866798485561333, 40.00000000000002132 ) ) ;
#12470=CARTESIAN_POINT ( 'NONE',  ( 19.06497207195981147, 1.521599808664285085E-13, -14.19242893257840521 ) ) ;
#12471=CARTESIAN_POINT ( 'NONE',  ( -86.96347745069644475, -15.38646221621796073, 41.18208027870593924 ) ) ;
#12472=( BOUNDED_CURVE ( )  B_SPLINE_CURVE ( 3, ( #15657, #3839, #13670, #18056 ),
 .UNSPECIFIED., .F., .F. ) 
 B_SPLINE_CURVE_WITH_KNOTS ( ( 4, 4 ),
 ( 0.01576650722535599680, 0.02368120503275411570 ),
 .UNSPECIFIED. ) 
 CURVE ( )  GEOMETRIC_REPRESENTATION_ITEM ( )  RATIONAL_B_SPLINE_CURVE ( ( 0.7232313460858506016, 0.6666666666666621888, 0.6208516971803421658, 0.5857864376268907547 ) ) 
 REPRESENTATION_ITEM ( '' )  );
#12473=CARTESIAN_POINT ( 'NONE',  ( 98.29820294267490510, 4.808046699556526995E-12, 20.00000000000513722 ) ) ;
#12474=CARTESIAN_POINT ( 'NONE',  ( -192.9588430854689705, -38.51493924976909966, -38.51493924976973915 ) ) ;
#12475=CARTESIAN_POINT ( 'NONE',  ( 91.82158438592158234, 12.16597498397773869, -12.16597498397759303 ) ) ;
#12478=CARTESIAN_POINT ( 'NONE',  ( 57.59792236341147031, -30.00663442387700641, 26.56190807104681895 ) ) ;
#12479=CARTESIAN_POINT ( 'NONE',  ( -88.38011430157065718, 8.298859908373991345, 20.03522014432801868 ) ) ;
#12480=CARTESIAN_POINT ( 'NONE',  ( 136.1360204305621551, 24.77266263493108411, 31.79587985999273769 ) ) ;
#12481=CARTESIAN_POINT ( 'NONE',  ( 19.66474694218199915, -43.90629905112487563, -18.18658454056792451 ) ) ;
#12484=CARTESIAN_POINT ( 'NONE',  ( 91.82158438592158234, -17.20528682183298486, 0.000000000000000000 ) ) ;
#12490=CARTESIAN_POINT ( 'NONE',  ( -190.0144721488272523, -43.47822244620601140, -23.79987203024255749 ) ) ;
#12491=CARTESIAN_POINT ( 'NONE',  ( 0.2972598230770030492, -1.921041075453695163E-13, 54.33493731733936016 ) ) ;
#12492=CARTESIAN_POINT ( 'NONE',  ( -105.3755690713226585, 18.24025645688350750, -40.00000000000002132 ) ) ;
#12495=CARTESIAN_POINT ( 'NONE',  ( 91.82158438592159655, -40.00000000000008527, 22.79471317813456110 ) ) ;
#12496=CARTESIAN_POINT ( 'NONE',  ( 136.1360204305621551, 40.00000000000017053, -35.03383547441281820 ) ) ;
#12498=CARTESIAN_POINT ( 'NONE',  ( -86.96347745069645896, 21.75974354311648895, -0.000000000000000000 ) ) ;
#12499=CARTESIAN_POINT ( 'NONE',  ( 57.59792236341148453, -37.56421063658185489, -2.449293598294708485E-15 ) ) ;
#12500=CARTESIAN_POINT ( 'NONE',  ( -56.48582580120558561, 6.472252184283903809, 50.09629031063968796 ) ) ;
#12501=CARTESIAN_POINT ( 'NONE',  ( 135.5356265174576720, -12.51227922893876787, -30.20731421070351530 ) ) ;
#12503=CARTESIAN_POINT ( 'NONE',  ( -208.1127848780265026, 5.403397259664334602E-13, -55.00245453012672670 ) ) ;
#12504=CARTESIAN_POINT ( 'NONE',  ( 19.06497207195981858, -1.881589693694111225E-13, 54.19242893257843008 ) ) ;
#12505=CARTESIAN_POINT ( 'NONE',  ( -135.8532207217289738, -6.472252184284190690, -6.472252184284188914 ) ) ;
#12506=CARTESIAN_POINT ( 'NONE',  ( 98.29820294273281434, -7.653668647304240125, 18.47759065023114644 ) ) ;
#12508=CARTESIAN_POINT ( 'NONE',  ( 19.06497207195982924, -66.60410523465823474, 10.03556273973400081 ) ) ;
#12510=CARTESIAN_POINT ( 'NONE',  ( -47.65341557546879869, 29.74088027398482481, -14.80716566708708370 ) ) ;
#12512=CARTESIAN_POINT ( 'NONE',  ( 151.7948205124836534, -6.767089262349000656, -40.00000000000002132 ) ) ;
#12513=CARTESIAN_POINT ( 'NONE',  ( -87.11162894489362429, -2.713946817493684271, -21.34897934681563569 ) ) ;
#12514=CARTESIAN_POINT ( 'NONE',  ( 4.995406935893289102, 10.78321810389013002, -10.78321810388986712 ) ) ;
#12515=VERTEX_POINT ( 'NONE', #14373 ) ;
#12518=CARTESIAN_POINT ( 'NONE',  ( -96.94449363886847948, 8.590991631032748543, -20.74048850978392977 ) ) ;
#12519=CARTESIAN_POINT ( 'NONE',  ( 6.615221834194239925, 24.79576599682247107, 44.82734842560557809 ) ) ;
#12520=VERTEX_POINT ( 'NONE', #8381 ) ;
#12522=CARTESIAN_POINT ( 'NONE',  ( -208.1127848780264742, 10.60833733270764867, 67.17687982763166588 ) ) ;
#12524=CARTESIAN_POINT ( 'NONE',  ( -114.7827252410166778, 0.6830184494088376024, 22.13181612764241279 ) ) ;
#12525=CARTESIAN_POINT ( 'NONE',  ( 85.88498484981873560, 23.37206192909128433, -8.769905300753718436 ) ) ;
#12526=CARTESIAN_POINT ( 'NONE',  ( -100.7734535825088500, 40.53558337403677569, -16.03295912088699993 ) ) ;
#12527=CARTESIAN_POINT ( 'NONE',  ( -199.9999999999999147, -14.17215463606695280, 49.28189405767609088 ) ) ;
#12529=CARTESIAN_POINT ( 'NONE',  ( 8.517493242715987734, 44.90626920808433198, -24.85395068094640081 ) ) ;
#12530=CARTESIAN_POINT ( 'NONE',  ( -208.1127848780265026, 5.403397259664334602E-13, -55.00245453012672670 ) ) ;
#12531=CARTESIAN_POINT ( 'NONE',  ( -208.1127848780264742, 40.00000000000014211, -15.00245453012627728 ) ) ;
#12532=CARTESIAN_POINT ( 'NONE',  ( 170.0000000000000000, 3.062538285713190422, -24.95097643316999481 ) ) ;
#12535=CARTESIAN_POINT ( 'NONE',  ( -187.7698581930736452, 13.79076165501289708, 46.80706826624406602 ) ) ;
#12536=CARTESIAN_POINT ( 'NONE',  ( 163.1118516004056573, 19.27778845538753316, 19.27778845538783870 ) ) ;
#12537=CARTESIAN_POINT ( 'NONE',  ( -200.0000000000000000, 16.05666331275189762, 47.66874763508933910 ) ) ;
#12538=CARTESIAN_POINT ( 'NONE',  ( -208.1127848780264742, 17.67593391476624021, 38.89260858015742883 ) ) ;
#12542=CARTESIAN_POINT ( 'NONE',  ( -162.0762913951020892, -1.198031840315659124, -57.76657433523998009 ) ) ;
#12544=CARTESIAN_POINT ( 'NONE',  ( 200.0000000000000000, 20.00000000000013856, 40.00000000000002132 ) ) ;
#12546=CARTESIAN_POINT ( 'NONE',  ( -56.48582580120559271, -6.472252184284276844, 6.472252184284108978 ) ) ;
#12547=CARTESIAN_POINT ( 'NONE',  ( 4.995406935893294431, -15.24977328854832415, 40.00000000000002132 ) ) ;
#12549=CARTESIAN_POINT ( 'NONE',  ( 136.1360204305621266, 7.947488714877270288E-14, -4.966164525587064560 ) ) ;
#12551=CARTESIAN_POINT ( 'NONE',  ( 155.4809970915716519, -11.45899766888376448, 27.66446758342024737 ) ) ;
#12552=ORIENTED_EDGE ( 'NONE', *, *, #3436, .T. ) ;
#12553=ORIENTED_EDGE ( 'NONE', *, *, #17029, .F. ) ;
#12554=CARTESIAN_POINT ( 'NONE',  ( -238.4067589809705794, 0.9644942799825385604, 40.00000000000002132 ) ) ;
#12557=CARTESIAN_POINT ( 'NONE',  ( 19.06497207195981147, 38.31983398719673772, -38.31983398719579981 ) ) ;
#12559=B_SPLINE_CURVE_WITH_KNOTS ( 'NONE', 3,
 ( #21244, #11368, #25114, #7246, #23368, #5144, #2761, #23491 ),
 .UNSPECIFIED., .F., .F.,
 ( 4, 2, 2, 4 ),
 ( 0.0002282271112605023934, 0.004312542793973171001, 0.006354700635329504736, 0.008396858476685838471 ),
 .UNSPECIFIED. ) ;
#12561=CARTESIAN_POINT ( 'NONE',  ( -189.4799804244524637, -43.33513910317152096, -23.69387126430435586 ) ) ;
#12564=CIRCLE ( 'NONE', #7043, 14.99999999999999822 ) ;
#12566=CARTESIAN_POINT ( 'NONE',  ( 57.59792236341147031, -30.00663442387662627, -26.56190807104723461 ) ) ;
#12567=CARTESIAN_POINT ( 'NONE',  ( -198.0356074513804572, -10.87444709759714634, -10.87444709759729911 ) ) ;
#12570=CARTESIAN_POINT ( 'NONE',  ( 4.995406935893291767, 40.00000000000059686, -55.24977328853165659 ) ) ;
#12572=CARTESIAN_POINT ( 'NONE',  ( -86.86493150571114086, -7.943527260496002107, 19.77569912839178912 ) ) ;
#12573=CARTESIAN_POINT ( 'NONE',  ( 163.1118516004056573, 27.26290988616875310, 0.000000000000000000 ) ) ;
#12574=CARTESIAN_POINT ( 'NONE',  ( -280.0000000000000000, -14.14213562373098831, -14.14213562373098654 ) ) ;
#12577=CARTESIAN_POINT ( 'NONE',  ( 146.6084372240433993, 24.48358557860341733, -24.48358557860313311 ) ) ;
#12578=CARTESIAN_POINT ( 'NONE',  ( -105.3755690713226869, 21.75974354311648540, -0.000000000000000000 ) ) ;
#12580=CARTESIAN_POINT ( 'NONE',  ( -280.0000000000000000, -1.237140859393462838E-13, 20.00000000000001421 ) ) ;
#12582=CIRCLE ( 'NONE', #1129, 14.99999999999999467 ) ;
#12583=CARTESIAN_POINT ( 'NONE',  ( 19.44355705749545393, 43.94967286772826043, -18.20455056366577651 ) ) ;
#12584=CARTESIAN_POINT ( 'NONE',  ( -86.96347745069644475, 18.24025645688351105, 2.449293598294708485E-15 ) ) ;
#12585=CARTESIAN_POINT ( 'NONE',  ( -100.7734535825088500, -44.31723036834903695, 12.25131212657476709 ) ) ;
#12586=CARTESIAN_POINT ( 'NONE',  ( -135.8532207217289738, -9.153146818113595984, 40.00000000000002132 ) ) ;
#12587=CARTESIAN_POINT ( 'NONE',  ( -47.50817905880760605, -30.33575659740361274, 12.56548180749028987 ) ) ;
#12588=CARTESIAN_POINT ( 'NONE',  ( 4.995406935893288214, 55.24977328853207581, 40.00000000000002132 ) ) ;
#12591=CARTESIAN_POINT ( 'NONE',  ( 22.26816181513974158, 23.58015273002503420, -43.18156009806470763 ) ) ;
#12592=CARTESIAN_POINT ( 'NONE',  ( -86.96347745069644475, -43.67073346367983788, 12.89780903124397149 ) ) ;
#12594=CARTESIAN_POINT ( 'NONE',  ( 6.202588567996412117, 24.77700748806132580, -44.80189419270392648 ) ) ;
#12597=CARTESIAN_POINT ( 'NONE',  ( 151.7948205124836250, -23.49921654116371883, 23.49921654116317526 ) ) ;
#12598=CARTESIAN_POINT ( 'NONE',  ( -86.86493150571114086, 7.943527260496203724, -19.77569912839170030 ) ) ;
#12600=CARTESIAN_POINT ( 'NONE',  ( -188.2652746676664606, -13.82569223135940994, 46.97858116095157754 ) ) ;
#12601=CARTESIAN_POINT ( 'NONE',  ( -86.96347745069644475, 15.38646221621772092, 15.38646221621800336 ) ) ;
#12602=CARTESIAN_POINT ( 'NONE',  ( 57.59792236341147031, -1.722363176414363206, -54.84617931850881689 ) ) ;
#12603=CARTESIAN_POINT ( 'NONE',  ( 169.9999999999999432, 22.62041470344884075, 9.369682556672378482 ) ) ;
#12604=CARTESIAN_POINT ( 'NONE',  ( 190.0000000000001137, 30.00000000000007461, 0.000000000000000000 ) ) ;
#12605=CARTESIAN_POINT ( 'NONE',  ( 91.82158438592158234, 44.40256751092319121, 12.16597498400105515 ) ) ;
#12606=CARTESIAN_POINT ( 'NONE',  ( 0.2972598230769938343, 10.13633138497486286, -10.13633138497461594 ) ) ;
#12607=CARTESIAN_POINT ( 'NONE',  ( 192.4448373802100889, -19.99999999996057198, -2.449293598294708485E-15 ) ) ;
#12608=CARTESIAN_POINT ( 'NONE',  ( -105.3755690713226727, 18.24025645688350750, 2.449293598294708485E-15 ) ) ;
#12609=CARTESIAN_POINT ( 'NONE',  ( -135.8532207217289738, -40.00000000000014211, 9.153146818113153671 ) ) ;
#12610=CARTESIAN_POINT ( 'NONE',  ( -259.2033419157646676, -6.730120644403570829, -6.730120644403545960 ) ) ;
#12612=CARTESIAN_POINT ( 'NONE',  ( -96.94449363889108895, 20.74048850978782710, -8.590991631004159856 ) ) ;
#12613=CARTESIAN_POINT ( 'NONE',  ( 130.8568914410475088, 24.07718906446937623, -32.49135343045455215 ) ) ;
#12614=CARTESIAN_POINT ( 'NONE',  ( -114.7823189589617812, -1.412059986362322217, 22.12960287296340667 ) ) ;
#12616=CARTESIAN_POINT ( 'NONE',  ( 4.995406935893297096, 10.78321810387837232, 67.35176059880234334 ) ) ;
#12617=CARTESIAN_POINT ( 'NONE',  ( -86.86578273022415431, 8.153770686794796774, 19.68494377654078420 ) ) ;
#12619=CARTESIAN_POINT ( 'NONE',  ( 200.0000000000000000, 14.14213562373083022, 42.42640687119289566 ) ) ;
#12620=CARTESIAN_POINT ( 'NONE',  ( -0.1993645192445167580, -44.04158448242537105, -18.24262160100613883 ) ) ;
#12621=ORIENTED_EDGE ( 'NONE', *, *, #6054, .F. ) ;
#12623=CARTESIAN_POINT ( 'NONE',  ( -77.55640685889153474, -14.66973468135498493, -16.62872065403529476 ) ) ;
#12628=CARTESIAN_POINT ( 'NONE',  ( -162.0762913951020892, 41.69427287682832173, 2.449293598294708485E-15 ) ) ;
#12631=CARTESIAN_POINT ( 'NONE',  ( -213.1075012329537230, -66.26714140136188291, -9.698598906438677503 ) ) ;
#12632=CARTESIAN_POINT ( 'NONE',  ( 0.2972598230770103767, -40.00000000000021316, 54.33493731733921805 ) ) ;
#12633=CARTESIAN_POINT ( 'NONE',  ( -198.0356074513804572, 39.99999999999979394, 55.37879056874835726 ) ) ;
#12635=CARTESIAN_POINT ( 'NONE',  ( -238.4067589809705794, -0.9644942799826263791, -40.00000000000002132 ) ) ;
#12636=CARTESIAN_POINT ( 'NONE',  ( -162.0762913951020892, -1.198031840385783919, 1.198031840385741731 ) ) ;
#12637=CARTESIAN_POINT ( 'NONE',  ( 163.1118516004056573, -12.73709011382471878, -40.00000000000002132 ) ) ;
#12638=CARTESIAN_POINT ( 'NONE',  ( -162.0762913951020892, -29.48230308784785692, 29.48230308784751230 ) ) ;
#12639=B_SPLINE_CURVE_WITH_KNOTS ( 'NONE', 3,
 ( #5469, #1358, #17187, #25451, #6945, #21325 ),
 .UNSPECIFIED., .F., .F.,
 ( 4, 2, 4 ),
 ( 5.976737427190428336E-15, 0.03937685942888527468, 0.07875371885776458192 ),
 .UNSPECIFIED. ) ;
#12640=CARTESIAN_POINT ( 'NONE',  ( 0.2972598230769957217, 1.502051041545559470E-13, -14.33493731733933352 ) ) ;
#12642=CARTESIAN_POINT ( 'NONE',  ( -114.6821015619858315, 12.10555619829009899, -18.42370988051194658 ) ) ;
#12643=CARTESIAN_POINT ( 'NONE',  ( -30.26275506840324425, 40.00000000000044764, -41.69427246844585255 ) ) ;
#12644=CARTESIAN_POINT ( 'NONE',  ( 0.2972598230770103767, -40.00000000000021316, 54.33493731733921805 ) ) ;
#12645=CARTESIAN_POINT ( 'NONE',  ( 57.59792236341147031, 26.56190807104693619, -30.00663442387692115 ) ) ;
#12647=CARTESIAN_POINT ( 'NONE',  ( -114.7756899093965615, -16.59394837943032286, 14.65087933327505532 ) ) ;
#12648=CARTESIAN_POINT ( 'NONE',  ( 136.1360204305621266, -3.511608612530379592, -53.05693388239318153 ) ) ;
#12650=CARTESIAN_POINT ( 'NONE',  ( -190.6721700386037810, 23.91541588165695842, -43.63442057298694721 ) ) ;
#12652=CARTESIAN_POINT ( 'NONE',  ( -105.3755690713226585, -18.24025645688353947, -40.00000000000002132 ) ) ;
#12654=CARTESIAN_POINT ( 'NONE',  ( 57.59792236341147031, -1.722363176415055985, 1.722363176415024677 ) ) ;
#12656=EDGE_LOOP ( 'NONE', ( #2990, #22978, #2115, #157 ) ) ;
#12659=CARTESIAN_POINT ( 'NONE',  ( 20.69615274311149378, 23.88537831998787908, 43.59383154590214815 ) ) ;
#12662=CARTESIAN_POINT ( 'NONE',  ( 184.8905102610680444, -14.79361573936379415, -14.79361573936387941 ) ) ;
#12664=CARTESIAN_POINT ( 'NONE',  ( -105.2333497863349550, 2.723647965520585856, 21.31134136414152991 ) ) ;
#12665=CARTESIAN_POINT ( 'NONE',  ( 130.8568914410475088, -52.36146031193419503, 4.207082182989537955 ) ) ;
#12667=CARTESIAN_POINT ( 'NONE',  ( 91.82158438592156813, 40.00000000000009948, -17.20528682183286051 ) ) ;
#12670=CARTESIAN_POINT ( 'NONE',  ( 57.59792236341147031, 40.00000000000042633, -37.56421063658144277 ) ) ;
#12671=CARTESIAN_POINT ( 'NONE',  ( -238.4067589809705794, 40.00000000000040501, -40.96449427990138759 ) ) ;
#12673=CARTESIAN_POINT ( 'NONE',  ( -86.86493150571114086, -19.60045294882784717, -8.366608963953355627 ) ) ;
#12675=CARTESIAN_POINT ( 'NONE',  ( -188.3508614409168445, 17.87647389380673246, 43.15762572182556767 ) ) ;
#12676=CARTESIAN_POINT ( 'NONE',  ( 4.995406935893293543, -10.78321810388990265, -10.78321810389009272 ) ) ;
#12677=CARTESIAN_POINT ( 'NONE',  ( -199.9999999999999716, -49.28189405767602693, 14.17215463606940595 ) ) ;
#12678=CARTESIAN_POINT ( 'NONE',  ( -91.56559293963834989, 16.03295912088683650, 40.53558337403684675 ) ) ;
#12680=CARTESIAN_POINT ( 'NONE',  ( -213.1075012329537230, -9.698598906462304825, -66.26714140138675191 ) ) ;
#12682=CARTESIAN_POINT ( 'NONE',  ( 14.38125909742181285, -15.17850393972633505, 0.000000000000000000 ) ) ;
#12683=CARTESIAN_POINT ( 'NONE',  ( -280.0000000000000568, 14.14213562373038968, 42.42640687119305198 ) ) ;
#12684=CARTESIAN_POINT ( 'NONE',  ( 130.8568914410475372, 34.05028731879791337, 0.000000000000000000 ) ) ;
#12687=CARTESIAN_POINT ( 'NONE',  ( 192.4448373802101173, -39.99999999999977973, -19.99999999996102673 ) ) ;
#12693=CARTESIAN_POINT ( 'NONE',  ( -208.1127848780265026, 55.00245453012668406, 2.449293598294708485E-15 ) ) ;
#12694=B_SPLINE_CURVE_WITH_KNOTS ( 'NONE', 3,
 ( #11738, #12010, #7737, #19723, #22130, #17851 ),
 .UNSPECIFIED., .F., .F.,
 ( 4, 2, 4 ),
 ( -6.000000002804640696E-08, 0.04017169238941901283, 0.08034344477883806346 ),
 .UNSPECIFIED. ) ;
#12696=CARTESIAN_POINT ( 'NONE',  ( 146.6084372240433993, 3.800685668858732935, -3.800685668858610367 ) ) ;
#12697=CARTESIAN_POINT ( 'NONE',  ( -114.7827252410749281, -22.13181612766661743, 0.6830184494021483976 ) ) ;
#12698=CARTESIAN_POINT ( 'NONE',  ( 130.8568914410475372, -24.07718906447222551, -24.07718906447233209 ) ) ;
#12699=CARTESIAN_POINT ( 'NONE',  ( -192.1131556193064682, 14.00853984552929354, -48.19965519933749931 ) ) ;
#12702=CARTESIAN_POINT ( 'NONE',  ( -162.0762913951021176, -27.08623940707584055, -29.48230308784799547 ) ) ;
#12703=CARTESIAN_POINT ( 'NONE',  ( 130.8568914410475088, -4.207082182990058428, 52.36146031193416661 ) ) ;
#12704=CARTESIAN_POINT ( 'NONE',  ( -96.94835807405050332, 20.73599944956087882, 8.589132201369160668 ) ) ;
#12705=CARTESIAN_POINT ( 'NONE',  ( -280.0000000000000568, 40.00000000000017764, -19.99999999999959144 ) ) ;
#12706=CARTESIAN_POINT ( 'NONE',  ( -280.0000000000000000, 14.14213562373078581, 14.14213562373108424 ) ) ;
#12707=CARTESIAN_POINT ( 'NONE',  ( 7.340276806054787606, 14.17250878947608861, 49.28408872342590286 ) ) ;
#12708=CARTESIAN_POINT ( 'NONE',  ( 19.06497207195980792, 10.03556273973433299, 10.03556273973436319 ) ) ;
#12709=CARTESIAN_POINT ( 'NONE',  ( 136.1360204305621551, -31.79587985999244282, -24.77266263493140386 ) ) ;
#12710=CARTESIAN_POINT ( 'NONE',  ( -208.1127848780265026, -15.00245453012673202, 0.000000000000000000 ) ) ;
#12712=CARTESIAN_POINT ( 'NONE',  ( 19.06497207195980792, 39.99999999999983658, 54.19242893257857929 ) ) ;
#12713=CARTESIAN_POINT ( 'NONE',  ( 37.15749683989281493, 41.79699086507442019, -12.76981037570198296 ) ) ;
#12714=CARTESIAN_POINT ( 'NONE',  ( -198.0356074513804572, 15.37879056873067007, 0.000000000000000000 ) ) ;
#12715=CARTESIAN_POINT ( 'NONE',  ( 151.7948205124836534, -51.78348778862535795, 4.785054706298367044 ) ) ;
#12716=CARTESIAN_POINT ( 'NONE',  ( 19.06497207195980792, 54.19242893257844429, 40.00000000000002132 ) ) ;
#12718=B_SPLINE_CURVE_WITH_KNOTS ( 'NONE', 3,
 ( #12572, #611, #6582, #19226, #10580, #23227, #4873, #1006, #14830, #2746, #18969, #17219 ),
 .UNSPECIFIED., .F., .F.,
 ( 4, 2, 2, 2, 2, 4 ),
 ( 9.771591248311271618E-17, 0.004680202113613741305, 0.009360404227227383731, 0.01170050528403420408, 0.01404060634084102616, 0.01872080845445462868 ),
 .UNSPECIFIED. ) ;
#12719=EDGE_CURVE ( 'NONE', #12515, #9554, #4132, .T. ) ;
#12720=CARTESIAN_POINT ( 'NONE',  ( -7.769366557096847536, -45.69637362127787839, 13.56374645827445136 ) ) ;
#12721=CARTESIAN_POINT ( 'NONE',  ( 192.4448373802101173, -20.00000000003938538, 40.00000000000002132 ) ) ;
#12723=ORIENTED_EDGE ( 'NONE', *, *, #10770, .T. ) ;
#12724=CARTESIAN_POINT ( 'NONE',  ( 73.43374752932638216, -12.96823637283634234, -26.88866000080070862 ) ) ;
#12725=B_SPLINE_CURVE_WITH_KNOTS ( 'NONE', 3,
 ( #13613, #23994, #3386, #11889, #5386, #9250, #19739, #13491, #21485, #9766, #21871, #9371, #5260, #1527, #17867, #19875 ),
 .UNSPECIFIED., .F., .F.,
 ( 4, 2, 2, 2, 2, 2, 2, 4 ),
 ( 0.0003132551814621161888, 0.004563509514629761864, 0.006688636681213585081, 0.007751200264505497123, 0.008813763847797409165, 0.01306401818096505907, 0.01518914534754888489, 0.01731427251413270724 ),
 .UNSPECIFIED. ) ;
#12726=CARTESIAN_POINT ( 'NONE',  ( -30.26275506840324070, -27.08623969584595770, 29.48230279907789608 ) ) ;
#12727=CARTESIAN_POINT ( 'NONE',  ( -3.564770973659789455, -17.92368662243711697, 43.27160733161164075 ) ) ;
#12730=CARTESIAN_POINT ( 'NONE',  ( -0.6848998192584003775, 13.98809697771244309, -48.06291537635669897 ) ) ;
#12732=CARTESIAN_POINT ( 'NONE',  ( -56.48582580120559982, 21.81201906317729922, 34.75652343174635917 ) ) ;
#12734=CARTESIAN_POINT ( 'NONE',  ( -87.13361725327075646, 0.6860286134974562522, 21.49321519333430786 ) ) ;
#12735=CARTESIAN_POINT ( 'NONE',  ( -188.3120606736142406, -13.82878088495403546, 46.99497558484350179 ) ) ;
#12736=CARTESIAN_POINT ( 'NONE',  ( -30.26275506840324070, -1.198031551616016266, -1.198031551616031587 ) ) ;
#12738=CARTESIAN_POINT ( 'NONE',  ( -30.26275506840324070, -27.08623969584554558, -29.48230279907826912 ) ) ;
#12739=CARTESIAN_POINT ( 'NONE',  ( 57.59792236341147031, 1.722363176415040886, 1.722363176415060426 ) ) ;
#12740=CARTESIAN_POINT ( 'NONE',  ( -280.0000000000000568, 42.42640687119294540, -14.14213562373059041 ) ) ;
#12741=CARTESIAN_POINT ( 'NONE',  ( -280.0000000000000568, -14.14213562373049449, -42.42640687119305198 ) ) ;
#12742=CARTESIAN_POINT ( 'NONE',  ( -135.8532207217289738, 21.81201906317729566, 34.75652343174635917 ) ) ;
#12743=CARTESIAN_POINT ( 'NONE',  ( -259.2033419157646676, -30.48217210827744950, 40.00000000000002132 ) ) ;
#12744=CARTESIAN_POINT ( 'NONE',  ( -30.26275506840324425, 1.694272468446254232, -40.00000000000002132 ) ) ;
#12745=CARTESIAN_POINT ( 'NONE',  ( 130.8568914410475088, -40.00000000000036238, 34.05028731879746573 ) ) ;
#12746=CARTESIAN_POINT ( 'NONE',  ( 14.38125909742180752, 10.73282306404720465, 10.73282306404724018 ) ) ;
#12747=CARTESIAN_POINT ( 'NONE',  ( -89.91646883266047041, 20.29783361045703316, -8.407637967992551253 ) ) ;
#12749=CARTESIAN_POINT ( 'NONE',  ( 151.7948205124836250, -4.785054706301600902, -4.785054706301715477 ) ) ;
#12750=CARTESIAN_POINT ( 'NONE',  ( -188.2652133075157224, 46.97855991888798854, -13.82568790539414572 ) ) ;
#12752=CARTESIAN_POINT ( 'NONE',  ( 151.7948205124836534, -23.49921654116027980, 33.06932595376354556 ) ) ;
#12754=CARTESIAN_POINT ( 'NONE',  ( -238.4067589809705794, -28.96627169325343942, 28.96627169325309126 ) ) ;
#12755=CARTESIAN_POINT ( 'NONE',  ( -3.473570583883275109, -43.29615835920788669, -17.93385599103721972 ) ) ;
#12757=CARTESIAN_POINT ( 'NONE',  ( 170.2234770963711128, -24.55285855007183926, 0.000000000000000000 ) ) ;
#12758=CARTESIAN_POINT ( 'NONE',  ( -110.0368417077420844, -7.992411109433259497, -18.51665893310629940 ) ) ;
#12761=CARTESIAN_POINT ( 'NONE',  ( 23.37394308801977161, 13.80096434448334186, -46.80823611210181667 ) ) ;
#12762=CARTESIAN_POINT ( 'NONE',  ( -56.48582580120559271, 30.84685318188643066, 2.449293598294708485E-15 ) ) ;
#12765=CARTESIAN_POINT ( 'NONE',  ( 91.82158438592159655, -44.40256751092341858, 12.16597498400012434 ) ) ;
#12766=CARTESIAN_POINT ( 'NONE',  ( 192.4448373802101173, -40.00000000000005684, 19.99999999996046185 ) ) ;
#12767=CARTESIAN_POINT ( 'NONE',  ( 163.1118516004056573, 40.00000000000014921, -27.26290988616858968 ) ) ;
#12768=CARTESIAN_POINT ( 'NONE',  ( -1.818469002956051073, 47.72215409237468720, -13.93708913181252562 ) ) ;
#12769=CARTESIAN_POINT ( 'NONE',  ( -105.3755690713226727, -18.24025645688354302, -2.449293598294708485E-15 ) ) ;
#12770=CARTESIAN_POINT ( 'NONE',  ( 22.17571259161183050, -23.59965736305000661, -43.20787961119341247 ) ) ;
#12772=CARTESIAN_POINT ( 'NONE',  ( -192.9588430854690273, -54.46834944101725284, -40.00000000000002132 ) ) ;
#12773=CARTESIAN_POINT ( 'NONE',  ( 4.995406935893305977, -39.06748935135212264, 39.06748935135171763 ) ) ;
#12774=AXIS2_PLACEMENT_3D ( 'NONE', #7324, #5597, #25322 ) ;
#12775=CARTESIAN_POINT ( 'NONE',  ( -110.0723150831391450, 10.27950330712184623, -17.37189535805912044 ) ) ;
#12776=CARTESIAN_POINT ( 'NONE',  ( 192.4448373802101173, 39.99999999999985079, 20.00000000003984013 ) ) ;
#12777=CARTESIAN_POINT ( 'NONE',  ( -56.48582580120559982, 39.99999999999990763, 30.84685318188658698 ) ) ;
#12778=CARTESIAN_POINT ( 'NONE',  ( 4.995406935893289102, 10.78321810388998081, 10.78321810389001811 ) ) ;
#12779=CARTESIAN_POINT ( 'NONE',  ( -83.21262154144254453, -13.72187187061479818, 33.12752917118424989 ) ) ;
#12781=CARTESIAN_POINT ( 'NONE',  ( -135.8532207217289738, -21.81201906317788186, 21.81201906317762962 ) ) ;
#12783=CARTESIAN_POINT ( 'NONE',  ( 184.8905102610680444, 14.79361573936375507, 14.79361573936398067 ) ) ;
#12784=CARTESIAN_POINT ( 'NONE',  ( -40.07203023075403792, 34.25109662815976463, -11.15662918589591079 ) ) ;
#12785=CARTESIAN_POINT ( 'NONE',  ( 151.0853911467766864, 29.06993079631229904, -12.04115959307975992 ) ) ;
#12786=CARTESIAN_POINT ( 'NONE',  ( -30.26275506840323004, -41.69427246844627888, -40.00000000000002132 ) ) ;
#12787=CARTESIAN_POINT ( 'NONE',  ( -87.04503123322949421, -4.710636111839787254, -20.91882565556209883 ) ) ;
#12792=CARTESIAN_POINT ( 'NONE',  ( -102.4068193528149777, 8.735227608997227833, -20.17396017424876220 ) ) ;
#12793=CARTESIAN_POINT ( 'NONE',  ( -94.58414068585072698, 8.590713000660940679, -20.73981583682874685 ) ) ;
#12794=CARTESIAN_POINT ( 'NONE',  ( 23.40652632867847061, 23.33303889678602516, 42.84715492600980014 ) ) ;
#12795=VERTEX_POINT ( 'NONE', #20630 ) ;
#12797=CARTESIAN_POINT ( 'NONE',  ( 200.0000000000000000, -42.42640687119293119, 14.14213562373082134 ) ) ;
#12800=CARTESIAN_POINT ( 'NONE',  ( -105.3239292022199152, -5.381957438726850285, 20.72686647364727364 ) ) ;
#12801=CARTESIAN_POINT ( 'NONE',  ( 151.7948205124836534, -23.49921654116027980, 33.06932595376354556 ) ) ;
#12804=B_SPLINE_CURVE_WITH_KNOTS ( 'NONE', 3,
 ( #24788, #14650, #22789, #14918, #4830, #12935 ),
 .UNSPECIFIED., .F., .F.,
 ( 4, 2, 4 ),
 ( 0.000000000000000000, 0.004090268262613940345, 0.008180536525227880690 ),
 .UNSPECIFIED. ) ;
#12806=CARTESIAN_POINT ( 'NONE',  ( -30.26275506840325136, 40.00000000000001421, 1.694272468446399227 ) ) ;
#12807=ADVANCED_FACE ( 'NONE', ( #14627 ), #15207, .T. ) ;
#12808=CARTESIAN_POINT ( 'NONE',  ( -200.0000000000000000, -20.90527768611929815, 45.34857661735442491 ) ) ;
#12810=CARTESIAN_POINT ( 'NONE',  ( -192.9588430854689989, 5.375290060580374156E-13, -54.46834944099972375 ) ) ;
#12811=CARTESIAN_POINT ( 'NONE',  ( -213.1075012329537230, 1.045191102001431893E-13, -13.71589010951911902 ) ) ;
#12815=CARTESIAN_POINT ( 'NONE',  ( -189.1288337602853460, 23.62383291543111241, 43.24060467048551715 ) ) ;
#12816=CARTESIAN_POINT ( 'NONE',  ( -259.2033419157646676, -21.55415060305872998, 35.01439189186525880 ) ) ;
#12817=DIRECTION ( 'NONE',  ( 0.01051738792037606486, 0.3656191332807844363, 0.9307051272719736312 ) ) ;
#12818=CARTESIAN_POINT ( 'NONE',  ( -192.9588430854690273, -10.23066800229550388, 66.79921049721887982 ) ) ;
#12820=AXIS2_PLACEMENT_3D ( 'NONE', #10397, #25049, #696 ) ;
#12821=CARTESIAN_POINT ( 'NONE',  ( 57.59792236341148453, 1.722363176415528940, -54.84617931850878136 ) ) ;
#12823=CARTESIAN_POINT ( 'NONE',  ( -83.21262154144251610, -13.72187187061454949, -33.12752917118435647 ) ) ;
#12825=CARTESIAN_POINT ( 'NONE',  ( -238.4067589809705794, 28.96627169325285678, 27.60227080167094726 ) ) ;
#12827=CARTESIAN_POINT ( 'NONE',  ( 130.8568914410475088, -5.949712681206671405, 40.00000000000002132 ) ) ;
#12829=VERTEX_POINT ( 'NONE', #6160 ) ;
#12830=CARTESIAN_POINT ( 'NONE',  ( 170.2234770963711128, 1.955190573858485757E-13, -15.44714144992816074 ) ) ;
#12834=ORIENTED_EDGE ( 'NONE', *, *, #6452, .F. ) ;
#12835=CARTESIAN_POINT ( 'NONE',  ( -238.4067589809705794, 40.96449427998256709, 2.449293598294708485E-15 ) ) ;
#12838=AXIS2_PLACEMENT_3D ( 'NONE', #25311, #7069, #20655 ) ;
#12839=CARTESIAN_POINT ( 'NONE',  ( -110.0471271034679575, -18.98461286763408040, -6.849398635789994749 ) ) ;
#12841=CARTESIAN_POINT ( 'NONE',  ( -77.59212294118390219, -13.55867551895970635, 17.46520578609403174 ) ) ;
#12842=CARTESIAN_POINT ( 'NONE',  ( 136.1360204305621551, -39.99999999999987921, -35.03383547441310242 ) ) ;
#12845=CARTESIAN_POINT ( 'NONE',  ( 200.0000000000000000, -42.42640687119272513, -14.14213562373140753 ) ) ;
#12846=CARTESIAN_POINT ( 'NONE',  ( -105.3755690713226727, 15.38646221621771737, 15.38646221621800514 ) ) ;
#12847=CARTESIAN_POINT ( 'NONE',  ( -103.9707779739353839, 20.03121292026044387, 8.297200062355283734 ) ) ;
#12848=CARTESIAN_POINT ( 'NONE',  ( -198.0356074513804572, 40.00000000000056843, -55.37879056871282302 ) ) ;
#12849=CARTESIAN_POINT ( 'NONE',  ( -259.2033419157646676, 6.730120644403426944, 6.730120644403592145 ) ) ;
#12850=CARTESIAN_POINT ( 'NONE',  ( -192.9588430854689989, 38.51493924976929861, 38.51493924976947625 ) ) ;
#12851=CARTESIAN_POINT ( 'NONE',  ( 192.4448373802100889, -14.14213562370313682, 14.14213562370301958 ) ) ;
#12854=CARTESIAN_POINT ( 'NONE',  ( 170.2234770963711128, 1.169953928977015745E-13, -24.55285855007187124 ) ) ;
#12855=CARTESIAN_POINT ( 'NONE',  ( -30.26275506840324070, 1.694272468446254232, 0.000000000000000000 ) ) ;
#12856=CARTESIAN_POINT ( 'NONE',  ( 163.1118516004056573, -19.27778845538761132, -19.27778845538770724 ) ) ;
#12857=CARTESIAN_POINT ( 'NONE',  ( 151.7948205124836534, -33.23291073765550863, 40.00000000000002132 ) ) ;
#12859=CARTESIAN_POINT ( 'NONE',  ( 11.38508063386201385, -49.30460303387604881, 14.17561098849807166 ) ) ;
#12860=CARTESIAN_POINT ( 'NONE',  ( 0.2972598230769930017, 54.33493731733936016, 40.00000000000002132 ) ) ;
#12863=CARTESIAN_POINT ( 'NONE',  ( 0.2972598230769938343, 10.13633138497472252, 10.13633138497475628 ) ) ;
#12864=CARTESIAN_POINT ( 'NONE',  ( -47.30403195827515361, -12.59259458036005164, 30.40121262124529267 ) ) ;
#12865=CARTESIAN_POINT ( 'NONE',  ( -213.1075012329537230, 9.698598906450410340, 9.698598906450483170 ) ) ;
#12866=CARTESIAN_POINT ( 'NONE',  ( -4.031723327955597291, 23.45082932595568437, -43.00750292060828173 ) ) ;
#12868=CARTESIAN_POINT ( 'NONE',  ( -30.26275506840325136, 29.48230279907760121, 27.08623969584625613 ) ) ;
#12869=CARTESIAN_POINT ( 'NONE',  ( -82.25136756411366434, -19.89060514489998610, 3.474794711464142427 ) ) ;
#12871=CARTESIAN_POINT ( 'NONE',  ( -194.4222169614207303, -24.44978956118232460, 44.35789444896035860 ) ) ;
#12872=CARTESIAN_POINT ( 'NONE',  ( 170.2234770963711128, -2.259079968736224833E-13, 24.55285855007187124 ) ) ;
#12873=EDGE_CURVE ( 'NONE', #12388, #162, #17118, .T. ) ;
#12874=CARTESIAN_POINT ( 'NONE',  ( 19.06497207195980792, 18.24870850772737185, 38.31983398719634692 ) ) ;
#12875=CARTESIAN_POINT ( 'NONE',  ( 192.4448373802101173, -14.14213562375826605, -42.42640687116518450 ) ) ;
#12876=CARTESIAN_POINT ( 'NONE',  ( -162.0762913951020892, -1.198031840385767266, -1.198031840385758384 ) ) ;
#12877=CARTESIAN_POINT ( 'NONE',  ( -162.0762913951020892, -1.198031840385767266, -1.198031840385758384 ) ) ;
#12878=CARTESIAN_POINT ( 'NONE',  ( -192.9588430854689989, 38.51493924976983152, -38.51493924976893624 ) ) ;
#12879=CARTESIAN_POINT ( 'NONE',  ( -162.0762913951021176, 57.76657433523994456, -1.198031840315424867 ) ) ;
#12880=CARTESIAN_POINT ( 'NONE',  ( 130.8568914410475088, 34.05028731879790627, 40.00000000000002132 ) ) ;
#12881=CARTESIAN_POINT ( 'NONE',  ( 200.0000000000000000, 19.99999999999996447, -40.00000000000002132 ) ) ;
#12882=CARTESIAN_POINT ( 'NONE',  ( -259.2033419157646676, 21.55415060305839958, -35.01439189186541512 ) ) ;
#12883=CARTESIAN_POINT ( 'NONE',  ( -259.2033419157646676, -1.438356298054549103E-14, -9.517827891722632216 ) ) ;
#12884=CARTESIAN_POINT ( 'NONE',  ( 91.82158438592159655, -44.40256751092341858, 12.16597498400012434 ) ) ;
#12885=ADVANCED_FACE ( 'NONE', ( #1780 ), #10411, .T. ) ;
#12886=CARTESIAN_POINT ( 'NONE',  ( -129.2303492456006211, 25.82246949204678899, -9.309000511913200882 ) ) ;
#12887=EDGE_LOOP ( 'NONE', ( #8841, #22397, #16381, #20343, #7561, #16282, #14475 ) ) ;
#12888=CARTESIAN_POINT ( 'NONE',  ( 57.59792236341147031, -1.722363176415123043, 54.84617931850879557 ) ) ;
#12889=CARTESIAN_POINT ( 'NONE',  ( -198.0012401002533124, 24.77357857137259600, 44.79720214428343894 ) ) ;
#12891=CARTESIAN_POINT ( 'NONE',  ( -213.1075012329537230, -9.698598906438496314, 66.26714140136188291 ) ) ;
#12892=CARTESIAN_POINT ( 'NONE',  ( 20.91285618071585617, -47.65039156503396356, -13.92631245146007757 ) ) ;
#12893=VERTEX_POINT ( 'NONE', #18257 ) ;
#12894=CARTESIAN_POINT ( 'NONE',  ( -100.0753760173596874, -20.72827493166422030, 8.149786832858520569 ) ) ;
#12895=CARTESIAN_POINT ( 'NONE',  ( -105.2054292633754784, -14.23662800545034024, -16.15936842200748202 ) ) ;
#12898=CARTESIAN_POINT ( 'NONE',  ( -213.1075012329537230, 53.71589010951910836, 2.449293598294708485E-15 ) ) ;
#12901=CARTESIAN_POINT ( 'NONE',  ( -208.1127848780264742, -38.89260858015753541, 17.67593391476614784 ) ) ;
#12902=CARTESIAN_POINT ( 'NONE',  ( -192.9588430854689989, -2.280704836619014309E-13, 54.46834944099972375 ) ) ;
#12903=CARTESIAN_POINT ( 'NONE',  ( 199.9999999999999432, -3.553951640073651008E-14, 19.99999999999992539 ) ) ;
#12906=CARTESIAN_POINT ( 'NONE',  ( 19.06497207195982924, -54.19242893257843008, -2.449293598294708485E-15 ) ) ;
#12907=CARTESIAN_POINT ( 'NONE',  ( 22.72189371636524768, -13.83659596078988052, -47.04833883278732998 ) ) ;
#12908=CARTESIAN_POINT ( 'NONE',  ( -100.7734535825088500, 16.03295912088713848, -16.03295912088698927 ) ) ;
#12909=CARTESIAN_POINT ( 'NONE',  ( -280.0000000000000568, -20.00000000000007105, 40.00000000000002132 ) ) ;
#12910=CARTESIAN_POINT ( 'NONE',  ( 136.1360204305621266, 53.05693388239316022, 3.511608612530967566 ) ) ;
#12911=CARTESIAN_POINT ( 'NONE',  ( -188.2995950289364373, 13.82811170417132196, 46.99046209955516673 ) ) ;
#12912=CARTESIAN_POINT ( 'NONE',  ( -114.6375327213591362, 18.99176668988436134, -11.19832436704016487 ) ) ;
#12913=CARTESIAN_POINT ( 'NONE',  ( -30.26275506840323359, 4.336144384597734078E-13, -41.69427246844629309 ) ) ;
#12914=CARTESIAN_POINT ( 'NONE',  ( 136.1360204305621266, -24.77266263493116583, -24.77266263493127951 ) ) ;
#12915=DIRECTION ( 'NONE',  ( 0.3301743741187893599, 0.000000000000000000, -0.9439199556505125654 ) ) ;
#12916=CARTESIAN_POINT ( 'NONE',  ( -114.6679276626374815, -11.81543316368266616, 18.60595090113752548 ) ) ;
#12917=CARTESIAN_POINT ( 'NONE',  ( -105.3755690713226585, 15.38646221621762678, 41.18208027870604582 ) ) ;
#12920=CARTESIAN_POINT ( 'NONE',  ( -77.70077460412264259, 5.497879648892802784, -21.35157292214961799 ) ) ;
#12921=CARTESIAN_POINT ( 'NONE',  ( -192.1167141818822586, 24.15421809699839528, -43.95739236919479964 ) ) ;
#12922=DIRECTION ( 'NONE',  ( 0.2259624730556991923, 0.9741360073267758546, 0.000000000000000000 ) ) ;
#12923=CARTESIAN_POINT ( 'NONE',  ( -56.48582580120557850, -30.84685318188645198, -2.449293598294708485E-15 ) ) ;
#12924=CARTESIAN_POINT ( 'NONE',  ( 170.0000000000000284, -12.70659020859091015, -21.59613885783092257 ) ) ;
#12925=CARTESIAN_POINT ( 'NONE',  ( -195.1686598214593573, 44.46432177479810832, -24.52826087131574440 ) ) ;
#12928=ORIENTED_EDGE ( 'NONE', *, *, #8162, .F. ) ;
#12930=CARTESIAN_POINT ( 'NONE',  ( -100.0968563617633720, 8.893120081483285588, -20.41799937591630965 ) ) ;
#12933=CARTESIAN_POINT ( 'NONE',  ( -162.0762913951021176, -27.08623940707624911, 29.48230308784761888 ) ) ;
#12935=CARTESIAN_POINT ( 'NONE',  ( -105.4741150117379789, -19.60045294982730724, -8.366608964594114184 ) ) ;
#12937=CARTESIAN_POINT ( 'NONE',  ( -30.26275506840324070, -27.08623969584595770, 29.48230279907789608 ) ) ;
#12938=CARTESIAN_POINT ( 'NONE',  ( -105.2054292635177006, 21.49321519473978981, 1.401583908954727953 ) ) ;
#12939=CARTESIAN_POINT ( 'NONE',  ( 192.4448373802100889, -3.692737725850373501E-14, 19.99999999996060751 ) ) ;
#12942=CARTESIAN_POINT ( 'NONE',  ( -162.0762913951020892, -39.99999999999961631, -41.69427287692722928 ) ) ;
#12943=CARTESIAN_POINT ( 'NONE',  ( 91.82158438592156813, 39.99999999999986500, 17.20528682183341473 ) ) ;
#12944=CARTESIAN_POINT ( 'NONE',  ( -109.1264249741455075, -13.72187187124534802, -33.12752917268997521 ) ) ;
#12947=CARTESIAN_POINT ( 'NONE',  ( -189.0115211946945237, 17.94954316430204599, 43.33403054566034740 ) ) ;
#12948=CARTESIAN_POINT ( 'NONE',  ( -192.9588430854689989, -10.23066800230742501, -10.23066800230756712 ) ) ;
#12949=CARTESIAN_POINT ( 'NONE',  ( -103.9474983245001738, 8.577167319634607878, 19.92928099173801826 ) ) ;
#12950=CARTESIAN_POINT ( 'NONE',  ( -56.48582580120559982, 34.75652343174597547, 21.81201906317791384 ) ) ;
#12951=CARTESIAN_POINT ( 'NONE',  ( -86.86493150571116928, -19.60045294882770861, 8.366608963953762412 ) ) ;
#12952=CARTESIAN_POINT ( 'NONE',  ( -192.9588430854690273, -10.23066800231931239, -66.79921049724377724 ) ) ;
#12953=CARTESIAN_POINT ( 'NONE',  ( -199.9999999999998863, 44.86667451853075050, -23.83166235904688435 ) ) ;
#12954=CARTESIAN_POINT ( 'NONE',  ( 192.4448373802101173, 20.00000000003945644, 40.00000000000002132 ) ) ;
#12955=CARTESIAN_POINT ( 'NONE',  ( 14.38125909742180220, 39.01709431150892016, 17.55144818341517166 ) ) ;
#12956=CARTESIAN_POINT ( 'NONE',  ( 184.8905102610680444, -19.07866798485554938, 40.00000000000002132 ) ) ;
#12957=DIRECTION ( 'NONE',  ( 0.2259624730536665960, 0.000000000000000000, -0.9741360073272474773 ) ) ;
#12959=CARTESIAN_POINT ( 'NONE',  ( -192.9588430854690273, -39.99999999999948841, -54.46834944098263520 ) ) ;
#12961=CARTESIAN_POINT ( 'NONE',  ( 149.5797498300188977, -12.18602109748358941, 29.41965740490864079 ) ) ;
#12962=VERTEX_POINT ( 'NONE', #20404 ) ;
#12963=ORIENTED_EDGE ( 'NONE', *, *, #15952, .T. ) ;
#12965=CARTESIAN_POINT ( 'NONE',  ( 19.06497207195980792, 54.19242893257843718, 2.449293598294708485E-15 ) ) ;
#12966=( NAMED_UNIT ( * ) PLANE_ANGLE_UNIT ( ) SI_UNIT ( $, .RADIAN. ) );
#12967=CARTESIAN_POINT ( 'NONE',  ( -105.2276882639529845, -21.34721338856009609, -2.726203881900004955 ) ) ;
#12968=CARTESIAN_POINT ( 'NONE',  ( -199.9999999999999432, 55.16984130226870064, 6.983587721173168283 ) ) ;
#12973=CARTESIAN_POINT ( 'NONE',  ( -105.3755690713226585, -15.38646221621738164, -41.18208027870615240 ) ) ;
#12974=CARTESIAN_POINT ( 'NONE',  ( -162.0762913951020892, -1.198031840385767266, -1.198031840385758384 ) ) ;
#12975=CARTESIAN_POINT ( 'NONE',  ( -110.1017833365194321, -15.17210968201788823, -13.38817875465654517 ) ) ;
#12976=CARTESIAN_POINT ( 'NONE',  ( 57.59792236341147742, 4.064940816252731242E-13, -37.56421063658186199 ) ) ;
#12978=CARTESIAN_POINT ( 'NONE',  ( -3.763361371728489946, 13.84281709279663808, 47.08953757622903424 ) ) ;
#12979=CARTESIAN_POINT ( 'NONE',  ( -135.8532207217289738, 6.472252184283881604, 50.09629031063969506 ) ) ;
#12980=FACE_OUTER_BOUND ( 'NONE', #22909, .T. ) ;
#12983=CARTESIAN_POINT ( 'NONE',  ( -192.9588430854689989, -8.596193650988133061E-14, 14.46834944099969533 ) ) ;
#12986=CARTESIAN_POINT ( 'NONE',  ( -238.4067589809705794, 0.6820004457340470561, 57.25054294065803617 ) ) ;
#12987=CARTESIAN_POINT ( 'NONE',  ( -192.9588430854690273, 14.46834944099966336, 40.00000000000002132 ) ) ;
#12988=ORIENTED_EDGE ( 'NONE', *, *, #10932, .F. ) ;
#12989=CARTESIAN_POINT ( 'NONE',  ( 21.25019396252282178, -43.56030393974950243, 18.04326867294216896 ) ) ;
#12991=AXIS2_PLACEMENT_3D ( 'NONE', #8693, #24401, #14667 ) ;
#12992=CARTESIAN_POINT ( 'NONE',  ( 4.995406935893288214, 15.24977328854832770, -40.00000000000002132 ) ) ;
#12994=CARTESIAN_POINT ( 'NONE',  ( -135.8532207217289738, -6.472252184284287502, 50.09629031063965243 ) ) ;
#12995=CARTESIAN_POINT ( 'NONE',  ( 199.9999999999999432, 1.065690307512836407E-13, -20.00000000000010303 ) ) ;
#12996=CARTESIAN_POINT ( 'NONE',  ( -82.24214707262626689, 20.09197113510544241, -2.401591935735043926 ) ) ;
#12998=CIRCLE ( 'NONE', #4076, 14.99999999999999822 ) ;
#13000=CARTESIAN_POINT ( 'NONE',  ( -62.69292774209460362, 11.76166271882766523, -24.97541154606644653 ) ) ;
#13002=CARTESIAN_POINT ( 'NONE',  ( -91.56559293963834989, -16.03295912088728414, 16.03295912088688269 ) ) ;
#13003=CARTESIAN_POINT ( 'NONE',  ( -77.70139926393163421, -21.34823270893657110, 5.508459030604740292 ) ) ;
#13005=CARTESIAN_POINT ( 'NONE',  ( -188.2957210513755797, -23.44847782072233144, 43.00408675155275517 ) ) ;
#13006=CARTESIAN_POINT ( 'NONE',  ( 4.995406935893290878, 1.606505379428369110E-13, -15.24977328854832592 ) ) ;
#13007=CARTESIAN_POINT ( 'NONE',  ( -56.48582580120559271, 6.472252184284211118, -6.472252184284153387 ) ) ;
#13009=CARTESIAN_POINT ( 'NONE',  ( -91.56559293963836410, 44.31723036834908669, -12.25131212657445801 ) ) ;
#13011=FACE_OUTER_BOUND ( 'NONE', #20979, .T. ) ;
#13012=CARTESIAN_POINT ( 'NONE',  ( 14.38125909742181108, 39.01709431150961649, -39.01709431150867147 ) ) ;
#13013=CARTESIAN_POINT ( 'NONE',  ( -198.0356074513804572, 10.87444709761036066, -67.44298959253325165 ) ) ;
#13014=CARTESIAN_POINT ( 'NONE',  ( -105.3755690713226727, -21.75974354311652093, 0.000000000000000000 ) ) ;
#13015=B_SPLINE_CURVE_WITH_KNOTS ( 'NONE', 3,
 ( #5944, #26049, #7786, #15768, #3417, #19772, #20050, #13778, #7397, #22186, #26188, #15637, #7654, #15902, #7927, #17512, #3960, #7529, #24031, #12058, #23640, #20177, #1428, #1828, #5810, #13915, #5418, #24169, #9407, #22050, #21775, #9528, #25651, #11925, #9666, #13519, #9930, #21645, #18036, #11519, #19644, #25779, #23763, #21908, #5543, #1561 ),
 .UNSPECIFIED., .F., .F.,
 ( 4, 2, 2, 2, 2, 2, 2, 2, 2, 2, 2, 2, 2, 2, 2, 2, 2, 2, 2, 2, 2, 2, 4 ),
 ( -5.298243351209276186E-05, 0.005693729153214702014, 0.01144044073994149660, 0.02293386391339508404, 0.04592071026030229708, 0.05741413343375589146, 0.06890755660720948583, 0.07465426819393627955, 0.07752762398729966253, 0.07896430188398136096, 0.08040097978066305939, 0.08614769136738986699, 0.09189440295411666071, 0.09476775874748007145, 0.09764111454084345443, 0.1033878261275702481, 0.1062611819209336589, 0.1076978598176153573, 0.1091345377142970419, 0.1148812493010238633, 0.1378680956479311215, 0.1608549419948383796, 0.1838417883417456655 ),
 .UNSPECIFIED. ) ;
#13016=CARTESIAN_POINT ( 'NONE',  ( 192.4448373802101173, 14.14213562370320076, -42.42640687122072762 ) ) ;
#13018=CARTESIAN_POINT ( 'NONE',  ( 57.59792236341148453, -54.84617931850879557, 1.722363176414566155 ) ) ;
#13019=CARTESIAN_POINT ( 'NONE',  ( -188.3065677117056396, 46.99298756134918875, -13.82848612971604751 ) ) ;
#13022=CARTESIAN_POINT ( 'NONE',  ( -192.9588430854689989, 38.51493924976929861, 38.51493924976947625 ) ) ;
#13024=CARTESIAN_POINT ( 'NONE',  ( -208.1127848780264742, 17.67593391476624021, 38.89260858015742883 ) ) ;
#13025=CARTESIAN_POINT ( 'NONE',  ( 98.29850319075929121, -18.72964005484536187, -7.044854747077215151 ) ) ;
#13027=CARTESIAN_POINT ( 'NONE',  ( -187.3036811847654803, -46.64553187115656385, 13.75782060302593379 ) ) ;
#13029=DIRECTION ( 'NONE',  ( 0.000000000000000000, 1.000000000000000000, 0.000000000000000000 ) ) ;
#13030=B_SPLINE_CURVE_WITH_KNOTS ( 'NONE', 3,
 ( #12673, #14797, #20936, #22928, #714, #2574 ),
 .UNSPECIFIED., .F., .F.,
 ( 4, 2, 4 ),
 ( 0.0002283644213467581811, 0.004316914013642671882, 0.008405463605938585936 ),
 .UNSPECIFIED. ) ;
#13031=( BOUNDED_CURVE ( )  B_SPLINE_CURVE ( 3, ( #26254, #16109, #6012, #16246 ),
 .UNSPECIFIED., .F., .T. ) 
 B_SPLINE_CURVE_WITH_KNOTS ( ( 4, 4 ),
 ( 0.007854122480103177539, 0.01576650722530729271 ),
 .UNSPECIFIED. ) 
 CURVE ( )  GEOMETRIC_REPRESENTATION_ITEM ( )  RATIONAL_B_SPLINE_CURVE ( ( 0.5857864376268384632, 0.5560595459730424128, 0.5340584217468479222, 0.5197830649482548804 ) ) 
 REPRESENTATION_ITEM ( '' )  );
#13032=CARTESIAN_POINT ( 'NONE',  ( -259.2033419157646676, 30.48217210827735713, -40.00000000000002132 ) ) ;
#13035=CARTESIAN_POINT ( 'NONE',  ( 14.38125909742181818, -39.01709431150928253, 17.55144818341435808 ) ) ;
#13036=CARTESIAN_POINT ( 'NONE',  ( 184.8905102610680444, -3.509827109981123710E-14, 19.07866798485558490 ) ) ;
#13037=CARTESIAN_POINT ( 'NONE',  ( -105.3755690713226585, 39.99999999999993605, 18.24025645688366737 ) ) ;
#13038=CARTESIAN_POINT ( 'NONE',  ( -192.1131556193065819, -24.17676952300933380, -43.98783656160069455 ) ) ;
#13039=CARTESIAN_POINT ( 'NONE',  ( -86.96347745069643054, -18.24025645688353947, -40.00000000000002132 ) ) ;
#13040=CARTESIAN_POINT ( 'NONE',  ( 23.17367289775620876, -23.38495170326278583, -42.91822977676284978 ) ) ;
#13042=CARTESIAN_POINT ( 'NONE',  ( -30.26275506840323004, -41.69427246844629309, 40.00000000000002132 ) ) ;
#13043=CARTESIAN_POINT ( 'NONE',  ( -30.26275506840325136, 27.08623969584573388, 29.48230279907808793 ) ) ;
#13044=CARTESIAN_POINT ( 'NONE',  ( -86.96347745069645896, 39.99999999999977973, 21.75974354311691883 ) ) ;
#13045=CARTESIAN_POINT ( 'NONE',  ( -110.0947178154681296, 15.96121929954245822, -12.38433105676308799 ) ) ;
#13046=CARTESIAN_POINT ( 'NONE',  ( 184.8905102610680444, 2.362515690532070066E-13, -19.07866798485558490 ) ) ;
#13047=CARTESIAN_POINT ( 'NONE',  ( -208.1127848780265026, 10.60833733269537049, 10.60833733269544510 ) ) ;
#13050=CARTESIAN_POINT ( 'NONE',  ( 170.2234770963711128, -10.92277846919202666, 10.92277846919193962 ) ) ;
#13052=CARTESIAN_POINT ( 'NONE',  ( -86.96347745069644475, 15.38646221621772092, 15.38646221621800336 ) ) ;
#13053=CARTESIAN_POINT ( 'NONE',  ( -47.50817905881116587, 30.33575659741672226, -12.56548180764576905 ) ) ;
#13054=CARTESIAN_POINT ( 'NONE',  ( 156.5537079553356818, 27.23618587942436164, -11.28159757857213208 ) ) ;
#13055=CARTESIAN_POINT ( 'NONE',  ( 163.1118516004056573, -12.73709011382472234, -2.449293598294708485E-15 ) ) ;
#13056=CARTESIAN_POINT ( 'NONE',  ( -114.4364955367327070, 8.644468109209567430, -20.04994829327642947 ) ) ;
#13057=CARTESIAN_POINT ( 'NONE',  ( -188.9478457324744625, 43.31767415847507152, -17.94276812689866674 ) ) ;
#13061=CARTESIAN_POINT ( 'NONE',  ( 159.7744820660626317, 10.75261058663767422, -25.95909830917682370 ) ) ;
#13062=ORIENTED_EDGE ( 'NONE', *, *, #2653, .T. ) ;
#13063=CIRCLE ( 'NONE', #294, 14.99999999999999822 ) ;
#13065=ORIENTED_EDGE ( 'NONE', *, *, #20542, .F. ) ;
#13067=CARTESIAN_POINT ( 'NONE',  ( -110.0563856373237002, -6.246938629525583764, 19.19543633473636746 ) ) ;
#13069=CARTESIAN_POINT ( 'NONE',  ( -86.96347745069644475, -43.67073346367983788, 12.89780903124397149 ) ) ;
#13070=AXIS2_PLACEMENT_3D ( 'NONE', #24442, #18581, #24578 ) ;
#13071=CARTESIAN_POINT ( 'NONE',  ( 0.2972598230769938343, 10.13633138497472252, 10.13633138497475628 ) ) ;
#13072=CARTESIAN_POINT ( 'NONE',  ( -56.48582580120559982, 39.99999999999990763, 30.84685318188658698 ) ) ;
#13073=CARTESIAN_POINT ( 'NONE',  ( -200.0000000000000568, -46.38610861938602881, 18.14877749763665804 ) ) ;
#13076=CARTESIAN_POINT ( 'NONE',  ( 4.995406935893306866, -39.99999999999944578, -55.24977328856505920 ) ) ;
#13077=CARTESIAN_POINT ( 'NONE',  ( -162.0762913951020892, 4.094006889353306706E-13, -41.69427287682835015 ) ) ;
#13078=CARTESIAN_POINT ( 'NONE',  ( -77.93386762624879793, 20.16917687840208373, 8.295512132613184875 ) ) ;
#13079=CARTESIAN_POINT ( 'NONE',  ( -87.11144460387475874, 13.16696799080288294, 17.02331989627854725 ) ) ;
#13081=CARTESIAN_POINT ( 'NONE',  ( 0.2972598230769976091, -10.13633138497479180, 10.13633138497468522 ) ) ;
#13082=CARTESIAN_POINT ( 'NONE',  ( 128.5824617753800396, 28.96492468983269220, 11.99766463964413354 ) ) ;
#13085=CARTESIAN_POINT ( 'NONE',  ( -77.70150415250706999, -11.19846400429647559, 18.99169997607589977 ) ) ;
#13086=CARTESIAN_POINT ( 'NONE',  ( 192.4448373802100889, -14.14213562370293431, -14.14213562370322030 ) ) ;
#13087=CARTESIAN_POINT ( 'NONE',  ( -173.7925586252259507, -12.78856870752416697, -41.93433064649377684 ) ) ;
#13088=CARTESIAN_POINT ( 'NONE',  ( -77.78698611455740775, 9.956332155370628101, 19.58753816231132205 ) ) ;
#13090=CARTESIAN_POINT ( 'NONE',  ( 14.38125909742180752, 10.73282306404735387, -10.73282306404708919 ) ) ;
#13094=CARTESIAN_POINT ( 'NONE',  ( 14.38125909742181818, 5.830552384690105017E-13, -55.17850393972636880 ) ) ;
#13096=CARTESIAN_POINT ( 'NONE',  ( -105.4894168351564048, 19.67999904371083275, 8.151722511394638104 ) ) ;
#13100=CARTESIAN_POINT ( 'NONE',  ( 184.8905102610680444, 19.07866798485562043, 2.449293598294708485E-15 ) ) ;
#13101=( LENGTH_UNIT ( ) NAMED_UNIT ( * ) SI_UNIT ( .MILLI., .METRE. ) );
#13102=CARTESIAN_POINT ( 'NONE',  ( -77.79405973474285929, -19.55084590669412137, 9.945757298486981313 ) ) ;
#13106=CARTESIAN_POINT ( 'NONE',  ( -192.9588430854689989, 10.23066800230756712, -10.23066800230735396 ) ) ;
#13107=CARTESIAN_POINT ( 'NONE',  ( 163.1118516004056573, 19.27778845538753316, 19.27778845538783870 ) ) ;
#13109=CARTESIAN_POINT ( 'NONE',  ( -91.56559293963834989, -39.99999999999985789, -17.32597176626853042 ) ) ;
#13110=CARTESIAN_POINT ( 'NONE',  ( 130.8568914410475372, 24.07718906447210472, 24.07718906447249907 ) ) ;
#13111=CARTESIAN_POINT ( 'NONE',  ( 4.995406935893307754, -55.24977328853207581, -40.00000000000002132 ) ) ;
#13112=CARTESIAN_POINT ( 'NONE',  ( -86.96347745069643054, 15.38646221621763210, 41.18208027870604582 ) ) ;
#13115=CARTESIAN_POINT ( 'NONE',  ( -280.0000000000000568, 40.00000000000004263, -19.99999999999987210 ) ) ;
#13116=CARTESIAN_POINT ( 'NONE',  ( 184.8905102610680444, -20.92133201514440799, 0.000000000000000000 ) ) ;
#13117=CARTESIAN_POINT ( 'NONE',  ( -213.1075012329537230, 9.698598906462684965, 66.26714140138669507 ) ) ;
#13118=CARTESIAN_POINT ( 'NONE',  ( 136.1360204305621266, -35.03383547441293899, 0.000000000000000000 ) ) ;
#13120=ORIENTED_EDGE ( 'NONE', *, *, #7013, .F. ) ;
#13121=CARTESIAN_POINT ( 'NONE',  ( 22.13784119383794291, -43.34234508276703224, 17.95298715833492764 ) ) ;
#13122=CARTESIAN_POINT ( 'NONE',  ( 0.2972598230769930017, 14.33493731733933352, -40.00000000000002132 ) ) ;
#13124=CARTESIAN_POINT ( 'NONE',  ( -208.1127848780265026, 38.89260858015724409, 38.89260858015741462 ) ) ;
#13125=CARTESIAN_POINT ( 'NONE',  ( -213.1075012329537230, -8.703598725189323045E-14, 13.71589010951911902 ) ) ;
#13126=CARTESIAN_POINT ( 'NONE',  ( -82.28220112168970957, 19.20590466794900664, -6.216954113673384796 ) ) ;
#13130=B_SPLINE_CURVE_WITH_KNOTS ( 'NONE', 3,
 ( #4195, #14017, #9897, #12288, #22547, #22147, #20416, #1923, #4328, #13881, #6561, #25076 ),
 .UNSPECIFIED., .F., .F.,
 ( 4, 2, 2, 2, 2, 4 ),
 ( 1.723928531167631343E-15, 0.004698945756008387348, 0.007048418634011698047, 0.009397891512015008747, 0.01409683726802167178, 0.01879578302402833481 ),
 .UNSPECIFIED. ) ;
#13131=CARTESIAN_POINT ( 'NONE',  ( 91.82158438592158234, -12.16597498397778843, 12.16597498397750954 ) ) ;
#13132=CARTESIAN_POINT ( 'NONE',  ( -82.24889283716301236, -19.94440861092025585, 3.157952835704525896 ) ) ;
#13133=CARTESIAN_POINT ( 'NONE',  ( 98.29820294267493352, -20.00000000000511235, 5.223721743777709619E-12 ) ) ;
#13134=AXIS2_PLACEMENT_3D ( 'NONE', #19224, #747, #25099 ) ;
#13135=CARTESIAN_POINT ( 'NONE',  ( -200.4318156386385965, -24.83634777281915618, 44.88237417767410875 ) ) ;
#13136=CARTESIAN_POINT ( 'NONE',  ( 199.9999999999999432, 14.14213562373093680, 14.14213562373114641 ) ) ;
#13137=CARTESIAN_POINT ( 'NONE',  ( -30.26275506840324070, -1.198031551616032919, 1.198031551616014712 ) ) ;
#13139=CARTESIAN_POINT ( 'NONE',  ( -100.7734535825088500, 16.03295912088691821, 16.03295912088721309 ) ) ;
#13140=CARTESIAN_POINT ( 'NONE',  ( 170.2234770963711128, 17.36149277826980253, 17.36149277827007253 ) ) ;
#13141=CARTESIAN_POINT ( 'NONE',  ( -208.1127848780265026, 38.89260858015777700, -38.89260858015687461 ) ) ;
#13142=CARTESIAN_POINT ( 'NONE',  ( -56.48582580120559982, -6.472252184283581400, -50.09629031063973059 ) ) ;
#13143=CARTESIAN_POINT ( 'NONE',  ( 136.1360204305621551, -35.03383547441293899, -40.00000000000002132 ) ) ;
#13144=CARTESIAN_POINT ( 'NONE',  ( -91.56559293963834989, -16.03295912088706388, -16.03295912088710651 ) ) ;
#13146=CARTESIAN_POINT ( 'NONE',  ( -192.9588430854690273, -38.51493924976957572, 18.05360324515410397 ) ) ;
#13147=CARTESIAN_POINT ( 'NONE',  ( -187.7698581930969510, 42.84913646251646924, -23.34605429453463543 ) ) ;
#13149=EDGE_CURVE ( 'NONE', #4428, #2784, #4736, .T. ) ;
#13150=CARTESIAN_POINT ( 'NONE',  ( 4.995406935893290878, 39.06748935135185263, 39.06748935135198764 ) ) ;
#13152=CARTESIAN_POINT ( 'NONE',  ( -62.69292774223515607, -25.97703433354730862, -9.343531400732226544 ) ) ;
#13156=CARTESIAN_POINT ( 'NONE',  ( 23.35928221536310190, -23.34300348377129453, 42.86167611819467993 ) ) ;
#13157=CARTESIAN_POINT ( 'NONE',  ( -91.56559293963834989, -22.67402823373193499, -40.00000000000002132 ) ) ;
#13160=CARTESIAN_POINT ( 'NONE',  ( -100.7734535825088500, -40.53558337403692491, 16.03295912088671571 ) ) ;
#13161=CARTESIAN_POINT ( 'NONE',  ( 4.995406935893283773, 39.99999999999997158, 15.24977328854846803 ) ) ;
#13163=CARTESIAN_POINT ( 'NONE',  ( -4.039451493210481026, -46.99046209229813797, 13.82811171175447917 ) ) ;
#13164=CARTESIAN_POINT ( 'NONE',  ( 184.8905102610680444, -19.07866798485553872, -40.00000000000002132 ) ) ;
#13165=CARTESIAN_POINT ( 'NONE',  ( 19.94008347559031691, -24.01421467035550350, -43.76810615268311011 ) ) ;
#13166=CARTESIAN_POINT ( 'NONE',  ( 151.7948205124836250, 23.49921654116361225, -23.49921654116333514 ) ) ;
#13167=CARTESIAN_POINT ( 'NONE',  ( 19.06497207195980792, -14.19242893257839988, 40.00000000000002132 ) ) ;
#13168=CARTESIAN_POINT ( 'NONE',  ( 184.8905102610680444, 14.79361573936396113, -14.79361573936377461 ) ) ;
#13169=CARTESIAN_POINT ( 'NONE',  ( 136.1360204305621551, 39.99999999999968026, 35.03383547441337953 ) ) ;
#13170=CARTESIAN_POINT ( 'NONE',  ( -105.4741150117381778, 8.366608964590609432, -19.60045294982858977 ) ) ;
#13171=CARTESIAN_POINT ( 'NONE',  ( -91.56559293963834989, -39.99999999999985789, -17.32597176626853042 ) ) ;
#13175=CARTESIAN_POINT ( 'NONE',  ( -135.8532207217289738, 34.75652343174594705, 21.81201906317792449 ) ) ;
#13176=VERTEX_POINT ( 'NONE', #20268 ) ;
#13178=CARTESIAN_POINT ( 'NONE',  ( -4.339409867971697921, 43.06267456183267939, -17.83714383556867489 ) ) ;
#13179=CARTESIAN_POINT ( 'NONE',  ( 136.1360204305621266, 35.03383547441298163, 40.00000000000002132 ) ) ;
#13180=AXIS2_PLACEMENT_3D ( 'NONE', #8528, #4557, #16514 ) ;
#13181=CARTESIAN_POINT ( 'NONE',  ( -188.4265004370346901, 47.03620155434742145, -13.83489460444945607 ) ) ;
#13183=ORIENTED_EDGE ( 'NONE', *, *, #6868, .T. ) ;
#13185=CARTESIAN_POINT ( 'NONE',  ( -96.93773665438806120, 9.001171854902148439, -20.58457565566403602 ) ) ;
#13187=CARTESIAN_POINT ( 'NONE',  ( 151.7948205124836250, 1.439163438361279259E-13, -33.23291073765553705 ) ) ;
#13189=( BOUNDED_SURFACE ( )  B_SPLINE_SURFACE ( 3, 3, ( 
 ( #18119, #8272, #16526, #10011, #10540, #16123, #22660, #2042, #12401, #6542, #10145, #18251, #22127, #16394, #33, #12271, #10280, #167, #20524, #6410, #14527, #6935, #10946, #10811, #19182, #23182, #11188, #6806, #572, #23059 ),
 ( #8944, #21314, #14919, #2563, #14651, #24922, #15053, #4831, #4962, #19053, #18922, #966, #13069, #19303, #12937, #16787, #25055, #17308, #16921, #25312, #835, #12665, #1088, #5088, #20927, #21052, #6674, #10678, #9196, #2837 ),
 ( #25440, #17051, #25186, #9070, #21186, #2958, #8677, #20792, #2706, #706, #3088, #8810, #22791, #4569, #11068, #17177, #18791, #7071, #14789, #15185, #23311, #13192, #22919, #4698, #12801, #19815, #1602, #13818, #21687, #21950 ),
 ( #3587, #5329, #13437, #23935, #3726, #23555, #19947, #7567, #15810, #17810, #7440, #5587, #11692, #13313, #19554, #19431, #9705, #25956, #13561, #1217, #5712, #21559, #15554, #21433, #7699, #1731, #5209, #11314, #11829, #9840 ),
 ( #7190, #17680, #25568, #3333, #23679, #1342, #5458, #17944, #3206, #21815, #15306, #9320, #23433, #3462, #11559, #19680, #13693, #17428, #23805, #7314, #25822, #15428, #11433, #9447, #17552, #25690, #1469, #9572, #15680, #22223 ),
 ( #3863, #2764, #14849, #22090, #26090, #12230, #16222, #13956, #3999, #11966, #8101, #10238, #129, #18349, #18079, #5985, #20354, #2130, #7826, #18207, #14223, #1998, #12098, #24074, #20090, #10367, #20486, #1869, #26230, #14359 ),
 ( #18478, #4138, #5850, #12865, #16490, #14094, #24351, #7965, #9972, #20983, #10105, #8233, #24615, #20222, #6737, #16351, #24484, #10873, #22983, #6246, #15944, #2260, #12356, #16084, #22488, #24213, #4268, #259, #6115, #22361 ) ),
 .UNSPECIFIED., .T., .F., .F. ) 
 B_SPLINE_SURFACE_WITH_KNOTS ( ( 4, 3, 4 ),
 ( 4, 2, 2, 2, 2, 2, 2, 2, 2, 2, 2, 2, 2, 2, 4 ),
 ( 0.000000000000000000, 0.5000000000000000000, 1.000000000000000000 ),
 ( 0.000000000000000000, 0.1357259735107005372, 0.1651108541090157700, 0.1944957347073310028, 0.3598804999793158710, 0.3867117631979620773, 0.4135430264166082281, 0.5789277916885930964, 0.6062785021374117456, 0.6336292125862302838, 0.8508620842112317728, 0.8814014469398914198, 0.9119408096685510667, 0.9559704048342755334, 1.000000000000000000 ),
 .UNSPECIFIED. ) 
 GEOMETRIC_REPRESENTATION_ITEM ( )  RATIONAL_B_SPLINE_SURFACE ( (
 ( 1.000000000000000000, 1.000000000000000000, 1.000000000000000000, 1.000000000000000000, 1.000000000000000000, 1.000000000000000000, 1.000000000000000000, 1.000000000000000000, 1.000000000000000000, 1.000000000000000000, 1.000000000000000000, 1.000000000000000000, 1.000000000000000000, 1.000000000000000000, 1.000000000000000000, 1.000000000000000000, 1.000000000000000000, 1.000000000000000000, 1.000000000000000000, 1.000000000000000000, 1.000000000000000000, 1.000000000000000000, 1.000000000000000000, 1.000000000000000000, 1.000000000000000000, 1.000000000000000000, 1.000000000000000000, 1.000000000000000000, 1.000000000000000000, 1.000000000000000000),
 ( 0.3333333333333333703, 0.3333333333333333703, 0.3333333333333333703, 0.3333333333333333703, 0.3333333333333333703, 0.3333333333333333703, 0.3333333333333333703, 0.3333333333333333703, 0.3333333333333333703, 0.3333333333333333703, 0.3333333333333333703, 0.3333333333333333703, 0.3333333333333333703, 0.3333333333333333703, 0.3333333333333333703, 0.3333333333333333703, 0.3333333333333333703, 0.3333333333333333703, 0.3333333333333333703, 0.3333333333333333703, 0.3333333333333333703, 0.3333333333333333703, 0.3333333333333333703, 0.3333333333333333703, 0.3333333333333333703, 0.3333333333333333703, 0.3333333333333333703, 0.3333333333333333703, 0.3333333333333333703, 0.3333333333333333703),
 ( 0.3333333333333333703, 0.3333333333333333703, 0.3333333333333333703, 0.3333333333333333703, 0.3333333333333333703, 0.3333333333333333703, 0.3333333333333333703, 0.3333333333333333703, 0.3333333333333333703, 0.3333333333333333703, 0.3333333333333333703, 0.3333333333333333703, 0.3333333333333333703, 0.3333333333333333703, 0.3333333333333333703, 0.3333333333333333703, 0.3333333333333333703, 0.3333333333333333703, 0.3333333333333333703, 0.3333333333333333703, 0.3333333333333333703, 0.3333333333333333703, 0.3333333333333333703, 0.3333333333333333703, 0.3333333333333333703, 0.3333333333333333703, 0.3333333333333333703, 0.3333333333333333703, 0.3333333333333333703, 0.3333333333333333703),
 ( 1.000000000000000000, 1.000000000000000000, 1.000000000000000000, 1.000000000000000000, 1.000000000000000000, 1.000000000000000000, 1.000000000000000000, 1.000000000000000000, 1.000000000000000000, 1.000000000000000000, 1.000000000000000000, 1.000000000000000000, 1.000000000000000000, 1.000000000000000000, 1.000000000000000000, 1.000000000000000000, 1.000000000000000000, 1.000000000000000000, 1.000000000000000000, 1.000000000000000000, 1.000000000000000000, 1.000000000000000000, 1.000000000000000000, 1.000000000000000000, 1.000000000000000000, 1.000000000000000000, 1.000000000000000000, 1.000000000000000000, 1.000000000000000000, 1.000000000000000000),
 ( 0.3333333333333333703, 0.3333333333333333703, 0.3333333333333333703, 0.3333333333333333703, 0.3333333333333333703, 0.3333333333333333703, 0.3333333333333333703, 0.3333333333333333703, 0.3333333333333333703, 0.3333333333333333703, 0.3333333333333333703, 0.3333333333333333703, 0.3333333333333333703, 0.3333333333333333703, 0.3333333333333333703, 0.3333333333333333703, 0.3333333333333333703, 0.3333333333333333703, 0.3333333333333333703, 0.3333333333333333703, 0.3333333333333333703, 0.3333333333333333703, 0.3333333333333333703, 0.3333333333333333703, 0.3333333333333333703, 0.3333333333333333703, 0.3333333333333333703, 0.3333333333333333703, 0.3333333333333333703, 0.3333333333333333703),
 ( 0.3333333333333333703, 0.3333333333333333703, 0.3333333333333333703, 0.3333333333333333703, 0.3333333333333333703, 0.3333333333333333703, 0.3333333333333333703, 0.3333333333333333703, 0.3333333333333333703, 0.3333333333333333703, 0.3333333333333333703, 0.3333333333333333703, 0.3333333333333333703, 0.3333333333333333703, 0.3333333333333333703, 0.3333333333333333703, 0.3333333333333333703, 0.3333333333333333703, 0.3333333333333333703, 0.3333333333333333703, 0.3333333333333333703, 0.3333333333333333703, 0.3333333333333333703, 0.3333333333333333703, 0.3333333333333333703, 0.3333333333333333703, 0.3333333333333333703, 0.3333333333333333703, 0.3333333333333333703, 0.3333333333333333703),
 ( 1.000000000000000000, 1.000000000000000000, 1.000000000000000000, 1.000000000000000000, 1.000000000000000000, 1.000000000000000000, 1.000000000000000000, 1.000000000000000000, 1.000000000000000000, 1.000000000000000000, 1.000000000000000000, 1.000000000000000000, 1.000000000000000000, 1.000000000000000000, 1.000000000000000000, 1.000000000000000000, 1.000000000000000000, 1.000000000000000000, 1.000000000000000000, 1.000000000000000000, 1.000000000000000000, 1.000000000000000000, 1.000000000000000000, 1.000000000000000000, 1.000000000000000000, 1.000000000000000000, 1.000000000000000000, 1.000000000000000000, 1.000000000000000000, 1.000000000000000000) ) ) 
 REPRESENTATION_ITEM ( '' )  SURFACE ( )  );
#13191=CARTESIAN_POINT ( 'NONE',  ( -138.9613193423076325, 13.65853114841885407, -27.95779829447911169 ) ) ;
#13192=CARTESIAN_POINT ( 'NONE',  ( 130.8568914410475088, -24.07718906446910623, 32.49135343045471558 ) ) ;
#13193=CARTESIAN_POINT ( 'NONE',  ( -86.96347745069644475, -15.38646221621786125, -15.38646221621789856 ) ) ;
#13194=CARTESIAN_POINT ( 'NONE',  ( 184.8905102610680444, 39.99999999999999289, 19.07866798485573057 ) ) ;
#13195=CARTESIAN_POINT ( 'NONE',  ( 7.307793755307396388, -14.18010697691874711, 49.33439594495636982 ) ) ;
#13196=DIRECTION ( 'NONE',  ( 0.9698969544411757404, 0.2249791741486417418, -0.09318942517865014263 ) ) ;
#13198=CARTESIAN_POINT ( 'NONE',  ( 192.4448373802101173, -39.99999999999977973, -19.99999999996102673 ) ) ;
#13199=CARTESIAN_POINT ( 'NONE',  ( -135.8532207217289738, 40.00000000000031974, -30.84685318188603986 ) ) ;
#13201=CARTESIAN_POINT ( 'NONE',  ( 170.2234770963711128, -10.92277846919171935, -45.64576402573189995 ) ) ;
#13202=CARTESIAN_POINT ( 'NONE',  ( -200.0000000000000853, 24.32899771311817716, -44.86773131993646757 ) ) ;
#13203=CARTESIAN_POINT ( 'NONE',  ( -193.3669111531647218, 18.32287347112285048, 44.23532963563830833 ) ) ;
#13204=CARTESIAN_POINT ( 'NONE',  ( 130.8888609958234781, 29.49786752803534995, 12.21841679119730273 ) ) ;
#13207=CARTESIAN_POINT ( 'NONE',  ( -188.2995950289364941, -43.00522595870984333, 23.44932284465888728 ) ) ;
#13208=CARTESIAN_POINT ( 'NONE',  ( -77.72621512577178748, 21.21705881579131514, -5.759696801490011175 ) ) ;
#13209=CARTESIAN_POINT ( 'NONE',  ( -105.3755690713226585, -12.89780903124444578, 43.67073346367968156 ) ) ;
#13212=ORIENTED_EDGE ( 'NONE', *, *, #12057, .F. ) ;
#13213=CARTESIAN_POINT ( 'NONE',  ( -86.96347745069644475, 12.89780903124419353, -12.89780903124389333 ) ) ;
#13215=CARTESIAN_POINT ( 'NONE',  ( 169.9999999999999432, 21.59613885783095810, -12.70659020859094568 ) ) ;
#13216=EDGE_LOOP ( 'NONE', ( #13120, #11732, #22584, #18383, #598, #3072 ) ) ;
#13217=CARTESIAN_POINT ( 'NONE',  ( -135.8532207217289738, -1.208299557080134822E-13, 9.153146818113572891 ) ) ;
#13223=VERTEX_POINT ( 'NONE', #4709 ) ;
#13225=CARTESIAN_POINT ( 'NONE',  ( -198.0356074513804572, 55.37879056873070027, 2.449293598294708485E-15 ) ) ;
#13226=CARTESIAN_POINT ( 'NONE',  ( -99.31364972218659659, -20.79869444141380086, -8.164808577121105415 ) ) ;
#13229=CARTESIAN_POINT ( 'NONE',  ( 151.7948205124836534, -39.99999999999987921, -33.23291073765567916 ) ) ;
#13232=CARTESIAN_POINT ( 'NONE',  ( -82.26522586992982156, 10.29063887125004939, 17.41030175917899214 ) ) ;
#13234=CARTESIAN_POINT ( 'NONE',  ( 192.4448373802100889, -14.14213562375896061, 14.14213562375865330 ) ) ;
#13235=CARTESIAN_POINT ( 'NONE',  ( -105.3755690713226585, 43.67073346367988051, -12.89780903124366418 ) ) ;
#13236=CARTESIAN_POINT ( 'NONE',  ( 151.7948205124836534, -39.99999999999992184, -6.767089262349454515 ) ) ;
#13237=CARTESIAN_POINT ( 'NONE',  ( -105.2054292635175585, -21.49321519473986442, -7.030298963786045751E-29 ) ) ;
#13238=CARTESIAN_POINT ( 'NONE',  ( 192.4448373802101173, 20.00000000003945644, -40.00000000000002132 ) ) ;
#13239=CARTESIAN_POINT ( 'NONE',  ( 192.4448373802101173, -42.42640687116490028, -14.14213562375904942 ) ) ;
#13240=CARTESIAN_POINT ( 'NONE',  ( -105.3755690713226585, -18.24025645688353947, -40.00000000000002132 ) ) ;
#13241=CARTESIAN_POINT ( 'NONE',  ( 23.09861257792924505, -42.94075326233385681, -23.40165480222905003 ) ) ;
#13242=CARTESIAN_POINT ( 'NONE',  ( -86.96347745069645896, 40.00000000000008527, -21.75974354311636461 ) ) ;
#13243=CARTESIAN_POINT ( 'NONE',  ( 57.59792236341147031, -2.435789363418150000, -40.00000000000002132 ) ) ;
#13244=CARTESIAN_POINT ( 'NONE',  ( 192.4448373802101173, -14.14213562375886291, 42.42640687116498555 ) ) ;
#13246=CARTESIAN_POINT ( 'NONE',  ( -56.48582580120559982, 30.84685318188643777, -40.00000000000002132 ) ) ;
#13248=CARTESIAN_POINT ( 'NONE',  ( 19.94008347559386962, -47.92933869853446538, 13.96811062197253328 ) ) ;
#13250=CARTESIAN_POINT ( 'NONE',  ( -105.2054292635176154, 15.67883240740060735, -14.71716402000391888 ) ) ;
#13251=CARTESIAN_POINT ( 'NONE',  ( 136.1360204305621551, -24.77266263493126885, 31.79587985999256006 ) ) ;
#13252=CARTESIAN_POINT ( 'NONE',  ( -86.96347745069643054, -39.99999999999995737, -21.75974354311664527 ) ) ;
#13253=CARTESIAN_POINT ( 'NONE',  ( -77.64097821994924686, 21.67328794148362192, 4.107454262294036873 ) ) ;
#13254=CARTESIAN_POINT ( 'NONE',  ( -70.30307074938296807, 10.20829450409786254, -22.52851052403980958 ) ) ;
#13257=CARTESIAN_POINT ( 'NONE',  ( 190.0000000000001137, 3.490243377569959927E-14, 0.000000000000000000 ) ) ;
#13258=CARTESIAN_POINT ( 'NONE',  ( 136.1360204305621551, 3.511608612530062512, 53.05693388239318864 ) ) ;
#13259=CARTESIAN_POINT ( 'NONE',  ( 151.7948205124835681, 51.78348778862544322, -4.785054706298002891 ) ) ;
#13260=CARTESIAN_POINT ( 'NONE',  ( -86.96347745069643054, 15.38646221621763210, 41.18208027870604582 ) ) ;
#13261=DIRECTION ( 'NONE',  ( 1.053136113562458437E-14, 0.7071067811865507924, -0.7071067811865442421 ) ) ;
#13262=CARTESIAN_POINT ( 'NONE',  ( -100.7734535825088500, 44.31723036834907958, -12.25131212657445801 ) ) ;
#13264=CARTESIAN_POINT ( 'NONE',  ( 163.1118516004056573, 47.56205970284970164, -9.006482792073828847 ) ) ;
#13265=CARTESIAN_POINT ( 'NONE',  ( 0.2972598230769990524, -18.14793986248671231, -38.42060263243687501 ) ) ;
#13266=CARTESIAN_POINT ( 'NONE',  ( 163.1118516004056573, 9.006482792069759213, -9.006482792069505194 ) ) ;
#13267=CARTESIAN_POINT ( 'NONE',  ( -162.0762913951021176, 1.694272876828294194, -40.00000000000002132 ) ) ;
#13268=CARTESIAN_POINT ( 'NONE',  ( 146.6084372240433993, -24.48358557860319706, -24.48358557860330720 ) ) ;
#13269=CARTESIAN_POINT ( 'NONE',  ( -162.0762913951020892, -3.568845385355699554E-14, 1.694272876828323948 ) ) ;
#13270=CARTESIAN_POINT ( 'NONE',  ( -30.26275506840324070, -29.48230279907817675, 27.08623969584564151 ) ) ;
#13271=CARTESIAN_POINT ( 'NONE',  ( -183.6284948306513911, 41.87131864457176533, -17.34366805702960335 ) ) ;
#13272=EDGE_LOOP ( 'NONE', ( #8139, #7895, #17082, #5614 ) ) ;
#13273=CARTESIAN_POINT ( 'NONE',  ( 130.8568914410475088, 32.49135343045483637, -24.07718906446901030 ) ) ;
#13274=CARTESIAN_POINT ( 'NONE',  ( -94.58366989427311466, -20.91926462023915079, -8.190486896679153972 ) ) ;
#13275=CARTESIAN_POINT ( 'NONE',  ( 12.96694272570746698, 24.77464205076635295, 44.79869582452549537 ) ) ;
#13276=CARTESIAN_POINT ( 'NONE',  ( -7.297127544325032744, -42.04314499753751022, -22.81351773421616258 ) ) ;
#13277=ORIENTED_EDGE ( 'NONE', *, *, #7756, .F. ) ;
#13278=CARTESIAN_POINT ( 'NONE',  ( -188.2506440019715797, -46.97351617221517017, 13.82466072834922244 ) ) ;
#13280=CARTESIAN_POINT ( 'NONE',  ( 60.28378959949315430, -10.93033916072590372, 33.17072922783161459 ) ) ;
#13281=CARTESIAN_POINT ( 'NONE',  ( 98.29820294267324243, 7.653668647304274764, -18.47759065023114999 ) ) ;
#13284=CARTESIAN_POINT ( 'NONE',  ( -77.78698619430412009, -6.810291944262315766, 20.89067062964120680 ) ) ;
#13285=CARTESIAN_POINT ( 'NONE',  ( -91.56559293963834989, 6.234561990864368500E-14, -22.67402823373191723 ) ) ;
#13286=CARTESIAN_POINT ( 'NONE',  ( -77.78738361196433004, -6.814606408068145882, 20.88860503098718979 ) ) ;
#13287=CARTESIAN_POINT ( 'NONE',  ( -199.9999999999999716, -19.51623549979280980, -45.81998439131055534 ) ) ;
#13288=CARTESIAN_POINT ( 'NONE',  ( -208.1127848780264742, -55.00245453014425578, -40.00000000000002132 ) ) ;
#13289=CARTESIAN_POINT ( 'NONE',  ( 17.65190074000733844, -14.05440436230720636, -48.50354960736758159 ) ) ;
#13291=CARTESIAN_POINT ( 'NONE',  ( -91.56559293963836410, 22.67402823373190301, 40.00000000000002132 ) ) ;
#13292=CARTESIAN_POINT ( 'NONE',  ( 146.6084372240433993, 24.48358557860341733, -24.48358557860313311 ) ) ;
#13293=CARTESIAN_POINT ( 'NONE',  ( 4.995406935893291767, 40.00000000000059686, -55.24977328853165659 ) ) ;
#13294=CARTESIAN_POINT ( 'NONE',  ( 192.4448373802100889, 2.472897170449861688E-13, -19.99999999996060751 ) ) ;
#13297=ORIENTED_EDGE ( 'NONE', *, *, #22659, .T. ) ;
#13299=CARTESIAN_POINT ( 'NONE',  ( 16.10036699868000554, 44.47262139758795030, -24.53427828610321271 ) ) ;
#13300=CARTESIAN_POINT ( 'NONE',  ( -91.56559293963834989, -17.32597176626812896, 40.00000000000002132 ) ) ;
#13303=CARTESIAN_POINT ( 'NONE',  ( -197.6434631109478346, 44.74794079767860921, -18.53520396667194703 ) ) ;
#13307=CARTESIAN_POINT ( 'NONE',  ( -198.0356074513804572, -10.87444709759729911, 10.87444709759714812 ) ) ;
#13313=CARTESIAN_POINT ( 'NONE',  ( -56.48582580120559271, 21.81201906317768291, 21.81201906317777173 ) ) ;
#13314=CARTESIAN_POINT ( 'NONE',  ( -121.8425463770985573, -22.74408395592868004, -9.420908036270656538 ) ) ;
#13315=CARTESIAN_POINT ( 'NONE',  ( -259.2033419157646676, -40.00000000000003553, -9.517827891722768996 ) ) ;
#13316=CARTESIAN_POINT ( 'NONE',  ( -189.2428623074475524, -23.64699222226070674, 43.27185639470918233 ) ) ;
#13318=CARTESIAN_POINT ( 'NONE',  ( 170.2234770963711128, -39.99999999999982947, -15.44714144992858529 ) ) ;
#13319=CARTESIAN_POINT ( 'NONE',  ( 146.6084372240433709, 40.00000000000010658, -5.374981219216549810 ) ) ;
#13320=CARTESIAN_POINT ( 'NONE',  ( -86.93850585862767844, 19.24776704638164659, 9.367985447339783889 ) ) ;
#13321=CARTESIAN_POINT ( 'NONE',  ( 4.995406935893293543, -10.78321810389005364, 10.78321810388994173 ) ) ;
#13322=CARTESIAN_POINT ( 'NONE',  ( -135.8532207217289738, 7.002209520526292428E-15, -9.153146818113572891 ) ) ;
#13323=CARTESIAN_POINT ( 'NONE',  ( -192.6562840316549341, 18.27409180090459628, 44.11756026579762846 ) ) ;
#13324=CARTESIAN_POINT ( 'NONE',  ( 125.5832160019860737, 28.05309928653993978, 11.61997419108395846 ) ) ;
#13326=CARTESIAN_POINT ( 'NONE',  ( 130.8568914410475088, 52.36146031193420924, 4.207082182989907437 ) ) ;
#13327=CARTESIAN_POINT ( 'NONE',  ( -87.11138134867678673, -17.02212146154200312, 13.16760794720353189 ) ) ;
#13328=CARTESIAN_POINT ( 'NONE',  ( -86.96347745069644475, -43.67073346367983788, 12.89780903124397149 ) ) ;
#13329=CARTESIAN_POINT ( 'NONE',  ( 4.995406935893305977, -39.06748935135157552, -39.06748935135225764 ) ) ;
#13330=FACE_OUTER_BOUND ( 'NONE', #19546, .T. ) ;
#13331=CARTESIAN_POINT ( 'NONE',  ( -105.4741150117390021, -7.943527260764932763, -19.77569912954469800 ) ) ;
#13332=VERTEX_POINT ( 'NONE', #21061 ) ;
#13333=CARTESIAN_POINT ( 'NONE',  ( 14.38125909742181463, 10.73282306403652875, -67.30136555895941797 ) ) ;
#13335=( BOUNDED_SURFACE ( )  B_SPLINE_SURFACE ( 3, 3, ( 
 ( #18505, #286, #24642, #6398, #18641, #22646, #16646, #4420, #22093, #18352, #24354, #20225, #14362, #2003, #10109, #25959, #132, #1734, #8236, #20093, #5716, #22226, #4142, #7702, #16354, #21955, #10241, #3729, #3213, #24487 ),
 ( #18210, #8104, #16225, #9843, #15948, #4002, #12101, #9708, #1872, #24217, #11969, #13959, #15813, #13821, #20358, #6249, #17813, #14097, #24079, #18083, #23939, #2133, #6118, #4271, #9975, #26234, #22492, #14226, #11832, #7968 ),
 ( #22365, #17947, #12359, #16087, #12234, #5988, #20490, #19950, #26094, #5853, #3867, #7830, #22751, #15017, #2263, #8771, #6636, #18481, #14750, #8371, #20887, #18750, #16748, #22623, #6372, #262, #14882, #4530, #533, #20755 ),
 ( #24880, #25016, #402, #12898, #4659, #23147, #2525, #12628, #25149, #22881, #16493, #10642, #8638, #12762, #2666, #20617, #17012, #10771, #23021, #18884, #662, #4398, #24618, #16619, #24752, #8902, #16885, #4919, #10371, #6770 ),
 ( #6506, #13032, #14616, #4797, #21013, #18619, #14490, #2795, #6900, #12492, #10907, #19019, #798, #2393, #10505, #8505, #19623, #1408, #11902, #9908, #11495, #7903, #21883, #3798, #5786, #21752, #19886, #17879, #927, #7507 ),
 ( #11033, #13627, #25759, #25276, #5923, #9509, #3526, #15617, #7026, #17747, #23740, #13157, #16022, #19143, #5521, #21150, #5650, #21277, #17614, #11627, #19749, #1539, #9037, #17142, #15145, #26028, #23275, #24147, #9644, #25889 ),
 ( #20027, #3397, #1805, #7631, #5051, #15745, #15878, #23874, #18014, #13755, #22027, #3660, #11768, #26162, #1670, #9778, #2924, #7765, #24006, #13893, #1937, #14031, #24290, #14429, #6182, #6310, #10313, #10178, #18556, #22559 ) ),
 .UNSPECIFIED., .T., .F., .F. ) 
 B_SPLINE_SURFACE_WITH_KNOTS ( ( 4, 3, 4 ),
 ( 4, 2, 2, 2, 2, 2, 2, 2, 2, 2, 2, 2, 2, 2, 4 ),
 ( 0.000000000000000000, 0.5000000000000000000, 1.000000000000000000 ),
 ( 0.000000000000000000, 0.1357259735107005372, 0.1651108541090157700, 0.1944957347073310028, 0.3598804999793158710, 0.3867117631979620773, 0.4135430264166082281, 0.5789277916885930964, 0.6062785021374117456, 0.6336292125862302838, 0.8508620842112317728, 0.8814014469398914198, 0.9119408096685510667, 0.9559704048342755334, 1.000000000000000000 ),
 .UNSPECIFIED. ) 
 GEOMETRIC_REPRESENTATION_ITEM ( )  RATIONAL_B_SPLINE_SURFACE ( (
 ( 1.000000000000000000, 1.000000000000000000, 1.000000000000000000, 1.000000000000000000, 1.000000000000000000, 1.000000000000000000, 1.000000000000000000, 1.000000000000000000, 1.000000000000000000, 1.000000000000000000, 1.000000000000000000, 1.000000000000000000, 1.000000000000000000, 1.000000000000000000, 1.000000000000000000, 1.000000000000000000, 1.000000000000000000, 1.000000000000000000, 1.000000000000000000, 1.000000000000000000, 1.000000000000000000, 1.000000000000000000, 1.000000000000000000, 1.000000000000000000, 1.000000000000000000, 1.000000000000000000, 1.000000000000000000, 1.000000000000000000, 1.000000000000000000, 1.000000000000000000),
 ( 0.3333333333333333703, 0.3333333333333333703, 0.3333333333333333703, 0.3333333333333333703, 0.3333333333333333703, 0.3333333333333333703, 0.3333333333333333703, 0.3333333333333333703, 0.3333333333333333703, 0.3333333333333333703, 0.3333333333333333703, 0.3333333333333333703, 0.3333333333333333703, 0.3333333333333333703, 0.3333333333333333703, 0.3333333333333333703, 0.3333333333333333703, 0.3333333333333333703, 0.3333333333333333703, 0.3333333333333333703, 0.3333333333333333703, 0.3333333333333333703, 0.3333333333333333703, 0.3333333333333333703, 0.3333333333333333703, 0.3333333333333333703, 0.3333333333333333703, 0.3333333333333333703, 0.3333333333333333703, 0.3333333333333333703),
 ( 0.3333333333333333703, 0.3333333333333333703, 0.3333333333333333703, 0.3333333333333333703, 0.3333333333333333703, 0.3333333333333333703, 0.3333333333333333703, 0.3333333333333333703, 0.3333333333333333703, 0.3333333333333333703, 0.3333333333333333703, 0.3333333333333333703, 0.3333333333333333703, 0.3333333333333333703, 0.3333333333333333703, 0.3333333333333333703, 0.3333333333333333703, 0.3333333333333333703, 0.3333333333333333703, 0.3333333333333333703, 0.3333333333333333703, 0.3333333333333333703, 0.3333333333333333703, 0.3333333333333333703, 0.3333333333333333703, 0.3333333333333333703, 0.3333333333333333703, 0.3333333333333333703, 0.3333333333333333703, 0.3333333333333333703),
 ( 1.000000000000000000, 1.000000000000000000, 1.000000000000000000, 1.000000000000000000, 1.000000000000000000, 1.000000000000000000, 1.000000000000000000, 1.000000000000000000, 1.000000000000000000, 1.000000000000000000, 1.000000000000000000, 1.000000000000000000, 1.000000000000000000, 1.000000000000000000, 1.000000000000000000, 1.000000000000000000, 1.000000000000000000, 1.000000000000000000, 1.000000000000000000, 1.000000000000000000, 1.000000000000000000, 1.000000000000000000, 1.000000000000000000, 1.000000000000000000, 1.000000000000000000, 1.000000000000000000, 1.000000000000000000, 1.000000000000000000, 1.000000000000000000, 1.000000000000000000),
 ( 0.3333333333333333703, 0.3333333333333333703, 0.3333333333333333703, 0.3333333333333333703, 0.3333333333333333703, 0.3333333333333333703, 0.3333333333333333703, 0.3333333333333333703, 0.3333333333333333703, 0.3333333333333333703, 0.3333333333333333703, 0.3333333333333333703, 0.3333333333333333703, 0.3333333333333333703, 0.3333333333333333703, 0.3333333333333333703, 0.3333333333333333703, 0.3333333333333333703, 0.3333333333333333703, 0.3333333333333333703, 0.3333333333333333703, 0.3333333333333333703, 0.3333333333333333703, 0.3333333333333333703, 0.3333333333333333703, 0.3333333333333333703, 0.3333333333333333703, 0.3333333333333333703, 0.3333333333333333703, 0.3333333333333333703),
 ( 0.3333333333333333703, 0.3333333333333333703, 0.3333333333333333703, 0.3333333333333333703, 0.3333333333333333703, 0.3333333333333333703, 0.3333333333333333703, 0.3333333333333333703, 0.3333333333333333703, 0.3333333333333333703, 0.3333333333333333703, 0.3333333333333333703, 0.3333333333333333703, 0.3333333333333333703, 0.3333333333333333703, 0.3333333333333333703, 0.3333333333333333703, 0.3333333333333333703, 0.3333333333333333703, 0.3333333333333333703, 0.3333333333333333703, 0.3333333333333333703, 0.3333333333333333703, 0.3333333333333333703, 0.3333333333333333703, 0.3333333333333333703, 0.3333333333333333703, 0.3333333333333333703, 0.3333333333333333703, 0.3333333333333333703),
 ( 1.000000000000000000, 1.000000000000000000, 1.000000000000000000, 1.000000000000000000, 1.000000000000000000, 1.000000000000000000, 1.000000000000000000, 1.000000000000000000, 1.000000000000000000, 1.000000000000000000, 1.000000000000000000, 1.000000000000000000, 1.000000000000000000, 1.000000000000000000, 1.000000000000000000, 1.000000000000000000, 1.000000000000000000, 1.000000000000000000, 1.000000000000000000, 1.000000000000000000, 1.000000000000000000, 1.000000000000000000, 1.000000000000000000, 1.000000000000000000, 1.000000000000000000, 1.000000000000000000, 1.000000000000000000, 1.000000000000000000, 1.000000000000000000, 1.000000000000000000) ) ) 
 REPRESENTATION_ITEM ( '' )  SURFACE ( )  );
#13340=CARTESIAN_POINT ( 'NONE',  ( -4.039451493210483690, -43.00522595894025812, 23.44932283416647323 ) ) ;
#13341=ORIENTED_EDGE ( 'NONE', *, *, #16052, .F. ) ;
#13342=ORIENTED_EDGE ( 'NONE', *, *, #3013, .F. ) ;
#13343=CARTESIAN_POINT ( 'NONE',  ( -198.0356074513804572, -39.15871834505905724, -17.40982414986491733 ) ) ;
#13344=CARTESIAN_POINT ( 'NONE',  ( 130.8568914410475088, 40.00000000000015632, -34.05028731879774284 ) ) ;
#13348=CARTESIAN_POINT ( 'NONE',  ( -162.0762913951020892, -3.568845385355699554E-14, 1.694272876828323948 ) ) ;
#13350=CARTESIAN_POINT ( 'NONE',  ( -87.13361725327074225, 15.19799821270826179, 15.19799821270854245 ) ) ;
#13351=CARTESIAN_POINT ( 'NONE',  ( -6.342283169554272959, -13.66521761902986754, -46.19215417243526645 ) ) ;
#13352=CARTESIAN_POINT ( 'NONE',  ( 57.59792236341148453, 1.722363176415528940, -54.84617931850878136 ) ) ;
#13353=CARTESIAN_POINT ( 'NONE',  ( -105.2502153031284422, -21.20171025720616953, 3.401878988847722329 ) ) ;
#13354=CARTESIAN_POINT ( 'NONE',  ( -208.1127848780264742, -39.99999999999948841, -55.00245453010965235 ) ) ;
#13355=CARTESIAN_POINT ( 'NONE',  ( 35.93702929138175506, 12.87541766509833785, 42.26928858764885177 ) ) ;
#13356=CARTESIAN_POINT ( 'NONE',  ( 57.59792236341148453, -37.56421063658185489, 40.00000000000002132 ) ) ;
#13357=CARTESIAN_POINT ( 'NONE',  ( -238.4067589809705794, -40.96449427990185654, -40.00000000000002132 ) ) ;
#13358=CARTESIAN_POINT ( 'NONE',  ( -105.3755690713226585, 43.67073346367970288, 12.89780903124427702 ) ) ;
#13359=CARTESIAN_POINT ( 'NONE',  ( 146.6084372240433993, 34.62501878078308692, 0.000000000000000000 ) ) ;
#13361=CARTESIAN_POINT ( 'NONE',  ( 163.1118516004056573, 40.00000000000014921, -27.26290988616858968 ) ) ;
#13363=CARTESIAN_POINT ( 'NONE',  ( 136.1360204305621551, 31.79587985999267374, -24.77266263493117293 ) ) ;
#13364=CARTESIAN_POINT ( 'NONE',  ( 184.8905102610680444, 19.07866798485561333, 40.00000000000002132 ) ) ;
#13366=CARTESIAN_POINT ( 'NONE',  ( 22.77497178454860816, -43.17449153292918851, 17.88345994150142815 ) ) ;
#13367=CARTESIAN_POINT ( 'NONE',  ( -105.2054292635175869, 15.19799821370233062, -15.19799821370219206 ) ) ;
#13369=CARTESIAN_POINT ( 'NONE',  ( -86.96347745069644475, 12.89780903124401057, 12.89780903124407629 ) ) ;
#13370=CARTESIAN_POINT ( 'NONE',  ( -259.2033419157646676, -40.00000000000003553, -9.517827891722768996 ) ) ;
#13371=CARTESIAN_POINT ( 'NONE',  ( -87.04641387366682181, 20.92787283706964985, -4.638221027435098343 ) ) ;
#13374=EDGE_CURVE ( 'NONE', #11522, #16316, #11098, .T. ) ;
#13375=CARTESIAN_POINT ( 'NONE',  ( -82.23726319249649919, -20.19517362732916510, -9.977985540125270190E-16 ) ) ;
#13377=CARTESIAN_POINT ( 'NONE',  ( -87.12812962371036463, 1.358531488422078937, -21.45735542732301226 ) ) ;
#13378=CARTESIAN_POINT ( 'NONE',  ( 184.8905102610680444, -14.79361573936399665, 14.79361573936367158 ) ) ;
#13379=CARTESIAN_POINT ( 'NONE',  ( -213.1075012329536946, -37.98287015391210275, -37.98287015391272092 ) ) ;
#13380=CARTESIAN_POINT ( 'NONE',  ( 14.38125909742181996, -10.73282306403606157, 67.30136555895948902 ) ) ;
#13382=CARTESIAN_POINT ( 'NONE',  ( -213.1075012329536946, -37.98287015391210275, -37.98287015391272092 ) ) ;
#13383=CARTESIAN_POINT ( 'NONE',  ( -105.3755690713226585, 15.38646221621820764, -41.18208027870583265 ) ) ;
#13384=CARTESIAN_POINT ( 'NONE',  ( -238.4067589809705794, -27.60227080167029001, -28.96627169325357798 ) ) ;
#13385=CARTESIAN_POINT ( 'NONE',  ( -135.8532207217289738, -6.472252184283586729, -50.09629031063973770 ) ) ;
#13388=CARTESIAN_POINT ( 'NONE',  ( 0.2972598230769957217, -4.999556039334937811E-14, 14.33493731733933352 ) ) ;
#13390=CARTESIAN_POINT ( 'NONE',  ( 184.8905102610680444, -13.49065550809840630, 43.07788698682565354 ) ) ;
#13391=CONICAL_SURFACE ( 'NONE', #17213, 60.00000000000009948, 0.7853981633974479459 ) ;
#13392=CARTESIAN_POINT ( 'NONE',  ( 57.59792236341147031, 37.56421063658187620, 40.00000000000002132 ) ) ;
#13394=CARTESIAN_POINT ( 'NONE',  ( -56.48582580120559982, 21.81201906317778594, -34.75652343174606074 ) ) ;
#13395=CARTESIAN_POINT ( 'NONE',  ( -86.86493150571111244, -19.60045294882784717, -8.366608963953344968 ) ) ;
#13396=CARTESIAN_POINT ( 'NONE',  ( 36.66494225440861499, 16.22659705908689531, 39.17447069130953707 ) ) ;
#13399=CARTESIAN_POINT ( 'NONE',  ( -188.8753211508388006, -43.29880796194907333, 17.93495349242729375 ) ) ;
#13402=CARTESIAN_POINT ( 'NONE',  ( 25.31597067608044682, -17.58652183057975193, 42.45761951829265968 ) ) ;
#13403=CARTESIAN_POINT ( 'NONE',  ( 98.29820294268672853, 20.00000000000089528, 2.652164898395847903 ) ) ;
#13408=CARTESIAN_POINT ( 'NONE',  ( -56.48582580120560692, 40.00000000000004263, -9.153146818113443217 ) ) ;
#13409=CARTESIAN_POINT ( 'NONE',  ( -77.70092821061149380, -5.501796661956294798, 21.35074465833452706 ) ) ;
#13410=CARTESIAN_POINT ( 'NONE',  ( 17.75917311731580384, 48.46615948699212595, -14.04884443869896593 ) ) ;
#13411=CARTESIAN_POINT ( 'NONE',  ( 200.0000000000000000, -19.99999999999989342, 40.00000000000002132 ) ) ;
#13412=CARTESIAN_POINT ( 'NONE',  ( -114.4364955367321528, 8.644468109209284989, -20.04994829327632999 ) ) ;
#13414=CARTESIAN_POINT ( 'NONE',  ( -100.7734535825088500, -17.32597176626813251, 40.00000000000002132 ) ) ;
#13416=CARTESIAN_POINT ( 'NONE',  ( 199.9999999999999432, 14.14213562373113398, -14.14213562373094923 ) ) ;
#13417=AXIS2_PLACEMENT_3D ( 'NONE', #14280, #1791, #24404 ) ;
#13418=CARTESIAN_POINT ( 'NONE',  ( -162.0762913951021176, 40.00000000000042633, -41.69427287672947102 ) ) ;
#13419=CARTESIAN_POINT ( 'NONE',  ( -213.1075012329537230, -39.99999999999991473, -13.71589010951953647 ) ) ;
#13420=CARTESIAN_POINT ( 'NONE',  ( 101.9643209985650003, -19.81985618488135259, -8.209653236061971171 ) ) ;
#13422=CARTESIAN_POINT ( 'NONE',  ( -16.41532015121172350, -42.70629200808449610, 12.95569205125167578 ) ) ;
#13423=CARTESIAN_POINT ( 'NONE',  ( -4.004886986944939942, 47.00296421444957673, -13.82996668233321458 ) ) ;
#13424=CARTESIAN_POINT ( 'NONE',  ( -135.8532207217289454, -30.84685318188649106, 40.00000000000002132 ) ) ;
#13426=CARTESIAN_POINT ( 'NONE',  ( -114.7826396787322665, 2.171560191748074081E-13, -22.13135001986799111 ) ) ;
#13428=ORIENTED_EDGE ( 'NONE', *, *, #16108, .T. ) ;
#13429=VERTEX_POINT ( 'NONE', #23191 ) ;
#13430=CARTESIAN_POINT ( 'NONE',  ( -102.4068193528169246, -20.17396017424864141, 8.735227608996771309 ) ) ;
#13431=CARTESIAN_POINT ( 'NONE',  ( 98.29820294273291381, -18.47759065023123526, -7.653668647304108674 ) ) ;
#13432=CARTESIAN_POINT ( 'NONE',  ( -86.86493150571111244, 7.943527260496201947, -19.77569912839169319 ) ) ;
#13437=CARTESIAN_POINT ( 'NONE',  ( -238.4067589809705794, 28.96627169325315165, 28.96627169325329731 ) ) ;
#13440=CARTESIAN_POINT ( 'NONE',  ( -192.9588430854689989, -8.596193650988133061E-14, 14.46834944099969533 ) ) ;
#13441=CARTESIAN_POINT ( 'NONE',  ( -105.4741150117383341, -8.366608964593364561, -19.60045294982747777 ) ) ;
#13442=CARTESIAN_POINT ( 'NONE',  ( -199.9999999999999147, -49.28189405767606956, -14.17215463606684267 ) ) ;
#13445=CARTESIAN_POINT ( 'NONE',  ( -86.96347745069643054, -39.99999999999985079, -18.24025645688394448 ) ) ;
#13446=CARTESIAN_POINT ( 'NONE',  ( 4.995406935893291767, 40.00000000000059686, -55.24977328853165659 ) ) ;
#13447=CARTESIAN_POINT ( 'NONE',  ( -87.13361725327069962, 15.19799821270825113, 15.19799821270852824 ) ) ;
#13448=B_SPLINE_CURVE_WITH_KNOTS ( 'NONE', 3,
 ( #11361, #3134, #19610, #19478, #13612, #1656, #25490, #11482, #1265, #21610, #25620, #21740, #3516, #7239, #5384, #13489, #15864, #3384, #17355, #19874, #9497, #17602, #25744, #13241, #7493, #11236, #9765 ),
 .UNSPECIFIED., .F., .F.,
 ( 4, 2, 1, 1, 2, 2, 2, 2, 2, 2, 2, 2, 1, 2, 4 ),
 ( -5.999999998738660203E-08, 0.0002171475752860161713, 0.0004343551505720197347, 0.0008687703011440245848, 0.001737600602288039055, 0.003475261204576066479, 0.006950582409152118724, 0.01390122481830422495, 0.02085186722745633117, 0.02432718843203238862, 0.02606484903432041561, 0.02693367933546442911, 0.02736809448603644279, 0.02758530206132244963, 0.02780250963660845301 ),
 .UNSPECIFIED. ) ;
#13449=CARTESIAN_POINT ( 'NONE',  ( 4.995406935893297984, -39.06748935135182421, -17.50105314357212549 ) ) ;
#13450=CARTESIAN_POINT ( 'NONE',  ( 57.59792236341147031, 1.908507979671054758E-14, -2.435789363418160658 ) ) ;
#13451=CARTESIAN_POINT ( 'NONE',  ( -100.7734535825088500, 16.03295912088713848, -16.03295912088698927 ) ) ;
#13452=DIRECTION ( 'NONE',  ( 0.01051738792038098801, -0.9307051272723525503, -0.3656191332798196525 ) ) ;
#13454=CARTESIAN_POINT ( 'NONE',  ( 151.7948205124835681, 51.78348778862537927, 4.785054706298732086 ) ) ;
#13455=CARTESIAN_POINT ( 'NONE',  ( 192.4448373802100889, 1.051811698935164031E-13, -20.00000000003942091 ) ) ;
#13456=CARTESIAN_POINT ( 'NONE',  ( -91.56559293963834989, -16.03295912088716335, 40.53558337403673306 ) ) ;
#13457=CARTESIAN_POINT ( 'NONE',  ( -198.0356074513804572, -67.44298959253333692, -10.87444709761016348 ) ) ;
#13459=CARTESIAN_POINT ( 'NONE',  ( 107.5473083967386572, -2.315402722108309326E-13, 23.99138244111235352 ) ) ;
#13461=CARTESIAN_POINT ( 'NONE',  ( -56.48582580120559982, -6.472252184283581400, -50.09629031063973059 ) ) ;
#13463=CARTESIAN_POINT ( 'NONE',  ( 170.0000000000000284, 6.285860131565048192, 24.25569233607182440 ) ) ;
#13465=CARTESIAN_POINT ( 'NONE',  ( 170.2234770963711128, -40.00000000000024158, 24.55285855007145202 ) ) ;
#13470=CARTESIAN_POINT ( 'NONE',  ( -100.7734535825088500, -12.25131212657462498, -44.31723036834905827 ) ) ;
#13471=CARTESIAN_POINT ( 'NONE',  ( 199.9999999999999432, -3.553951640073651008E-14, 19.99999999999992539 ) ) ;
#13472=ADVANCED_FACE ( 'NONE', ( #2966 ), #8818, .T. ) ;
#13473=CARTESIAN_POINT ( 'NONE',  ( -109.1264249741460048, 33.12752917269234132, -13.72187187123960150 ) ) ;
#13474=DIRECTION ( 'NONE',  ( 0.000000000000000000, 1.000000000000000000, 0.000000000000000000 ) ) ;
#13475=CARTESIAN_POINT ( 'NONE',  ( -259.2033419157646676, -40.00000000000017764, 30.48217210827725054 ) ) ;
#13477=CARTESIAN_POINT ( 'NONE',  ( -135.8532207217289738, 40.00000000000002842, -9.153146818113432559 ) ) ;
#13479=CARTESIAN_POINT ( 'NONE',  ( -8.720657192081592513, -22.53512351407530190, -41.62108041047272167 ) ) ;
#13480=CARTESIAN_POINT ( 'NONE',  ( 130.8568914410475088, 52.36146031193427319, -4.207082182989173802 ) ) ;
#13481=( BOUNDED_CURVE ( )  B_SPLINE_CURVE ( 3, ( #17952, #21960, #11837, #26099 ),
 .UNSPECIFIED., .F., .F. ) 
 B_SPLINE_CURVE_WITH_KNOTS ( ( 4, 4 ),
 ( 0.004183487405659398924, 0.01388163287021780198 ),
 .UNSPECIFIED. ) 
 CURVE ( )  GEOMETRIC_REPRESENTATION_ITEM ( )  RATIONAL_B_SPLINE_CURVE ( ( 0.6809743333591580239, 0.7608653435686170141, 0.8672072324488977468, 1.000000000000000000 ) ) 
 REPRESENTATION_ITEM ( '' )  );
#13482=CARTESIAN_POINT ( 'NONE',  ( 165.3321726438349515, -18.76308274332846437, 18.76308274332804160 ) ) ;
#13483=CARTESIAN_POINT ( 'NONE',  ( -162.0762913951020892, 4.094006889353306706E-13, -41.69427287682835015 ) ) ;
#13485=CARTESIAN_POINT ( 'NONE',  ( -208.1127848780264742, -15.00245453012673202, 40.00000000000002132 ) ) ;
#13486=CARTESIAN_POINT ( 'NONE',  ( -105.3755690713226585, 21.75974354311648185, -40.00000000000002132 ) ) ;
#13487=CARTESIAN_POINT ( 'NONE',  ( 200.0000000000000000, 42.42640687119290988, 14.14213562373111976 ) ) ;
#13488=CARTESIAN_POINT ( 'NONE',  ( 199.9999999999999432, 20.00000000000013856, 0.000000000000000000 ) ) ;
#13489=CARTESIAN_POINT ( 'NONE',  ( 17.76569343199606621, -44.20364726159867530, -24.33587863439580090 ) ) ;
#13490=CARTESIAN_POINT ( 'NONE',  ( -87.13361725327069962, -14.22820481747974775, -16.16779160793708314 ) ) ;
#13491=CARTESIAN_POINT ( 'NONE',  ( -114.7818785417170488, 22.12720011206953430, -0.5288015316098635399 ) ) ;
#13492=CARTESIAN_POINT ( 'NONE',  ( 184.8905102610680444, 13.49065550809807945, 13.49065550809809544 ) ) ;
#13493=CARTESIAN_POINT ( 'NONE',  ( -208.1127848780265026, 55.00245453012668406, 2.449293598294708485E-15 ) ) ;
#13494=ORIENTED_EDGE ( 'NONE', *, *, #25912, .F. ) ;
#13495=CARTESIAN_POINT ( 'NONE',  ( 25.62979979008718701, -42.16299361905902288, 22.88075396655817073 ) ) ;
#13497=CARTESIAN_POINT ( 'NONE',  ( 57.59792236341147031, 26.56190807104684382, 26.56190807104692553 ) ) ;
#13498=CARTESIAN_POINT ( 'NONE',  ( -135.8532207217289738, -40.00000000000001421, -9.153146818113709671 ) ) ;
#13499=CARTESIAN_POINT ( 'NONE',  ( -87.10593701843048109, 21.31294500819610249, 2.647731699010448025 ) ) ;
#13502=CARTESIAN_POINT ( 'NONE',  ( 170.0000000000133014, 17.64300463311800016, 17.64300463311827016 ) ) ;
#13503=CARTESIAN_POINT ( 'NONE',  ( -208.1127848780264742, 38.89260858015707356, 17.67593391476696141 ) ) ;
#13504=CARTESIAN_POINT ( 'NONE',  ( -280.0000000000000568, 14.14213562373127431, -42.42640687119274645 ) ) ;
#13505=CARTESIAN_POINT ( 'NONE',  ( -105.3145050212642104, 20.78637605557719326, -5.350913199671561316 ) ) ;
#13507=CARTESIAN_POINT ( 'NONE',  ( -86.96347745069643054, 15.38646221621821297, -41.18208027870583265 ) ) ;
#13508=CARTESIAN_POINT ( 'NONE',  ( 200.0000000000000000, 42.42640687119310172, -14.14213562373052646 ) ) ;
#13509=CARTESIAN_POINT ( 'NONE',  ( -238.4067589809705794, 0.6820004457912851592, -0.6820004457913123597 ) ) ;
#13510=CARTESIAN_POINT ( 'NONE',  ( 184.8905102610680444, 41.77492675555983936, 14.79361573936436081 ) ) ;
#13511=CARTESIAN_POINT ( 'NONE',  ( 199.9999999999999432, -20.00000000000006750, 0.000000000000000000 ) ) ;
#13512=DIRECTION ( 'NONE',  ( 0.000000000000000000, 1.000000000000000000, 0.000000000000000000 ) ) ;
#13514=CARTESIAN_POINT ( 'NONE',  ( -56.48582580120558561, -40.00000000000000000, -9.153146818113723882 ) ) ;
#13516=CARTESIAN_POINT ( 'NONE',  ( -238.4067589809705794, 40.96449427998256709, 2.449293598294708485E-15 ) ) ;
#13518=CARTESIAN_POINT ( 'NONE',  ( 57.59792236341147031, 26.56190807104693619, -30.00663442387692115 ) ) ;
#13519=CARTESIAN_POINT ( 'NONE',  ( -5.517256387798515682, 41.88221099414148085, 17.34817981594498804 ) ) ;
#13520=CARTESIAN_POINT ( 'NONE',  ( 25.05785482536065700, 17.61697374401906657, 42.53113694077252660 ) ) ;
#13521=CARTESIAN_POINT ( 'NONE',  ( -62.62756078658142656, -25.40230989543398010, -10.52198127449926623 ) ) ;
#13522=EDGE_CURVE ( 'NONE', #15233, #25714, #13030, .T. ) ;
#13524=ORIENTED_EDGE ( 'NONE', *, *, #18838, .T. ) ;
#13525=CARTESIAN_POINT ( 'NONE',  ( -166.3490444785109048, -39.29840179227969088, 12.23457652159771669 ) ) ;
#13527=CARTESIAN_POINT ( 'NONE',  ( 83.07250971288124219, -9.939191265011873000, 23.99533035163431194 ) ) ;
#13531=CARTESIAN_POINT ( 'NONE',  ( -77.90255099906767100, -8.064892378658175431, 20.29001641120675004 ) ) ;
#13532=CARTESIAN_POINT ( 'NONE',  ( 146.6084372240433709, 40.00000000000017053, -34.62501878078291639 ) ) ;
#13534=CARTESIAN_POINT ( 'NONE',  ( -200.0000000000000284, -22.85346793133670928, -44.96258949770064106 ) ) ;
#13535=CARTESIAN_POINT ( 'NONE',  ( -30.26275506840324425, -1.694272468446265334, 40.00000000000002132 ) ) ;
#13536=CARTESIAN_POINT ( 'NONE',  ( -129.2303573022295495, 9.309001179022315497, -25.82247248365979786 ) ) ;
#13538=CARTESIAN_POINT ( 'NONE',  ( -198.0356074513804572, -15.37879056873074290, 40.00000000000002132 ) ) ;
#13539=CARTESIAN_POINT ( 'NONE',  ( 192.4448373802101173, 20.00000000003945644, -40.00000000000002132 ) ) ;
#13540=CARTESIAN_POINT ( 'NONE',  ( 151.7948205124836250, -33.23291073765550863, 0.000000000000000000 ) ) ;
#13541=CARTESIAN_POINT ( 'NONE',  ( 57.59792236341147031, -1.493297263419786540E-14, 2.435789363418160658 ) ) ;
#13542=CARTESIAN_POINT ( 'NONE',  ( 57.59792236341149163, -39.99999999999961631, -37.56421063658228832 ) ) ;
#13543=CARTESIAN_POINT ( 'NONE',  ( -28.75808802781891416, -35.61482992978318407, 18.59445401971624889 ) ) ;
#13544=ORIENTED_EDGE ( 'NONE', *, *, #10058, .T. ) ;
#13545=CARTESIAN_POINT ( 'NONE',  ( -86.86493150571114086, -19.77569912839162569, 7.943527260496431985 ) ) ;
#13546=CARTESIAN_POINT ( 'NONE',  ( 5.823571940253781776, 44.77584346942675353, -24.75780943189465688 ) ) ;
#13547=CARTESIAN_POINT ( 'NONE',  ( 19.06497207195982924, -54.19242893257843008, 40.00000000000002132 ) ) ;
#13549=CARTESIAN_POINT ( 'NONE',  ( -93.01741312764114866, -8.946232117585104504, 20.50009083230827756 ) ) ;
#13551=ORIENTED_EDGE ( 'NONE', *, *, #1673, .T. ) ;
#13553=CARTESIAN_POINT ( 'NONE',  ( -86.86493150571118349, -19.60045294882770506, 8.366608963953762412 ) ) ;
#13554=CARTESIAN_POINT ( 'NONE',  ( 153.3020327024397034, 11.77299484472959890, -28.42252382389417775 ) ) ;
#13557=CARTESIAN_POINT ( 'NONE',  ( -100.0753760173618332, 8.149786832858671559, -20.72827493166386859 ) ) ;
#13558=ORIENTED_EDGE ( 'NONE', *, *, #7793, .T. ) ;
#13560=CARTESIAN_POINT ( 'NONE',  ( -87.13361725327072804, 5.903697393916396424E-14, -21.49321519333428299 ) ) ;
#13561=CARTESIAN_POINT ( 'NONE',  ( 19.06497207195981147, 38.31983398719620482, 38.31983398719633271 ) ) ;
#13562=CARTESIAN_POINT ( 'NONE',  ( -105.2054292635175727, 7.329160573984922335E-13, -21.49321519473985020 ) ) ;
#13563=CARTESIAN_POINT ( 'NONE',  ( -135.8532207217289738, 7.002209520526292428E-15, -9.153146818113572891 ) ) ;
#13564=FACE_OUTER_BOUND ( 'NONE', #6954, .T. ) ;
#13565=CARTESIAN_POINT ( 'NONE',  ( -90.07798792367796636, -2.498525064387717877E-13, 22.27377874500495381 ) ) ;
#13568=CARTESIAN_POINT ( 'NONE',  ( -192.9588430854690273, -39.99999999999948841, -54.46834944098263520 ) ) ;
#13569=CARTESIAN_POINT ( 'NONE',  ( -199.9999999999999716, -48.57705986237291995, -14.87399974031227501 ) ) ;
#13570=CARTESIAN_POINT ( 'NONE',  ( 130.8568914410475372, 24.07718906447243867, -24.07718906447216156 ) ) ;
#13571=CARTESIAN_POINT ( 'NONE',  ( -162.0762913951020892, -3.568845385355699554E-14, 1.694272876828323948 ) ) ;
#13572=CARTESIAN_POINT ( 'NONE',  ( -198.9234529669031701, 14.16707775658443857, 49.24835336340146341 ) ) ;
#13574=CARTESIAN_POINT ( 'NONE',  ( -259.2033419157646676, 6.730120644403521979, -6.730120644403498886 ) ) ;
#13575=CARTESIAN_POINT ( 'NONE',  ( -100.7734535825088358, 6.065416334915073333E-14, -22.67402823373191723 ) ) ;
#13576=CARTESIAN_POINT ( 'NONE',  ( 19.06497207195980792, -18.24870850772763475, 38.31983398719622613 ) ) ;
#13577=CARTESIAN_POINT ( 'NONE',  ( -30.26275506840322294, -57.76657404653985139, -1.198031551616531853 ) ) ;
#13579=CARTESIAN_POINT ( 'NONE',  ( -2.937533998744902508, 23.68967259522915114, 43.32931883109763760 ) ) ;
#13580=ORIENTED_EDGE ( 'NONE', *, *, #21416, .T. ) ;
#13581=CARTESIAN_POINT ( 'NONE',  ( 163.1118516004056573, 37.29075403953132906, 19.27778845539275565 ) ) ;
#13585=CARTESIAN_POINT ( 'NONE',  ( 4.995406935893290878, 1.606505379428369110E-13, -15.24977328854832592 ) ) ;
#13586=CARTESIAN_POINT ( 'NONE',  ( -3.971463587458989863, -23.46415232637805204, 43.02522237042967390 ) ) ;
#13587=CARTESIAN_POINT ( 'NONE',  ( 7.340276910564550228, -44.87059041559395922, 24.82763627182874089 ) ) ;
#13589=ORIENTED_EDGE ( 'NONE', *, *, #8428, .T. ) ;
#13590=CARTESIAN_POINT ( 'NONE',  ( 19.06497207195980792, 54.19242893257844429, -40.00000000000002132 ) ) ;
#13591=CARTESIAN_POINT ( 'NONE',  ( -30.26275506840324070, -1.198031551616032919, 1.198031551616014712 ) ) ;
#13592=CARTESIAN_POINT ( 'NONE',  ( 151.7948205124836534, 40.00000000000002842, 6.767089262349174739 ) ) ;
#13593=CARTESIAN_POINT ( 'NONE',  ( -94.58414068586590417, -20.73981583695825037, -8.590713000584871750 ) ) ;
#13596=CARTESIAN_POINT ( 'NONE',  ( 91.82158438592156813, 39.99999999999986500, 17.20528682183341473 ) ) ;
#13597=CARTESIAN_POINT ( 'NONE',  ( 184.8905102610680444, -40.00000000000005684, 19.07866798485543569 ) ) ;
#13599=CARTESIAN_POINT ( 'NONE',  ( 130.8568914410475088, 40.00000000000015632, -34.05028731879774284 ) ) ;
#13600=EDGE_CURVE ( 'NONE', #23212, #4362, #12694, .T. ) ;
#13601=FACE_OUTER_BOUND ( 'NONE', #4291, .T. ) ;
#13602=CARTESIAN_POINT ( 'NONE',  ( -62.79433447037396832, -9.335111860870215494, -25.93934121798541881 ) ) ;
#13603=CARTESIAN_POINT ( 'NONE',  ( 199.9999999999999432, 14.14213562373093680, 14.14213562373114641 ) ) ;
#13604=CARTESIAN_POINT ( 'NONE',  ( -87.01701082927806397, -18.46482525710459299, 10.86389608312037680 ) ) ;
#13605=CARTESIAN_POINT ( 'NONE',  ( -162.0762913951021176, -40.00000000000003553, -1.694272876828743168 ) ) ;
#13606=CARTESIAN_POINT ( 'NONE',  ( 73.43438319819851756, 9.843172589490714941, 28.18283897611961919 ) ) ;
#13607=CARTESIAN_POINT ( 'NONE',  ( -86.96347745069645896, 21.75974354311648895, -0.000000000000000000 ) ) ;
#13608=CARTESIAN_POINT ( 'NONE',  ( 200.0000000000000000, 20.00000000000013856, -40.00000000000002132 ) ) ;
#13609=EDGE_CURVE ( 'NONE', #1209, #13720, #16199, .T. ) ;
#13610=CARTESIAN_POINT ( 'NONE',  ( -30.26275506840324070, -1.198031551616032919, 1.198031551616014712 ) ) ;
#13611=CARTESIAN_POINT ( 'NONE',  ( 130.8568914410475372, 34.05028731879791337, 0.000000000000000000 ) ) ;
#13612=CARTESIAN_POINT ( 'NONE',  ( -3.555049149807454345, -43.14507846637731348, -23.55301256057186166 ) ) ;
#13613=CARTESIAN_POINT ( 'NONE',  ( -114.4364955367328349, 20.29001642038852538, -8.064892380842216824 ) ) ;
#13614=CARTESIAN_POINT ( 'NONE',  ( 0.2972598230769907257, 66.70487387989857098, 10.13633138497486641 ) ) ;
#13615=ADVANCED_FACE ( 'NONE', ( #5756 ), #22526, .T. ) ;
#13616=CARTESIAN_POINT ( 'NONE',  ( 146.6084372240433709, 5.374981219217002781, -40.00000000000002132 ) ) ;
#13617=B_SPLINE_CURVE_WITH_KNOTS ( 'NONE', 3,
 ( #4103, #14195, #16461, #22327, #2101, #25696 ),
 .UNSPECIFIED., .F., .F.,
 ( 4, 2, 4 ),
 ( -6.000000000394485207E-08, 0.04016968416333294850, 0.08033942832666590705 ),
 .UNSPECIFIED. ) ;
#13618=ORIENTED_EDGE ( 'NONE', *, *, #22424, .T. ) ;
#13620=CARTESIAN_POINT ( 'NONE',  ( 22.78333232259052110, -43.17211919388228836, 17.88247728649368895 ) ) ;
#13622=CARTESIAN_POINT ( 'NONE',  ( -105.3755690713226585, 12.89780903124410472, -43.67073346367977393 ) ) ;
#13623=CARTESIAN_POINT ( 'NONE',  ( 0.2972598230770030492, -1.921041075453695163E-13, 54.33493731733936016 ) ) ;
#13625=CARTESIAN_POINT ( 'NONE',  ( 146.6084372240433709, 3.800685668858042821, 52.76785682606522698 ) ) ;
#13627=CARTESIAN_POINT ( 'NONE',  ( -259.2033419157646676, -9.517827891722680178, -40.00000000000002132 ) ) ;
#13631=CARTESIAN_POINT ( 'NONE',  ( -82.30220482034330587, -7.441767004318580625, -18.74474319042437642 ) ) ;
#13632=CARTESIAN_POINT ( 'NONE',  ( 14.38125909742180220, 39.01709431150892016, 17.55144818341517166 ) ) ;
#13633=CARTESIAN_POINT ( 'NONE',  ( 184.8905102610680444, 14.79361573936424890, -41.77492675555986068 ) ) ;
#13634=CARTESIAN_POINT ( 'NONE',  ( -110.0579415639987388, 19.23682107564352961, -6.226559743088629695 ) ) ;
#13635=CARTESIAN_POINT ( 'NONE',  ( 57.59792236341147031, -1.493297263419786540E-14, 2.435789363418160658 ) ) ;
#13636=CARTESIAN_POINT ( 'NONE',  ( 130.8568914410475088, 52.36146031193427319, -4.207082182989173802 ) ) ;
#13637=CARTESIAN_POINT ( 'NONE',  ( -56.48582580120558561, 6.472252184284607246, -50.09629031063960269 ) ) ;
#13638=CARTESIAN_POINT ( 'NONE',  ( -213.1075012329537230, 9.698598906438871126, -66.26714140136179765 ) ) ;
#13639=CARTESIAN_POINT ( 'NONE',  ( -280.0000000000000000, -14.14213562373118549, 14.14213562373078936 ) ) ;
#13641=CARTESIAN_POINT ( 'NONE',  ( 163.1118516004056573, -19.27778845538761132, -19.27778845538770724 ) ) ;
#13643=CARTESIAN_POINT ( 'NONE',  ( 4.995406935893305089, -40.00000000000021316, 55.24977328853194791 ) ) ;
#13644=CARTESIAN_POINT ( 'NONE',  ( 57.59792236341148453, -26.56190807104700369, 26.56190807104673723 ) ) ;
#13647=CARTESIAN_POINT ( 'NONE',  ( -162.0762913951020892, 41.69427287682832173, 2.449293598294708485E-15 ) ) ;
#13648=ORIENTED_EDGE ( 'NONE', *, *, #22837, .T. ) ;
#13649=CARTESIAN_POINT ( 'NONE',  ( -208.1127848780265026, 10.60833733269537049, 10.60833733269544510 ) ) ;
#13650=B_SPLINE_CURVE_WITH_KNOTS ( 'NONE', 3,
 ( #18342, #12351, #20480, #2254, #18745, #16485, #8631, #18878, #10362, #391, #16742, #24875 ),
 .UNSPECIFIED., .F., .F.,
 ( 4, 2, 2, 2, 2, 4 ),
 ( -5.998499567893129066E-08, 0.003531500499830294692, 0.007063060984656268325, 0.01412618195430822773, 0.02118930292396017934, 0.02825242389361213441 ),
 .UNSPECIFIED. ) ;
#13652=CARTESIAN_POINT ( 'NONE',  ( 44.46627453567793964, 15.24062802624261437, 36.79413088023001421 ) ) ;
#13653=CARTESIAN_POINT ( 'NONE',  ( 98.29820294267493352, -20.00000000000511235, 5.223721743777709619E-12 ) ) ;
#13654=VERTEX_POINT ( 'NONE', #5464 ) ;
#13655=CARTESIAN_POINT ( 'NONE',  ( -188.3392535381713913, -47.00481007172062675, 13.83023904993491371 ) ) ;
#13657=CARTESIAN_POINT ( 'NONE',  ( 22.75882399337420026, -17.88527043150875429, 43.17886244245843130 ) ) ;
#13659=CARTESIAN_POINT ( 'NONE',  ( 23.39921416754922134, 13.79910252519628955, -46.79910576274355094 ) ) ;
#13662=CARTESIAN_POINT ( 'NONE',  ( 190.0000000000000000, 70.00000000000000000, 0.000000000000000000 ) ) ;
#13663=CARTESIAN_POINT ( 'NONE',  ( 57.59792236341146321, 40.00000000000004263, -2.435789363418021214 ) ) ;
#13666=CARTESIAN_POINT ( 'NONE',  ( 0.2972598230770129857, -54.33493731733938148, 40.00000000000002132 ) ) ;
#13667=CARTESIAN_POINT ( 'NONE',  ( -183.1091233172239185, 13.45963571009543891, -45.18843800006289513 ) ) ;
#13669=EDGE_CURVE ( 'NONE', #1902, #15674, #10147, .T. ) ;
#13670=CARTESIAN_POINT ( 'NONE',  ( 98.29820294268675696, -2.727061086135049273, -20.00000000000119371 ) ) ;
#13671=CARTESIAN_POINT ( 'NONE',  ( -192.9588430854690273, -54.46834944101725284, -40.00000000000002132 ) ) ;
#13672=CARTESIAN_POINT ( 'NONE',  ( -30.26275506840324425, 1.694272468446254232, 40.00000000000002132 ) ) ;
#13673=CARTESIAN_POINT ( 'NONE',  ( 4.995406935893306866, -39.99999999999944578, -55.24977328856505920 ) ) ;
#13675=CARTESIAN_POINT ( 'NONE',  ( 19.06497207195981147, -10.03556273973425483, -10.03556273973443247 ) ) ;
#13676=ORIENTED_EDGE ( 'NONE', *, *, #7036, .F. ) ;
#13677=CARTESIAN_POINT ( 'NONE',  ( -28.75808802591297209, -38.33175228464053674, 12.03522322449780724 ) ) ;
#13678=CARTESIAN_POINT ( 'NONE',  ( 4.995406935893289102, 10.78321810388998081, 10.78321810389001811 ) ) ;
#13680=FACE_OUTER_BOUND ( 'NONE', #16521, .T. ) ;
#13683=VERTEX_POINT ( 'NONE', #8071 ) ;
#13684=VECTOR ( 'NONE', #17703, 1000.000000000000000 ) ;
#13686=CARTESIAN_POINT ( 'NONE',  ( 60.28378959955089300, -33.17072922786156397, -10.93033916064820055 ) ) ;
#13688=CARTESIAN_POINT ( 'NONE',  ( 151.7948205124836534, -33.23291073765550863, -40.00000000000002132 ) ) ;
#13689=CARTESIAN_POINT ( 'NONE',  ( -97.73860346104272878, -20.56359266937362662, 8.987542150667973573 ) ) ;
#13692=CARTESIAN_POINT ( 'NONE',  ( -190.6721449140024447, 13.94344083317847272, 47.76494005424133604 ) ) ;
#13693=CARTESIAN_POINT ( 'NONE',  ( 4.995406935893287326, 67.35176059882533650, 10.78321810390163549 ) ) ;
#13695=CARTESIAN_POINT ( 'NONE',  ( 57.59792236341147031, 1.908507979671054758E-14, -2.435789363418160658 ) ) ;
#13697=CARTESIAN_POINT ( 'NONE',  ( 170.0000000000000000, 3.122849337825751958E-14, 0.000000000000000000 ) ) ;
#13699=CARTESIAN_POINT ( 'NONE',  ( 192.4448373802100889, -1.741373372144848397E-13, 20.00000000003942091 ) ) ;
#13700=CARTESIAN_POINT ( 'NONE',  ( 19.06497207195982924, -39.99999999999945288, -54.19242893257885640 ) ) ;
#13701=CARTESIAN_POINT ( 'NONE',  ( -105.4293522939502310, -9.002736003369118833, 19.36070119851716598 ) ) ;
#13702=CARTESIAN_POINT ( 'NONE',  ( -208.1127848780265026, -10.60833733269551971, 10.60833733269537049 ) ) ;
#13703=CARTESIAN_POINT ( 'NONE',  ( -238.4067589809705794, -4.716212492215116094E-14, 0.9644942799825824142 ) ) ;
#13705=CARTESIAN_POINT ( 'NONE',  ( -198.0356074513804572, -67.44298959250878056, 10.87444709758448447 ) ) ;
#13707=CARTESIAN_POINT ( 'NONE',  ( -83.21262154144248768, 13.72187187061462232, 33.12752917118429963 ) ) ;
#13708=CARTESIAN_POINT ( 'NONE',  ( 136.1360204305621266, -3.419521671106983309E-13, 35.03383547441296741 ) ) ;
#13709=CARTESIAN_POINT ( 'NONE',  ( 184.8905102610680444, -39.99999999999991473, -20.92133201514458207 ) ) ;
#13710=CARTESIAN_POINT ( 'NONE',  ( -198.0356074513804572, 39.15871834505901461, 39.15871834505919935 ) ) ;
#13711=CARTESIAN_POINT ( 'NONE',  ( -162.0762913951020892, -1.198031840385767266, -1.198031840385758384 ) ) ;
#13712=CARTESIAN_POINT ( 'NONE',  ( -188.2871287166310594, -23.44689273421379738, -43.00155302796976287 ) ) ;
#13713=CARTESIAN_POINT ( 'NONE',  ( 136.1360204305621266, 24.77266263493138965, -24.77266263493110188 ) ) ;
#13715=CARTESIAN_POINT ( 'NONE',  ( -213.1075012329537230, 9.698598906438871126, -66.26714140136179765 ) ) ;
#13716=CARTESIAN_POINT ( 'NONE',  ( -91.56559293963836410, 22.67402823373190301, -40.00000000000002132 ) ) ;
#13718=CARTESIAN_POINT ( 'NONE',  ( -198.0356074513804572, -17.40982414986427429, -39.15871834505933435 ) ) ;
#13719=CARTESIAN_POINT ( 'NONE',  ( -87.07756624669964651, 3.737545040615061875, 21.12895881758995387 ) ) ;
#13720=VERTEX_POINT ( 'NONE', #2232 ) ;
#13723=CARTESIAN_POINT ( 'NONE',  ( 2.303792037522391922, 18.40682559462096179, 44.43800799080432995 ) ) ;
#13724=ORIENTED_EDGE ( 'NONE', *, *, #18043, .F. ) ;
#13725=VERTEX_POINT ( 'NONE', #4240 ) ;
#13726=CARTESIAN_POINT ( 'NONE',  ( -208.1127848780264742, 55.00245453010919050, -40.00000000000002132 ) ) ;
#13727=CARTESIAN_POINT ( 'NONE',  ( -105.3755690713226727, 15.38646221621793231, -15.38646221621779020 ) ) ;
#13728=CARTESIAN_POINT ( 'NONE',  ( -91.56559293963836410, 40.00000000000008527, -22.67402823373177867 ) ) ;
#13729=CARTESIAN_POINT ( 'NONE',  ( -97.73806390048314086, -20.71810467718897542, -8.581719943884214885 ) ) ;
#13731=CARTESIAN_POINT ( 'NONE',  ( 57.59792236341146321, 40.00000000000000711, 2.435789363418579434 ) ) ;
#13734=CARTESIAN_POINT ( 'NONE',  ( -3.993758944536813349, -23.45926997169897277, -43.01863922058836209 ) ) ;
#13735=CARTESIAN_POINT ( 'NONE',  ( 4.995406935893300648, -10.78321810387790514, -67.35176059880241439 ) ) ;
#13736=CARTESIAN_POINT ( 'NONE',  ( -77.78697283798516082, -20.89074004981921462, 6.810146944722274220 ) ) ;
#13737=CARTESIAN_POINT ( 'NONE',  ( 19.06497207195981858, -38.31983398719616218, -18.24870850772777331 ) ) ;
#13738=CARTESIAN_POINT ( 'NONE',  ( -56.48582580120559271, -1.062504017861011783E-13, 9.153146818113587102 ) ) ;
#13739=CARTESIAN_POINT ( 'NONE',  ( -105.2940237833728219, -20.91877113668857291, -4.710801307200714660 ) ) ;
#13740=CARTESIAN_POINT ( 'NONE',  ( -198.0356074513804572, -15.37879056873074290, 0.000000000000000000 ) ) ;
#13741=CARTESIAN_POINT ( 'NONE',  ( -91.56559293963834989, -17.32597176626812896, -2.449293598294708485E-15 ) ) ;
#13742=CARTESIAN_POINT ( 'NONE',  ( 57.59792236341147031, 30.00663442387683588, 26.56190807104703211 ) ) ;
#13743=CARTESIAN_POINT ( 'NONE',  ( -162.0762913951020892, -41.69427287672991866, -40.00000000000002132 ) ) ;
#13744=CARTESIAN_POINT ( 'NONE',  ( -109.1264249741454790, 13.72187187123907393, 33.12752917269271080 ) ) ;
#13745=CARTESIAN_POINT ( 'NONE',  ( 91.82158438592158234, -1.633484621919921769E-13, 17.20528682183300262 ) ) ;
#13746=CARTESIAN_POINT ( 'NONE',  ( -208.1127848780264742, 67.17687982760683951, 10.60833733268317403 ) ) ;
#13747=CARTESIAN_POINT ( 'NONE',  ( -213.1075012329537230, 53.71589010950162191, -40.00000000000002132 ) ) ;
#13750=CARTESIAN_POINT ( 'NONE',  ( -53.37717264285771535, -10.11115224722899342, 29.42738956023912777 ) ) ;
#13751=CARTESIAN_POINT ( 'NONE',  ( 151.7948205124836534, 4.785054706298574878, -51.78348778862537927 ) ) ;
#13752=CARTESIAN_POINT ( 'NONE',  ( 163.1118516004056573, -1.695744499706194789E-14, 12.73709011382475254 ) ) ;
#13753=CARTESIAN_POINT ( 'NONE',  ( 57.59792236341147031, -1.722363176415055985, 1.722363176415024677 ) ) ;
#13754=CARTESIAN_POINT ( 'NONE',  ( -259.2033419157646676, -9.517827891722680178, 0.000000000000000000 ) ) ;
#13755=CARTESIAN_POINT ( 'NONE',  ( -105.3755690713226727, -21.75974354311652093, 0.000000000000000000 ) ) ;
#13759=CARTESIAN_POINT ( 'NONE',  ( -77.84504298467653882, -7.440570986992908864, -20.58891737387387977 ) ) ;
#13760=CARTESIAN_POINT ( 'NONE',  ( 192.4448373802100889, -14.14213562375896061, 14.14213562375865330 ) ) ;
#13761=CARTESIAN_POINT ( 'NONE',  ( -56.48582580120559982, 34.75652343174628101, -21.81201906317743067 ) ) ;
#13762=EDGE_CURVE ( 'NONE', #22287, #22653, #13617, .T. ) ;
#13763=CARTESIAN_POINT ( 'NONE',  ( -105.2143515744611477, 21.43501564603285559, -1.534306871497952640 ) ) ;
#13764=CARTESIAN_POINT ( 'NONE',  ( -77.55658273868580466, 16.64052652070787985, -14.65657382810189802 ) ) ;
#13765=CARTESIAN_POINT ( 'NONE',  ( -162.0762913951020892, -29.48230308784744125, -29.48230308784792442 ) ) ;
#13766=CARTESIAN_POINT ( 'NONE',  ( -238.4067589809705794, -0.6820004457337348613, -57.25054294065803617 ) ) ;
#13767=CARTESIAN_POINT ( 'NONE',  ( -56.48582580120559982, -34.75652343174584047, -21.81201906317815187 ) ) ;
#13768=CARTESIAN_POINT ( 'NONE',  ( -56.48582580120559982, -34.75652343174584047, -21.81201906317815187 ) ) ;
#13770=CARTESIAN_POINT ( 'NONE',  ( 151.7948205124836250, 33.23291073765556547, 0.000000000000000000 ) ) ;
#13772=CARTESIAN_POINT ( 'NONE',  ( 146.6084372240433993, 1.478241399363601114E-13, -34.62501878078305850 ) ) ;
#13773=CARTESIAN_POINT ( 'NONE',  ( -100.7734535825088500, 44.31723036834890905, 12.25131212657507795 ) ) ;
#13775=CARTESIAN_POINT ( 'NONE',  ( 4.995406935893288214, 15.24977328854832770, 40.00000000000002132 ) ) ;
#13776=ORIENTED_EDGE ( 'NONE', *, *, #7337, .T. ) ;
#13777=CARTESIAN_POINT ( 'NONE',  ( 170.2234770963711128, 10.92277846919210660, -45.64576402573182889 ) ) ;
#13778=CARTESIAN_POINT ( 'NONE',  ( 69.64403118996989406, 28.54215590813338110, 11.82254807651625761 ) ) ;
#13779=CARTESIAN_POINT ( 'NONE',  ( -4.039451493210483690, -13.82811171175408127, -46.99046209229819482 ) ) ;
#13780=CARTESIAN_POINT ( 'NONE',  ( -192.9588430854689989, 14.46834944099965981, 0.000000000000000000 ) ) ;
#13781=ORIENTED_EDGE ( 'NONE', *, *, #6614, .F. ) ;
#13782=CARTESIAN_POINT ( 'NONE',  ( -3.901164313503196812, 23.47934491069935703, -43.04571088859049866 ) ) ;
#13784=CARTESIAN_POINT ( 'NONE',  ( -3.966425590329204720, -13.83202835294355459, 47.01685867532394525 ) ) ;
#13785=CARTESIAN_POINT ( 'NONE',  ( 17.91733029159264490, 24.32486282482700091, -44.18858371746296143 ) ) ;
#13787=CARTESIAN_POINT ( 'NONE',  ( -86.84962968273566730, 19.67999904273991163, 8.151722510992470916 ) ) ;
#13788=FACE_OUTER_BOUND ( 'NONE', #4883, .T. ) ;
#13789=CARTESIAN_POINT ( 'NONE',  ( 136.1360204305621551, 31.79587985999232558, 24.77266263493161702 ) ) ;
#13790=CARTESIAN_POINT ( 'NONE',  ( -192.9588430854690273, -14.46834944099973264, 40.00000000000002132 ) ) ;
#13794=CARTESIAN_POINT ( 'NONE',  ( -192.9588430854689989, 10.23066800230756712, -10.23066800230735396 ) ) ;
#13795=CARTESIAN_POINT ( 'NONE',  ( -238.4067589809705794, -0.9644942799826263791, -40.00000000000002132 ) ) ;
#13796=CARTESIAN_POINT ( 'NONE',  ( -192.9588430854690273, 54.46834944101718889, 40.00000000000002132 ) ) ;
#13797=CARTESIAN_POINT ( 'NONE',  ( 57.59792236341149163, -39.99999999999961631, -37.56421063658228832 ) ) ;
#13798=CARTESIAN_POINT ( 'NONE',  ( 98.29820294267409508, -12.20973600809984738, 15.89413956775044845 ) ) ;
#13799=CARTESIAN_POINT ( 'NONE',  ( -208.1127848780265026, -10.60833733269537227, -10.60833733269551793 ) ) ;
#13801=CARTESIAN_POINT ( 'NONE',  ( 98.29820294267436509, 14.14213562374297695, -14.14213562372651189 ) ) ;
#13802=CARTESIAN_POINT ( 'NONE',  ( 136.1360204305621266, 35.03383547441298873, 0.000000000000000000 ) ) ;
#13803=CARTESIAN_POINT ( 'NONE',  ( -105.4741150117391015, -7.943527260750077978, 19.77569912955109288 ) ) ;
#13806=ORIENTED_EDGE ( 'NONE', *, *, #9711, .T. ) ;
#13808=CARTESIAN_POINT ( 'NONE',  ( 170.2234770963711128, 17.36149277827004411, -17.36149277826983095 ) ) ;
#13809=CARTESIAN_POINT ( 'NONE',  ( 83.07250971316962307, -23.99533035190363961, -9.939191265417465004 ) ) ;
#13811=CARTESIAN_POINT ( 'NONE',  ( 184.8905102610680444, -20.92133201514440799, -40.00000000000002132 ) ) ;
#13812=CARTESIAN_POINT ( 'NONE',  ( -114.4364955367335881, -20.04994829326802019, 8.644468109231409514 ) ) ;
#13818=CARTESIAN_POINT ( 'NONE',  ( 184.8905102610680444, -14.79361573936389540, 41.77492675555996016 ) ) ;
#13820=CARTESIAN_POINT ( 'NONE',  ( -198.0356074513804572, -9.007331120208026888E-14, 15.37879056873070560 ) ) ;
#13821=CARTESIAN_POINT ( 'NONE',  ( -56.48582580120559982, -9.153146818113595984, 40.00000000000002132 ) ) ;
#13825=CARTESIAN_POINT ( 'NONE',  ( -208.1127848780265026, -9.061048840815752106E-14, 15.00245453012669472 ) ) ;
#13826=CARTESIAN_POINT ( 'NONE',  ( -162.0762913951020892, -1.202636532414034422E-14, -1.694272876828323948 ) ) ;
#13828=CARTESIAN_POINT ( 'NONE',  ( 19.06497207195982568, -38.31983398719646061, 38.31983398719606271 ) ) ;
#13829=CARTESIAN_POINT ( 'NONE',  ( 4.995406935893294431, -15.24977328854832415, -40.00000000000002132 ) ) ;
#13830=CARTESIAN_POINT ( 'NONE',  ( -135.8532207217289738, -21.81201906317758343, -34.75652343174620995 ) ) ;
#13832=CARTESIAN_POINT ( 'NONE',  ( -2.654373026594509355, -47.46285323120914512, 13.89837698318172343 ) ) ;
#13833=CARTESIAN_POINT ( 'NONE',  ( 14.38125909742181108, 1.616281842095393922E-13, -15.17850393972633682 ) ) ;
#13834=CARTESIAN_POINT ( 'NONE',  ( -91.56559293963834989, -39.99999999999995737, -22.67402823373205933 ) ) ;
#13835=CARTESIAN_POINT ( 'NONE',  ( 170.2234770963711128, 10.92277846919201068, 10.92277846919202133 ) ) ;
#13837=CARTESIAN_POINT ( 'NONE',  ( -192.9588430854689989, -10.23066800230742501, -10.23066800230756712 ) ) ;
#13838=CARTESIAN_POINT ( 'NONE',  ( -188.3392995398617700, -23.45797413244939378, -43.01688924974088479 ) ) ;
#13839=CARTESIAN_POINT ( 'NONE',  ( 199.9999999999999432, 14.14213562373113398, -14.14213562373094923 ) ) ;
#13841=CARTESIAN_POINT ( 'NONE',  ( 146.6084372240433709, -52.76785682606510619, -3.800685668859292043 ) ) ;
#13842=CARTESIAN_POINT ( 'NONE',  ( -86.96347745069644475, 15.38646221621793586, -15.38646221621778842 ) ) ;
#13844=EDGE_CURVE ( 'NONE', #10098, #19642, #22168, .T. ) ;
#13846=CARTESIAN_POINT ( 'NONE',  ( -208.1127848780264742, -17.67593391476605547, -38.89260858015755673 ) ) ;
#13847=CARTESIAN_POINT ( 'NONE',  ( 48.46027384457784137, -35.02097776273539864, 18.19770403991817886 ) ) ;
#13848=ORIENTED_EDGE ( 'NONE', *, *, #11755, .T. ) ;
#13852=CARTESIAN_POINT ( 'NONE',  ( -4.004886986946478267, 23.45685150724344581, 43.01537795656734176 ) ) ;
#13854=ORIENTED_EDGE ( 'NONE', *, *, #17113, .F. ) ;
#13858=CARTESIAN_POINT ( 'NONE',  ( 19.06497207195981858, -1.881589693694111225E-13, 54.19242893257843008 ) ) ;
#13864=( BOUNDED_SURFACE ( )  B_SPLINE_SURFACE ( 3, 3, ( 
 ( #12574, #24971, #8587, #14440, #24831, #20706, #22305, #22570, #18566, #24565, #20568, #4082, #2472, #10582, #482, #14704, #2214, #12183, #12708, #22441, #18834, #16439, #22835, #10323, #8316, #614, #6320, #20304, #4612, #2611 ),
 ( #8720, #18292, #18430, #78, #8187, #207, #16304, #24428, #6194, #4218, #12309, #3223, #13328, #11329, #7585, #1619, #11713, #23696, #13576, #19833, #9338, #21575, #1233, #19445, #5347, #9462, #3349, #15444, #17446, #9726 ),
 ( #11449, #25841, #25584, #1486, #21703, #19698, #21835, #19320, #22964, #17696, #17569, #13456, #7331, #25706, #15572, #23572, #7457, #19572, #21449, #17828, #1363, #5476, #3480, #3604, #10852, #15697, #23821, #4744, #1102, #9212 ),
 ( #11578, #25975, #9591, #14832, #5603, #13710, #12850, #20967, #2748, #17323, #25457, #7208, #15323, #23449, #5224, #3742, #20504, #14240, #14376, #1884, #2276, #7715, #22380, #12117, #23956, #20241, #13835, #12, #24233, #22242 ),
 ( #6263, #10385, #2022, #4017, #10124, #7983, #14114, #24092, #12251, #2148, #22509, #18225, #16240, #8123, #21970, #6006, #24369, #9857, #5731, #6132, #20373, #1749, #4156, #5867, #11847, #10258, #15967, #17960, #18367, #13973 ),
 ( #18496, #147, #15826, #19968, #8251, #22107, #16369, #24502, #4287, #3883, #26107, #12376, #11983, #7846, #20107, #9989, #18099, #26248, #16101, #12645, #8788, #679, #20633, #20770, #4547, #16506, #18632, #2540, #19034, #551 ),
 ( #16900, #276, #2938, #6519, #13047, #23162, #14767, #21031, #12505, #8655, #23037, #25164, #11048, #8919, #14897, #8384, #12778, #15032, #20905, #6652, #10922, #10658, #12914, #25032, #4812, #6915, #4411, #24631, #2814, #2683 ) ),
 .UNSPECIFIED., .T., .F., .T. ) 
 B_SPLINE_SURFACE_WITH_KNOTS ( ( 4, 3, 4 ),
 ( 4, 2, 2, 2, 2, 2, 2, 2, 2, 2, 2, 2, 2, 2, 4 ),
 ( 0.000000000000000000, 0.5000000000000000000, 1.000000000000000000 ),
 ( 0.000000000000000000, 0.1357259735107005372, 0.1651108541090157700, 0.1944957347073310028, 0.3598804999793158710, 0.3867117631979620773, 0.4135430264166082281, 0.5789277916885930964, 0.6062785021374117456, 0.6336292125862302838, 0.8508620842112317728, 0.8814014469398914198, 0.9119408096685510667, 0.9559704048342755334, 1.000000000000000000 ),
 .UNSPECIFIED. ) 
 GEOMETRIC_REPRESENTATION_ITEM ( )  RATIONAL_B_SPLINE_SURFACE ( (
 ( 1.000000000000000000, 1.000000000000000000, 1.000000000000000000, 1.000000000000000000, 1.000000000000000000, 1.000000000000000000, 1.000000000000000000, 1.000000000000000000, 1.000000000000000000, 1.000000000000000000, 1.000000000000000000, 1.000000000000000000, 1.000000000000000000, 1.000000000000000000, 1.000000000000000000, 1.000000000000000000, 1.000000000000000000, 1.000000000000000000, 1.000000000000000000, 1.000000000000000000, 1.000000000000000000, 1.000000000000000000, 1.000000000000000000, 1.000000000000000000, 1.000000000000000000, 1.000000000000000000, 1.000000000000000000, 1.000000000000000000, 1.000000000000000000, 1.000000000000000000),
 ( 0.3333333333333333703, 0.3333333333333333703, 0.3333333333333333703, 0.3333333333333333703, 0.3333333333333333703, 0.3333333333333333703, 0.3333333333333333703, 0.3333333333333333703, 0.3333333333333333703, 0.3333333333333333703, 0.3333333333333333703, 0.3333333333333333703, 0.3333333333333333703, 0.3333333333333333703, 0.3333333333333333703, 0.3333333333333333703, 0.3333333333333333703, 0.3333333333333333703, 0.3333333333333333703, 0.3333333333333333703, 0.3333333333333333703, 0.3333333333333333703, 0.3333333333333333703, 0.3333333333333333703, 0.3333333333333333703, 0.3333333333333333703, 0.3333333333333333703, 0.3333333333333333703, 0.3333333333333333703, 0.3333333333333333703),
 ( 0.3333333333333333703, 0.3333333333333333703, 0.3333333333333333703, 0.3333333333333333703, 0.3333333333333333703, 0.3333333333333333703, 0.3333333333333333703, 0.3333333333333333703, 0.3333333333333333703, 0.3333333333333333703, 0.3333333333333333703, 0.3333333333333333703, 0.3333333333333333703, 0.3333333333333333703, 0.3333333333333333703, 0.3333333333333333703, 0.3333333333333333703, 0.3333333333333333703, 0.3333333333333333703, 0.3333333333333333703, 0.3333333333333333703, 0.3333333333333333703, 0.3333333333333333703, 0.3333333333333333703, 0.3333333333333333703, 0.3333333333333333703, 0.3333333333333333703, 0.3333333333333333703, 0.3333333333333333703, 0.3333333333333333703),
 ( 1.000000000000000000, 1.000000000000000000, 1.000000000000000000, 1.000000000000000000, 1.000000000000000000, 1.000000000000000000, 1.000000000000000000, 1.000000000000000000, 1.000000000000000000, 1.000000000000000000, 1.000000000000000000, 1.000000000000000000, 1.000000000000000000, 1.000000000000000000, 1.000000000000000000, 1.000000000000000000, 1.000000000000000000, 1.000000000000000000, 1.000000000000000000, 1.000000000000000000, 1.000000000000000000, 1.000000000000000000, 1.000000000000000000, 1.000000000000000000, 1.000000000000000000, 1.000000000000000000, 1.000000000000000000, 1.000000000000000000, 1.000000000000000000, 1.000000000000000000),
 ( 0.3333333333333333703, 0.3333333333333333703, 0.3333333333333333703, 0.3333333333333333703, 0.3333333333333333703, 0.3333333333333333703, 0.3333333333333333703, 0.3333333333333333703, 0.3333333333333333703, 0.3333333333333333703, 0.3333333333333333703, 0.3333333333333333703, 0.3333333333333333703, 0.3333333333333333703, 0.3333333333333333703, 0.3333333333333333703, 0.3333333333333333703, 0.3333333333333333703, 0.3333333333333333703, 0.3333333333333333703, 0.3333333333333333703, 0.3333333333333333703, 0.3333333333333333703, 0.3333333333333333703, 0.3333333333333333703, 0.3333333333333333703, 0.3333333333333333703, 0.3333333333333333703, 0.3333333333333333703, 0.3333333333333333703),
 ( 0.3333333333333333703, 0.3333333333333333703, 0.3333333333333333703, 0.3333333333333333703, 0.3333333333333333703, 0.3333333333333333703, 0.3333333333333333703, 0.3333333333333333703, 0.3333333333333333703, 0.3333333333333333703, 0.3333333333333333703, 0.3333333333333333703, 0.3333333333333333703, 0.3333333333333333703, 0.3333333333333333703, 0.3333333333333333703, 0.3333333333333333703, 0.3333333333333333703, 0.3333333333333333703, 0.3333333333333333703, 0.3333333333333333703, 0.3333333333333333703, 0.3333333333333333703, 0.3333333333333333703, 0.3333333333333333703, 0.3333333333333333703, 0.3333333333333333703, 0.3333333333333333703, 0.3333333333333333703, 0.3333333333333333703),
 ( 1.000000000000000000, 1.000000000000000000, 1.000000000000000000, 1.000000000000000000, 1.000000000000000000, 1.000000000000000000, 1.000000000000000000, 1.000000000000000000, 1.000000000000000000, 1.000000000000000000, 1.000000000000000000, 1.000000000000000000, 1.000000000000000000, 1.000000000000000000, 1.000000000000000000, 1.000000000000000000, 1.000000000000000000, 1.000000000000000000, 1.000000000000000000, 1.000000000000000000, 1.000000000000000000, 1.000000000000000000, 1.000000000000000000, 1.000000000000000000, 1.000000000000000000, 1.000000000000000000, 1.000000000000000000, 1.000000000000000000, 1.000000000000000000, 1.000000000000000000) ) ) 
 REPRESENTATION_ITEM ( '' )  SURFACE ( )  );
#13866=CARTESIAN_POINT ( 'NONE',  ( -87.11181950073759594, -21.35018704950691060, -2.713672234369203018 ) ) ;
#13867=CARTESIAN_POINT ( 'NONE',  ( -77.90255099906859471, -8.644468104251766150, 20.04994828524300843 ) ) ;
#13869=CARTESIAN_POINT ( 'NONE',  ( -144.1957000270774927, 12.48102028655531903, 30.13184844817395458 ) ) ;
#13870=CARTESIAN_POINT ( 'NONE',  ( -4.112199523540041923, -23.43514144949427447, -42.98379141459099628 ) ) ;
#13871=CARTESIAN_POINT ( 'NONE',  ( 170.2234770963711128, 17.36149277827028925, -39.20704971665377059 ) ) ;
#13873=DIRECTION ( 'NONE',  ( 1.000000000000000000, 1.836970198721030181E-16, 0.000000000000000000 ) ) ;
#13874=CARTESIAN_POINT ( 'NONE',  ( 14.38125909742181818, -39.01709431150904095, -17.55144818341490165 ) ) ;
#13875=CARTESIAN_POINT ( 'NONE',  ( -259.2033419157646676, -40.00000000000017053, 9.517827891722212996 ) ) ;
#13876=DIRECTION ( 'NONE',  ( 0.000000000000000000, -1.000000000000000000, 0.000000000000000000 ) ) ;
#13877=CARTESIAN_POINT ( 'NONE',  ( -91.56559293963836410, 16.03295912088692177, 16.03295912088721664 ) ) ;
#13878=CARTESIAN_POINT ( 'NONE',  ( -198.0356074513804288, -55.37879056873077133, -2.449293598294708485E-15 ) ) ;
#13879=CARTESIAN_POINT ( 'NONE',  ( -162.0762913951021176, 27.08623940707598265, 29.48230308784781428 ) ) ;
#13880=CARTESIAN_POINT ( 'NONE',  ( 136.1360204305621551, -4.966164525587036138, -40.00000000000002132 ) ) ;
#13881=CARTESIAN_POINT ( 'NONE',  ( -89.92902785008674016, 20.44110050034136705, -8.088236460649897097 ) ) ;
#13883=CARTESIAN_POINT ( 'NONE',  ( 151.7948205124836534, 4.785054706298574878, -51.78348778862537927 ) ) ;
#13884=CARTESIAN_POINT ( 'NONE',  ( 146.6084372240433709, -34.62501878078303008, -40.00000000000002132 ) ) ;
#13885=VERTEX_POINT ( 'NONE', #20855 ) ;
#13886=CARTESIAN_POINT ( 'NONE',  ( 23.36462152323021613, -42.86003749000681040, 23.34178792078220965 ) ) ;
#13887=CARTESIAN_POINT ( 'NONE',  ( 135.5356265174576151, 12.51227922893862399, 30.20731421070357925 ) ) ;
#13889=CARTESIAN_POINT ( 'NONE',  ( 184.8905102610680444, 13.49065550809807945, 13.49065550809809544 ) ) ;
#13890=CARTESIAN_POINT ( 'NONE',  ( 4.995406935893305089, -40.00000000000021316, 55.24977328853194791 ) ) ;
#13891=CARTESIAN_POINT ( 'NONE',  ( 146.6084372240433993, -24.48358557860353457, 24.48358557860296258 ) ) ;
#13892=CARTESIAN_POINT ( 'NONE',  ( -56.48582580120559271, -9.153146818113595984, 0.000000000000000000 ) ) ;
#13893=CARTESIAN_POINT ( 'NONE',  ( 57.59792236341147031, -2.435789363418150444, 0.000000000000000000 ) ) ;
#13897=B_SPLINE_CURVE_WITH_KNOTS ( 'NONE', 3,
 ( #11250, #7130, #9125, #21248, #1026, #16982, #897, #6995, #7378, #5269, #15489, #10874, #15242, #5149, #25244, #4890, #1276, #19369, #1156, #21120, #20984, #17367, #25504, #2897, #15116, #23247 ),
 .UNSPECIFIED., .F., .F.,
 ( 4, 2, 1, 2, 2, 2, 2, 2, 2, 2, 2, 1, 2, 4 ),
 ( -5.999999998908891326E-08, 0.0004354487530732538848, 0.0008709575061464967880, 0.001741975012292981727, 0.003484010024585949654, 0.006968080049171881604, 0.01045215007375781269, 0.01393622009834374550, 0.02090436014751561114, 0.02438843017210155090, 0.02613046518439452251, 0.02700148269054100658, 0.02743699144361424341, 0.02787250019668748025 ),
 .UNSPECIFIED. ) ;
#13898=CARTESIAN_POINT ( 'NONE',  ( -86.96347745069644475, 12.89780903124419353, -12.89780903124389333 ) ) ;
#13899=CARTESIAN_POINT ( 'NONE',  ( 0.2972598230770027716, -38.42060263243681817, 18.14793986248684377 ) ) ;
#13900=CARTESIAN_POINT ( 'NONE',  ( -114.4364955367327781, 20.29001642038848274, -8.064892380842206165 ) ) ;
#13901=CARTESIAN_POINT ( 'NONE',  ( -87.13368444204334651, 14.72469439730582152, -15.67192210925590068 ) ) ;
#13902=CARTESIAN_POINT ( 'NONE',  ( 19.06497207195981858, -10.03556273973377166, -66.60410523465827737 ) ) ;
#13903=CARTESIAN_POINT ( 'NONE',  ( -280.0000000000000568, -42.42640687119305198, 14.14213562373058686 ) ) ;
#13904=CARTESIAN_POINT ( 'NONE',  ( -77.90255099907052738, 8.064892378688679031, 20.29001641119211641 ) ) ;
#13905=CARTESIAN_POINT ( 'NONE',  ( 4.995406935893297984, 10.78321810390233892, -67.35176059882522281 ) ) ;
#13909=CARTESIAN_POINT ( 'NONE',  ( -238.4067589809705794, -40.00000000000021316, 40.96449427990166470 ) ) ;
#13910=CARTESIAN_POINT ( 'NONE',  ( -280.0000000000000000, 14.14213562373098299, -14.14213562373088706 ) ) ;
#13911=CARTESIAN_POINT ( 'NONE',  ( -105.3755690713226727, 15.38646221621771737, 15.38646221621800514 ) ) ;
#13912=CARTESIAN_POINT ( 'NONE',  ( 184.8905102610680444, 19.07866798485561333, 40.00000000000002132 ) ) ;
#13914=CARTESIAN_POINT ( 'NONE',  ( 184.8905102610680444, -14.79361573936379415, -14.79361573936387941 ) ) ;
#13915=CARTESIAN_POINT ( 'NONE',  ( 9.807832026182905949, 43.71718838542761176, 18.10825233806385270 ) ) ;
#13916=CARTESIAN_POINT ( 'NONE',  ( 23.46661716382963192, 13.79413593526274262, 46.77475180958831658 ) ) ;
#13917=CARTESIAN_POINT ( 'NONE',  ( -105.3220005116004785, -5.373930277592323890, 20.73876282934741866 ) ) ;
#13918=ORIENTED_EDGE ( 'NONE', *, *, #12873, .F. ) ;
#13919=CARTESIAN_POINT ( 'NONE',  ( -191.2489946133628393, -43.85245824699192241, 18.16428294931126786 ) ) ;
#13922=CARTESIAN_POINT ( 'NONE',  ( 13.28449813596001228, -14.15462405556703018, 49.16593779330992220 ) ) ;
#13923=CARTESIAN_POINT ( 'NONE',  ( 25.88393124174635318, 22.82896322164242875, -42.08451360837176480 ) ) ;
#13925=CARTESIAN_POINT ( 'NONE',  ( 135.5356265174576151, -30.20731421070357214, 12.51227922893874656 ) ) ;
#13926=CARTESIAN_POINT ( 'NONE',  ( -121.8425463767455597, -9.420908037836060345, 22.74408395719867571 ) ) ;
#13927=CARTESIAN_POINT ( 'NONE',  ( 146.6084372240433709, 32.08495691632030145, 24.48358557860365181 ) ) ;
#13928=CARTESIAN_POINT ( 'NONE',  ( 19.06497207195982924, -54.19242893257843008, 40.00000000000002132 ) ) ;
#13929=CARTESIAN_POINT ( 'NONE',  ( 90.68848816920421996, -8.337973095858520978, -21.47805809303278934 ) ) ;
#13930=CARTESIAN_POINT ( 'NONE',  ( -192.9588430854689989, 10.23066800230756712, -10.23066800230735396 ) ) ;
#13931=CARTESIAN_POINT ( 'NONE',  ( 57.59792236341147031, 2.435789363418171760, 0.000000000000000000 ) ) ;
#13933=CARTESIAN_POINT ( 'NONE',  ( -91.56559293963836410, 22.67402823373189946, -0.000000000000000000 ) ) ;
#13934=CARTESIAN_POINT ( 'NONE',  ( -100.7734535825088500, -22.67402823373193499, 40.00000000000002132 ) ) ;
#13935=CARTESIAN_POINT ( 'NONE',  ( 4.995406935893298872, 5.820775922023080204E-13, -55.24977328854835434 ) ) ;
#13936=CARTESIAN_POINT ( 'NONE',  ( -135.8532207217289738, -1.208299557080134822E-13, 9.153146818113572891 ) ) ;
#13937=CARTESIAN_POINT ( 'NONE',  ( -30.26275506840325136, 27.08623969584614244, -29.48230279907770779 ) ) ;
#13938=ADVANCED_FACE ( 'NONE', ( #25247 ), #2306, .T. ) ;
#13939=ORIENTED_EDGE ( 'NONE', *, *, #13600, .T. ) ;
#13940=CARTESIAN_POINT ( 'NONE',  ( 98.29820294267416614, 12.20973600806160775, -15.89413956777835679 ) ) ;
#13941=CARTESIAN_POINT ( 'NONE',  ( 184.8905102610680444, 20.92133201514447549, 0.000000000000000000 ) ) ;
#13942=CARTESIAN_POINT ( 'NONE',  ( -189.4799703873391081, 47.39666448643376384, -13.88847319136868563 ) ) ;
#13945=ORIENTED_EDGE ( 'NONE', *, *, #16296, .F. ) ;
#13946=CARTESIAN_POINT ( 'NONE',  ( 4.995406935893297984, -39.06748935135182421, -17.50105314357212549 ) ) ;
#13947=CARTESIAN_POINT ( 'NONE',  ( 23.32574057153218305, -42.87194976637074717, -23.35062444423069294 ) ) ;
#13948=VERTEX_POINT ( 'NONE', #366 ) ;
#13949=CARTESIAN_POINT ( 'NONE',  ( -100.7734535825088500, -22.67402823373193499, -40.00000000000002132 ) ) ;
#13950=CARTESIAN_POINT ( 'NONE',  ( -114.4364955367322949, 8.644468109217019247, 20.04994829327305794 ) ) ;
#13955=CARTESIAN_POINT ( 'NONE',  ( -105.4741150117367283, 19.77569912955882359, -7.943527260733686646 ) ) ;
#13956=CARTESIAN_POINT ( 'NONE',  ( -162.0762913951021176, 29.48230308784768638, -27.08623940707612121 ) ) ;
#13957=CARTESIAN_POINT ( 'NONE',  ( -189.0540493709901568, -43.34488811517300633, -17.95404051684990776 ) ) ;
#13958=CARTESIAN_POINT ( 'NONE',  ( 57.59792236341149163, -40.00000000000014211, 37.56421063658172699 ) ) ;
#13959=CARTESIAN_POINT ( 'NONE',  ( -91.56559293963834989, -22.67402823373193499, 40.00000000000002132 ) ) ;
#13962=CARTESIAN_POINT ( 'NONE',  ( 91.82158438592158234, 7.693928927950222250E-14, -17.20528682183300262 ) ) ;
#13963=CARTESIAN_POINT ( 'NONE',  ( 4.995406935893306866, -39.99999999999944578, -55.24977328856505920 ) ) ;
#13965=CARTESIAN_POINT ( 'NONE',  ( -105.3755690713226585, 15.38646221621762678, 41.18208027870604582 ) ) ;
#13966=CARTESIAN_POINT ( 'NONE',  ( -91.56559293963836410, 22.67402823373189946, -0.000000000000000000 ) ) ;
#13967=CARTESIAN_POINT ( 'NONE',  ( -91.56559293963836410, -12.25131212657462321, -44.31723036834905827 ) ) ;
#13971=CARTESIAN_POINT ( 'NONE',  ( -100.7734535825088358, -2.560096224687585342E-13, 22.67402823373191723 ) ) ;
#13972=CARTESIAN_POINT ( 'NONE',  ( 57.59792236341147031, 1.908507979671054758E-14, -2.435789363418160658 ) ) ;
#13973=CARTESIAN_POINT ( 'NONE',  ( 200.0000000000000000, 42.42640687119288856, -14.14213562373094746 ) ) ;
#13975=CARTESIAN_POINT ( 'NONE',  ( -188.9478905404521640, -17.94277290414830262, -43.31768569177597783 ) ) ;
#13979=CARTESIAN_POINT ( 'NONE',  ( 200.0000000000000000, -42.42640687119272513, -14.14213562373140753 ) ) ;
#13980=CARTESIAN_POINT ( 'NONE',  ( -87.11144460458852734, -13.16695842547661499, -17.02332938628118342 ) ) ;
#13981=CARTESIAN_POINT ( 'NONE',  ( 163.1118516004056573, 19.27778845538780317, -19.27778845538757224 ) ) ;
#13982=CARTESIAN_POINT ( 'NONE',  ( -77.90255099906769942, -20.29001641120677846, -8.064892378658084837 ) ) ;
#13983=DIRECTION ( 'NONE',  ( 0.000000000000000000, -0.3995982397846142287, 0.9166903767145360149 ) ) ;
#13984=CARTESIAN_POINT ( 'NONE',  ( -162.0762913951020892, 1.198031840456041497, -57.76657433537918251 ) ) ;
#13985=( NAMED_UNIT ( * ) SI_UNIT ( $, .STERADIAN. ) SOLID_ANGLE_UNIT ( ) );
#13990=CARTESIAN_POINT ( 'NONE',  ( 3.468680970031286392, 14.11592159093371812, 48.91035688725572328 ) ) ;
#13992=ORIENTED_EDGE ( 'NONE', *, *, #9534, .T. ) ;
#13994=CARTESIAN_POINT ( 'NONE',  ( -259.2033419157646676, -6.730120644403570829, -6.730120644403545960 ) ) ;
#13996=FACE_OUTER_BOUND ( 'NONE', #26111, .T. ) ;
#13999=AXIS2_PLACEMENT_3D ( 'NONE', #11483, #7367, #4163 ) ;
#14000=CARTESIAN_POINT ( 'NONE',  ( -213.1075012329537230, 40.00000000000012790, -13.71589010951869980 ) ) ;
#14005=CARTESIAN_POINT ( 'NONE',  ( -184.2925746397123135, 41.26799595407793220, 17.09376361613362150 ) ) ;
#14006=CARTESIAN_POINT ( 'NONE',  ( -4.201409602818406697, -23.41774994521158249, -42.95750343186449527 ) ) ;
#14007=ADVANCED_FACE ( 'NONE', ( #21251 ), #5184, .T. ) ;
#14008=CARTESIAN_POINT ( 'NONE',  ( 170.2234770963711128, -10.92277846919187034, -10.92277846919209594 ) ) ;
#14009=CARTESIAN_POINT ( 'NONE',  ( -114.7826396787322665, -15.64922767586156915, -15.64922767586183383 ) ) ;
#14010=CARTESIAN_POINT ( 'NONE',  ( 136.1360204305621551, -31.79587985999244282, -24.77266263493140386 ) ) ;
#14011=CARTESIAN_POINT ( 'NONE',  ( -105.3755690713226585, -40.00000000000027711, 21.75974354311608749 ) ) ;
#14012=CARTESIAN_POINT ( 'NONE',  ( -280.0000000000000000, 14.14213562373078581, 14.14213562373108424 ) ) ;
#14013=CARTESIAN_POINT ( 'NONE',  ( -30.26275506840323004, -41.69427246844629309, 40.00000000000002132 ) ) ;
#14014=EDGE_CURVE ( 'NONE', #8031, #11219, #11310, .T. ) ;
#14016=CARTESIAN_POINT ( 'NONE',  ( 57.59792236341148453, -37.56421063658185489, -40.00000000000002132 ) ) ;
#14017=CARTESIAN_POINT ( 'NONE',  ( -103.9474983245025044, 20.15710290851490427, -8.027156558344678672 ) ) ;
#14019=CARTESIAN_POINT ( 'NONE',  ( -192.9588430854690273, 40.00000000000055422, -54.46834944101679810 ) ) ;
#14020=CARTESIAN_POINT ( 'NONE',  ( -238.4067589809705794, 28.96627169325324758, -27.60227080167054581 ) ) ;
#14021=CARTESIAN_POINT ( 'NONE',  ( 170.2234770963711128, 15.44714144992819627, -40.00000000000002132 ) ) ;
#14024=CARTESIAN_POINT ( 'NONE',  ( -208.1127848780264742, 15.00245453012665742, 40.00000000000002132 ) ) ;
#14025=DIRECTION ( 'NONE',  ( 1.000000000000000000, 0.000000000000000000, 0.000000000000000000 ) ) ;
#14026=( BOUNDED_SURFACE ( )  B_SPLINE_SURFACE ( 3, 3, ( 
 ( #4773, #18999, #6750, #2644, #9020, #7006, #7139, #12877, #21132, #10751, #25387, #21259, #4638, #9135, #24997, #15254, #20993, #14862, #510, #23257, #8615, #24857, #14729, #6611, #5033, #11140, #13140, #2907, #22861, #3031 ),
 ( #12740, #20860, #643, #8749, #2775, #11015, #10887, #16993, #19125, #8882, #25128, #907, #14994, #23129, #4901, #19896, #21631, #21386, #19379, #3670, #17501, #9786, #23384, #3536, #1417, #13264, #9518, #3158, #15626, #13508 ),
 ( #5531, #15498, #13766, #5158, #19634, #11508, #23628, #3407, #11260, #13383, #9394, #11778, #17624, #13637, #25768, #1166, #7518, #11380, #9269, #1681, #23749, #7774, #17888, #21763, #21510, #17377, #11636, #5278, #15382, #25516 ),
 ( #5407, #1286, #7263, #19759, #23504, #1549, #3282, #9653, #25641, #19501, #17758, #7387, #25899, #7640, #15755, #21893, #23883, #5660, #26037, #9917, #20036, #1814, #18023, #22037, #15889, #3809, #26172, #24017, #11914, #5796 ),
 ( #13903, #20758, #20892, #12631, #4800, #2528, #10774, #537, #21153, #3053, #13160, #17145, #18755, #22756, #10645, #14619, #4534, #6773, #2800, #16888, #12765, #19146, #931, #17274, #23025, #23150, #2669, #9162, #5054, #14754 ),
 ( #8642, #1056, #21280, #18887, #12901, #16751, #25020, #25408, #9040, #25279, #11158, #24885, #19273, #23278, #6640, #7033, #22884, #13035, #4663, #801, #2927, #666, #8775, #14885, #21017, #19022, #10911, #8906, #4924, #17016 ),
 ( #25152, #6903, #15150, #15020, #11036, #8925, #684, #8793, #2943, #17162, #21170, #22902, #13052, #23042, #24902, #15290, #9057, #19417, #21419, #4946, #6790, #6657, #15037, #16905, #25037, #14772, #4680, #12783, #20910, #19289 ) ),
 .UNSPECIFIED., .T., .F., .F. ) 
 B_SPLINE_SURFACE_WITH_KNOTS ( ( 4, 3, 4 ),
 ( 4, 2, 2, 2, 2, 2, 2, 2, 2, 2, 2, 2, 2, 2, 4 ),
 ( 0.000000000000000000, 0.5000000000000000000, 1.000000000000000000 ),
 ( 0.000000000000000000, 0.1357259735107005372, 0.1651108541090157700, 0.1944957347073310028, 0.3598804999793158710, 0.3867117631979620773, 0.4135430264166082281, 0.5789277916885930964, 0.6062785021374117456, 0.6336292125862302838, 0.8508620842112317728, 0.8814014469398914198, 0.9119408096685510667, 0.9559704048342755334, 1.000000000000000000 ),
 .UNSPECIFIED. ) 
 GEOMETRIC_REPRESENTATION_ITEM ( )  RATIONAL_B_SPLINE_SURFACE ( (
 ( 1.000000000000000000, 1.000000000000000000, 1.000000000000000000, 1.000000000000000000, 1.000000000000000000, 1.000000000000000000, 1.000000000000000000, 1.000000000000000000, 1.000000000000000000, 1.000000000000000000, 1.000000000000000000, 1.000000000000000000, 1.000000000000000000, 1.000000000000000000, 1.000000000000000000, 1.000000000000000000, 1.000000000000000000, 1.000000000000000000, 1.000000000000000000, 1.000000000000000000, 1.000000000000000000, 1.000000000000000000, 1.000000000000000000, 1.000000000000000000, 1.000000000000000000, 1.000000000000000000, 1.000000000000000000, 1.000000000000000000, 1.000000000000000000, 1.000000000000000000),
 ( 0.3333333333333333703, 0.3333333333333333703, 0.3333333333333333703, 0.3333333333333333703, 0.3333333333333333703, 0.3333333333333333703, 0.3333333333333333703, 0.3333333333333333703, 0.3333333333333333703, 0.3333333333333333703, 0.3333333333333333703, 0.3333333333333333703, 0.3333333333333333703, 0.3333333333333333703, 0.3333333333333333703, 0.3333333333333333703, 0.3333333333333333703, 0.3333333333333333703, 0.3333333333333333703, 0.3333333333333333703, 0.3333333333333333703, 0.3333333333333333703, 0.3333333333333333703, 0.3333333333333333703, 0.3333333333333333703, 0.3333333333333333703, 0.3333333333333333703, 0.3333333333333333703, 0.3333333333333333703, 0.3333333333333333703),
 ( 0.3333333333333333703, 0.3333333333333333703, 0.3333333333333333703, 0.3333333333333333703, 0.3333333333333333703, 0.3333333333333333703, 0.3333333333333333703, 0.3333333333333333703, 0.3333333333333333703, 0.3333333333333333703, 0.3333333333333333703, 0.3333333333333333703, 0.3333333333333333703, 0.3333333333333333703, 0.3333333333333333703, 0.3333333333333333703, 0.3333333333333333703, 0.3333333333333333703, 0.3333333333333333703, 0.3333333333333333703, 0.3333333333333333703, 0.3333333333333333703, 0.3333333333333333703, 0.3333333333333333703, 0.3333333333333333703, 0.3333333333333333703, 0.3333333333333333703, 0.3333333333333333703, 0.3333333333333333703, 0.3333333333333333703),
 ( 1.000000000000000000, 1.000000000000000000, 1.000000000000000000, 1.000000000000000000, 1.000000000000000000, 1.000000000000000000, 1.000000000000000000, 1.000000000000000000, 1.000000000000000000, 1.000000000000000000, 1.000000000000000000, 1.000000000000000000, 1.000000000000000000, 1.000000000000000000, 1.000000000000000000, 1.000000000000000000, 1.000000000000000000, 1.000000000000000000, 1.000000000000000000, 1.000000000000000000, 1.000000000000000000, 1.000000000000000000, 1.000000000000000000, 1.000000000000000000, 1.000000000000000000, 1.000000000000000000, 1.000000000000000000, 1.000000000000000000, 1.000000000000000000, 1.000000000000000000),
 ( 0.3333333333333333703, 0.3333333333333333703, 0.3333333333333333703, 0.3333333333333333703, 0.3333333333333333703, 0.3333333333333333703, 0.3333333333333333703, 0.3333333333333333703, 0.3333333333333333703, 0.3333333333333333703, 0.3333333333333333703, 0.3333333333333333703, 0.3333333333333333703, 0.3333333333333333703, 0.3333333333333333703, 0.3333333333333333703, 0.3333333333333333703, 0.3333333333333333703, 0.3333333333333333703, 0.3333333333333333703, 0.3333333333333333703, 0.3333333333333333703, 0.3333333333333333703, 0.3333333333333333703, 0.3333333333333333703, 0.3333333333333333703, 0.3333333333333333703, 0.3333333333333333703, 0.3333333333333333703, 0.3333333333333333703),
 ( 0.3333333333333333703, 0.3333333333333333703, 0.3333333333333333703, 0.3333333333333333703, 0.3333333333333333703, 0.3333333333333333703, 0.3333333333333333703, 0.3333333333333333703, 0.3333333333333333703, 0.3333333333333333703, 0.3333333333333333703, 0.3333333333333333703, 0.3333333333333333703, 0.3333333333333333703, 0.3333333333333333703, 0.3333333333333333703, 0.3333333333333333703, 0.3333333333333333703, 0.3333333333333333703, 0.3333333333333333703, 0.3333333333333333703, 0.3333333333333333703, 0.3333333333333333703, 0.3333333333333333703, 0.3333333333333333703, 0.3333333333333333703, 0.3333333333333333703, 0.3333333333333333703, 0.3333333333333333703, 0.3333333333333333703),
 ( 1.000000000000000000, 1.000000000000000000, 1.000000000000000000, 1.000000000000000000, 1.000000000000000000, 1.000000000000000000, 1.000000000000000000, 1.000000000000000000, 1.000000000000000000, 1.000000000000000000, 1.000000000000000000, 1.000000000000000000, 1.000000000000000000, 1.000000000000000000, 1.000000000000000000, 1.000000000000000000, 1.000000000000000000, 1.000000000000000000, 1.000000000000000000, 1.000000000000000000, 1.000000000000000000, 1.000000000000000000, 1.000000000000000000, 1.000000000000000000, 1.000000000000000000, 1.000000000000000000, 1.000000000000000000, 1.000000000000000000, 1.000000000000000000, 1.000000000000000000) ) ) 
 REPRESENTATION_ITEM ( '' )  SURFACE ( )  );
#14027=CARTESIAN_POINT ( 'NONE',  ( 4.995406935893287326, 67.35176059882533650, 10.78321810390163549 ) ) ;
#14028=CARTESIAN_POINT ( 'NONE',  ( 146.6084372240433709, -39.99999999999987921, -34.62501878078319351 ) ) ;
#14029=CARTESIAN_POINT ( 'NONE',  ( 151.7948205124836534, 4.785054706297857230, 51.78348778862544322 ) ) ;
#14030=CARTESIAN_POINT ( 'NONE',  ( -208.1127848780265026, 15.00245453012665564, 0.000000000000000000 ) ) ;
#14031=CARTESIAN_POINT ( 'NONE',  ( 130.8568914410475372, -34.05028731879786363, 0.000000000000000000 ) ) ;
#14035=CARTESIAN_POINT ( 'NONE',  ( -280.0000000000000000, 14.14213562373108246, -14.14213562373078581 ) ) ;
#14036=CARTESIAN_POINT ( 'NONE',  ( 19.06497207195982924, -66.60410523465809263, -10.03556273973493163 ) ) ;
#14038=CARTESIAN_POINT ( 'NONE',  ( 170.2234770963711128, -39.20704971665404059, 17.36149277826957160 ) ) ;
#14040=CARTESIAN_POINT ( 'NONE',  ( -135.8532207217289738, -34.75652343174584757, -21.81201906317816253 ) ) ;
#14041=ADVANCED_FACE ( 'NONE', ( #1279 ), #18982, .F. ) ;
#14042=CARTESIAN_POINT ( 'NONE',  ( -280.0000000000000568, -14.14213562373078226, -42.42640687119295251 ) ) ;
#14045=CARTESIAN_POINT ( 'NONE',  ( -56.48582580120557850, -40.00000000000014211, 30.84685318188629921 ) ) ;
#14046=B_SPLINE_CURVE_WITH_KNOTS ( 'NONE', 3,
 ( #1571, #23649, #7286, #15401, #23526, #17523, #7538, #23775, #5553, #7407, #11661, #19785 ),
 .UNSPECIFIED., .F., .F.,
 ( 4, 2, 2, 2, 2, 4 ),
 ( 5.045153280873417672E-16, 0.004698945756007614528, 0.007048418634011168957, 0.009397891512014724252, 0.01409683726802183311, 0.01879578302402894197 ),
 .UNSPECIFIED. ) ;
#14047=CARTESIAN_POINT ( 'NONE',  ( -100.7734535825088500, 16.03295912088691821, 16.03295912088721309 ) ) ;
#14048=CARTESIAN_POINT ( 'NONE',  ( 2.303792037526079639, 44.43800799081192565, -18.40682559463163415 ) ) ;
#14049=CARTESIAN_POINT ( 'NONE',  ( 184.8905102610680444, 19.07866798485562043, 2.449293598294708485E-15 ) ) ;
#14051=CARTESIAN_POINT ( 'NONE',  ( 14.38125909742180752, 10.73282306404720465, 10.73282306404724018 ) ) ;
#14054=CARTESIAN_POINT ( 'NONE',  ( 91.82158438592158234, -17.20528682183298486, 0.000000000000000000 ) ) ;
#14056=CARTESIAN_POINT ( 'NONE',  ( -194.7885354600801975, -44.44047100927770799, 18.40784581028790612 ) ) ;
#14057=AXIS2_PLACEMENT_3D ( 'NONE', #21373, #3141, #6864 ) ;
#14061=CARTESIAN_POINT ( 'NONE',  ( 6.202588568023359450, -14.15973318136377301, 49.19971320596261677 ) ) ;
#14062=CARTESIAN_POINT ( 'NONE',  ( 23.32574057153200187, 23.35062444423039807, -42.87194976637071164 ) ) ;
#14064=CARTESIAN_POINT ( 'NONE',  ( 149.5797498300190398, -29.41965740490887882, 12.18602109748309559 ) ) ;
#14065=CARTESIAN_POINT ( 'NONE',  ( -185.5190930961058484, -17.55874694108397804, 42.39056500340862499 ) ) ;
#14066=CARTESIAN_POINT ( 'NONE',  ( -238.4067589809705794, 28.96627169325354956, -28.96627169325289231 ) ) ;
#14067=CARTESIAN_POINT ( 'NONE',  ( -87.02160487651677556, -5.405486468710360981, 20.76754707253114063 ) ) ;
#14069=CARTESIAN_POINT ( 'NONE',  ( -192.1964066538111808, 24.16259023443393517, -43.96877160661179573 ) ) ;
#14070=CARTESIAN_POINT ( 'NONE',  ( -56.48582580120559271, -6.472252184284276844, 6.472252184284108978 ) ) ;
#14071=CARTESIAN_POINT ( 'NONE',  ( 184.8905102610680444, 20.92133201514447549, 0.000000000000000000 ) ) ;
#14072=CARTESIAN_POINT ( 'NONE',  ( 19.06497207195980792, -14.19242893257839988, -40.00000000000002132 ) ) ;
#14074=CARTESIAN_POINT ( 'NONE',  ( -105.3755690713226585, -21.75974354311652448, 40.00000000000002132 ) ) ;
#14075=CARTESIAN_POINT ( 'NONE',  ( 151.7948205124836534, 40.00000000000012079, -6.767089262348609857 ) ) ;
#14076=CARTESIAN_POINT ( 'NONE',  ( -162.0762913951020892, 29.48230308784758691, 29.48230308784772191 ) ) ;
#14078=CARTESIAN_POINT ( 'NONE',  ( 151.7948205124835681, 51.78348778862544322, -4.785054706298002891 ) ) ;
#14080=CARTESIAN_POINT ( 'NONE',  ( 4.995406935893289102, 10.78321810388998081, 10.78321810389001811 ) ) ;
#14081=CARTESIAN_POINT ( 'NONE',  ( -86.86493150571118349, -8.366608963954250910, 19.60045294882748124 ) ) ;
#14084=CARTESIAN_POINT ( 'NONE',  ( 163.1118516004056573, -37.29075403953139300, -19.27778845539249630 ) ) ;
#14085=CARTESIAN_POINT ( 'NONE',  ( 22.81400246987437441, -43.16348862150560706, -17.87890238636475360 ) ) ;
#14086=ORIENTED_EDGE ( 'NONE', *, *, #25603, .T. ) ;
#14087=CARTESIAN_POINT ( 'NONE',  ( 192.4448373802101173, 19.99999999996065014, -40.00000000000002132 ) ) ;
#14088=FACE_OUTER_BOUND ( 'NONE', #25594, .T. ) ;
#14089=ORIENTED_EDGE ( 'NONE', *, *, #21579, .F. ) ;
#14092=CARTESIAN_POINT ( 'NONE',  ( -105.2333882009265693, 21.31109190976440715, -2.724924291338312266 ) ) ;
#14093=EDGE_CURVE ( 'NONE', #9873, #7172, #14183, .T. ) ;
#14094=CARTESIAN_POINT ( 'NONE',  ( -198.0356074513804572, 10.87444709759714989, 10.87444709759722450 ) ) ;
#14095=CARTESIAN_POINT ( 'NONE',  ( -188.2871287166140917, -43.00155302796438406, -23.44689273421207076 ) ) ;
#14096=CARTESIAN_POINT ( 'NONE',  ( -198.0356074513804572, -40.00000000000011369, 15.37879056873056527 ) ) ;
#14097=CARTESIAN_POINT ( 'NONE',  ( 14.38125909742180752, 15.17850393972634038, 40.00000000000002132 ) ) ;
#14100=CARTESIAN_POINT ( 'NONE',  ( 184.8905102610680444, 1.070102760522089011E-13, -20.92133201514444352 ) ) ;
#14101=CARTESIAN_POINT ( 'NONE',  ( -105.3755690713226585, -40.00000000000010658, 18.24025645688337249 ) ) ;
#14102=CARTESIAN_POINT ( 'NONE',  ( -86.96347745069644475, -2.438961472018186339E-13, 21.75974354311649961 ) ) ;
#14103=CARTESIAN_POINT ( 'NONE',  ( 19.06497207195979726, 39.99999999999997158, 14.19242893257854554 ) ) ;
#14104=CARTESIAN_POINT ( 'NONE',  ( -105.2333497862889686, -16.99530394072478856, 13.14348404883646815 ) ) ;
#14105=CARTESIAN_POINT ( 'NONE',  ( 14.38125909742182529, -39.01709431150933938, 39.01709431150894147 ) ) ;
#14106=CARTESIAN_POINT ( 'NONE',  ( -86.96347745069645896, 21.75974354311648895, -0.000000000000000000 ) ) ;
#14108=CARTESIAN_POINT ( 'NONE',  ( -259.2033419157646676, -49.83842185052031937, -6.730120644403796426 ) ) ;
#14110=EDGE_CURVE ( 'NONE', #6927, #3040, #6885, .T. ) ;
#14112=CARTESIAN_POINT ( 'NONE',  ( 57.59792236341147031, -1.493297263419786540E-14, 2.435789363418160658 ) ) ;
#14113=CARTESIAN_POINT ( 'NONE',  ( 170.2234770963711128, -40.00000000000004263, 15.44714144992801685 ) ) ;
#14114=CARTESIAN_POINT ( 'NONE',  ( -192.9588430854690273, 66.79921049721887982, 10.23066800229522677 ) ) ;
#14116=CARTESIAN_POINT ( 'NONE',  ( -114.4098922876147384, 20.15198150140922451, 8.347224046571190215 ) ) ;
#14117=CARTESIAN_POINT ( 'NONE',  ( -188.9001659262688690, -17.93767091109449652, -43.30536839095078250 ) ) ;
#14118=FACE_OUTER_BOUND ( 'NONE', #19913, .T. ) ;
#14119=ORIENTED_EDGE ( 'NONE', *, *, #22424, .F. ) ;
#14120=CARTESIAN_POINT ( 'NONE',  ( -213.1075012329537230, 9.698598906450543566, -9.698598906450348167 ) ) ;
#14121=CARTESIAN_POINT ( 'NONE',  ( -259.2033419157646676, 9.517827891722584255, -0.000000000000000000 ) ) ;
#14123=CARTESIAN_POINT ( 'NONE',  ( 0.2972598230770011618, 10.13633138497555919, -66.70487387989845729 ) ) ;
#14124=CARTESIAN_POINT ( 'NONE',  ( -77.55640685880874230, 0.6928334182872019076, 22.13135000835299593 ) ) ;
#14125=ORIENTED_EDGE ( 'NONE', *, *, #10379, .F. ) ;
#14127=CARTESIAN_POINT ( 'NONE',  ( 21.15138808362599221, -23.80076113581848318, 43.47948264999429568 ) ) ;
#14128=CARTESIAN_POINT ( 'NONE',  ( -4.339409867980440261, 17.83714383556808869, 43.06267456183103093 ) ) ;
#14130=ORIENTED_EDGE ( 'NONE', *, *, #10058, .F. ) ;
#14131=CARTESIAN_POINT ( 'NONE',  ( -192.9588430854689989, 10.23066800230742679, 10.23066800230749607 ) ) ;
#14136=CARTESIAN_POINT ( 'NONE',  ( -105.3755690713226585, 39.99999999999977263, 21.75974354311691883 ) ) ;
#14137=CARTESIAN_POINT ( 'NONE',  ( 98.29820294267415193, 2.605266741687827903, -19.87244099730190072 ) ) ;
#14138=CARTESIAN_POINT ( 'NONE',  ( -82.28158677657542341, -19.22558455003817102, -6.254308823251737870 ) ) ;
#14139=DIRECTION ( 'NONE',  ( 0.9698969544100564111, 0.09318942523058482141, 0.2249791742612868850 ) ) ;
#14142=CARTESIAN_POINT ( 'NONE',  ( -4.037857402784335470, -23.44963359339763898, -43.00569567200361831 ) ) ;
#14143=CARTESIAN_POINT ( 'NONE',  ( 184.8905102610680444, 14.79361573936424890, -41.77492675555986068 ) ) ;
#14144=CARTESIAN_POINT ( 'NONE',  ( 200.0000000000000000, 60.00000000000007816, 7.960204194457792519E-15 ) ) ;
#14145=CARTESIAN_POINT ( 'NONE',  ( -238.4067589809705794, -28.96627169325343942, 28.96627169325309126 ) ) ;
#14148=CARTESIAN_POINT ( 'NONE',  ( 192.4448373802101173, -19.99999999996057554, 40.00000000000002132 ) ) ;
#14150=CARTESIAN_POINT ( 'NONE',  ( -259.2033419157646676, -30.48217210827744239, -2.449293598294708485E-15 ) ) ;
#14151=CARTESIAN_POINT ( 'NONE',  ( -110.1014694628346575, 14.86203413257348771, 13.68874972777938304 ) ) ;
#14152=CARTESIAN_POINT ( 'NONE',  ( -100.7734535825088500, 40.00000000000017764, -17.32597176626768487 ) ) ;
#14153=CARTESIAN_POINT ( 'NONE',  ( 146.6084372240433709, 3.800685668858776900, -52.76785682606518435 ) ) ;
#14154=CARTESIAN_POINT ( 'NONE',  ( -208.1127848780265026, 15.00245453012665564, 0.000000000000000000 ) ) ;
#14155=ORIENTED_EDGE ( 'NONE', *, *, #23310, .T. ) ;
#14156=ORIENTED_EDGE ( 'NONE', *, *, #944, .F. ) ;
#14157=CARTESIAN_POINT ( 'NONE',  ( -192.9588430854690273, 14.46834944099966336, 40.00000000000002132 ) ) ;
#14158=CARTESIAN_POINT ( 'NONE',  ( 151.0853911467767432, 12.04115959307956452, 29.06993079631229548 ) ) ;
#14159=CARTESIAN_POINT ( 'NONE',  ( -30.26275506840323359, -1.535832457777009877E-13, 41.69427246844629309 ) ) ;
#14160=CARTESIAN_POINT ( 'NONE',  ( -86.96347745069644475, 12.89780903124349898, 43.67073346367994446 ) ) ;
#14163=CARTESIAN_POINT ( 'NONE',  ( 170.0000000000428315, 17.64300463311351308, -17.64300463311329992 ) ) ;
#14166=CARTESIAN_POINT ( 'NONE',  ( 170.2234770963711128, 10.92277846919216522, -10.92277846919186501 ) ) ;
#14167=CARTESIAN_POINT ( 'NONE',  ( 57.59792236341148453, -54.84617931850879557, 1.722363176414566155 ) ) ;
#14169=CARTESIAN_POINT ( 'NONE',  ( -77.59243545050232171, 13.54949188064891530, -17.47199274921711876 ) ) ;
#14170=CARTESIAN_POINT ( 'NONE',  ( 192.4448373802100889, -14.14213562370293431, -14.14213562370322030 ) ) ;
#14171=CARTESIAN_POINT ( 'NONE',  ( -30.26275506840324070, 1.198031551616030033, -1.198031551616006496 ) ) ;
#14172=CARTESIAN_POINT ( 'NONE',  ( 136.1360204305621551, -53.05693388239309627, -3.511608612531332163 ) ) ;
#14173=CARTESIAN_POINT ( 'NONE',  ( 91.82158438592156813, -16.11829626348402655, -40.45024623143966380 ) ) ;
#14176=CARTESIAN_POINT ( 'NONE',  ( 19.06497207195981858, -1.881589693694111225E-13, 54.19242893257843008 ) ) ;
#14178=CARTESIAN_POINT ( 'NONE',  ( 23.38399212876566935, 46.80460545930672822, -13.80022400692470974 ) ) ;
#14179=CARTESIAN_POINT ( 'NONE',  ( 184.8905102610680444, 19.07866798485562398, -40.00000000000002132 ) ) ;
#14181=CARTESIAN_POINT ( 'NONE',  ( -105.3755690713226727, -15.38646221621786481, -15.38646221621789856 ) ) ;
#14183=( BOUNDED_CURVE ( )  B_SPLINE_CURVE ( 3, ( #13502, #3400, #7512, #15620 ),
 .UNSPECIFIED., .F., .F. ) 
 B_SPLINE_CURVE_WITH_KNOTS ( ( 4, 4 ),
 ( 0.01388163287021833454, 0.02359082919310023091 ),
 .UNSPECIFIED. ) 
 CURVE ( )  GEOMETRIC_REPRESENTATION_ITEM ( )  RATIONAL_B_SPLINE_CURVE ( ( 1.000000000000000000, 0.8672072324488980799, 0.7608653435686176802, 0.6809743333591588010 ) ) 
 REPRESENTATION_ITEM ( '' )  );
#14184=CARTESIAN_POINT ( 'NONE',  ( -70.35386311763890888, -22.51194464688922636, 10.19784241824625681 ) ) ;
#14185=CARTESIAN_POINT ( 'NONE',  ( -213.1075012329537230, 13.71589010951907817, 40.00000000000002132 ) ) ;
#14186=EDGE_CURVE ( 'NONE', #10069, #12261, #924, .T. ) ;
#14188=CARTESIAN_POINT ( 'NONE',  ( 22.68416413276406729, 23.49220544186221105, -43.06288726621002638 ) ) ;
#14190=CARTESIAN_POINT ( 'NONE',  ( 6.371015797575695139, -18.55864253218550530, 44.80452650039092788 ) ) ;
#14193=CARTESIAN_POINT ( 'NONE',  ( 23.32574057153225056, 13.80366151303488031, -46.82643129194528342 ) ) ;
#14195=CARTESIAN_POINT ( 'NONE',  ( 35.93702929055792339, -42.26928858464287231, 12.87541766862415571 ) ) ;
#14198=CARTESIAN_POINT ( 'NONE',  ( 199.9999999999999432, 14.14213562373110911, -14.14213562373072364 ) ) ;
#14199=CARTESIAN_POINT ( 'NONE',  ( -102.2610585947572872, -22.27377874548545833, 0.000000000000000000 ) ) ;
#14200=CARTESIAN_POINT ( 'NONE',  ( -188.3392995398497192, 23.45797413244903495, -43.01688924973676365 ) ) ;
#14201=CARTESIAN_POINT ( 'NONE',  ( 0.2972598230769938343, 10.13633138497486286, -10.13633138497461594 ) ) ;
#14203=CARTESIAN_POINT ( 'NONE',  ( 91.82158438592159655, -22.79471317813468545, -2.449293598294708485E-15 ) ) ;
#14204=CARTESIAN_POINT ( 'NONE',  ( -30.26275506840324425, 41.69427246844627177, 40.00000000000002132 ) ) ;
#14205=CARTESIAN_POINT ( 'NONE',  ( -30.26275506840323359, -39.99999999999959499, -41.69427246844670520 ) ) ;
#14206=CARTESIAN_POINT ( 'NONE',  ( -100.7734535825088500, 40.53558337403677569, -16.03295912088699993 ) ) ;
#14207=CARTESIAN_POINT ( 'NONE',  ( 98.29820294268671432, 20.00000000000122213, -2.727061086135174062 ) ) ;
#14208=CARTESIAN_POINT ( 'NONE',  ( -192.9588430854689989, -10.23066800230742501, -10.23066800230756712 ) ) ;
#14210=CARTESIAN_POINT ( 'NONE',  ( 57.59792236341147031, -1.722363176415032004, -1.722363176415048880 ) ) ;
#14213=ORIENTED_EDGE ( 'NONE', *, *, #7999, .F. ) ;
#14215=CARTESIAN_POINT ( 'NONE',  ( -162.0762913951021176, -29.48230308784755493, -27.08623940707632372 ) ) ;
#14216=CARTESIAN_POINT ( 'NONE',  ( 60.07376046255615876, -31.81923430144854237, -13.17995839187771701 ) ) ;
#14217=ORIENTED_EDGE ( 'NONE', *, *, #970, .F. ) ;
#14218=CARTESIAN_POINT ( 'NONE',  ( 146.6084372240433709, -34.62501878078303008, -40.00000000000002132 ) ) ;
#14219=CARTESIAN_POINT ( 'NONE',  ( -99.31267923333899716, -20.62886818714040515, 8.544756979565530486 ) ) ;
#14223=CARTESIAN_POINT ( 'NONE',  ( 91.82158438592158234, 16.11829626348434630, -40.45024623143955012 ) ) ;
#14224=CARTESIAN_POINT ( 'NONE',  ( -184.9730489279452570, -42.02334742175309401, -22.80026000643668382 ) ) ;
#14225=CARTESIAN_POINT ( 'NONE',  ( -100.7734535825088500, -39.99999999999995737, -22.67402823373205578 ) ) ;
#14226=CARTESIAN_POINT ( 'NONE',  ( 184.8905102610680444, -20.92133201514440799, 40.00000000000002132 ) ) ;
#14229=CARTESIAN_POINT ( 'NONE',  ( 0.2972598230769957217, -4.999556039334937811E-14, 14.33493731733933352 ) ) ;
#14230=CARTESIAN_POINT ( 'NONE',  ( 170.2234770963711128, -2.511315425431857630E-14, 15.44714144992816074 ) ) ;
#14231=CARTESIAN_POINT ( 'NONE',  ( -91.56559293963836410, 40.00000000000008527, -22.67402823373177867 ) ) ;
#14232=CARTESIAN_POINT ( 'NONE',  ( -91.56559293963836410, 22.67402823373190301, -40.00000000000002132 ) ) ;
#14233=CARTESIAN_POINT ( 'NONE',  ( -162.0762913951020892, -29.48230308784785692, 29.48230308784751230 ) ) ;
#14234=CARTESIAN_POINT ( 'NONE',  ( 136.1360204305621266, 35.03383547441298873, 0.000000000000000000 ) ) ;
#14235=CARTESIAN_POINT ( 'NONE',  ( 146.6084372240433709, -32.08495691632041513, -24.48358557860343154 ) ) ;
#14238=CARTESIAN_POINT ( 'NONE',  ( 130.8568914410475372, 24.07718906447210472, 24.07718906447249907 ) ) ;
#14239=CARTESIAN_POINT ( 'NONE',  ( 184.8905102610680444, -3.509827109981123710E-14, 19.07866798485558490 ) ) ;
#14240=CARTESIAN_POINT ( 'NONE',  ( 14.38125909742181108, 39.01709431150907648, 39.01709431150921858 ) ) ;
#14241=CARTESIAN_POINT ( 'NONE',  ( 163.1118516004056573, -9.006482792074626431, 47.56205970284951690 ) ) ;
#14242=CARTESIAN_POINT ( 'NONE',  ( -188.3611024622183265, -13.83140737835580580, -47.01268868734971562 ) ) ;
#14243=CARTESIAN_POINT ( 'NONE',  ( -105.3755690713226727, 15.38646221621793231, -15.38646221621779020 ) ) ;
#14244=ORIENTED_EDGE ( 'NONE', *, *, #24271, .F. ) ;
#14245=CARTESIAN_POINT ( 'NONE',  ( -135.8532207217289738, -34.75652343174584757, -21.81201906317816253 ) ) ;
#14247=CARTESIAN_POINT ( 'NONE',  ( -162.0762913951020892, -1.694272876828353702, 0.000000000000000000 ) ) ;
#14249=CARTESIAN_POINT ( 'NONE',  ( -238.4067589809705794, 0.6820004458491113475, -57.25054294077229144 ) ) ;
#14251=CARTESIAN_POINT ( 'NONE',  ( -83.21262154144250189, 13.72187187061492075, 33.12752917118417173 ) ) ;
#14253=VERTEX_POINT ( 'NONE', #3506 ) ;
#14256=CARTESIAN_POINT ( 'NONE',  ( 17.76569343199600226, -24.33587863439579024, 44.20364726159875346 ) ) ;
#14257=CARTESIAN_POINT ( 'NONE',  ( -1.087763065865680279, 13.97201973057867619, 47.95583523901584755 ) ) ;
#14260=CARTESIAN_POINT ( 'NONE',  ( 130.8568914410475372, -34.05028731879786363, 0.000000000000000000 ) ) ;
#14265=CARTESIAN_POINT ( 'NONE',  ( -97.73806390046838999, -8.581719943991895860, -20.71810467719076598 ) ) ;
#14266=CARTESIAN_POINT ( 'NONE',  ( -56.48582580120559982, 40.00000000000034106, -30.84685318188602210 ) ) ;
#14267=CARTESIAN_POINT ( 'NONE',  ( 98.29820294267348402, 5.160908283043466938, -19.33391160836868750 ) ) ;
#14273=CARTESIAN_POINT ( 'NONE',  ( -3.856733984653721414, -17.89110409353214948, -43.19294614843406777 ) ) ;
#14274=CARTESIAN_POINT ( 'NONE',  ( -192.9588430854690273, -66.79921049721887982, -10.23066800229569040 ) ) ;
#14275=CARTESIAN_POINT ( 'NONE',  ( -114.7539999570855400, -13.57343626010274740, -17.50303175002473566 ) ) ;
#14276=CARTESIAN_POINT ( 'NONE',  ( 151.7948205124836534, -33.06932595376343897, -23.49921654116042902 ) ) ;
#14278=CARTESIAN_POINT ( 'NONE',  ( 163.1118516004056573, 27.26290988616875310, 0.000000000000000000 ) ) ;
#14279=CARTESIAN_POINT ( 'NONE',  ( -213.1075012329537230, -13.71589010951915810, 40.00000000000002132 ) ) ;
#14280=CARTESIAN_POINT ( 'NONE',  ( -200.0000000000000000, 75.00000000000000000, 0.000000000000000000 ) ) ;
#14281=CARTESIAN_POINT ( 'NONE',  ( -105.3755690713226585, -18.24025645688355013, 40.00000000000002132 ) ) ;
#14282=CARTESIAN_POINT ( 'NONE',  ( -114.7122376710347424, 18.03507107370589679, 12.72361799391042858 ) ) ;
#14283=CARTESIAN_POINT ( 'NONE',  ( -162.0762913951020892, 4.094006889353306706E-13, -41.69427287682835015 ) ) ;
#14284=CARTESIAN_POINT ( 'NONE',  ( 184.8905102610680444, 13.49065550809817715, -43.07788698682574591 ) ) ;
#14285=ADVANCED_FACE ( 'NONE', ( #9487 ), #7482, .T. ) ;
#14286=CARTESIAN_POINT ( 'NONE',  ( 163.1118516004056573, -27.26290988616869626, 0.000000000000000000 ) ) ;
#14289=ORIENTED_EDGE ( 'NONE', *, *, #14753, .T. ) ;
#14290=CARTESIAN_POINT ( 'NONE',  ( -135.8532207217289738, -9.153146818113595984, 0.000000000000000000 ) ) ;
#14291=CARTESIAN_POINT ( 'NONE',  ( 169.9999999999999716, -22.62041470344880523, -9.369682556672316309 ) ) ;
#14292=( BOUNDED_CURVE ( )  B_SPLINE_CURVE ( 3, ( #37, #12532, #20403, #24931 ),
 .UNSPECIFIED., .F., .F. ) 
 B_SPLINE_CURVE_WITH_KNOTS ( ( 4, 4 ),
 ( 0.01388163287021780372, 0.02359082919310006438 ),
 .UNSPECIFIED. ) 
 CURVE ( )  GEOMETRIC_REPRESENTATION_ITEM ( )  RATIONAL_B_SPLINE_CURVE ( ( 1.000000000000000000, 0.8672072324488987460, 0.7608653435686186794, 0.6809743333591599113 ) ) 
 REPRESENTATION_ITEM ( '' )  );
#14293=CARTESIAN_POINT ( 'NONE',  ( 170.2234770963711128, 40.00000000000000000, 15.44714144992830462 ) ) ;
#14294=CARTESIAN_POINT ( 'NONE',  ( -100.7734535825088500, 40.53558337403654832, 16.03295912088756481 ) ) ;
#14295=CARTESIAN_POINT ( 'NONE',  ( 192.4448373802100889, -1.741373372144848397E-13, 20.00000000003942091 ) ) ;
#14301=CARTESIAN_POINT ( 'NONE',  ( -135.8532207217289738, 50.09629031063956006, 6.472252184284782217 ) ) ;
#14302=CARTESIAN_POINT ( 'NONE',  ( 146.6084372240433709, -32.08495691632075619, 24.48358557860298035 ) ) ;
#14304=CARTESIAN_POINT ( 'NONE',  ( -280.0000000000000568, 39.99999999999976552, 20.00000000000043343 ) ) ;
#14305=CARTESIAN_POINT ( 'NONE',  ( 151.7948205124836534, -33.06932595376376582, 23.49921654115996006 ) ) ;
#14306=CARTESIAN_POINT ( 'NONE',  ( -87.12803293485033862, 14.20621343982535834, -16.13817828096302165 ) ) ;
#14307=CARTESIAN_POINT ( 'NONE',  ( 184.8905102610680444, -14.79361573936399665, 14.79361573936367158 ) ) ;
#14308=CARTESIAN_POINT ( 'NONE',  ( 0.2972598230769976091, -10.13633138497479180, 10.13633138497468522 ) ) ;
#14311=CARTESIAN_POINT ( 'NONE',  ( -56.48582580120558561, -1.205267837095813407E-13, 30.84685318188644132 ) ) ;
#14313=CARTESIAN_POINT ( 'NONE',  ( 22.13784119383518600, 43.34234508276902176, -17.95298715833884629 ) ) ;
#14314=CARTESIAN_POINT ( 'NONE',  ( 91.82158438592158234, 22.79471317813472098, 2.449293598294708485E-15 ) ) ;
#14316=CARTESIAN_POINT ( 'NONE',  ( -2.937533998801357349, -23.68967259551906324, -43.32931883107454496 ) ) ;
#14318=CARTESIAN_POINT ( 'NONE',  ( -24.88648382771808798, -39.69105101982836459, 12.31763033300906152 ) ) ;
#14319=CARTESIAN_POINT ( 'NONE',  ( -135.8532207217289738, 30.84685318188643066, 2.449293598294708485E-15 ) ) ;
#14324=CARTESIAN_POINT ( 'NONE',  ( 2.332272417610701698, -14.08759251168401860, 48.72342300853175345 ) ) ;
#14325=B_SPLINE_CURVE_WITH_KNOTS ( 'NONE', 3,
 ( #21341, #23464, #23708, #11590, #3112, #11217, #1244, #25854, #13587, #9225, #17334, #25468, #11341, #7219, #15335, #13340 ),
 .UNSPECIFIED., .F., .F.,
 ( 4, 2, 2, 2, 2, 2, 2, 4 ),
 ( -5.998499567629515208E-08, 0.003520343011582079042, 0.007040746008159834424, 0.01408155200131533044, 0.01760195499789308018, 0.02112235799447082646, 0.02464276099104857620, 0.02816316398762632248 ),
 .UNSPECIFIED. ) ;
#14326=CARTESIAN_POINT ( 'NONE',  ( 2.692156443674271760, 18.42752958144669506, -44.48799183654966782 ) ) ;
#14328=CARTESIAN_POINT ( 'NONE',  ( -86.96347745069644475, -2.438961472018186339E-13, 21.75974354311649961 ) ) ;
#14330=CARTESIAN_POINT ( 'NONE',  ( -166.3490736463351993, -12.23457872950100267, 39.29841219613869896 ) ) ;
#14332=CARTESIAN_POINT ( 'NONE',  ( -91.56559293963834989, 12.25131212657497848, -12.25131212657469426 ) ) ;
#14333=CARTESIAN_POINT ( 'NONE',  ( -105.3895334812061293, 9.637394427376211326, -19.08270859416220944 ) ) ;
#14334=CARTESIAN_POINT ( 'NONE',  ( -189.6939645179747629, 18.01965094556769387, -43.50328570201348555 ) ) ;
#14335=CARTESIAN_POINT ( 'NONE',  ( 4.995406935893283773, 39.06748935135171052, 17.50105314357239195 ) ) ;
#14336=CARTESIAN_POINT ( 'NONE',  ( 199.9999999999999432, -14.14213562373115884, 14.14213562373085153 ) ) ;
#14337=CARTESIAN_POINT ( 'NONE',  ( 19.06497207195982924, -54.19242893257843008, -40.00000000000002132 ) ) ;
#14338=CARTESIAN_POINT ( 'NONE',  ( -56.48582580120559271, 30.84685318188643066, 2.449293598294708485E-15 ) ) ;
#14340=CARTESIAN_POINT ( 'NONE',  ( 146.6084372240433709, -40.00000000000036238, 34.62501878078263218 ) ) ;
#14341=CARTESIAN_POINT ( 'NONE',  ( -91.56559293963834989, 12.25131212657480440, 12.25131212657486834 ) ) ;
#14342=( BOUNDED_SURFACE ( )  B_SPLINE_SURFACE ( 3, 2, ( 
 ( #1598, #11686, #19676 ),
 ( #9565, #20216, #15937 ),
 ( #17940, #22085, #11824 ),
 ( #8096, #15676, #17675 ),
 ( #18202, #14219, #25817 ),
 ( #13689, #26086, #22355 ),
 ( #21484, #19942, #16216 ),
 ( #7821, #7563, #21810 ),
 ( #7961, #5980, #4133 ),
 ( #24070, #17806, #3858 ),
 ( #7694, #16079, #3995 ),
 ( #15806, #23931, #24207 ) ),
 .UNSPECIFIED., .F., .F., .F. ) 
 B_SPLINE_SURFACE_WITH_KNOTS ( ( 4, 2, 2, 2, 2, 4 ),
 ( 3, 3 ),
 ( 0.006022589392323847955, 0.01254516766564278685, 0.01580645680230225586, 0.01906774593896172487, 0.02559032421228066290, 0.03211290248559960092 ),
 ( 0.000000000000000000, 1.000000000000000000 ),
 .UNSPECIFIED. ) 
 GEOMETRIC_REPRESENTATION_ITEM ( )  RATIONAL_B_SPLINE_SURFACE ( (
 ( 1.000000000000000000, 0.9998834880171260098, 1.000000000000000000),
 ( 1.000000000000000000, 0.9998139205012248620, 1.000000000000000000),
 ( 1.000000000000000000, 0.9997315632444678801, 1.000000000000000000),
 ( 1.000000000000000000, 0.9996405464946959141, 1.000000000000000000),
 ( 1.000000000000000000, 0.9996155081777534646, 1.000000000000000000),
 ( 1.000000000000000000, 0.9995814087510496160, 1.000000000000000000),
 ( 1.000000000000000000, 0.9995724100939920032, 1.000000000000000000),
 ( 1.000000000000000000, 0.9995726760936896049, 1.000000000000000000),
 ( 1.000000000000000000, 0.9996103361817947341, 1.000000000000000000),
 ( 1.000000000000000000, 0.9997312749795597142, 1.000000000000000000),
 ( 1.000000000000000000, 0.9998135910915183500, 1.000000000000000000),
 ( 1.000000000000000000, 0.9998834880173385065, 1.000000000000000000) ) ) 
 REPRESENTATION_ITEM ( '' )  SURFACE ( )  );
#14343=CARTESIAN_POINT ( 'NONE',  ( 98.29820294267403824, -2.605266741685067888, 19.87244099730234481 ) ) ;
#14344=CARTESIAN_POINT ( 'NONE',  ( -91.56559293963834989, -12.25131212657475466, -12.25131212657495361 ) ) ;
#14348=CARTESIAN_POINT ( 'NONE',  ( -259.2033419157646676, -35.01439189186554302, 21.55415060305832498 ) ) ;
#14349=CARTESIAN_POINT ( 'NONE',  ( -89.91646883265939039, 8.407637968706790588, 20.29783361022716193 ) ) ;
#14351=CARTESIAN_POINT ( 'NONE',  ( -86.96347745069643054, -41.18208027870589660, -15.38646221621809040 ) ) ;
#14352=CARTESIAN_POINT ( 'NONE',  ( 8.556015491681991492, -49.31947911770831894, -14.17785852676117209 ) ) ;
#14354=CARTESIAN_POINT ( 'NONE',  ( 199.9999999999999432, -20.00000000000006750, 0.000000000000000000 ) ) ;
#14355=CARTESIAN_POINT ( 'NONE',  ( -82.30220482034326324, -7.992411108785252516, -18.51665893431348309 ) ) ;
#14356=ORIENTED_EDGE ( 'NONE', *, *, #16711, .T. ) ;
#14359=CARTESIAN_POINT ( 'NONE',  ( 200.0000000000000000, 14.14213562373100608, -42.42640687119291698 ) ) ;
#14360=CARTESIAN_POINT ( 'NONE',  ( -188.6013942375920749, -43.09289976588301840, -23.51434495930372393 ) ) ;
#14361=CARTESIAN_POINT ( 'NONE',  ( 192.4448373802101173, -39.99999999999991473, -20.00000000003956302 ) ) ;
#14362=CARTESIAN_POINT ( 'NONE',  ( -86.96347745069644475, -21.75974354311651737, 0.000000000000000000 ) ) ;
#14365=CARTESIAN_POINT ( 'NONE',  ( 192.4448373802101173, -39.99999999999991473, -20.00000000003956302 ) ) ;
#14366=CARTESIAN_POINT ( 'NONE',  ( 192.4448373802101173, -39.99999999999991473, -20.00000000003956302 ) ) ;
#14367=CARTESIAN_POINT ( 'NONE',  ( 151.7948205124836534, 40.00000000000002842, 6.767089262349174739 ) ) ;
#14368=CARTESIAN_POINT ( 'NONE',  ( 163.1118516004056573, 27.26290988616875310, 0.000000000000000000 ) ) ;
#14369=CARTESIAN_POINT ( 'NONE',  ( 57.59792236341148453, -26.56190807104700369, 26.56190807104673723 ) ) ;
#14370=CARTESIAN_POINT ( 'NONE',  ( -162.0762913951020607, -41.69427287682838568, -2.449293598294708485E-15 ) ) ;
#14371=CARTESIAN_POINT ( 'NONE',  ( 192.4448373802101173, 14.14213562375862665, 42.42640687116509213 ) ) ;
#14372=CARTESIAN_POINT ( 'NONE',  ( -163.5815475687390403, 12.03526863292960236, 38.33196416462965317 ) ) ;
#14373=CARTESIAN_POINT ( 'NONE',  ( -188.2995950289364657, -23.44932284466040784, 43.00522595870950937 ) ) ;
#14374=CARTESIAN_POINT ( 'NONE',  ( -91.56559293963836410, 40.00000000000019185, -17.32597176626768487 ) ) ;
#14375=CARTESIAN_POINT ( 'NONE',  ( 200.0000000000000000, -40.00000000000005684, 19.99999999999978328 ) ) ;
#14376=CARTESIAN_POINT ( 'NONE',  ( 19.06497207195981147, 38.31983398719620482, 38.31983398719633271 ) ) ;
#14379=CARTESIAN_POINT ( 'NONE',  ( -208.1127848780264742, -67.17687982763172272, 10.60833733270744617 ) ) ;
#14380=EDGE_CURVE ( 'NONE', #2026, #5206, #20693, .T. ) ;
#14382=CARTESIAN_POINT ( 'NONE',  ( -105.3755690713226727, -15.38646221621807619, 15.38646221621768362 ) ) ;
#14383=CARTESIAN_POINT ( 'NONE',  ( -83.87175289014592749, 19.20738476421698238, 7.955959267057188811 ) ) ;
#14384=CARTESIAN_POINT ( 'NONE',  ( 170.2234770963711128, -15.44714144992812699, -40.00000000000002132 ) ) ;
#14385=DIRECTION ( 'NONE',  ( 0.9352143328345648987, -0.3271292286618222023, -0.1355013631515235850 ) ) ;
#14386=CARTESIAN_POINT ( 'NONE',  ( 91.82158438592158234, -12.16597498397778843, 12.16597498397750954 ) ) ;
#14388=ORIENTED_EDGE ( 'NONE', *, *, #3799, .T. ) ;
#14391=CARTESIAN_POINT ( 'NONE',  ( -77.90255099906769942, -8.644468104261466834, -20.04994828523962980 ) ) ;
#14392=CARTESIAN_POINT ( 'NONE',  ( 23.26364522860060191, 13.80713620122610941, 46.84987168987027673 ) ) ;
#14393=ORIENTED_EDGE ( 'NONE', *, *, #2327, .T. ) ;
#14395=CARTESIAN_POINT ( 'NONE',  ( -162.0762913951020892, 1.198031840385716418, 1.198031840385750169 ) ) ;
#14397=CARTESIAN_POINT ( 'NONE',  ( -198.0012401002533977, -44.79720214428356684, 24.77357857137259955 ) ) ;
#14399=B_SPLINE_CURVE_WITH_KNOTS ( 'NONE', 3,
 ( #15267, #21398, #11274, #1179, #19646, #1430, #17006, #9281 ),
 .UNSPECIFIED., .F., .F.,
 ( 4, 2, 2, 4 ),
 ( 0.0002278873370217108000, 0.004309043385688178691, 0.006349621410021411526, 0.008390199434354645228 ),
 .UNSPECIFIED. ) ;
#14401=CARTESIAN_POINT ( 'NONE',  ( -99.31364972223276766, -8.164808577092738773, -20.79869444142337187 ) ) ;
#14402=CARTESIAN_POINT ( 'NONE',  ( -56.48582580120558561, 3.151766524733697544E-13, -30.84685318188644132 ) ) ;
#14403=CARTESIAN_POINT ( 'NONE',  ( -198.0356074513804572, 1.247057299367198800E-13, -15.37879056873070560 ) ) ;
#14404=CARTESIAN_POINT ( 'NONE',  ( -175.9234132798436292, 42.70618380303040595, -12.95567000669884905 ) ) ;
#14405=CARTESIAN_POINT ( 'NONE',  ( -16.41582555442421665, -21.03675245956757323, 39.35881747731896496 ) ) ;
#14407=CARTESIAN_POINT ( 'NONE',  ( -184.9729924863079020, 13.59277144552584815, 45.83719276897330985 ) ) ;
#14408=CARTESIAN_POINT ( 'NONE',  ( 23.42154907652914630, -23.32998349128497750, -42.84253412640330794 ) ) ;
#14409=CARTESIAN_POINT ( 'NONE',  ( -238.4067589809705794, -57.25054294077233408, -0.6820004458489551391 ) ) ;
#14410=CARTESIAN_POINT ( 'NONE',  ( -86.86493150571116928, 19.60045294882758071, -8.366608963953975575 ) ) ;
#14411=CARTESIAN_POINT ( 'NONE',  ( -91.56559293963836410, 44.31723036834890905, 12.25131212657507795 ) ) ;
#14412=CARTESIAN_POINT ( 'NONE',  ( -77.55640685876512919, -9.396736996787174904E-14, 22.13135000837103661 ) ) ;
#14413=CARTESIAN_POINT ( 'NONE',  ( 170.2234770963711128, 17.36149277826980253, 17.36149277827007253 ) ) ;
#14414=CARTESIAN_POINT ( 'NONE',  ( 0.2972598230769983307, -14.33493731733933352, 40.00000000000002132 ) ) ;
#14416=CARTESIAN_POINT ( 'NONE',  ( -56.48582580120558561, -30.84685318188645908, 40.00000000000002132 ) ) ;
#14417=CARTESIAN_POINT ( 'NONE',  ( -105.4282329516590977, 9.018643079774772531, 19.35470593465534250 ) ) ;
#14418=CARTESIAN_POINT ( 'NONE',  ( 151.7948205124836534, 40.00000000000012079, -6.767089262348609857 ) ) ;
#14419=CARTESIAN_POINT ( 'NONE',  ( 4.995406935893283773, 39.06748935135195211, -17.50105314357185193 ) ) ;
#14420=CARTESIAN_POINT ( 'NONE',  ( 0.2972598230769930017, 14.33493731733933352, -40.00000000000002132 ) ) ;
#14423=CARTESIAN_POINT ( 'NONE',  ( 136.1360204305621266, -35.03383547441293899, 0.000000000000000000 ) ) ;
#14425=AXIS2_PLACEMENT_3D ( 'NONE', #17479, #15479, #19611 ) ;
#14426=CARTESIAN_POINT ( 'NONE',  ( -86.96347745069644475, 41.18208027870576871, 15.38646221621837107 ) ) ;
#14427=CARTESIAN_POINT ( 'NONE',  ( -105.2502192157103877, -21.20168261174586988, 3.402547493086664154 ) ) ;
#14428=ADVANCED_FACE ( 'NONE', ( #13601 ), #21494, .T. ) ;
#14429=CARTESIAN_POINT ( 'NONE',  ( 146.6084372240433993, -34.62501878078303008, 0.000000000000000000 ) ) ;
#14434=CARTESIAN_POINT ( 'NONE',  ( 192.4448373802101173, 14.14213562370261279, 42.42640687122091236 ) ) ;
#14435=CARTESIAN_POINT ( 'NONE',  ( 146.6084372240433993, -3.800685668858596156, -3.800685668858692967 ) ) ;
#14436=CARTESIAN_POINT ( 'NONE',  ( -105.2334388082176844, 21.30961024024002626, 2.995222947295622440 ) ) ;
#14437=CARTESIAN_POINT ( 'NONE',  ( -162.0762913951021176, 40.00000000000042633, -41.69427287672947102 ) ) ;
#14438=CARTESIAN_POINT ( 'NONE',  ( 91.82158438592159655, -16.11829626346125011, -16.11829626346154853 ) ) ;
#14440=CARTESIAN_POINT ( 'NONE',  ( -213.1075012329537230, 9.698598906450410340, 9.698598906450483170 ) ) ;
#14441=EDGE_CURVE ( 'NONE', #15233, #5232, #18130, .T. ) ;
#14442=CARTESIAN_POINT ( 'NONE',  ( 14.38125909742181818, -39.01709431150904095, -17.55144818341490165 ) ) ;
#14444=CIRCLE ( 'NONE', #13999, 14.99999999999999645 ) ;
#14445=EDGE_CURVE ( 'NONE', #15843, #19424, #5073, .T. ) ;
#14447=CARTESIAN_POINT ( 'NONE',  ( -192.9588430854689989, -2.280704836619014309E-13, 54.46834944099972375 ) ) ;
#14449=CARTESIAN_POINT ( 'NONE',  ( 23.64688638900486595, 46.70960658758650652, -13.78084749393357811 ) ) ;
#14450=CARTESIAN_POINT ( 'NONE',  ( -30.26275506840324425, 41.69427246844628598, -40.00000000000002132 ) ) ;
#14451=CARTESIAN_POINT ( 'NONE',  ( -280.0000000000000000, 19.99999999999996092, -0.000000000000000000 ) ) ;
#14452=CARTESIAN_POINT ( 'NONE',  ( -91.56559293963834989, -16.03295912088706388, -16.03295912088710651 ) ) ;
#14453=CARTESIAN_POINT ( 'NONE',  ( -5.866564133086563437, -46.35727274689649136, 13.69896896866318592 ) ) ;
#14454=CARTESIAN_POINT ( 'NONE',  ( -162.0762913951021176, 41.69427287672986182, 40.00000000000002132 ) ) ;
#14457=CARTESIAN_POINT ( 'NONE',  ( -213.1075012329537230, 9.698598906450410340, 9.698598906450483170 ) ) ;
#14458=CARTESIAN_POINT ( 'NONE',  ( -5.859158571325972176, -23.09435402965430129, 42.46836465823860607 ) ) ;
#14459=CARTESIAN_POINT ( 'NONE',  ( 8.556015491705554865, 24.84887822174884064, -44.89939803569809129 ) ) ;
#14461=CARTESIAN_POINT ( 'NONE',  ( -16.41654234031583570, -42.70586891223516091, -12.95560590424196690 ) ) ;
#14462=CARTESIAN_POINT ( 'NONE',  ( 144.1620285550791323, -30.21661402164567889, 12.51613133675847678 ) ) ;
#14463=CARTESIAN_POINT ( 'NONE',  ( -190.7346372394825380, -23.92885340724453158, 43.65255821758466936 ) ) ;
#14464=CARTESIAN_POINT ( 'NONE',  ( 91.82158438592158234, -12.16597498399995203, -44.40256751092347542 ) ) ;
#14465=CARTESIAN_POINT ( 'NONE',  ( -188.2957210513757218, 23.44847782072239184, -43.00408675155262728 ) ) ;
#14466=CARTESIAN_POINT ( 'NONE',  ( 57.59792236341147031, 26.56190807104652052, 30.00663442387728708 ) ) ;
#14467=CARTESIAN_POINT ( 'NONE',  ( 14.38125909742180220, 39.01709431150892016, 17.55144818341517166 ) ) ;
#14468=CARTESIAN_POINT ( 'NONE',  ( -213.1075012329536946, -53.71589010951918652, -2.449293598294708485E-15 ) ) ;
#14469=CARTESIAN_POINT ( 'NONE',  ( 151.7948205124836534, 6.767089262349056611, 40.00000000000002132 ) ) ;
#14470=CARTESIAN_POINT ( 'NONE',  ( 19.06497207195981858, -39.99999999999987210, -14.19242893257882621 ) ) ;
#14471=CARTESIAN_POINT ( 'NONE',  ( -238.4067589809705794, 28.96627169325315165, 28.96627169325329731 ) ) ;
#14472=CARTESIAN_POINT ( 'NONE',  ( -88.37877758184212951, 20.15391234942320509, -8.026456973658891769 ) ) ;
#14473=CARTESIAN_POINT ( 'NONE',  ( -192.9588430854690273, -10.23066800231931239, -66.79921049724377724 ) ) ;
#14474=CARTESIAN_POINT ( 'NONE',  ( 200.0000000000000000, 42.42640687119290988, 14.14213562373111976 ) ) ;
#14475=ORIENTED_EDGE ( 'NONE', *, *, #15195, .F. ) ;
#14476=DIRECTION ( 'NONE',  ( 0.000000000000000000, -1.000000000000000000, 0.000000000000000000 ) ) ;
#14477=AXIS2_PLACEMENT_3D ( 'NONE', #2718, #24801, #17066 ) ;
#14478=CARTESIAN_POINT ( 'NONE',  ( -88.37877758183735466, 8.575405934691293197, 19.92653024471085033 ) ) ;
#14479=CARTESIAN_POINT ( 'NONE',  ( -192.9588430854689705, -38.51493924976963967, 38.51493924976919914 ) ) ;
#14480=CARTESIAN_POINT ( 'NONE',  ( -4.061681315507726708, -42.99867639910917916, -23.44498947467575789 ) ) ;
#14482=CARTESIAN_POINT ( 'NONE',  ( 184.8905102610680444, -20.92133201514440799, 0.000000000000000000 ) ) ;
#14483=CARTESIAN_POINT ( 'NONE',  ( -82.23726319249651340, -14.28014421912411080, -14.28014421912424581 ) ) ;
#14485=ORIENTED_EDGE ( 'NONE', *, *, #24547, .F. ) ;
#14487=CARTESIAN_POINT ( 'NONE',  ( 22.27434459962515234, 13.86259002496867154, -47.22399357564341926 ) ) ;
#14488=CARTESIAN_POINT ( 'NONE',  ( -188.2507053402904660, -42.99082124348477407, -23.43979243030716475 ) ) ;
#14489=CARTESIAN_POINT ( 'NONE',  ( -30.26275506840324070, -40.00000000000003553, 1.694272468446120117 ) ) ;
#14490=CARTESIAN_POINT ( 'NONE',  ( -192.9588430854690273, 54.46834944098218756, -40.00000000000002132 ) ) ;
#14495=CARTESIAN_POINT ( 'NONE',  ( 57.59792236341147742, -1.230234673553095937E-13, 37.56421063658186199 ) ) ;
#14496=CARTESIAN_POINT ( 'NONE',  ( -198.0356074513804572, 39.99999999999992895, 15.37879056873084771 ) ) ;
#14497=DIRECTION ( 'NONE',  ( 0.000000000000000000, 1.000000000000000000, 0.000000000000000000 ) ) ;
#14498=FACE_OUTER_BOUND ( 'NONE', #4853, .T. ) ;
#14499=CARTESIAN_POINT ( 'NONE',  ( -208.1127848780264742, -55.00245453010926866, 40.00000000000002132 ) ) ;
#14500=CARTESIAN_POINT ( 'NONE',  ( 19.06497207195981858, -10.03556273973469715, 66.60410523465813526 ) ) ;
#14501=CARTESIAN_POINT ( 'NONE',  ( -30.26275506840324070, 1.218738420030236455E-14, -1.694272468446259783 ) ) ;
#14503=CARTESIAN_POINT ( 'NONE',  ( 4.995406935893291767, 40.00000000000059686, -55.24977328853165659 ) ) ;
#14504=CARTESIAN_POINT ( 'NONE',  ( -208.1127848780264742, -40.00000000000025580, 55.00245453014408525 ) ) ;
#14507=CARTESIAN_POINT ( 'NONE',  ( -105.4741150117383341, -8.366608964593364561, -19.60045294982747777 ) ) ;
#14508=CARTESIAN_POINT ( 'NONE',  ( -259.2033419157646676, -49.83842185052031937, -6.730120644403796426 ) ) ;
#14510=CARTESIAN_POINT ( 'NONE',  ( 170.2234770963711128, -17.36149277827010096, 17.36149277826970660 ) ) ;
#14511=CARTESIAN_POINT ( 'NONE',  ( 146.5090579137182374, 29.94463907179421369, -12.40347562390439329 ) ) ;
#14512=CARTESIAN_POINT ( 'NONE',  ( 184.8905102610680444, -19.07866798485553872, -40.00000000000002132 ) ) ;
#14513=CARTESIAN_POINT ( 'NONE',  ( -114.7252611291635702, 17.87002000140834568, -12.98773421616931856 ) ) ;
#14514=CARTESIAN_POINT ( 'NONE',  ( 163.1118516004056573, -19.27778845538787422, 19.27778845538743724 ) ) ;
#14515=ORIENTED_EDGE ( 'NONE', *, *, #9534, .F. ) ;
#14519=CARTESIAN_POINT ( 'NONE',  ( 118.9130007099546873, 10.68958087202350704, -25.80693111732284351 ) ) ;
#14520=CARTESIAN_POINT ( 'NONE',  ( 21.60666276258909591, 18.00814241471010391, 43.47550165074856920 ) ) ;
#14524=CARTESIAN_POINT ( 'NONE',  ( -238.4067589809705794, 0.6820004457340470561, 57.25054294065803617 ) ) ;
#14526=CARTESIAN_POINT ( 'NONE',  ( -105.3846709043738628, 6.705972854959187934, 20.33574920591904700 ) ) ;
#14527=CARTESIAN_POINT ( 'NONE',  ( 91.82158438592158234, -12.16597498397761967, -12.16597498397768007 ) ) ;
#14528=CARTESIAN_POINT ( 'NONE',  ( -162.0762913951020892, 57.76657433537918251, 1.198031840455469066 ) ) ;
#14529=CARTESIAN_POINT ( 'NONE',  ( -109.1264249741455927, -33.12752917269520481, -13.72187187123273411 ) ) ;
#14531=ADVANCED_FACE ( 'NONE', ( #20270 ), #19619, .T. ) ;
#14532=CARTESIAN_POINT ( 'NONE',  ( -99.31267923333118119, -8.544756979489637416, -20.62886818714801507 ) ) ;
#14533=CARTESIAN_POINT ( 'NONE',  ( 170.2234770963711128, 1.955190573858485757E-13, -15.44714144992816074 ) ) ;
#14534=CARTESIAN_POINT ( 'NONE',  ( 146.6084372240433709, 39.99999999999968026, 34.62501878078347772 ) ) ;
#14539=CARTESIAN_POINT ( 'NONE',  ( -188.3065677117054122, 13.82848612971594804, 46.99298756134906085 ) ) ;
#14540=CARTESIAN_POINT ( 'NONE',  ( -30.26275506840324070, -1.198031551616016266, -1.198031551616031587 ) ) ;
#14541=CARTESIAN_POINT ( 'NONE',  ( 98.29820294267436509, 14.14213562374297695, -14.14213562372651189 ) ) ;
#14542=CARTESIAN_POINT ( 'NONE',  ( -86.96347745069643054, 15.38646221621763210, 41.18208027870604582 ) ) ;
#14544=CARTESIAN_POINT ( 'NONE',  ( -198.0356074513804572, -10.87444709758429262, -67.44298959250878056 ) ) ;
#14546=CARTESIAN_POINT ( 'NONE',  ( -56.48582580120559271, 9.153146818113576444, -0.000000000000000000 ) ) ;
#14547=CARTESIAN_POINT ( 'NONE',  ( -86.96347745069644475, -15.38646221621807442, 15.38646221621768184 ) ) ;
#14548=CARTESIAN_POINT ( 'NONE',  ( -30.26275506840324425, -1.694272468446265334, 40.00000000000002132 ) ) ;
#14550=CARTESIAN_POINT ( 'NONE',  ( 19.06497207195980792, 40.00000000000059686, -54.19242893257802507 ) ) ;
#14552=CARTESIAN_POINT ( 'NONE',  ( 140.2235668266256141, -12.60094438999861666, 30.42137084504290812 ) ) ;
#14553=EDGE_LOOP ( 'NONE', ( #17132, #5236 ) ) ;
#14555=CARTESIAN_POINT ( 'NONE',  ( 91.82158438592158234, -17.20528682183298486, 0.000000000000000000 ) ) ;
#14556=CARTESIAN_POINT ( 'NONE',  ( 154.0339099654742654, 11.67508747798851587, 28.18615453125295645 ) ) ;
#14557=CARTESIAN_POINT ( 'NONE',  ( 192.4448373802101173, 42.42640687116487896, 14.14213562375934075 ) ) ;
#14559=CARTESIAN_POINT ( 'NONE',  ( -190.1935349183499397, -43.51927535257652835, -23.83022391594517586 ) ) ;
#14563=CARTESIAN_POINT ( 'NONE',  ( 0.2972598230769990524, -18.14793986248671231, -38.42060263243687501 ) ) ;
#14564=CARTESIAN_POINT ( 'NONE',  ( 192.4448373802100889, 14.14213562375873678, 14.14213562375894817 ) ) ;
#14566=CARTESIAN_POINT ( 'NONE',  ( 192.4448373802100889, -1.741373372144848397E-13, 20.00000000003942091 ) ) ;
#14567=CARTESIAN_POINT ( 'NONE',  ( -100.7734535825088500, -40.53558337403692491, 16.03295912088671571 ) ) ;
#14568=CARTESIAN_POINT ( 'NONE',  ( -86.96347745069645896, 21.75974354311648895, -0.000000000000000000 ) ) ;
#14569=CARTESIAN_POINT ( 'NONE',  ( 151.7948205124836250, -23.49921654116371883, 23.49921654116317526 ) ) ;
#14570=CARTESIAN_POINT ( 'NONE',  ( 57.59792236341147031, 1.722363176415065089, -1.722363176415036445 ) ) ;
#14574=CARTESIAN_POINT ( 'NONE',  ( 0.2972598230770030492, -1.921041075453695163E-13, 54.33493731733936016 ) ) ;
#14576=CARTESIAN_POINT ( 'NONE',  ( 23.17367289775668837, 42.91822977676283557, -23.38495170326041617 ) ) ;
#14577=CARTESIAN_POINT ( 'NONE',  ( -100.7734535825088358, 17.32597176626809343, 2.449293598294708485E-15 ) ) ;
#14579=CARTESIAN_POINT ( 'NONE',  ( -162.0762913951021176, 1.694272876828294194, 40.00000000000002132 ) ) ;
#14580=CARTESIAN_POINT ( 'NONE',  ( -70.35386311710972507, -23.12931224182874956, 8.707385197621585249 ) ) ;
#14581=CARTESIAN_POINT ( 'NONE',  ( 200.0000000000000000, -20.00000000000006750, 40.00000000000002132 ) ) ;
#14582=EDGE_LOOP ( 'NONE', ( #12621, #698, #22315, #18744, #24737 ) ) ;
#14583=CARTESIAN_POINT ( 'NONE',  ( -200.0000000000000000, 43.94911113647449241, 34.07282666716778152 ) ) ;
#14584=CARTESIAN_POINT ( 'NONE',  ( -105.3755690713226585, -43.67073346367983788, 12.89780903124397149 ) ) ;
#14587=CARTESIAN_POINT ( 'NONE',  ( -3.534370630407255742, 17.92707699455486292, -43.27979241395905774 ) ) ;
#14589=CARTESIAN_POINT ( 'NONE',  ( 146.6084372240433993, -24.48358557860353457, 24.48358557860296258 ) ) ;
#14590=CARTESIAN_POINT ( 'NONE',  ( -87.02123777076587885, -20.76518631980179563, 5.414077845906299480 ) ) ;
#14591=CARTESIAN_POINT ( 'NONE',  ( -188.2652746676491233, -23.44263257803716627, 42.99511404081857080 ) ) ;
#14592=CARTESIAN_POINT ( 'NONE',  ( 57.59792236341148453, -40.00000000000003553, 2.435789363417741438 ) ) ;
#14593=CARTESIAN_POINT ( 'NONE',  ( -105.3755690713226585, -43.67073346367964604, -12.89780903124457545 ) ) ;
#14594=CARTESIAN_POINT ( 'NONE',  ( 57.59792236341147031, 2.435789363418171760, 0.000000000000000000 ) ) ;
#14595=CARTESIAN_POINT ( 'NONE',  ( -188.6890294954778824, 13.84869711777474954, -47.12920239600426697 ) ) ;
#14596=CARTESIAN_POINT ( 'NONE',  ( -192.9588430854690273, 66.79921049724377724, -10.23066800231904239 ) ) ;
#14597=CARTESIAN_POINT ( 'NONE',  ( 136.1360204305621266, -24.77266263493151044, 24.77266263493093135 ) ) ;
#14598=CARTESIAN_POINT ( 'NONE',  ( 163.1118516004056573, -12.73709011382471878, -40.00000000000002132 ) ) ;
#14599=CARTESIAN_POINT ( 'NONE',  ( 4.995406935893288214, 55.24977328853207581, 40.00000000000002132 ) ) ;
#14600=CARTESIAN_POINT ( 'NONE',  ( -208.1127848780265026, 1.189126717069624012E-13, -15.00245453012669472 ) ) ;
#14601=CARTESIAN_POINT ( 'NONE',  ( -213.1075012329537230, 37.98287015391228749, 37.98287015391245802 ) ) ;
#14602=CARTESIAN_POINT ( 'NONE',  ( -100.0957100001388937, 20.56213589530717911, -8.517115559260082236 ) ) ;
#14603=CARTESIAN_POINT ( 'NONE',  ( 136.1360204305621266, -3.511608612530630058, -3.511608612530719764 ) ) ;
#14604=CARTESIAN_POINT ( 'NONE',  ( -114.7252611291633997, 3.452297386453677230, 21.81972725943348834 ) ) ;
#14606=CARTESIAN_POINT ( 'NONE',  ( -162.0762913951021176, -27.08623940707624911, 29.48230308784761888 ) ) ;
#14607=CARTESIAN_POINT ( 'NONE',  ( 192.4448373802101173, 14.14213562375862665, 42.42640687116509213 ) ) ;
#14608=CARTESIAN_POINT ( 'NONE',  ( -3.786831587088177020, -47.08106124085814059, -13.84155926340365639 ) ) ;
#14611=CARTESIAN_POINT ( 'NONE',  ( -200.0000000000000284, -30.70179486994606677, 44.88127304974057097 ) ) ;
#14614=DIRECTION ( 'NONE',  ( -1.000000000000000000, -1.836970198721024264E-16, 0.000000000000000000 ) ) ;
#14615=CARTESIAN_POINT ( 'NONE',  ( -91.56559293963834989, -7.976292724337646577E-14, 17.32597176626811120 ) ) ;
#14616=CARTESIAN_POINT ( 'NONE',  ( -238.4067589809705794, 40.96449428006337001, -40.00000000000002132 ) ) ;
#14619=CARTESIAN_POINT ( 'NONE',  ( 0.2972598230770153171, -66.70487387989849992, -10.13633138497533004 ) ) ;
#14620=CARTESIAN_POINT ( 'NONE',  ( 151.7948205124836250, 1.807796684091926154E-15, 6.767089262349031742 ) ) ;
#14621=CARTESIAN_POINT ( 'NONE',  ( -86.96347745069645896, 40.00000000000008527, -21.75974354311636461 ) ) ;
#14623=CARTESIAN_POINT ( 'NONE',  ( -105.3755690713226585, 21.75974354311648185, -40.00000000000002132 ) ) ;
#14624=CARTESIAN_POINT ( 'NONE',  ( 0.2972598230770129857, -54.33493731733936016, -40.00000000000002132 ) ) ;
#14625=CARTESIAN_POINT ( 'NONE',  ( -86.96347745069643054, 15.38646221621763210, 41.18208027870604582 ) ) ;
#14626=CARTESIAN_POINT ( 'NONE',  ( -259.2033419157646676, -1.473088368616265084E-13, 9.517827891722632216 ) ) ;
#14627=FACE_OUTER_BOUND ( 'NONE', #19984, .T. ) ;
#14628=CARTESIAN_POINT ( 'NONE',  ( -86.96347745069644475, 1.775309070576523494E-13, -18.24025645688352881 ) ) ;
#14629=CARTESIAN_POINT ( 'NONE',  ( -192.9588430854689989, -2.280704836619014309E-13, 54.46834944099972375 ) ) ;
#14631=CARTESIAN_POINT ( 'NONE',  ( 48.46158931187873975, -18.19743074333925748, 35.02055581498667181 ) ) ;
#14633=CARTESIAN_POINT ( 'NONE',  ( -100.7734535825088358, -12.25131212657493052, 12.25131212657478130 ) ) ;
#14634=VERTEX_POINT ( 'NONE', #25198 ) ;
#14635=CARTESIAN_POINT ( 'NONE',  ( -62.79433447046256589, 24.94280497471530111, -11.74096317463568795 ) ) ;
#14636=CARTESIAN_POINT ( 'NONE',  ( 135.5356265174577572, 30.20731421070355083, -12.51227922893884248 ) ) ;
#14637=CARTESIAN_POINT ( 'NONE',  ( 19.06497207195980792, -14.19242893257839988, -40.00000000000002132 ) ) ;
#14639=CARTESIAN_POINT ( 'NONE',  ( -188.2995950289364089, -43.00522595870943832, -23.44932284466036521 ) ) ;
#14641=VERTEX_POINT ( 'NONE', #25701 ) ;
#14642=EDGE_CURVE ( 'NONE', #13720, #12829, #12639, .T. ) ;
#14644=CARTESIAN_POINT ( 'NONE',  ( -88.38011429762325122, 8.298859915237940754, -20.03522015860023942 ) ) ;
#14645=CARTESIAN_POINT ( 'NONE',  ( 20.17262239842997928, 18.14389419514546375, 43.80323544018629178 ) ) ;
#14646=ORIENTED_EDGE ( 'NONE', *, *, #20204, .T. ) ;
#14647=ORIENTED_EDGE ( 'NONE', *, *, #21180, .T. ) ;
#14648=CARTESIAN_POINT ( 'NONE',  ( 57.59792236341147031, -1.722363176415032004, -1.722363176415048880 ) ) ;
#14650=CARTESIAN_POINT ( 'NONE',  ( -105.2054292635174875, -16.16779360711802127, -14.22820282028660799 ) ) ;
#14651=CARTESIAN_POINT ( 'NONE',  ( -208.1127848780264742, -17.67593391476659548, 38.89260858015730804 ) ) ;
#14653=CARTESIAN_POINT ( 'NONE',  ( -102.2610585947573298, 5.898343112255980222E-14, -22.27377874548543701 ) ) ;
#14655=CARTESIAN_POINT ( 'NONE',  ( -213.1075012329537230, 5.259461644596141978E-13, -53.71589010951915100 ) ) ;
#14657=CARTESIAN_POINT ( 'NONE',  ( 91.82158438592158234, -1.633484621919921769E-13, 17.20528682183300262 ) ) ;
#14658=CARTESIAN_POINT ( 'NONE',  ( -4.039451493210496125, 23.44932283416649454, 43.00522595894017286 ) ) ;
#14661=CARTESIAN_POINT ( 'NONE',  ( -189.6939181379233901, 18.01964634722543579, 43.50327460064161755 ) ) ;
#14662=CARTESIAN_POINT ( 'NONE',  ( 184.8905102610680444, 14.79361573936375507, 14.79361573936398067 ) ) ;
#14663=ADVANCED_FACE ( 'NONE', ( #23443 ), #21351, .T. ) ;
#14665=B_SPLINE_CURVE_WITH_KNOTS ( 'NONE', 3,
 ( #11696, #15558, #19821, #24081, #13565, #25826 ),
 .UNSPECIFIED., .F., .F.,
 ( 4, 2, 4 ),
 ( 0.3689590070116581244, 0.3867117631979620773, 0.4044645193949217843 ),
 .UNSPECIFIED. ) ;
#14666=CARTESIAN_POINT ( 'NONE',  ( 199.9999999999999432, -14.14213562373093680, 14.14213562373082311 ) ) ;
#14667=DIRECTION ( 'NONE',  ( 0.000000000000000000, 0.3656393565213325592, 0.9307566067252307507 ) ) ;
#14669=CIRCLE ( 'NONE', #12991, 15.00000000000000178 ) ;
#14670=CARTESIAN_POINT ( 'NONE',  ( 200.0000000000000000, 14.14213562373142352, -42.42640687119268961 ) ) ;
#14671=CARTESIAN_POINT ( 'NONE',  ( -199.9999999999998579, 44.86878812508723513, -24.82633483071237634 ) ) ;
#14672=CARTESIAN_POINT ( 'NONE',  ( 0.2972598230769983307, -14.33493731733933352, 0.000000000000000000 ) ) ;
#14673=ADVANCED_FACE ( 'NONE', ( #1196 ), #6038, .T. ) ;
#14674=CARTESIAN_POINT ( 'NONE',  ( 91.82158438592158234, 16.11829626348378142, 40.45024623143977749 ) ) ;
#14675=CARTESIAN_POINT ( 'NONE',  ( 57.59792236341147031, 2.435789363418171760, 0.000000000000000000 ) ) ;
#14677=B_SPLINE_CURVE_WITH_KNOTS ( 'NONE', 3,
 ( #17038, #4419, #559, #18640, #8664, #22775 ),
 .UNSPECIFIED., .F., .F.,
 ( 4, 2, 4 ),
 ( 0.000000000000000000, 0.004089908668607722744, 0.008179817337215445489 ),
 .UNSPECIFIED. ) ;
#14678=CARTESIAN_POINT ( 'NONE',  ( 136.1360204305621551, -39.99999999999994316, -4.966164525587488221 ) ) ;
#14683=EDGE_LOOP ( 'NONE', ( #2037, #7850, #7681, #1958 ) ) ;
#14684=ORIENTED_EDGE ( 'NONE', *, *, #10872, .T. ) ;
#14685=ORIENTED_EDGE ( 'NONE', *, *, #6062, .T. ) ;
#14686=CARTESIAN_POINT ( 'NONE',  ( -208.1127848780264742, 55.00245453014418473, 40.00000000000002132 ) ) ;
#14687=CARTESIAN_POINT ( 'NONE',  ( 147.2817042152898921, 12.35516179550106131, 29.82799917201331752 ) ) ;
#14690=CARTESIAN_POINT ( 'NONE',  ( -208.1127848780265026, 38.89260858015777700, -38.89260858015687461 ) ) ;
#14691=CARTESIAN_POINT ( 'NONE',  ( -110.1003821002955476, -20.16525298256173926, 1.261039542895599830 ) ) ;
#14692=PLANE ( 'NONE',  #20219 ) ;
#14693=DIRECTION ( 'NONE',  ( -0.7071067811865499042, -0.7071067811865451302, 0.000000000000000000 ) ) ;
#14697=CARTESIAN_POINT ( 'NONE',  ( 163.1118516004056573, -47.56205970284945295, -9.006482792074823607 ) ) ;
#14698=CARTESIAN_POINT ( 'NONE',  ( 151.7948205124835681, -4.785054706298876859, 51.78348778862533663 ) ) ;
#14699=CARTESIAN_POINT ( 'NONE',  ( -114.4364955367327212, -20.04994829327665684, -8.644468109209087814 ) ) ;
#14700=CARTESIAN_POINT ( 'NONE',  ( 57.59792236341146321, 40.00000000000000711, 2.435789363418579434 ) ) ;
#14702=CARTESIAN_POINT ( 'NONE',  ( -83.21262154144250189, 33.12752917118434226, -13.72187187061452107 ) ) ;
#14703=CARTESIAN_POINT ( 'NONE',  ( -280.0000000000000000, 19.99999999999996092, -0.000000000000000000 ) ) ;
#14704=CARTESIAN_POINT ( 'NONE',  ( 0.2972598230769938343, 10.13633138497472252, 10.13633138497475628 ) ) ;
#14705=CARTESIAN_POINT ( 'NONE',  ( 0.2972598230770153171, -66.70487387989861361, 10.13633138497438324 ) ) ;
#14708=CARTESIAN_POINT ( 'NONE',  ( -105.3755690713226585, 39.99999999999993605, 18.24025645688366737 ) ) ;
#14710=CARTESIAN_POINT ( 'NONE',  ( 23.58679727197014842, 42.79169916605225410, -23.29637218065878201 ) ) ;
#14711=CARTESIAN_POINT ( 'NONE',  ( -208.1127848780265026, 15.00245453012665564, 0.000000000000000000 ) ) ;
#14712=CARTESIAN_POINT ( 'NONE',  ( -162.0762913951021176, 1.198031840315997298, 57.76657433523996588 ) ) ;
#14713=CARTESIAN_POINT ( 'NONE',  ( 57.59792236341147031, -2.435789363418150000, 40.00000000000002132 ) ) ;
#14714=CARTESIAN_POINT ( 'NONE',  ( -47.65341557551062834, -31.50022537346376694, 10.55973086694773855 ) ) ;
#14715=CARTESIAN_POINT ( 'NONE',  ( 170.2234770963711128, -24.55285855007184281, 40.00000000000002132 ) ) ;
#14716=EDGE_LOOP ( 'NONE', ( #2978, #24983, #17419, #957 ) ) ;
#14718=CARTESIAN_POINT ( 'NONE',  ( -192.9588430854690273, -18.05360324515454096, 38.51493924976936967 ) ) ;
#14719=CARTESIAN_POINT ( 'NONE',  ( -4.421177063212223146, -13.80119274858222944, 46.85829989839683662 ) ) ;
#14720=CARTESIAN_POINT ( 'NONE',  ( -5.379830816902851254, 23.18791234549835423, -42.60994460517710536 ) ) ;
#14722=CARTESIAN_POINT ( 'NONE',  ( 170.2234770963711128, -17.36149277827010096, 17.36149277826970660 ) ) ;
#14724=CARTESIAN_POINT ( 'NONE',  ( -87.02142894580205734, 5.408203463865087102, 20.76642173393088342 ) ) ;
#14725=CARTESIAN_POINT ( 'NONE',  ( -188.9266751785327756, -17.94050871568869354, 43.31221945728800193 ) ) ;
#14726=CARTESIAN_POINT ( 'NONE',  ( -198.0356074513804572, -10.87444709759714634, -10.87444709759729911 ) ) ;
#14727=CARTESIAN_POINT ( 'NONE',  ( 151.7948205124836534, -51.78348778862529400, -4.785054706299085581 ) ) ;
#14728=DIRECTION ( 'NONE',  ( 0.000000000000000000, 1.000000000000000000, 0.000000000000000000 ) ) ;
#14729=CARTESIAN_POINT ( 'NONE',  ( 136.1360204305621266, 24.77266263493104148, 24.77266263493145004 ) ) ;
#14730=CARTESIAN_POINT ( 'NONE',  ( 91.82158438592158234, 16.11829626346161604, -16.11829626346121103 ) ) ;
#14731=CARTESIAN_POINT ( 'NONE',  ( 184.8905102610680444, 13.49065550809757497, 43.07788698682593065 ) ) ;
#14732=CARTESIAN_POINT ( 'NONE',  ( -208.1127848780264742, -55.00245453012676222, -2.449293598294708485E-15 ) ) ;
#14733=CARTESIAN_POINT ( 'NONE',  ( 0.2972598230769930572, 54.33493731733936016, 2.449293598294708485E-15 ) ) ;
#14734=CARTESIAN_POINT ( 'NONE',  ( 151.7948205124836534, -40.00000000000034817, 33.23291073765511072 ) ) ;
#14735=CARTESIAN_POINT ( 'NONE',  ( 4.995406935893287326, 67.35176059882533650, 10.78321810390163549 ) ) ;
#14737=CARTESIAN_POINT ( 'NONE',  ( -100.0968563617409330, 20.72609133245494917, -8.149320301549584755 ) ) ;
#14738=CARTESIAN_POINT ( 'NONE',  ( 19.06497207195982568, -38.31983398719592770, -38.31983398719660272 ) ) ;
#14739=CARTESIAN_POINT ( 'NONE',  ( -30.26275506840324070, -1.198031551616032919, 1.198031551616014712 ) ) ;
#14741=CARTESIAN_POINT ( 'NONE',  ( -259.2033419157646676, 49.83842185052027673, -6.730120644403441155 ) ) ;
#14742=CARTESIAN_POINT ( 'NONE',  ( -190.6721700386038378, -13.94344193548887567, -47.76494742512097247 ) ) ;
#14743=ADVANCED_FACE ( 'NONE', ( #20141 ), #24938, .T. ) ;
#14744=CARTESIAN_POINT ( 'NONE',  ( -30.26275506840323359, -1.198031551616339341, 57.76657404653985139 ) ) ;
#14745=CARTESIAN_POINT ( 'NONE',  ( -3.696864809816581943, -43.10456217110744603, -23.52297716615256817 ) ) ;
#14750=CARTESIAN_POINT ( 'NONE',  ( 19.06497207195980792, 54.19242893257844429, 40.00000000000002132 ) ) ;
#14753=EDGE_CURVE ( 'NONE', #15843, #61, #5654, .T. ) ;
#14754=CARTESIAN_POINT ( 'NONE',  ( 200.0000000000000000, -42.42640687119290988, 14.14213562373064903 ) ) ;
#14755=CARTESIAN_POINT ( 'NONE',  ( 4.995406935893305089, -40.00000000000021316, 55.24977328853194791 ) ) ;
#14756=CARTESIAN_POINT ( 'NONE',  ( 4.995406935893283773, 39.99999999999997158, 15.24977328854846803 ) ) ;
#14757=CARTESIAN_POINT ( 'NONE',  ( -3.071327051952984721, 47.32824404903822568, -13.87830843099591505 ) ) ;
#14758=CARTESIAN_POINT ( 'NONE',  ( 57.59792236341147031, 2.435789363418170872, -40.00000000000002132 ) ) ;
#14760=CARTESIAN_POINT ( 'NONE',  ( -238.4067589809705510, -40.96449427998265946, -2.449293598294708485E-15 ) ) ;
#14762=CARTESIAN_POINT ( 'NONE',  ( -135.8532207217289738, -21.81201906317788186, 21.81201906317762962 ) ) ;
#14763=CARTESIAN_POINT ( 'NONE',  ( 151.0853911467767432, -12.04115959307973505, -29.06993079631223154 ) ) ;
#14764=CARTESIAN_POINT ( 'NONE',  ( -110.0368417077420418, 18.51665893310598676, -7.992411109433959382 ) ) ;
#14765=CARTESIAN_POINT ( 'NONE',  ( -105.3755690713226585, 40.00000000000019185, -18.24025645688310249 ) ) ;
#14766=CARTESIAN_POINT ( 'NONE',  ( -100.7734535825088500, 39.99999999999994316, 17.32597176626825686 ) ) ;
#14767=CARTESIAN_POINT ( 'NONE',  ( -192.9588430854689989, 10.23066800230742679, 10.23066800230749607 ) ) ;
#14768=DIRECTION ( 'NONE',  ( 0.9698969544100306539, 0.2249791742633133473, -0.09318942522595978495 ) ) ;
#14769=CARTESIAN_POINT ( 'NONE',  ( -114.6318783467470723, -11.20407312246388720, 18.94416332742964926 ) ) ;
#14770=CARTESIAN_POINT ( 'NONE',  ( 19.06497207195982568, -38.31983398719646061, 38.31983398719606271 ) ) ;
#14772=CARTESIAN_POINT ( 'NONE',  ( 163.1118516004056573, 19.27778845538753316, 19.27778845538783870 ) ) ;
#14773=CARTESIAN_POINT ( 'NONE',  ( 199.9999999999999432, -14.14213562373115884, 14.14213562373085153 ) ) ;
#14774=CARTESIAN_POINT ( 'NONE',  ( 147.2817042152898637, 29.82799917201328554, -12.35516179550128157 ) ) ;
#14775=CARTESIAN_POINT ( 'NONE',  ( -280.0000000000000568, -20.00000000000006395, -40.00000000000002132 ) ) ;
#14776=EDGE_CURVE ( 'NONE', #8230, #24877, #18678, .T. ) ;
#14777=CARTESIAN_POINT ( 'NONE',  ( -86.91014751117381820, -7.317915707774015566, -20.05881702300846925 ) ) ;
#14778=CARTESIAN_POINT ( 'NONE',  ( 14.38125909742180752, 10.73282306404735387, -10.73282306404708919 ) ) ;
#14779=EDGE_LOOP ( 'NONE', ( #22111, #20788, #22258, #11343, #5743, #19458, #20685 ) ) ;
#14783=CARTESIAN_POINT ( 'NONE',  ( 22.77497178454752458, 17.88345994150152762, 43.17449153292939457 ) ) ;
#14784=ORIENTED_EDGE ( 'NONE', *, *, #13149, .F. ) ;
#14786=CARTESIAN_POINT ( 'NONE',  ( -100.7734535825088500, -16.03295912088716335, 40.53558337403673306 ) ) ;
#14788=CARTESIAN_POINT ( 'NONE',  ( -105.2109270642729939, 1.359352815179485363, 21.45728911408426498 ) ) ;
#14789=CARTESIAN_POINT ( 'NONE',  ( 19.06497207195981858, 10.03556273973424062, 66.60410523465820631 ) ) ;
#14790=CARTESIAN_POINT ( 'NONE',  ( -105.4741150117382915, -19.60045294982753461, 8.366608964593266862 ) ) ;
#14791=CARTESIAN_POINT ( 'NONE',  ( 192.4448373802101173, 39.99999999999998579, 19.99999999996075317 ) ) ;
#14794=CARTESIAN_POINT ( 'NONE',  ( -259.2033419157646676, 40.00000000000029843, -30.48217210827696988 ) ) ;
#14795=CARTESIAN_POINT ( 'NONE',  ( -100.7734535825088358, -2.560096224687585342E-13, 22.67402823373191723 ) ) ;
#14797=CARTESIAN_POINT ( 'NONE',  ( -86.95492379317086318, -19.11844895728714988, -9.645497522856738115 ) ) ;
#14799=CARTESIAN_POINT ( 'NONE',  ( -188.2870673237561050, 13.82722856953796864, 46.98612534495544679 ) ) ;
#14800=CARTESIAN_POINT ( 'NONE',  ( -56.48582580120559982, -21.81201906317804173, 34.75652343174591152 ) ) ;
#14801=CARTESIAN_POINT ( 'NONE',  ( -196.0240758340697198, -48.96019759410239658, 14.12332442061111237 ) ) ;
#14802=CARTESIAN_POINT ( 'NONE',  ( 19.06497207195982568, -38.31983398719646061, 38.31983398719606271 ) ) ;
#14804=CARTESIAN_POINT ( 'NONE',  ( -100.7734535825088358, -12.25131212657475643, -12.25131212657495539 ) ) ;
#14806=CARTESIAN_POINT ( 'NONE',  ( -83.21262154144250189, -33.12752917118400831, 13.72187187061544122 ) ) ;
#14807=CARTESIAN_POINT ( 'NONE',  ( 57.59792236341147031, 26.56190807104652052, 30.00663442387728708 ) ) ;
#14808=CARTESIAN_POINT ( 'NONE',  ( 192.4448373802101173, 20.00000000003945644, 40.00000000000002132 ) ) ;
#14810=EDGE_LOOP ( 'NONE', ( #25077, #24549, #21812, #23929 ) ) ;
#14811=CARTESIAN_POINT ( 'NONE',  ( -91.56559293963834989, -40.00000000000027711, 22.67402823373149801 ) ) ;
#14813=CARTESIAN_POINT ( 'NONE',  ( 164.1122551457365546, -10.10009781492445491, 24.38379312608483573 ) ) ;
#14814=ORIENTED_EDGE ( 'NONE', *, *, #5708, .T. ) ;
#14816=CARTESIAN_POINT ( 'NONE',  ( 163.1118516004056573, 12.73709011382477918, 40.00000000000002132 ) ) ;
#14818=EDGE_CURVE ( 'NONE', #18174, #8800, #13063, .T. ) ;
#14819=CARTESIAN_POINT ( 'NONE',  ( -114.6821015619773902, -21.58745106897183419, -4.467609313250024528 ) ) ;
#14820=EDGE_CURVE ( 'NONE', #19333, #25051, #9808, .T. ) ;
#14821=CARTESIAN_POINT ( 'NONE',  ( -200.0000000000000000, 55.16984130227019989, -4.865628651907604407 ) ) ;
#14822=CARTESIAN_POINT ( 'NONE',  ( 14.38125909742181818, -40.00000000000007816, 15.17850393972619649 ) ) ;
#14825=CARTESIAN_POINT ( 'NONE',  ( -105.2054292635175727, 7.329160573984922335E-13, -21.49321519473985020 ) ) ;
#14826=CARTESIAN_POINT ( 'NONE',  ( -259.2033419157646676, -6.730120644403663199, 6.730120644403451813 ) ) ;
#14827=CARTESIAN_POINT ( 'NONE',  ( -213.1075012329537230, -9.698598906450422774, -9.698598906450550672 ) ) ;
#14828=CARTESIAN_POINT ( 'NONE',  ( -77.90255099906863734, -20.04994828524331396, -8.644468104250957907 ) ) ;
#14829=CARTESIAN_POINT ( 'NONE',  ( 170.2234770963711128, -2.259079968736224833E-13, 24.55285855007187124 ) ) ;
#14830=CARTESIAN_POINT ( 'NONE',  ( -100.0753760173601989, -8.149786832859113872, 20.72827493166387924 ) ) ;
#14831=CARTESIAN_POINT ( 'NONE',  ( 23.37394308801976450, 13.80096434448266685, 46.80823611210199431 ) ) ;
#14832=CARTESIAN_POINT ( 'NONE',  ( -213.1075012329537230, 37.98287015391228749, 37.98287015391245802 ) ) ;
#14833=CARTESIAN_POINT ( 'NONE',  ( 151.7948205124836534, -33.06932595376343897, -23.49921654116042902 ) ) ;
#14836=CARTESIAN_POINT ( 'NONE',  ( 57.59792236341147031, 1.908507979671054758E-14, -2.435789363418160658 ) ) ;
#14837=CARTESIAN_POINT ( 'NONE',  ( 60.14720761588395703, 33.22245024480380238, -10.94158980388390923 ) ) ;
#14838=CARTESIAN_POINT ( 'NONE',  ( 0.2972598230769930017, 14.33493731733933352, -40.00000000000002132 ) ) ;
#14839=CARTESIAN_POINT ( 'NONE',  ( -30.26275506840324070, -27.08623969584595770, 29.48230279907789608 ) ) ;
#14840=CARTESIAN_POINT ( 'NONE',  ( 170.2234770963711128, -24.55285855007184281, 40.00000000000002132 ) ) ;
#14842=VERTEX_POINT ( 'NONE', #21032 ) ;
#14843=CARTESIAN_POINT ( 'NONE',  ( -2.557884977116120506, -47.52441970262191262, 13.90734923102589704 ) ) ;
#14844=CARTESIAN_POINT ( 'NONE',  ( 19.06497207195980792, 14.19242893257840699, 40.00000000000002132 ) ) ;
#14847=FACE_OUTER_BOUND ( 'NONE', #2866, .T. ) ;
#14848=CARTESIAN_POINT ( 'NONE',  ( -3.838270362644687239, -17.89317813950069436, 43.19795333834606765 ) ) ;
#14849=CARTESIAN_POINT ( 'NONE',  ( -238.4067589809705794, 28.96627169325324758, -27.60227080167054581 ) ) ;
#14850=CARTESIAN_POINT ( 'NONE',  ( -3.921555385249997805, 23.47492146734898810, -43.03974577853578154 ) ) ;
#14852=CARTESIAN_POINT ( 'NONE',  ( 0.2972598230769938343, 10.13633138497486286, -10.13633138497461594 ) ) ;
#14854=CARTESIAN_POINT ( 'NONE',  ( -77.90255099906769942, -20.29001641120677846, -8.064892378658084837 ) ) ;
#14856=CARTESIAN_POINT ( 'NONE',  ( -188.3392995398617700, -13.83024151208848807, 47.00482667599631270 ) ) ;
#14857=CARTESIAN_POINT ( 'NONE',  ( -91.56559293963836410, 16.03295912088692177, 16.03295912088721664 ) ) ;
#14858=CIRCLE ( 'NONE', #19121, 14.99999999999999822 ) ;
#14859=CARTESIAN_POINT ( 'NONE',  ( 4.995406935893301537, -10.78321810390187530, 67.35176059882529387 ) ) ;
#14860=CARTESIAN_POINT ( 'NONE',  ( -30.26275506840324070, 1.198031551616030033, -1.198031551616006496 ) ) ;
#14861=CARTESIAN_POINT ( 'NONE',  ( -213.1075012329537230, 18.58567234101174037, -37.98287015391222354 ) ) ;
#14862=CARTESIAN_POINT ( 'NONE',  ( 14.38125909742181285, -10.73282306404712472, -10.73282306404731301 ) ) ;
#14863=CARTESIAN_POINT ( 'NONE',  ( -105.3755690713226585, 41.18208027870575449, 15.38646221621837107 ) ) ;
#14864=CARTESIAN_POINT ( 'NONE',  ( 151.7948205124836250, -23.49921654116371883, 23.49921654116317526 ) ) ;
#14865=CARTESIAN_POINT ( 'NONE',  ( 151.7948205124835681, 33.23291073765556547, 40.00000000000002132 ) ) ;
#14866=CARTESIAN_POINT ( 'NONE',  ( 136.1360204305621551, 4.966164525587093870, -40.00000000000002132 ) ) ;
#14867=CARTESIAN_POINT ( 'NONE',  ( 4.995406935893283773, 39.06748935135195211, -17.50105314357185193 ) ) ;
#14869=CARTESIAN_POINT ( 'NONE',  ( -198.0356074513804288, -39.15871834505882276, -39.15871834505946936 ) ) ;
#14870=CARTESIAN_POINT ( 'NONE',  ( -184.9729924864769259, 45.83719276903030959, -13.59277144553964689 ) ) ;
#14872=CARTESIAN_POINT ( 'NONE',  ( -91.56559293963834989, -16.03295912088716335, 40.53558337403673306 ) ) ;
#14873=CARTESIAN_POINT ( 'NONE',  ( -82.23726319249649919, -14.28014421912411080, -14.28014421912425114 ) ) ;
#14874=CARTESIAN_POINT ( 'NONE',  ( -208.1127848780264742, -38.89260858015758515, 38.89260858015713751 ) ) ;
#14875=CARTESIAN_POINT ( 'NONE',  ( -4.031723327955770486, -43.00750292060831725, -23.45082932595563818 ) ) ;
#14876=ORIENTED_EDGE ( 'NONE', *, *, #14186, .F. ) ;
#14878=CARTESIAN_POINT ( 'NONE',  ( -105.2054292635175869, -15.19799821370180126, -15.19799821370278892 ) ) ;
#14881=CARTESIAN_POINT ( 'NONE',  ( 7.307793755307390171, 14.18010697691907929, -49.33439594495632008 ) ) ;
#14882=CARTESIAN_POINT ( 'NONE',  ( 170.2234770963711128, 15.44714144992818738, 40.00000000000002132 ) ) ;
#14885=CARTESIAN_POINT ( 'NONE',  ( 146.6084372240433709, -3.800685668859084210, 52.76785682606516303 ) ) ;
#14886=CARTESIAN_POINT ( 'NONE',  ( 200.0000000000000000, -40.00000000000005684, 19.99999999999978328 ) ) ;
#14887=CARTESIAN_POINT ( 'NONE',  ( -162.0762913951020892, 39.99999999999985079, 41.69427287692695216 ) ) ;
#14888=CARTESIAN_POINT ( 'NONE',  ( -198.0012279766649783, -24.77357825137635317, -44.79720171007490848 ) ) ;
#14889=CARTESIAN_POINT ( 'NONE',  ( -192.9588430854690273, -54.46834944101725284, -40.00000000000002132 ) ) ;
#14890=CARTESIAN_POINT ( 'NONE',  ( 22.77497178454834881, -17.88345994150125051, -43.17449153292930220 ) ) ;
#14891=CARTESIAN_POINT ( 'NONE',  ( 0.2972598230769976091, -10.13633138497479180, 10.13633138497468522 ) ) ;
#14892=CARTESIAN_POINT ( 'NONE',  ( 170.2234770963711128, -15.44714144992812876, -2.449293598294708485E-15 ) ) ;
#14893=CARTESIAN_POINT ( 'NONE',  ( 151.7948205124835681, 51.78348778862537927, 4.785054706298732086 ) ) ;
#14894=CARTESIAN_POINT ( 'NONE',  ( 155.4809970915716804, -11.45899766888342164, -27.66446758342039658 ) ) ;
#14895=CARTESIAN_POINT ( 'NONE',  ( -114.6297772182939951, 11.19545617573264451, -18.93772329698290235 ) ) ;
#14896=CARTESIAN_POINT ( 'NONE',  ( 146.6084372240433709, 40.00000000000010658, -5.374981219216549810 ) ) ;
#14897=CARTESIAN_POINT ( 'NONE',  ( -30.26275506840324070, 1.198031551616013601, 1.198031551616023371 ) ) ;
#14900=CARTESIAN_POINT ( 'NONE',  ( -105.3755690713226727, -12.89780903124413847, 12.89780903124398037 ) ) ;
#14901=ORIENTED_EDGE ( 'NONE', *, *, #7653, .F. ) ;
#14903=CARTESIAN_POINT ( 'NONE',  ( -47.65341557548335061, 31.50022537338118767, -10.55973086711139786 ) ) ;
#14905=CARTESIAN_POINT ( 'NONE',  ( -100.7734535825088358, -17.32597176626813251, -2.449293598294708485E-15 ) ) ;
#14906=CARTESIAN_POINT ( 'NONE',  ( -163.5815475691942709, -35.61501186087241422, 18.59457173339187364 ) ) ;
#14909=VERTEX_POINT ( 'NONE', #23038 ) ;
#14912=VERTEX_POINT ( 'NONE', #18901 ) ;
#14914=PRODUCT_DEFINITION ( 'UNKNOWN', '', #7447, #23345 ) ;
#14915=CARTESIAN_POINT ( 'NONE',  ( -238.4067589809705794, -27.60227080167069147, 28.96627169325319429 ) ) ;
#14918=CARTESIAN_POINT ( 'NONE',  ( -105.3174603216987890, -18.50736914802315880, -10.86220755232618096 ) ) ;
#14919=CARTESIAN_POINT ( 'NONE',  ( -238.4067589809705794, -27.60227080167069147, 28.96627169325319429 ) ) ;
#14922=CARTESIAN_POINT ( 'NONE',  ( -91.56559293963836410, 39.99999999999994316, 17.32597176626825330 ) ) ;
#14926=CARTESIAN_POINT ( 'NONE',  ( -88.37877758185183552, -8.026456973205808865, -20.15391234962195810 ) ) ;
#14927=EDGE_CURVE ( 'NONE', #12388, #7311, #9219, .T. ) ;
#14928=CARTESIAN_POINT ( 'NONE',  ( 91.82158438592159655, -40.00000000000017764, 17.20528682183258340 ) ) ;
#14929=CARTESIAN_POINT ( 'NONE',  ( 0.2972598230769883387, 40.00000000000017053, -14.33493731733891607 ) ) ;
#14933=CARTESIAN_POINT ( 'NONE',  ( -188.4701769959665967, 13.83721050406949793, 47.05181236278358625 ) ) ;
#14934=B_SPLINE_CURVE_WITH_KNOTS ( 'NONE', 3,
 ( #18256, #14404, #2435, #10284, #8276, #16401 ),
 .UNSPECIFIED., .F., .F.,
 ( 4, 2, 4 ),
 ( -6.000000002263262234E-08, 0.03937727647057992497, 0.07875461294115987387 ),
 .UNSPECIFIED. ) ;
#14935=CARTESIAN_POINT ( 'NONE',  ( -105.3755690713226727, 15.38646221621771737, 15.38646221621800514 ) ) ;
#14937=CARTESIAN_POINT ( 'NONE',  ( -105.3755690713226585, 43.67073346367970288, 12.89780903124427702 ) ) ;
#14938=CARTESIAN_POINT ( 'NONE',  ( -77.90255099906768521, -20.04994828523974348, 8.644468104261179064 ) ) ;
#14940=CARTESIAN_POINT ( 'NONE',  ( -259.2033419157646676, 6.730120644403918995, -49.83842185052024831 ) ) ;
#14942=CARTESIAN_POINT ( 'NONE',  ( -199.9999999999997726, -24.82633483071077762, 44.86878812508861358 ) ) ;
#14943=CARTESIAN_POINT ( 'NONE',  ( 151.7948205124836250, -23.49921654116371883, 23.49921654116317526 ) ) ;
#14944=B_SPLINE_CURVE_WITH_KNOTS ( 'NONE', 3,
 ( #25012, #20610, #6765, #12894, #24744, #16346, #22482, #2661, #22615, #24478, #4261, #10766 ),
 .UNSPECIFIED., .F., .F.,
 ( 4, 2, 2, 2, 2, 4 ),
 ( 2.733202585622216256E-15, 0.004698945756009177514, 0.007048418634012399743, 0.009397891512015622839, 0.01409683726802202566, 0.01879578302402842849 ),
 .UNSPECIFIED. ) ;
#14945=CARTESIAN_POINT ( 'NONE',  ( 163.1118516004056573, -12.73709011382472589, 40.00000000000002132 ) ) ;
#14947=ORIENTED_EDGE ( 'NONE', *, *, #23589, .T. ) ;
#14948=CARTESIAN_POINT ( 'NONE',  ( 151.7948205124836250, 1.012150473917908975E-13, -6.767089262349031742 ) ) ;
#14949=CARTESIAN_POINT ( 'NONE',  ( 199.9999999999999432, -14.14213562373096345, -14.14213562373104871 ) ) ;
#14950=CARTESIAN_POINT ( 'NONE',  ( 104.1600437297060608, -8.548029201781588426, 20.63676802900535634 ) ) ;
#14954=CARTESIAN_POINT ( 'NONE',  ( 170.2234770963711128, 15.44714144992818738, 40.00000000000002132 ) ) ;
#14955=CARTESIAN_POINT ( 'NONE',  ( 170.0000000000000000, 30.00000000000007105, 0.000000000000000000 ) ) ;
#14957=B_SPLINE_CURVE_WITH_KNOTS ( 'NONE', 3,
 ( #25023, #2399, #13038, #6776, #14888, #18758 ),
 .UNSPECIFIED., .F., .F.,
 ( 4, 2, 4 ),
 ( -5.998616620282925083E-08, 0.005995031700373402127, 0.01199012338691300694 ),
 .UNSPECIFIED. ) ;
#14958=CARTESIAN_POINT ( 'NONE',  ( -114.6659165474202524, -21.50057250525921759, -4.804252803513915815 ) ) ;
#14959=CARTESIAN_POINT ( 'NONE',  ( -200.0000000000000000, 53.44529986889376261, -10.02640517461949088 ) ) ;
#14960=CARTESIAN_POINT ( 'NONE',  ( 0.2972598230769957217, -4.999556039334937811E-14, 14.33493731733933352 ) ) ;
#14963=CARTESIAN_POINT ( 'NONE',  ( -208.1127848780264742, 10.60833733268383483, -67.17687982760675425 ) ) ;
#14964=CARTESIAN_POINT ( 'NONE',  ( -213.1075012329537230, -9.698598906450422774, -9.698598906450550672 ) ) ;
#14965=CARTESIAN_POINT ( 'NONE',  ( -102.4332189563017153, 20.29361511516604466, 8.405890610281785413 ) ) ;
#14966=CARTESIAN_POINT ( 'NONE',  ( 192.4448373802101173, 40.00000000000026290, -19.99999999996018474 ) ) ;
#14967=CARTESIAN_POINT ( 'NONE',  ( 4.995406935893293543, -10.78321810388990265, -10.78321810389009272 ) ) ;
#14968=CARTESIAN_POINT ( 'NONE',  ( -3.486753633152349874, 13.85715877881432334, 47.18604396268653289 ) ) ;
#14969=CARTESIAN_POINT ( 'NONE',  ( -91.56559293963834989, -12.25131212657492874, 12.25131212657477953 ) ) ;
#14972=CARTESIAN_POINT ( 'NONE',  ( -56.48582580120559271, 2.158176344243877536E-14, -9.153146818113587102 ) ) ;
#14975=CARTESIAN_POINT ( 'NONE',  ( 4.995406935893294431, -17.50105314357198694, 39.06748935135188816 ) ) ;
#14976=CARTESIAN_POINT ( 'NONE',  ( -105.3755690713226585, -21.75974354311652448, 40.00000000000002132 ) ) ;
#14977=EDGE_LOOP ( 'NONE', ( #24317, #16487, #2197, #9862 ) ) ;
#14978=CARTESIAN_POINT ( 'NONE',  ( 6.762329110759959683, -44.82519229649959414, 18.56720258519549915 ) ) ;
#14979=CARTESIAN_POINT ( 'NONE',  ( -91.56559293963834989, -22.67402823373193499, -40.00000000000002132 ) ) ;
#14980=CARTESIAN_POINT ( 'NONE',  ( -105.3841681040940443, 19.11869201643232330, -9.644852623852500528 ) ) ;
#14981=CARTESIAN_POINT ( 'NONE',  ( 146.6084372240433709, -24.48358557860329299, 32.08495691632052882 ) ) ;
#14982=CARTESIAN_POINT ( 'NONE',  ( -7.297127544299105928, -22.81351773423399010, 42.04314499754483592 ) ) ;
#14983=CARTESIAN_POINT ( 'NONE',  ( -87.00234866557609337, 20.64508794607625930, -5.655436908802629503 ) ) ;
#14984=CARTESIAN_POINT ( 'NONE',  ( -39.81953879993383794, 11.17638696932933584, -34.34246706536494287 ) ) ;
#14986=CARTESIAN_POINT ( 'NONE',  ( 163.1118516004056573, -19.27778845538787422, 19.27778845538743724 ) ) ;
#14989=CARTESIAN_POINT ( 'NONE',  ( -192.1964066538514544, -24.16259023442852083, 43.96877160662082673 ) ) ;
#14990=CARTESIAN_POINT ( 'NONE',  ( -192.9588430854690273, 18.05360324515473280, -38.51493924976924177 ) ) ;
#14991=CARTESIAN_POINT ( 'NONE',  ( -162.0762913951021176, 27.08623940707598265, 29.48230308784781428 ) ) ;
#14992=CARTESIAN_POINT ( 'NONE',  ( 184.8905102610680444, -43.07788698682556827, -13.49065550809859104 ) ) ;
#14993=CARTESIAN_POINT ( 'NONE',  ( -86.96347745069645896, 43.67073346367988762, -12.89780903124366418 ) ) ;
#14994=CARTESIAN_POINT ( 'NONE',  ( -86.96347745069645896, 43.67073346367988762, -12.89780903124366418 ) ) ;
#14995=CARTESIAN_POINT ( 'NONE',  ( -30.26275506840323715, 29.48230279907829754, -29.48230279907758344 ) ) ;
#14996=CARTESIAN_POINT ( 'NONE',  ( -213.1075012329537230, 37.98287015391280619, -37.98287015391192512 ) ) ;
#14997=CARTESIAN_POINT ( 'NONE',  ( -192.9588430854689989, 14.46834944099965981, 0.000000000000000000 ) ) ;
#14998=CARTESIAN_POINT ( 'NONE',  ( 57.59792236341147031, -1.722363176415032004, -1.722363176415048880 ) ) ;
#15001=B_SPLINE_CURVE_WITH_KNOTS ( 'NONE', 3,
 ( #3476, #21326, #23692, #21444, #3219, #13324, #1098, #11325, #13082, #19441, #13204, #1228, #5220, #9333, #17442, #25836, #21571, #11574, #19315, #2969, #19568, #3344, #9208, #17564, #25580, #1359, #7580, #9458, #7326, #15440, #5470, #15567, #3098, #25702 ),
 .UNSPECIFIED., .F., .F.,
 ( 4, 2, 2, 2, 2, 2, 2, 2, 2, 2, 2, 2, 2, 2, 2, 2, 4 ),
 ( -5.298243351200284084E-05, 0.01887868273877495867, 0.02834451532491844006, 0.03071097347145433296, 0.03307743161799021892, 0.03544388976452611528, 0.03781034791106200471, 0.04254326420413379051, 0.04727618049720556243, 0.04964263864374145879, 0.05200909679027735516, 0.05674201308334905769, 0.05910847122988491242, 0.06029170030315288142, 0.06147492937642085042, 0.06620784566949271255, 0.07567367825563642292 ),
 .UNSPECIFIED. ) ;
#15002=CARTESIAN_POINT ( 'NONE',  ( 91.82158438592156813, -16.11829626348459144, 40.45024623143943643 ) ) ;
#15004=CARTESIAN_POINT ( 'NONE',  ( -151.4802849339473028, 33.96623543943421453, -11.09498666339088224 ) ) ;
#15005=VERTEX_POINT ( 'NONE', #20906 ) ;
#15006=CARTESIAN_POINT ( 'NONE',  ( 184.8905102610680444, -14.79361573936389540, 41.77492675555996016 ) ) ;
#15007=CARTESIAN_POINT ( 'NONE',  ( -86.86493150571121191, -19.77569912839188149, -7.943527260495856446 ) ) ;
#15008=CARTESIAN_POINT ( 'NONE',  ( -56.48582580120558561, 6.472252184283903809, 50.09629031063968796 ) ) ;
#15014=CARTESIAN_POINT ( 'NONE',  ( -105.2272268089240157, -13.17799186901662445, -17.01573394474107204 ) ) ;
#15017=CARTESIAN_POINT ( 'NONE',  ( -56.48582580120559982, 30.84685318188643421, 40.00000000000002132 ) ) ;
#15018=CARTESIAN_POINT ( 'NONE',  ( 83.11963132829231427, 10.90660717629898180, -23.63628489317784798 ) ) ;
#15020=CARTESIAN_POINT ( 'NONE',  ( -213.1075012329537230, -9.698598906450422774, -9.698598906450550672 ) ) ;
#15021=CARTESIAN_POINT ( 'NONE',  ( -135.8532207217289738, 39.99999999999989342, 30.84685318188660474 ) ) ;
#15022=CARTESIAN_POINT ( 'NONE',  ( -238.4067589809705794, 39.99999999999997158, 0.9644942799827220803 ) ) ;
#15024=CARTESIAN_POINT ( 'NONE',  ( 4.995406935893294431, -15.24977328854832415, -40.00000000000002132 ) ) ;
#15025=CARTESIAN_POINT ( 'NONE',  ( 25.62979979008176556, -13.63460241475589285, -45.99287499156992709 ) ) ;
#15027=CARTESIAN_POINT ( 'NONE',  ( -213.1075012329537230, -13.71589010951915810, 0.000000000000000000 ) ) ;
#15028=CARTESIAN_POINT ( 'NONE',  ( 170.2234770963711128, 45.64576402573181468, 10.92277846919223627 ) ) ;
#15029=CARTESIAN_POINT ( 'NONE',  ( -259.2033419157646676, 39.99999999999987921, 9.517827891723049660 ) ) ;
#15030=CARTESIAN_POINT ( 'NONE',  ( -110.0737093975827321, 17.41451009901375002, -10.28294049092901297 ) ) ;
#15031=CARTESIAN_POINT ( 'NONE',  ( 19.06497207195982924, -39.99999999999945288, -54.19242893257885640 ) ) ;
#15032=CARTESIAN_POINT ( 'NONE',  ( 14.38125909742180752, 10.73282306404720465, 10.73282306404724018 ) ) ;
#15033=CARTESIAN_POINT ( 'NONE',  ( -4.039451493210483690, -43.00522595894025812, 23.44932283416647323 ) ) ;
#15035=CARTESIAN_POINT ( 'NONE',  ( -238.4067589809705794, -0.6820004458488042598, 57.25054294077229855 ) ) ;
#15037=CARTESIAN_POINT ( 'NONE',  ( 136.1360204305621266, 24.77266263493104148, 24.77266263493145004 ) ) ;
#15038=CARTESIAN_POINT ( 'NONE',  ( -5.304449574949627433, 42.80137191221132298, -17.72890873421417623 ) ) ;
#15039=CARTESIAN_POINT ( 'NONE',  ( 155.4809970915716519, 27.66446758342043566, -11.45899766888336124 ) ) ;
#15040=CARTESIAN_POINT ( 'NONE',  ( 170.2234770963711128, -15.44714144992813409, 40.00000000000002132 ) ) ;
#15041=CARTESIAN_POINT ( 'NONE',  ( -114.7469200037858172, 17.46524160228967304, -13.55861222481908612 ) ) ;
#15042=CARTESIAN_POINT ( 'NONE',  ( -194.4222775679850770, 44.35790405182663676, -24.44979664543170372 ) ) ;
#15046=CARTESIAN_POINT ( 'NONE',  ( 98.29820294272414571, 7.653668647302724004, 18.47759065022804137 ) ) ;
#15047=ORIENTED_EDGE ( 'NONE', *, *, #7657, .F. ) ;
#15049=( BOUNDED_SURFACE ( )  B_SPLINE_SURFACE ( 3, 3, ( 
 ( #6329, #7683, #2349, #10462, #23791, #11814, #1717, #354, #23921, #17930, #8458, #24708, #6463, #22707, #19669, #9556, #13678, #9116, #6727, #20714, #22972, #15101, #11119, #6857, #756, #12856, #16845, #5012, #18707, #18843 ),
 ( #490, #8727, #24839, #19104, #1013, #19233, #23236, #16707, #2480, #10592, #12585, #8597, #4750, #8860, #14839, #6590, #14975, #23362, #17227, #20974, #21108, #10732, #7121, #3012, #12715, #25367, #2755, #2887, #621, #24978 ),
 ( #25234, #888, #12986, #13117, #6986, #23109, #10858, #14712, #22844, #15231, #4619, #20843, #8997, #2618, #17101, #18977, #16972, #10995, #25108, #4881, #21238, #19482, #17481, #9767, #5261, #5387, #17868, #11485, #13244, #7621 ),
 ( #17357, #15867, #26018, #3650, #7242, #19740, #21486, #1528, #3137, #1147, #3518, #9251, #17605, #11618, #9372, #25623, #7755, #7369, #9500, #15481, #3260, #23862, #11756, #5139, #25748, #1399, #19613, #13492, #7496, #23608 ),
 ( #25877, #19876, #21613, #5640, #13746, #11239, #25493, #21369, #15607, #15363, #23731, #3387, #21872, #19357, #5512, #13614, #23486, #9634, #21743, #17736, #15736, #1658, #13363, #11364, #1268, #8427, #12161, #3929, #4197, #6174 ),
 ( #26289, #16418, #14020, #16012, #10426, #24279, #12027, #12290, #10303, #3787, #20549, #20283, #18409, #9899, #57, #22421, #14419, #12420, #6301, #20418, #23995, #10168, #5776, #14153, #13883, #4059, #18003, #14284, #22549, #20147 ),
 ( #4330, #184, #1795, #22017, #11890, #20010, #26149, #16146, #2062, #8028, #7893, #18271, #24138, #2318, #6048, #2195, #22149, #18544, #326, #5911, #1925, #10032, #18141, #22285, #8167, #16280, #24408, #8291, #24546, #14949 ) ),
 .UNSPECIFIED., .T., .F., .F. ) 
 B_SPLINE_SURFACE_WITH_KNOTS ( ( 4, 3, 4 ),
 ( 4, 2, 2, 2, 2, 2, 2, 2, 2, 2, 2, 2, 2, 2, 4 ),
 ( 0.000000000000000000, 0.5000000000000000000, 1.000000000000000000 ),
 ( 0.000000000000000000, 0.1357259735107005372, 0.1651108541090157700, 0.1944957347073310028, 0.3598804999793158710, 0.3867117631979620773, 0.4135430264166082281, 0.5789277916885930964, 0.6062785021374117456, 0.6336292125862302838, 0.8508620842112317728, 0.8814014469398914198, 0.9119408096685510667, 0.9559704048342755334, 1.000000000000000000 ),
 .UNSPECIFIED. ) 
 GEOMETRIC_REPRESENTATION_ITEM ( )  RATIONAL_B_SPLINE_SURFACE ( (
 ( 1.000000000000000000, 1.000000000000000000, 1.000000000000000000, 1.000000000000000000, 1.000000000000000000, 1.000000000000000000, 1.000000000000000000, 1.000000000000000000, 1.000000000000000000, 1.000000000000000000, 1.000000000000000000, 1.000000000000000000, 1.000000000000000000, 1.000000000000000000, 1.000000000000000000, 1.000000000000000000, 1.000000000000000000, 1.000000000000000000, 1.000000000000000000, 1.000000000000000000, 1.000000000000000000, 1.000000000000000000, 1.000000000000000000, 1.000000000000000000, 1.000000000000000000, 1.000000000000000000, 1.000000000000000000, 1.000000000000000000, 1.000000000000000000, 1.000000000000000000),
 ( 0.3333333333333333703, 0.3333333333333333703, 0.3333333333333333703, 0.3333333333333333703, 0.3333333333333333703, 0.3333333333333333703, 0.3333333333333333703, 0.3333333333333333703, 0.3333333333333333703, 0.3333333333333333703, 0.3333333333333333703, 0.3333333333333333703, 0.3333333333333333703, 0.3333333333333333703, 0.3333333333333333703, 0.3333333333333333703, 0.3333333333333333703, 0.3333333333333333703, 0.3333333333333333703, 0.3333333333333333703, 0.3333333333333333703, 0.3333333333333333703, 0.3333333333333333703, 0.3333333333333333703, 0.3333333333333333703, 0.3333333333333333703, 0.3333333333333333703, 0.3333333333333333703, 0.3333333333333333703, 0.3333333333333333703),
 ( 0.3333333333333333703, 0.3333333333333333703, 0.3333333333333333703, 0.3333333333333333703, 0.3333333333333333703, 0.3333333333333333703, 0.3333333333333333703, 0.3333333333333333703, 0.3333333333333333703, 0.3333333333333333703, 0.3333333333333333703, 0.3333333333333333703, 0.3333333333333333703, 0.3333333333333333703, 0.3333333333333333703, 0.3333333333333333703, 0.3333333333333333703, 0.3333333333333333703, 0.3333333333333333703, 0.3333333333333333703, 0.3333333333333333703, 0.3333333333333333703, 0.3333333333333333703, 0.3333333333333333703, 0.3333333333333333703, 0.3333333333333333703, 0.3333333333333333703, 0.3333333333333333703, 0.3333333333333333703, 0.3333333333333333703),
 ( 1.000000000000000000, 1.000000000000000000, 1.000000000000000000, 1.000000000000000000, 1.000000000000000000, 1.000000000000000000, 1.000000000000000000, 1.000000000000000000, 1.000000000000000000, 1.000000000000000000, 1.000000000000000000, 1.000000000000000000, 1.000000000000000000, 1.000000000000000000, 1.000000000000000000, 1.000000000000000000, 1.000000000000000000, 1.000000000000000000, 1.000000000000000000, 1.000000000000000000, 1.000000000000000000, 1.000000000000000000, 1.000000000000000000, 1.000000000000000000, 1.000000000000000000, 1.000000000000000000, 1.000000000000000000, 1.000000000000000000, 1.000000000000000000, 1.000000000000000000),
 ( 0.3333333333333333703, 0.3333333333333333703, 0.3333333333333333703, 0.3333333333333333703, 0.3333333333333333703, 0.3333333333333333703, 0.3333333333333333703, 0.3333333333333333703, 0.3333333333333333703, 0.3333333333333333703, 0.3333333333333333703, 0.3333333333333333703, 0.3333333333333333703, 0.3333333333333333703, 0.3333333333333333703, 0.3333333333333333703, 0.3333333333333333703, 0.3333333333333333703, 0.3333333333333333703, 0.3333333333333333703, 0.3333333333333333703, 0.3333333333333333703, 0.3333333333333333703, 0.3333333333333333703, 0.3333333333333333703, 0.3333333333333333703, 0.3333333333333333703, 0.3333333333333333703, 0.3333333333333333703, 0.3333333333333333703),
 ( 0.3333333333333333703, 0.3333333333333333703, 0.3333333333333333703, 0.3333333333333333703, 0.3333333333333333703, 0.3333333333333333703, 0.3333333333333333703, 0.3333333333333333703, 0.3333333333333333703, 0.3333333333333333703, 0.3333333333333333703, 0.3333333333333333703, 0.3333333333333333703, 0.3333333333333333703, 0.3333333333333333703, 0.3333333333333333703, 0.3333333333333333703, 0.3333333333333333703, 0.3333333333333333703, 0.3333333333333333703, 0.3333333333333333703, 0.3333333333333333703, 0.3333333333333333703, 0.3333333333333333703, 0.3333333333333333703, 0.3333333333333333703, 0.3333333333333333703, 0.3333333333333333703, 0.3333333333333333703, 0.3333333333333333703),
 ( 1.000000000000000000, 1.000000000000000000, 1.000000000000000000, 1.000000000000000000, 1.000000000000000000, 1.000000000000000000, 1.000000000000000000, 1.000000000000000000, 1.000000000000000000, 1.000000000000000000, 1.000000000000000000, 1.000000000000000000, 1.000000000000000000, 1.000000000000000000, 1.000000000000000000, 1.000000000000000000, 1.000000000000000000, 1.000000000000000000, 1.000000000000000000, 1.000000000000000000, 1.000000000000000000, 1.000000000000000000, 1.000000000000000000, 1.000000000000000000, 1.000000000000000000, 1.000000000000000000, 1.000000000000000000, 1.000000000000000000, 1.000000000000000000, 1.000000000000000000) ) ) 
 REPRESENTATION_ITEM ( '' )  SURFACE ( )  );
#15050=CARTESIAN_POINT ( 'NONE',  ( 130.8568914410475088, -52.36146031193419503, 4.207082182989537955 ) ) ;
#15052=CARTESIAN_POINT ( 'NONE',  ( -110.1017491837607594, -1.278135197250002353, 20.19444236855598973 ) ) ;
#15053=CARTESIAN_POINT ( 'NONE',  ( -192.9588430854690273, -18.05360324515454096, 38.51493924976936967 ) ) ;
#15054=CARTESIAN_POINT ( 'NONE',  ( 19.06497207195980792, 10.03556273973433299, 10.03556273973436319 ) ) ;
#15055=CARTESIAN_POINT ( 'NONE',  ( 184.8905102610680444, -3.509827109981123710E-14, 19.07866798485558490 ) ) ;
#15056=CARTESIAN_POINT ( 'NONE',  ( -199.9999999999999716, -14.87399974031237093, 48.57705986237296969 ) ) ;
#15057=CARTESIAN_POINT ( 'NONE',  ( -86.86493150571116928, 19.60045294882758071, -8.366608963953975575 ) ) ;
#15058=CARTESIAN_POINT ( 'NONE',  ( -280.0000000000000000, -2.609240458947769655E-13, 20.00000000000001421 ) ) ;
#15059=CARTESIAN_POINT ( 'NONE',  ( -86.96347745069644475, 1.775309070576523494E-13, -18.24025645688352881 ) ) ;
#15060=CARTESIAN_POINT ( 'NONE',  ( -105.4741150117382773, -19.60045294982755593, 8.366608964593277520 ) ) ;
#15063=CARTESIAN_POINT ( 'NONE',  ( -197.4154352059659630, 24.72550168627608258, 44.73190714600578843 ) ) ;
#15064=CARTESIAN_POINT ( 'NONE',  ( -86.96347745069644475, 15.38646221621772092, 15.38646221621800336 ) ) ;
#15066=CARTESIAN_POINT ( 'NONE',  ( -86.96347745069644475, 15.38646221621793586, -15.38646221621778842 ) ) ;
#15067=CARTESIAN_POINT ( 'NONE',  ( -77.65358652877148415, 21.60549460849031433, -4.394725072386959752 ) ) ;
#15068=CARTESIAN_POINT ( 'NONE',  ( 184.8905102610680444, 14.79361573936424890, -41.77492675555986068 ) ) ;
#15070=CARTESIAN_POINT ( 'NONE',  ( 18.89824403360311678, 24.18164459663371346, 43.99464769172828937 ) ) ;
#15072=CARTESIAN_POINT ( 'NONE',  ( -259.2033419157646676, 21.55415060305790931, 35.01439189186571355 ) ) ;
#15073=CARTESIAN_POINT ( 'NONE',  ( 0.2972598230769983307, -14.33493731733933352, 0.000000000000000000 ) ) ;
#15075=ORIENTED_EDGE ( 'NONE', *, *, #21671, .F. ) ;
#15076=CARTESIAN_POINT ( 'NONE',  ( -86.96347745069644475, 1.775309070576523494E-13, -18.24025645688352881 ) ) ;
#15079=VERTEX_POINT ( 'NONE', #416 ) ;
#15082=CARTESIAN_POINT ( 'NONE',  ( 14.38125909742180752, 55.17850393972636880, 2.449293598294708485E-15 ) ) ;
#15085=CARTESIAN_POINT ( 'NONE',  ( -199.9999999999999716, 55.16984130226958172, 2.449293598294708091E-15 ) ) ;
#15086=CARTESIAN_POINT ( 'NONE',  ( 130.8568914410475372, 1.429239637432775288E-13, -34.05028731879788495 ) ) ;
#15089=CARTESIAN_POINT ( 'NONE',  ( 184.8905102610680444, -14.79361573936399665, 14.79361573936367158 ) ) ;
#15090=CARTESIAN_POINT ( 'NONE',  ( 0.2972598230769976091, -10.13633138497465147, -10.13633138497482733 ) ) ;
#15091=CARTESIAN_POINT ( 'NONE',  ( -110.0738128638427753, -17.41070106609949519, -10.28999680567891417 ) ) ;
#15092=CARTESIAN_POINT ( 'NONE',  ( 151.7948205124836250, 1.012150473917908975E-13, -6.767089262349031742 ) ) ;
#15093=CARTESIAN_POINT ( 'NONE',  ( 184.8905102610680444, 14.79361573936375507, 14.79361573936398067 ) ) ;
#15094=CARTESIAN_POINT ( 'NONE',  ( 18.89824444022306338, 14.00990882958421224, 48.20791849611957502 ) ) ;
#15096=CARTESIAN_POINT ( 'NONE',  ( -91.56559293963834989, 16.03295912088683650, 40.53558337403684675 ) ) ;
#15099=CARTESIAN_POINT ( 'NONE',  ( 151.7948205124836250, 1.439163438361279259E-13, -33.23291073765553705 ) ) ;
#15100=CARTESIAN_POINT ( 'NONE',  ( 14.38125909742180752, 15.17850393972634038, -40.00000000000002132 ) ) ;
#15101=CARTESIAN_POINT ( 'NONE',  ( 130.8568914410475372, -24.07718906447222551, -24.07718906447233209 ) ) ;
#15102=CARTESIAN_POINT ( 'NONE',  ( -238.4067589809705794, 0.9644942799825385604, 40.00000000000002132 ) ) ;
#15103=ORIENTED_EDGE ( 'NONE', *, *, #1436, .T. ) ;
#15104=CARTESIAN_POINT ( 'NONE',  ( 22.17571259161223196, -47.24006242885573670, 13.86510691867743716 ) ) ;
#15105=( GEOMETRIC_REPRESENTATION_CONTEXT ( 3 ) GLOBAL_UNCERTAINTY_ASSIGNED_CONTEXT ( ( #8043 ) ) GLOBAL_UNIT_ASSIGNED_CONTEXT ( ( #13101, #12966, #19214 ) ) REPRESENTATION_CONTEXT ( 'NONE', 'WORKASPACE' ) );
#15106=CARTESIAN_POINT ( 'NONE',  ( 151.7948205124836250, 6.767089262349059275, 2.449293598294708485E-15 ) ) ;
#15107=B_SPLINE_CURVE_WITH_KNOTS ( 'NONE', 3,
 ( #1151, #14980, #9256, #5265, #762, #11126, #13250, #13367 ),
 .UNSPECIFIED., .F., .F.,
 ( 4, 2, 2, 4 ),
 ( 0.0002282271114959515861, 0.004312393619948575417, 0.006354476874174890856, 0.008396560128401207163 ),
 .UNSPECIFIED. ) ;
#15109=CARTESIAN_POINT ( 'NONE',  ( -192.9588430854690273, 10.23066800231970319, 66.79921049724369198 ) ) ;
#15110=CARTESIAN_POINT ( 'NONE',  ( -280.0000000000000568, -40.00000000000000000, -20.00000000000015277 ) ) ;
#15111=CARTESIAN_POINT ( 'NONE',  ( -77.66892440555722033, 21.52311491811582300, -4.720041493164197632 ) ) ;
#15112=AXIS2_PLACEMENT_3D ( 'NONE', #9645, #8041, #24292 ) ;
#15114=AXIS2_PLACEMENT_3D ( 'NONE', #24122, #9752, #24392 ) ;
#15116=CARTESIAN_POINT ( 'NONE',  ( 23.23834162558064165, -13.80856396592285762, -46.85950693578323722 ) ) ;
#15118=CARTESIAN_POINT ( 'NONE',  ( 136.1360204305621551, 3.511608612530062512, 53.05693388239318864 ) ) ;
#15119=CARTESIAN_POINT ( 'NONE',  ( -82.28159816595656650, -19.22531893655055768, 6.254964767081538923 ) ) ;
#15121=FACE_OUTER_BOUND ( 'NONE', #6859, .T. ) ;
#15122=CARTESIAN_POINT ( 'NONE',  ( 192.4448373802100889, -1.741373372144848397E-13, 20.00000000003942091 ) ) ;
#15123=CARTESIAN_POINT ( 'NONE',  ( 19.06497207195981858, -10.03556273973469715, 66.60410523465813526 ) ) ;
#15124=CARTESIAN_POINT ( 'NONE',  ( -82.26533530499490610, 10.28306516078108146, -17.41444274468024034 ) ) ;
#15125=CARTESIAN_POINT ( 'NONE',  ( 146.6084372240433993, 24.48358557860307272, 24.48358557860347418 ) ) ;
#15127=CARTESIAN_POINT ( 'NONE',  ( -109.1264249741456780, -33.12752917268968389, 13.72187187124619712 ) ) ;
#15128=CARTESIAN_POINT ( 'NONE',  ( 19.06497207195981147, 38.31983398719673772, -38.31983398719579981 ) ) ;
#15129=CARTESIAN_POINT ( 'NONE',  ( -86.96347745069644475, -15.38646221621738164, -41.18208027870615240 ) ) ;
#15130=CARTESIAN_POINT ( 'NONE',  ( -30.26275506840324425, 41.69427246844628598, -40.00000000000002132 ) ) ;
#15131=CARTESIAN_POINT ( 'NONE',  ( 14.38125909742180220, 39.01709431150916885, -17.55144818341463164 ) ) ;
#15132=CARTESIAN_POINT ( 'NONE',  ( -238.4067589809705794, -4.716212492215116094E-14, 0.9644942799825824142 ) ) ;
#15133=CARTESIAN_POINT ( 'NONE',  ( -238.4067589809705794, -28.96627169325352469, 27.60227080167035041 ) ) ;
#15135=ORIENTED_EDGE ( 'NONE', *, *, #23619, .F. ) ;
#15137=CARTESIAN_POINT ( 'NONE',  ( -86.96347745069644475, 12.89780903124401057, 12.89780903124407629 ) ) ;
#15138=CARTESIAN_POINT ( 'NONE',  ( -77.90255099906769942, 20.29001641120678201, -8.064892378658056415 ) ) ;
#15139=CARTESIAN_POINT ( 'NONE',  ( -30.26275506840325136, 27.08623969584573388, 29.48230279907808793 ) ) ;
#15140=CARTESIAN_POINT ( 'NONE',  ( -8.255580677125012201, -45.52720393892308692, -13.52904896324569251 ) ) ;
#15141=VERTEX_POINT ( 'NONE', #18768 ) ;
#15145=CARTESIAN_POINT ( 'NONE',  ( 151.7948205124836534, -33.23291073765550863, -40.00000000000002132 ) ) ;
#15146=CARTESIAN_POINT ( 'NONE',  ( 83.07250971299875175, 9.939191265075709936, -23.99533035167571882 ) ) ;
#15148=( BOUNDED_SURFACE ( )  B_SPLINE_SURFACE ( 3, 2, ( 
 ( #25850, #9868, #5613 ),
 ( #20251, #15706, #4029 ),
 ( #7857, #12127, #7594 ),
 ( #10134, #15978, #13719 ),
 ( #18238, #25986, #8133 ),
 ( #1629, #23830, #20118 ),
 ( #1896, #19978, #5879 ),
 ( #15837, #23, #21844 ),
 ( #14124, #19708, #17838 ),
 ( #16250, #3489, #7725 ) ),
 .UNSPECIFIED., .F., .F., .F. ) 
 B_SPLINE_SURFACE_WITH_KNOTS ( ( 4, 2, 2, 2, 4 ),
 ( 3, 3 ),
 ( 0.04143701731387906817, 0.04847035109426007377, 0.05022868453935531996, 0.05198701798445057309, 0.05550368487464107936 ),
 ( 0.000000000000000000, 1.000000000000000000 ),
 .UNSPECIFIED. ) 
 GEOMETRIC_REPRESENTATION_ITEM ( )  RATIONAL_B_SPLINE_SURFACE ( (
 ( 1.000000000000000000, 0.9541700779530978282, 1.000000000000000000),
 ( 1.000000000000000000, 0.9520138072646129324, 1.000000000000000000),
 ( 1.000000000000000000, 0.9503242346225281301, 1.000000000000000000),
 ( 1.000000000000000000, 0.9488844900984083619, 1.000000000000000000),
 ( 1.000000000000000000, 0.9486296596065902920, 1.000000000000000000),
 ( 1.000000000000000000, 0.9481942170211746790, 1.000000000000000000),
 ( 1.000000000000000000, 0.9480132043933685582, 1.000000000000000000),
 ( 1.000000000000000000, 0.9475791817278753637, 1.000000000000000000),
 ( 1.000000000000000000, 0.9474351099635109907, 1.000000000000000000),
 ( 1.000000000000000000, 0.9474350314971535791, 1.000000000000000000) ) ) 
 REPRESENTATION_ITEM ( '' )  SURFACE ( )  );
#15150=CARTESIAN_POINT ( 'NONE',  ( -238.4067589809705794, -0.6820004457913585449, -0.6820004457913265705 ) ) ;
#15151=CARTESIAN_POINT ( 'NONE',  ( 136.1360204305621551, 40.00000000000017053, -35.03383547441281820 ) ) ;
#15152=CARTESIAN_POINT ( 'NONE',  ( -135.8532207217289738, 7.002209520526292428E-15, -9.153146818113572891 ) ) ;
#15155=CARTESIAN_POINT ( 'NONE',  ( 19.06497207195982924, -54.19242893257843008, -40.00000000000002132 ) ) ;
#15156=CARTESIAN_POINT ( 'NONE',  ( 22.31419732600015138, -17.93420418956245399, -43.29699898481643316 ) ) ;
#15159=CARTESIAN_POINT ( 'NONE',  ( 163.1118516004056573, -12.73709011382472589, 40.00000000000002132 ) ) ;
#15161=CARTESIAN_POINT ( 'NONE',  ( -100.7734535825088500, 16.03295912088713848, -16.03295912088698927 ) ) ;
#15162=CARTESIAN_POINT ( 'NONE',  ( -30.26275506840324425, 40.00000000000044764, -41.69427246844585255 ) ) ;
#15163=CARTESIAN_POINT ( 'NONE',  ( -114.4940140761915330, 9.297404372810827766, -19.81979918804517737 ) ) ;
#15164=CARTESIAN_POINT ( 'NONE',  ( 130.8568914410475088, -40.00000000000036238, 34.05028731879746573 ) ) ;
#15168=CARTESIAN_POINT ( 'NONE',  ( 91.82158438592159655, 12.16597498400028776, 44.40256751092339016 ) ) ;
#15170=CARTESIAN_POINT ( 'NONE',  ( -77.59212294118373165, 2.762334042793177513, -21.93719684953127569 ) ) ;
#15171=CARTESIAN_POINT ( 'NONE',  ( -3.856733984653753389, 43.19294614843423830, -17.89110409353217079 ) ) ;
#15172=CARTESIAN_POINT ( 'NONE',  ( 4.995406935893294431, -15.24977328854832415, 40.00000000000002132 ) ) ;
#15174=CARTESIAN_POINT ( 'NONE',  ( -190.0144222802798879, 43.47820992357031145, -23.79986276082225771 ) ) ;
#15177=VERTEX_POINT ( 'NONE', #5067 ) ;
#15178=CARTESIAN_POINT ( 'NONE',  ( -30.26275506840324070, -1.198031551616032919, 1.198031551616014712 ) ) ;
#15185=CARTESIAN_POINT ( 'NONE',  ( 57.59792236341147031, -1.722363176415123043, 54.84617931850879557 ) ) ;
#15186=CARTESIAN_POINT ( 'NONE',  ( -56.48582580120559271, -6.472252184284187138, -6.472252184284199572 ) ) ;
#15187=CARTESIAN_POINT ( 'NONE',  ( -238.4067589809705794, 39.99999999999997158, 0.9644942799827220803 ) ) ;
#15190=CARTESIAN_POINT ( 'NONE',  ( -91.56559293963834989, -40.00000000000027711, 22.67402823373149801 ) ) ;
#15191=CARTESIAN_POINT ( 'NONE',  ( -238.4067589809705794, 3.877349844572403567E-13, -40.96449427998260973 ) ) ;
#15192=CARTESIAN_POINT ( 'NONE',  ( 190.0000000000001137, 3.490243377569959927E-14, 0.000000000000000000 ) ) ;
#15193=CARTESIAN_POINT ( 'NONE',  ( -208.1127848780264742, -67.17687982763172272, 10.60833733270744617 ) ) ;
#15194=CARTESIAN_POINT ( 'NONE',  ( -200.0000000000000568, 22.84381638316583008, -44.98788141756660508 ) ) ;
#15195=EDGE_CURVE ( 'NONE', #9216, #12216, #5334, .T. ) ;
#15196=CARTESIAN_POINT ( 'NONE',  ( -194.4222775680397319, 24.44979664543011566, 44.35790405183560381 ) ) ;
#15197=CARTESIAN_POINT ( 'NONE',  ( -105.4741150117389168, 7.943527260764259523, 19.77569912954497866 ) ) ;
#15198=CARTESIAN_POINT ( 'NONE',  ( -188.5332420855862097, -47.07509783859007513, 13.84065984181806819 ) ) ;
#15199=DIRECTION ( 'NONE',  ( 1.000000000000000000, 1.836970198721030181E-16, 0.000000000000000000 ) ) ;
#15200=CARTESIAN_POINT ( 'NONE',  ( -82.26674357278778871, -17.37244534973704191, 10.27857254525268083 ) ) ;
#15201=CARTESIAN_POINT ( 'NONE',  ( -208.1127848780264742, -38.89260858015753541, 17.67593391476614784 ) ) ;
#15203=CARTESIAN_POINT ( 'NONE',  ( 170.0000000000000000, 12.70659020859108601, -21.59613885783087284 ) ) ;
#15205=CARTESIAN_POINT ( 'NONE',  ( -208.1127848780264742, 67.17687982763172272, -10.60833733270698254 ) ) ;
#15206=CARTESIAN_POINT ( 'NONE',  ( 169.9999999999999716, 22.62041470344888339, -9.369682556672254137 ) ) ;
#15207=( BOUNDED_SURFACE ( )  B_SPLINE_SURFACE ( 3, 2, ( 
 ( #16634, #14764, #10787 ),
 ( #18764, #6913, #4810 ),
 ( #12912, #15030, #17155 ),
 ( #23160, #24763, #6516 ),
 ( #9050, #13045, #2537 ),
 ( #19032, #22764, #548 ),
 ( #6649, #20767, #4939 ),
 ( #8785, #2936, #10655 ),
 ( #16898, #4544, #11046 ),
 ( #12642, #25289, #16760 ),
 ( #7046, #24894, #22894 ),
 ( #14895, #12775, #25030 ),
 ( #4673, #2680, #6783 ),
 ( #23035, #9173, #5064 ),
 ( #15163, #17286, #25420 ),
 ( #23288, #3065, #13170 ) ),
 .UNSPECIFIED., .F., .F., .F. ) 
 B_SPLINE_SURFACE_WITH_KNOTS ( ( 4, 2, 2, 2, 2, 2, 2, 4 ),
 ( 3, 3 ),
 ( 0.04143342415525530509, 0.04844520228004854656, 0.05195109134244516036, 0.05545698040484178110, 0.06246875852963501563, 0.06422170306083332947, 0.06597464759203164331, 0.06948053665442825710 ),
 ( 0.000000000000000000, 1.000000000000000000 ),
 .UNSPECIFIED. ) 
 GEOMETRIC_REPRESENTATION_ITEM ( )  RATIONAL_B_SPLINE_SURFACE ( (
 ( 1.000000000000000000, 0.9541700777564544600, 1.000000000000000000),
 ( 1.000000000000000000, 0.9520170179167380953, 1.000000000000000000),
 ( 1.000000000000000000, 0.9503264940257962756, 1.000000000000000000),
 ( 1.000000000000000000, 0.9485966650361820074, 1.000000000000000000),
 ( 1.000000000000000000, 0.9481601953988942899, 1.000000000000000000),
 ( 1.000000000000000000, 0.9475786562870265328, 1.000000000000000000),
 ( 1.000000000000000000, 0.9474333041668372424, 1.000000000000000000),
 ( 1.000000000000000000, 0.9474385324107064132, 1.000000000000000000),
 ( 1.000000000000000000, 0.9480205960585557090, 1.000000000000000000),
 ( 1.000000000000000000, 0.9494433550395547927, 1.000000000000000000),
 ( 1.000000000000000000, 0.9497628485354062677, 1.000000000000000000),
 ( 1.000000000000000000, 0.9504717112743313878, 1.000000000000000000),
 ( 1.000000000000000000, 0.9508623530679617408, 1.000000000000000000),
 ( 1.000000000000000000, 0.9521262215771475468, 1.000000000000000000),
 ( 1.000000000000000000, 0.9530922057181885343, 1.000000000000000000),
 ( 1.000000000000000000, 0.9541700777564462443, 1.000000000000000000) ) ) 
 REPRESENTATION_ITEM ( '' )  SURFACE ( )  );
#15209=ORIENTED_EDGE ( 'NONE', *, *, #24791, .F. ) ;
#15210=CARTESIAN_POINT ( 'NONE',  ( -208.1127848780264742, -39.99999999999948841, -55.00245453010965235 ) ) ;
#15212=CARTESIAN_POINT ( 'NONE',  ( -53.37769371738607305, 13.65853730965348589, 27.95780717557936157 ) ) ;
#15213=ORIENTED_EDGE ( 'NONE', *, *, #15610, .F. ) ;
#15214=ORIENTED_EDGE ( 'NONE', *, *, #3287, .T. ) ;
#15215=CARTESIAN_POINT ( 'NONE',  ( -162.0762913951020892, 41.69427287682832173, 2.449293598294708485E-15 ) ) ;
#15217=CARTESIAN_POINT ( 'NONE',  ( -175.9235640284969122, -12.95568063919091273, 42.70623598242575270 ) ) ;
#15218=CARTESIAN_POINT ( 'NONE',  ( 14.38125909742181108, -5.035366881890652543E-14, 15.17850393972633682 ) ) ;
#15220=CARTESIAN_POINT ( 'NONE',  ( -17.28139728231351313, -12.88180358351685406, -42.38047544416907186 ) ) ;
#15221=CARTESIAN_POINT ( 'NONE',  ( -280.0000000000000568, 14.14213562373127431, -42.42640687119274645 ) ) ;
#15222=CARTESIAN_POINT ( 'NONE',  ( -110.0961830520393505, -15.97565819499239481, -12.41691170628179286 ) ) ;
#15223=CARTESIAN_POINT ( 'NONE',  ( 91.82158438592159655, -39.99999999999976552, -22.79471317813512599 ) ) ;
#15225=CARTESIAN_POINT ( 'NONE',  ( 136.1360204305621266, 35.03383547441298163, -40.00000000000002132 ) ) ;
#15226=CARTESIAN_POINT ( 'NONE',  ( 184.8905102610680444, -41.77492675555986779, -14.79361573936407304 ) ) ;
#15227=CARTESIAN_POINT ( 'NONE',  ( 163.1118516004056573, 27.26290988616876021, -40.00000000000002132 ) ) ;
#15229=CARTESIAN_POINT ( 'NONE',  ( -192.9588430854690273, 39.99999999999992895, 14.46834944099983922 ) ) ;
#15230=CARTESIAN_POINT ( 'NONE',  ( 151.7948205124836250, -33.23291073765550863, 0.000000000000000000 ) ) ;
#15231=CARTESIAN_POINT ( 'NONE',  ( -105.3755690713226585, -15.38646221621796251, 41.18208027870593924 ) ) ;
#15232=CARTESIAN_POINT ( 'NONE',  ( -238.4067589809705794, 40.96449427998256709, 2.449293598294708485E-15 ) ) ;
#15233=VERTEX_POINT ( 'NONE', #7419 ) ;
#15234=CARTESIAN_POINT ( 'NONE',  ( 19.94008347562200711, -43.76810615267664417, 24.01421467034317914 ) ) ;
#15235=CARTESIAN_POINT ( 'NONE',  ( -259.2033419157646676, 30.48217210827735713, -40.00000000000002132 ) ) ;
#15237=CARTESIAN_POINT ( 'NONE',  ( 170.2234770963711128, -45.64576402573183600, 10.92277846919191653 ) ) ;
#15238=B_SPLINE_CURVE_WITH_KNOTS ( 'NONE', 3,
 ( #13432, #25436, #17422, #11183, #21309, #7434, #7310, #23675, #13557, #21683, #3457, #25563 ),
 .UNSPECIFIED., .F., .F.,
 ( 4, 2, 2, 2, 2, 4 ),
 ( 2.797157557069881010E-17, 0.004680202113614255650, 0.009360404227228483545, 0.01170050528403559879, 0.01404060634084271231, 0.01872080845445698097 ),
 .UNSPECIFIED. ) ;
#15239=CARTESIAN_POINT ( 'NONE',  ( -192.9588430854690273, -40.00000000000011369, 14.46834944099955855 ) ) ;
#15242=CARTESIAN_POINT ( 'NONE',  ( 7.340276806054849779, -14.17250878947572446, -49.28408872342600944 ) ) ;
#15245=EDGE_CURVE ( 'NONE', #15766, #3292, #1854, .T. ) ;
#15246=CARTESIAN_POINT ( 'NONE',  ( -87.11138134864528126, -2.725552644157975379, -21.34736238710377521 ) ) ;
#15247=CARTESIAN_POINT ( 'NONE',  ( -100.7734535825088500, 12.25131212657428748, 44.31723036834913643 ) ) ;
#15248=VECTOR ( 'NONE', #13873, 1000.000000000000000 ) ;
#15249=CARTESIAN_POINT ( 'NONE',  ( -100.7734535825088500, 44.31723036834907958, -12.25131212657445801 ) ) ;
#15251=CARTESIAN_POINT ( 'NONE',  ( -135.8532207217289738, 34.75652343174594705, 21.81201906317792449 ) ) ;
#15252=CARTESIAN_POINT ( 'NONE',  ( -83.28983882461061228, -25.45044590560980424, -25.45044590561024478 ) ) ;
#15253=CARTESIAN_POINT ( 'NONE',  ( -238.4067589809705794, 27.60227080167080160, -28.96627169325299533 ) ) ;
#15254=CARTESIAN_POINT ( 'NONE',  ( 0.2972598230769976091, -10.13633138497465147, -10.13633138497482733 ) ) ;
#15255=CARTESIAN_POINT ( 'NONE',  ( -259.2033419157646676, -35.01439189186523748, -21.55415060305881170 ) ) ;
#15256=CARTESIAN_POINT ( 'NONE',  ( 200.0000000000000000, 42.42640687119267540, 14.14213562373153543 ) ) ;
#15257=CIRCLE ( 'NONE', #12774, 15.00000000000000000 ) ;
#15258=CARTESIAN_POINT ( 'NONE',  ( -162.0762913951020892, 1.694272876828294194, 0.000000000000000000 ) ) ;
#15260=CARTESIAN_POINT ( 'NONE',  ( -91.56559293963834989, 6.234561990864368500E-14, -22.67402823373191723 ) ) ;
#15261=CARTESIAN_POINT ( 'NONE',  ( -105.3755690713226585, -12.89780903124444578, 43.67073346367968156 ) ) ;
#15262=CARTESIAN_POINT ( 'NONE',  ( -188.3508614409174129, 43.15762572182595136, -17.87647389380071772 ) ) ;
#15264=CARTESIAN_POINT ( 'NONE',  ( -198.0356074513804572, 39.15871834505901461, 39.15871834505919935 ) ) ;
#15266=CARTESIAN_POINT ( 'NONE',  ( 11.38508063392505321, 14.17561098846279144, 49.30460303391076593 ) ) ;
#15267=CARTESIAN_POINT ( 'NONE',  ( -86.86493150571114086, -19.77569912839162569, 7.943527260496431985 ) ) ;
#15271=CARTESIAN_POINT ( 'NONE',  ( 22.89002945277442791, -17.87003923493671920, 43.14209108112122237 ) ) ;
#15273=FACE_OUTER_BOUND ( 'NONE', #3197, .T. ) ;
#15275=CARTESIAN_POINT ( 'NONE',  ( 98.29820294270304259, -18.47759065022024672, 7.653668647299475047 ) ) ;
#15276=CARTESIAN_POINT ( 'NONE',  ( 0.2972598230769957217, -4.999556039334937811E-14, 14.33493731733933352 ) ) ;
#15277=CARTESIAN_POINT ( 'NONE',  ( -87.02160325129693774, -5.407498138847803837, 20.76752817463990652 ) ) ;
#15278=CARTESIAN_POINT ( 'NONE',  ( 5.009865950673472845, 49.09576456953151080, -14.14399394884951455 ) ) ;
#15279=CARTESIAN_POINT ( 'NONE',  ( -100.7734535825088358, -17.32597176626813251, -2.449293598294708485E-15 ) ) ;
#15280=CARTESIAN_POINT ( 'NONE',  ( 21.80824205439828134, -23.67346680102911094, -43.30754100652708871 ) ) ;
#15281=CARTESIAN_POINT ( 'NONE',  ( -56.48582580120559271, 6.472252184284211118, -6.472252184284153387 ) ) ;
#15282=CARTESIAN_POINT ( 'NONE',  ( 146.6084372240433709, 34.62501878078307982, 40.00000000000002132 ) ) ;
#15283=CARTESIAN_POINT ( 'NONE',  ( -259.2033419157646676, 9.517827891722584255, -0.000000000000000000 ) ) ;
#15284=CARTESIAN_POINT ( 'NONE',  ( 184.8905102610680444, -1.851754852062639767E-13, 20.92133201514444352 ) ) ;
#15285=CARTESIAN_POINT ( 'NONE',  ( -213.1075012329537230, -39.99999999999948841, -53.71589010950208376 ) ) ;
#15287=CARTESIAN_POINT ( 'NONE',  ( 121.8729990817667641, -26.81364411578696405, -11.10657504940452611 ) ) ;
#15289=ORIENTED_EDGE ( 'NONE', *, *, #18838, .F. ) ;
#15290=CARTESIAN_POINT ( 'NONE',  ( 0.2972598230769976091, -10.13633138497465147, -10.13633138497482733 ) ) ;
#15291=CARTESIAN_POINT ( 'NONE',  ( -3.439026802539385752, 43.30533194338906355, -17.93765581402026754 ) ) ;
#15292=CARTESIAN_POINT ( 'NONE',  ( 199.9999999999999432, -19.99999999999988987, -2.449293598294708485E-15 ) ) ;
#15293=ADVANCED_FACE ( 'NONE', ( #26344 ), #18617, .T. ) ;
#15295=CARTESIAN_POINT ( 'NONE',  ( -188.3392535381850621, 43.01687576774367727, -23.45796413246022638 ) ) ;
#15301=CARTESIAN_POINT ( 'NONE',  ( 136.1360204305621266, 1.473277640373554421E-13, -35.03383547441296741 ) ) ;
#15304=CARTESIAN_POINT ( 'NONE',  ( -188.2995950289364373, 13.82811170417132196, 46.99046209955516673 ) ) ;
#15306=CARTESIAN_POINT ( 'NONE',  ( -100.7734535825088500, 40.53558337403677569, -16.03295912088699993 ) ) ;
#15308=CARTESIAN_POINT ( 'NONE',  ( -208.1127848780265026, -9.061048840815752106E-14, 15.00245453012669472 ) ) ;
#15309=CARTESIAN_POINT ( 'NONE',  ( 0.4226707250629958557, -14.03458789212657720, 48.37218667320259868 ) ) ;
#15312=CARTESIAN_POINT ( 'NONE',  ( 57.59792236341149163, -39.99999999999961631, -37.56421063658228832 ) ) ;
#15313=CARTESIAN_POINT ( 'NONE',  ( -198.0356074513804572, 5.461327841961909642E-13, -55.37879056873073580 ) ) ;
#15314=CARTESIAN_POINT ( 'NONE',  ( -110.0574180503312363, -18.01801597171421676, 9.169691069511660686 ) ) ;
#15315=CARTESIAN_POINT ( 'NONE',  ( -238.4067589809705794, -57.25054294065807881, 0.6820004457338858517 ) ) ;
#15316=CARTESIAN_POINT ( 'NONE',  ( 192.4448373802101173, 40.00000000000012790, -20.00000000003928236 ) ) ;
#15319=B_SPLINE_CURVE_WITH_KNOTS ( 'NONE', 3,
 ( #12527, #15056, #16528, #24790, #20526, #4701, #20661, #22922, #12808, #24656, #838, #20930, #4434, #22662 ),
 .UNSPECIFIED., .F., .F.,
 ( 4, 2, 2, 2, 2, 2, 4 ),
 ( 1.734723475976806902E-18, 0.002941681445496980695, 0.004412522168245476897, 0.005883362890993972666, 0.008825044336490964203, 0.01029588505923946344, 0.01176672578198796268 ),
 .UNSPECIFIED. ) ;
#15321=CARTESIAN_POINT ( 'NONE',  ( 4.995406935893293543, -10.78321810389005364, 10.78321810388994173 ) ) ;
#15322=CARTESIAN_POINT ( 'NONE',  ( -77.90255099906779890, -8.644468104261020969, 20.04994828523974704 ) ) ;
#15323=CARTESIAN_POINT ( 'NONE',  ( -86.96347745069644475, 12.89780903124401057, 12.89780903124407629 ) ) ;
#15324=CARTESIAN_POINT ( 'NONE',  ( 199.9999999999999432, -14.14213562373073607, -14.14213562373102206 ) ) ;
#15325=CARTESIAN_POINT ( 'NONE',  ( -144.0562696876088182, -10.50947022294722011, -31.27040355054280951 ) ) ;
#15326=CARTESIAN_POINT ( 'NONE',  ( 170.0000000000000000, 15.47746304364920356, -19.80854622259135311 ) ) ;
#15327=ORIENTED_EDGE ( 'NONE', *, *, #11555, .T. ) ;
#15328=CARTESIAN_POINT ( 'NONE',  ( 163.1118516004056573, 9.006482792069759213, -9.006482792069505194 ) ) ;
#15333=CARTESIAN_POINT ( 'NONE',  ( 14.38125909742181108, 1.616281842095393922E-13, -15.17850393972633682 ) ) ;
#15335=CARTESIAN_POINT ( 'NONE',  ( -2.937533998796872048, -43.32931883107630711, 23.68967259549630455 ) ) ;
#15337=ORIENTED_EDGE ( 'NONE', *, *, #3381, .T. ) ;
#15339=CARTESIAN_POINT ( 'NONE',  ( -259.2033419157646676, -21.55415060305824326, -35.01439189186556433 ) ) ;
#15340=CARTESIAN_POINT ( 'NONE',  ( 163.1118516004056573, -1.695744499706194789E-14, 12.73709011382475254 ) ) ;
#15341=EDGE_CURVE ( 'NONE', #18786, #15843, #10428, .T. ) ;
#15342=EDGE_CURVE ( 'NONE', #3040, #8031, #1291, .T. ) ;
#15349=CARTESIAN_POINT ( 'NONE',  ( -83.21262154144247347, -13.72187187061530977, 33.12752917118402962 ) ) ;
#15351=CARTESIAN_POINT ( 'NONE',  ( -47.65341557553326624, -14.80716566697267211, -29.74088027399182010 ) ) ;
#15352=CARTESIAN_POINT ( 'NONE',  ( 19.06497207195981858, -10.03556273973377166, -66.60410523465827737 ) ) ;
#15353=CARTESIAN_POINT ( 'NONE',  ( 98.29820294267423719, -14.14213562374330024, 14.14213562372619926 ) ) ;
#15354=CARTESIAN_POINT ( 'NONE',  ( -105.3755690713226727, 1.741486606973311632E-13, -18.24025645688352881 ) ) ;
#15356=CARTESIAN_POINT ( 'NONE',  ( 4.995406935893294431, -15.24977328854832415, 40.00000000000002132 ) ) ;
#15357=CARTESIAN_POINT ( 'NONE',  ( -213.1075012329537230, -13.71589010951915810, -40.00000000000002132 ) ) ;
#15358=CARTESIAN_POINT ( 'NONE',  ( -192.9588430854690273, 18.05360324515418924, 38.51493924976949756 ) ) ;
#15359=CARTESIAN_POINT ( 'NONE',  ( -86.96347745069643054, -18.24025645688353947, -40.00000000000002132 ) ) ;
#15360=CARTESIAN_POINT ( 'NONE',  ( 98.29820294272737158, 12.38338430224885656, 15.90088694521805301 ) ) ;
#15361=CARTESIAN_POINT ( 'NONE',  ( -198.0356074513804572, 39.99999999999992895, 15.37879056873084771 ) ) ;
#15363=CARTESIAN_POINT ( 'NONE',  ( -105.3755690713226585, 41.18208027870598187, -15.38646221621779731 ) ) ;
#15364=CARTESIAN_POINT ( 'NONE',  ( 146.6084372240433993, 5.374981219216999229, 2.449293598294708485E-15 ) ) ;
#15366=CARTESIAN_POINT ( 'NONE',  ( 23.26364522860174944, -42.89098160628003598, 23.36474233297283121 ) ) ;
#15369=CARTESIAN_POINT ( 'NONE',  ( 14.38125909742181463, 10.73282306405862485, 67.30136555898259587 ) ) ;
#15370=CARTESIAN_POINT ( 'NONE',  ( 136.1360204305621266, 1.473277640373554421E-13, -35.03383547441296741 ) ) ;
#15371=CARTESIAN_POINT ( 'NONE',  ( -77.56706372485132306, 22.07323241864502350, 1.630297477738017475 ) ) ;
#15372=CARTESIAN_POINT ( 'NONE',  ( -8.255580677152625668, 22.62611236875380882, -41.75907689858282623 ) ) ;
#15375=CARTESIAN_POINT ( 'NONE',  ( -77.79459117303389348, -6.798990169609631096, -20.85444474317636221 ) ) ;
#15376=CARTESIAN_POINT ( 'NONE',  ( -280.0000000000000568, 14.14213562373038968, 42.42640687119305198 ) ) ;
#15377=CARTESIAN_POINT ( 'NONE',  ( -238.4067589809705794, -28.96627169325303797, -28.96627169325349627 ) ) ;
#15378=CARTESIAN_POINT ( 'NONE',  ( -280.0000000000000000, 14.14213562373098299, -14.14213562373088706 ) ) ;
#15379=CARTESIAN_POINT ( 'NONE',  ( 4.995406935893289102, 10.78321810389013002, -10.78321810388986712 ) ) ;
#15380=CARTESIAN_POINT ( 'NONE',  ( 91.82158438592159655, 12.16597498400091304, -44.40256751092321963 ) ) ;
#15382=CARTESIAN_POINT ( 'NONE',  ( 192.4448373802101173, 14.14213562375922884, -42.42640687116488607 ) ) ;
#15383=CARTESIAN_POINT ( 'NONE',  ( 163.1118516004056573, -19.27778845539181063, -37.29075403953176959 ) ) ;
#15384=CARTESIAN_POINT ( 'NONE',  ( 57.59792236341147031, 26.56190807104720975, -26.56190807104655249 ) ) ;
#15385=CARTESIAN_POINT ( 'NONE',  ( -105.3895334812081046, -9.637394427343657810, 19.08270859417689636 ) ) ;
#15387=CARTESIAN_POINT ( 'NONE',  ( 151.7948205124835681, -4.785054706298876859, 51.78348778862533663 ) ) ;
#15388=CARTESIAN_POINT ( 'NONE',  ( -188.2506440019887464, 42.99080317017362063, -23.43978047293228073 ) ) ;
#15390=CARTESIAN_POINT ( 'NONE',  ( -192.9588430854690273, 38.51493924976939098, -18.05360324515436687 ) ) ;
#15391=CARTESIAN_POINT ( 'NONE',  ( -77.90255099906777048, -20.04994828523985362, -8.644468104260763397 ) ) ;
#15392=CARTESIAN_POINT ( 'NONE',  ( 23.64688638900176798, 13.78084749393323705, 46.70960658758804129 ) ) ;
#15393=CARTESIAN_POINT ( 'NONE',  ( -7.726389047727876047, -42.14052505959300987, -17.45517700519032900 ) ) ;
#15395=CARTESIAN_POINT ( 'NONE',  ( -174.2681662547478822, -39.26785901283194136, 16.26527976840799639 ) ) ;
#15398=CARTESIAN_POINT ( 'NONE',  ( 27.79909650601494064, -22.43832426414681080, 41.49206490658713875 ) ) ;
#15399=CARTESIAN_POINT ( 'NONE',  ( 170.0000000000427178, -17.64300463311358769, 17.64300463311318268 ) ) ;
#15401=CARTESIAN_POINT ( 'NONE',  ( -100.0753760173616058, -20.41987330121787636, -8.894334231739460250 ) ) ;
#15402=CARTESIAN_POINT ( 'NONE',  ( -56.48582580120559982, 39.99999999999990763, 30.84685318188658698 ) ) ;
#15403=CARTESIAN_POINT ( 'NONE',  ( -83.21262154144264400, 13.72187187061491720, -33.12752917118420726 ) ) ;
#15404=CARTESIAN_POINT ( 'NONE',  ( -199.9999999999999432, -21.40989205436278908, -45.24754806069001489 ) ) ;
#15405=CARTESIAN_POINT ( 'NONE',  ( -135.8532207217289454, -30.84685318188649106, 40.00000000000002132 ) ) ;
#15406=CARTESIAN_POINT ( 'NONE',  ( 67.79414719528381283, -10.30785037377898661, -30.31905270957335929 ) ) ;
#15408=CARTESIAN_POINT ( 'NONE',  ( 4.995406935893294431, -15.24977328854832415, 40.00000000000002132 ) ) ;
#15409=CARTESIAN_POINT ( 'NONE',  ( -162.0762913951020892, -1.694272876828353702, 0.000000000000000000 ) ) ;
#15410=CARTESIAN_POINT ( 'NONE',  ( 146.6084372240433709, 39.99999999999968026, 34.62501878078347772 ) ) ;
#15411=CARTESIAN_POINT ( 'NONE',  ( -259.2033419157646676, -40.00000000000017053, 9.517827891722212996 ) ) ;
#15412=CARTESIAN_POINT ( 'NONE',  ( 156.1976257969618587, -27.38429663762786248, -11.34294706335341196 ) ) ;
#15413=ORIENTED_EDGE ( 'NONE', *, *, #12425, .F. ) ;
#15414=FACE_OUTER_BOUND ( 'NONE', #5618, .T. ) ;
#15415=CARTESIAN_POINT ( 'NONE',  ( -4.112199523539852741, 42.98379141459112418, -23.43514144949442723 ) ) ;
#15416=CARTESIAN_POINT ( 'NONE',  ( 136.1360204305621551, -4.966164525587043244, 40.00000000000002132 ) ) ;
#15417=CARTESIAN_POINT ( 'NONE',  ( -126.6834154282210108, -24.89646316986487662, 9.107266658309272955 ) ) ;
#15418=CARTESIAN_POINT ( 'NONE',  ( -188.4265004370459735, 43.04236487214743789, -23.47686928852965593 ) ) ;
#15422=CARTESIAN_POINT ( 'NONE',  ( -96.93773665439012177, -20.58457565566412129, 9.001171854901890867 ) ) ;
#15423=CARTESIAN_POINT ( 'NONE',  ( 133.2080217031554525, 12.38638889282743527, -29.90338805389109922 ) ) ;
#15425=EDGE_LOOP ( 'NONE', ( #14289, #10430, #25654, #1332, #10866 ) ) ;
#15428=CARTESIAN_POINT ( 'NONE',  ( 130.8568914410475088, 32.49135343045483637, -24.07718906446901030 ) ) ;
#15430=CARTESIAN_POINT ( 'NONE',  ( -86.96347745069644475, 5.999880687339585546E-14, -21.75974354311649961 ) ) ;
#15434=CARTESIAN_POINT ( 'NONE',  ( -208.1127848780264742, -39.99999999999948841, -55.00245453010965235 ) ) ;
#15435=CARTESIAN_POINT ( 'NONE',  ( 163.1118516004056573, 1.658263919738574066E-13, -12.73709011382475254 ) ) ;
#15436=CARTESIAN_POINT ( 'NONE',  ( -82.23879574654692703, 15.18736141609909751, 13.32665427271416014 ) ) ;
#15437=CARTESIAN_POINT ( 'NONE',  ( 19.06497207195981147, -10.03556273973439517, 10.03556273973429214 ) ) ;
#15438=CARTESIAN_POINT ( 'NONE',  ( -213.1075012329537230, -8.703598725189323045E-14, 13.71589010951911902 ) ) ;
#15439=CARTESIAN_POINT ( 'NONE',  ( 163.1118516004056573, 19.27778845538780317, -19.27778845538757224 ) ) ;
#15440=CARTESIAN_POINT ( 'NONE',  ( 158.3379117892986585, 26.51167085133952739, 10.98149362779641791 ) ) ;
#15441=CARTESIAN_POINT ( 'NONE',  ( -77.90255099906859471, -8.644468104251766150, 20.04994828524300843 ) ) ;
#15443=CARTESIAN_POINT ( 'NONE',  ( -77.79459117301121296, -19.55393134993891380, 9.938707241634757494 ) ) ;
#15444=CARTESIAN_POINT ( 'NONE',  ( 184.8905102610680444, -43.07788698682576722, 13.49065550809799063 ) ) ;
#15445=CARTESIAN_POINT ( 'NONE',  ( -135.8532207217289738, -21.81201906317806305, 34.75652343174590442 ) ) ;
#15450=CARTESIAN_POINT ( 'NONE',  ( -192.9588430854690273, 10.23066800229588758, -66.79921049721882298 ) ) ;
#15452=CARTESIAN_POINT ( 'NONE',  ( -109.1264249741456780, -13.72187187121290108, 33.12752917270401554 ) ) ;
#15455=CARTESIAN_POINT ( 'NONE',  ( -3.901164313503183045, -23.47934491069901597, 43.04571088859064787 ) ) ;
#15456=CARTESIAN_POINT ( 'NONE',  ( -77.90255099907078318, 8.064892378657827265, 20.29001641120558830 ) ) ;
#15458=ORIENTED_EDGE ( 'NONE', *, *, #9390, .T. ) ;
#15459=CARTESIAN_POINT ( 'NONE',  ( -200.5022929845067949, -44.86988025226713717, -18.58571294254476314 ) ) ;
#15460=CARTESIAN_POINT ( 'NONE',  ( 57.59792236341147742, -1.230234673553095937E-13, 37.56421063658186199 ) ) ;
#15461=CARTESIAN_POINT ( 'NONE',  ( -89.91646883266054147, -20.29783361042684575, -8.407637968085085234 ) ) ;
#15464=CARTESIAN_POINT ( 'NONE',  ( -91.56559293963834989, -40.00000000000009948, 17.32597176626796553 ) ) ;
#15467=CARTESIAN_POINT ( 'NONE',  ( -77.90022806218901508, -8.352332316461509976, -20.16431395584806907 ) ) ;
#15468=CARTESIAN_POINT ( 'NONE',  ( 130.8568914410475372, 24.07718906447210472, 24.07718906447249907 ) ) ;
#15470=CARTESIAN_POINT ( 'NONE',  ( -198.0356074513804572, -39.99999999999948130, -55.37879056874863437 ) ) ;
#15471=CARTESIAN_POINT ( 'NONE',  ( -105.2054292635175585, -21.49321519473986442, -7.030298963786045751E-29 ) ) ;
#15472=CARTESIAN_POINT ( 'NONE',  ( -213.1075012329537230, -13.71589010951915810, 40.00000000000002132 ) ) ;
#15473=CARTESIAN_POINT ( 'NONE',  ( -213.1075012329537230, -53.71589010953668719, -40.00000000000002132 ) ) ;
#15475=EDGE_CURVE ( 'NONE', #11726, #17509, #603, .T. ) ;
#15476=CARTESIAN_POINT ( 'NONE',  ( -86.96347745069644475, 15.38646221621793586, -15.38646221621778842 ) ) ;
#15477=CARTESIAN_POINT ( 'NONE',  ( -162.0762913951021176, -1.694272876828353702, -40.00000000000002132 ) ) ;
#15479=DIRECTION ( 'NONE',  ( 0.9352143323239480166, -0.1355013636715377279, -0.3271292299062040776 ) ) ;
#15480=CARTESIAN_POINT ( 'NONE',  ( 19.06497207195981147, 1.521599808664285085E-13, -14.19242893257840521 ) ) ;
#15481=CARTESIAN_POINT ( 'NONE',  ( 57.59792236341147031, 26.56190807104684382, 26.56190807104692553 ) ) ;
#15482=CARTESIAN_POINT ( 'NONE',  ( -259.2033419157646676, 30.48217210827734647, 2.449293598294708485E-15 ) ) ;
#15484=CARTESIAN_POINT ( 'NONE',  ( 25.05785482535806707, -42.53113694076518669, 17.61697374403330585 ) ) ;
#15486=CARTESIAN_POINT ( 'NONE',  ( 0.2972598230769959993, 38.42060263243659080, 38.42060263243672580 ) ) ;
#15487=CARTESIAN_POINT ( 'NONE',  ( -208.1127848780265026, -9.061048840815752106E-14, 15.00245453012669472 ) ) ;
#15488=CARTESIAN_POINT ( 'NONE',  ( -87.13563633338503678, 21.50639108511650122, -1.206565891102790777 ) ) ;
#15489=CARTESIAN_POINT ( 'NONE',  ( 3.854699808470068767, -14.12217777258740270, -48.95177852071788038 ) ) ;
#15491=CARTESIAN_POINT ( 'NONE',  ( -86.86493150571118349, -19.77569912839185307, -7.943527260495925724 ) ) ;
#15492=CARTESIAN_POINT ( 'NONE',  ( -87.13348102042543530, -1.376917454623202364, -21.49232615835870419 ) ) ;
#15493=CARTESIAN_POINT ( 'NONE',  ( -198.0356074513804572, 10.87444709759730088, -10.87444709759707173 ) ) ;
#15494=CARTESIAN_POINT ( 'NONE',  ( -100.7734535825088358, -12.25131212657475643, -12.25131212657495539 ) ) ;
#15495=CARTESIAN_POINT ( 'NONE',  ( -110.1004897823566324, 20.16745930835667266, -1.096875637590350339 ) ) ;
#15496=CARTESIAN_POINT ( 'NONE',  ( -86.86493150571114086, -8.366608963953616751, 19.60045294882772993 ) ) ;
#15497=CARTESIAN_POINT ( 'NONE',  ( -198.0356074513804572, -10.87444709758429262, -67.44298959250878056 ) ) ;
#15498=CARTESIAN_POINT ( 'NONE',  ( -259.2033419157646676, 6.730120644403918995, -49.83842185052024831 ) ) ;
#15499=CARTESIAN_POINT ( 'NONE',  ( -208.1127848780264742, -17.67593391476605547, -38.89260858015755673 ) ) ;
#15500=CARTESIAN_POINT ( 'NONE',  ( 91.82158438592158234, 16.11829626346161604, -16.11829626346121103 ) ) ;
#15503=CARTESIAN_POINT ( 'NONE',  ( 130.8568914410475088, -39.99999999999988631, -34.05028731879802706 ) ) ;
#15505=CARTESIAN_POINT ( 'NONE',  ( -208.1127848780264742, -38.89260858015753541, 17.67593391476614784 ) ) ;
#15507=CARTESIAN_POINT ( 'NONE',  ( -259.2033419157646676, 30.48217210827734647, 2.449293598294708485E-15 ) ) ;
#15509=CARTESIAN_POINT ( 'NONE',  ( -259.2033419157646676, 21.55415060305839958, -35.01439189186541512 ) ) ;
#15511=CARTESIAN_POINT ( 'NONE',  ( 67.67011021022710793, 12.13550330113689668, 29.29769665552182545 ) ) ;
#15512=CARTESIAN_POINT ( 'NONE',  ( -5.296937277115072007, -42.80341339122408328, -17.72975434250616544 ) ) ;
#15514=DIRECTION ( 'NONE',  ( 0.000000000000000000, -0.3656393565653344724, -0.9307566067079450223 ) ) ;
#15516=CARTESIAN_POINT ( 'NONE',  ( 67.90397382975598362, -14.12691053344105541, 28.69135535066940434 ) ) ;
#15517=CARTESIAN_POINT ( 'NONE',  ( 98.29820294268672853, 19.47931871582185792, 5.235283165533769711 ) ) ;
#15519=AXIS2_PLACEMENT_3D ( 'NONE', #6707, #22953, #4865 ) ;
#15520=CARTESIAN_POINT ( 'NONE',  ( 104.1600437297061319, -20.63676802948826960, 8.548029200615774315 ) ) ;
#15521=B_SPLINE_CURVE_WITH_KNOTS ( 'NONE', 3,
 ( #248, #8627, #2381, #22346, #10762, #14742, #4256, #22610, #16607, #22873, #6104, #20877 ),
 .UNSPECIFIED., .F., .F.,
 ( 4, 2, 2, 2, 2, 4 ),
 ( 2.860979249076398407E-17, 0.005971652981263952074, 0.008957479471895872167, 0.01045039271721183091, 0.01119684933986976778, 0.01194330596252770292 ),
 .UNSPECIFIED. ) ;
#15522=CARTESIAN_POINT ( 'NONE',  ( 130.8568914410475088, 40.00000000000002842, 5.949712681206834830 ) ) ;
#15523=CARTESIAN_POINT ( 'NONE',  ( 146.6084372240433993, 1.478241399363601114E-13, -34.62501878078305850 ) ) ;
#15525=CARTESIAN_POINT ( 'NONE',  ( -100.7734535825088500, 22.67402823373189946, 40.00000000000002132 ) ) ;
#15526=CARTESIAN_POINT ( 'NONE',  ( -151.4802930568654062, 16.17241674359067360, -31.86309827670526929 ) ) ;
#15528=CARTESIAN_POINT ( 'NONE',  ( -280.0000000000000568, 19.99999999999996092, 40.00000000000002132 ) ) ;
#15530=CARTESIAN_POINT ( 'NONE',  ( 4.995406935893294431, -15.24977328854832415, -40.00000000000002132 ) ) ;
#15531=CARTESIAN_POINT ( 'NONE',  ( -192.9588430854689989, 14.46834944099965981, 0.000000000000000000 ) ) ;
#15532=CARTESIAN_POINT ( 'NONE',  ( 14.38125909742180220, 40.00000000000017764, -15.17850393972591760 ) ) ;
#15533=CARTESIAN_POINT ( 'NONE',  ( 130.8568914410475088, -39.99999999999992895, -5.949712681207114606 ) ) ;
#15534=CARTESIAN_POINT ( 'NONE',  ( -77.90255099906769942, -20.04994828523962269, 8.644468104261498809 ) ) ;
#15537=CARTESIAN_POINT ( 'NONE',  ( -4.439300432586643197, 46.85201324744569717, -13.79990882516952055 ) ) ;
#15538=CARTESIAN_POINT ( 'NONE',  ( -30.26275506840323004, -41.69427246844629309, 40.00000000000002132 ) ) ;
#15540=CARTESIAN_POINT ( 'NONE',  ( -200.4317933031570078, 44.88237357214676138, -24.83634732651982446 ) ) ;
#15544=AXIS2_PLACEMENT_3D ( 'NONE', #12226, #24876, #24479 ) ;
#15545=CARTESIAN_POINT ( 'NONE',  ( -94.58366989427446470, -20.58370269626843907, 9.000605044545363143 ) ) ;
#15554=CARTESIAN_POINT ( 'NONE',  ( 136.1360204305621266, 3.511608612530704665, 3.511608612530695339 ) ) ;
#15556=CARTESIAN_POINT ( 'NONE',  ( -208.1127848780265026, -9.061048840815752106E-14, 15.00245453012669472 ) ) ;
#15558=CARTESIAN_POINT ( 'NONE',  ( -102.2610585947572872, -2.520905002189730703E-13, 22.27377874548543701 ) ) ;
#15559=EDGE_CURVE ( 'NONE', #23081, #15005, #9155, .T. ) ;
#15562=CARTESIAN_POINT ( 'NONE',  ( -86.96347745069645896, 40.00000000000019895, -18.24025645688310249 ) ) ;
#15563=CARTESIAN_POINT ( 'NONE',  ( -114.7824662269369327, -14.65611376398954135, 16.64100530753757567 ) ) ;
#15564=CARTESIAN_POINT ( 'NONE',  ( -91.56559293963836410, 16.03295912088714203, -16.03295912088699282 ) ) ;
#15565=CARTESIAN_POINT ( 'NONE',  ( -105.3755690713226727, 5.661656051307470077E-14, -21.75974354311649961 ) ) ;
#15566=CARTESIAN_POINT ( 'NONE',  ( -135.8532207217289738, 6.472252184284186249, -6.472252184284142729 ) ) ;
#15567=CARTESIAN_POINT ( 'NONE',  ( 164.1122551457364693, 24.38379312608498850, 10.10009781492419911 ) ) ;
#15568=ADVANCED_FACE ( 'NONE', ( #15273 ), #26092, .T. ) ;
#15570=CARTESIAN_POINT ( 'NONE',  ( 170.2234770963711128, 17.36149277827004411, -17.36149277826983095 ) ) ;
#15571=CARTESIAN_POINT ( 'NONE',  ( -56.48582580120558561, -40.00000000000000000, -9.153146818113723882 ) ) ;
#15572=CARTESIAN_POINT ( 'NONE',  ( -30.26275506840324070, 1.198031551615912571, 57.76657404653985139 ) ) ;
#15573=CARTESIAN_POINT ( 'NONE',  ( -192.9588430854690273, -66.79921049721887982, -10.23066800229569040 ) ) ;
#15575=CARTESIAN_POINT ( 'NONE',  ( -102.2610585947572872, 15.74993999358138907, 15.74993999358168040 ) ) ;
#15577=CARTESIAN_POINT ( 'NONE',  ( 19.06497207195980792, 66.60410523465830579, -10.03556273973354251 ) ) ;
#15578=B_SPLINE_CURVE_WITH_KNOTS ( 'NONE', 3,
 ( #12207, #18319, #4373, #2365, #18593, #14333, #20733, #2501 ),
 .UNSPECIFIED., .F., .F.,
 ( 4, 2, 2, 4 ),
 ( 0.008396560128401207163, 0.01250087472271541912, 0.01455303201987252423, 0.01660518931702962761 ),
 .UNSPECIFIED. ) ;
#15579=CARTESIAN_POINT ( 'NONE',  ( 170.0000000000000000, 19.80854622259149878, -15.47746304364901171 ) ) ;
#15581=ORIENTED_EDGE ( 'NONE', *, *, #25881, .T. ) ;
#15582=CARTESIAN_POINT ( 'NONE',  ( 57.59792236341148453, -40.00000000000003553, 2.435789363417741438 ) ) ;
#15584=CARTESIAN_POINT ( 'NONE',  ( -199.9999999999999432, 14.17215463606722459, -49.28189405767596298 ) ) ;
#15586=ORIENTED_EDGE ( 'NONE', *, *, #14753, .F. ) ;
#15587=CARTESIAN_POINT ( 'NONE',  ( -200.4318156386385965, -44.88237417767405191, -24.83634777281914197 ) ) ;
#15588=CARTESIAN_POINT ( 'NONE',  ( 130.8568914410475088, 40.00000000000002842, 5.949712681206834830 ) ) ;
#15591=CARTESIAN_POINT ( 'NONE',  ( -100.7734535825088500, -40.00000000000009948, 17.32597176626796909 ) ) ;
#15593=CARTESIAN_POINT ( 'NONE',  ( 136.1360204305621266, 1.473277640373554421E-13, -35.03383547441296741 ) ) ;
#15595=CARTESIAN_POINT ( 'NONE',  ( -91.56559293963834989, -16.03295912088728414, 16.03295912088688269 ) ) ;
#15596=CARTESIAN_POINT ( 'NONE',  ( -135.8532207217289738, 6.472252184284583265, -50.09629031063960980 ) ) ;
#15597=CARTESIAN_POINT ( 'NONE',  ( -105.2110227778633202, -21.45666521040888597, 1.366831978263496117 ) ) ;
#15598=CARTESIAN_POINT ( 'NONE',  ( -280.0000000000000000, -2.609240458947769655E-13, 20.00000000000001421 ) ) ;
#15600=CARTESIAN_POINT ( 'NONE',  ( -135.8532207217289738, 9.153146818113548022, 40.00000000000002132 ) ) ;
#15601=CARTESIAN_POINT ( 'NONE',  ( 57.59792236341148453, -37.56421063658185489, -40.00000000000002132 ) ) ;
#15602=CARTESIAN_POINT ( 'NONE',  ( -105.3755690713226727, 15.38646221621793231, -15.38646221621779020 ) ) ;
#15603=CARTESIAN_POINT ( 'NONE',  ( 200.0000000000000000, 20.00000000000013856, -40.00000000000002132 ) ) ;
#15606=CARTESIAN_POINT ( 'NONE',  ( 192.4448373802100889, -1.741373372144848397E-13, 20.00000000003942091 ) ) ;
#15607=CARTESIAN_POINT ( 'NONE',  ( -135.8532207217289738, 50.09629031063965243, -6.472252184284084109 ) ) ;
#15608=CARTESIAN_POINT ( 'NONE',  ( 192.4448373802101173, 19.99999999996063949, 40.00000000000002132 ) ) ;
#15610=EDGE_CURVE ( 'NONE', #12795, #13332, #13897, .T. ) ;
#15611=CARTESIAN_POINT ( 'NONE',  ( 83.06440094986135136, -24.44702070088743540, 9.006081069514475956 ) ) ;
#15613=CARTESIAN_POINT ( 'NONE',  ( 19.06497207195980792, 66.60410523465817789, 10.03556273973446800 ) ) ;
#15614=CARTESIAN_POINT ( 'NONE',  ( -135.8532207217289738, -1.351063376314938213E-13, 30.84685318188645553 ) ) ;
#15615=CARTESIAN_POINT ( 'NONE',  ( -30.26275506840325136, 29.48230279907760121, 27.08623969584625613 ) ) ;
#15617=CARTESIAN_POINT ( 'NONE',  ( -162.0762913951021176, 1.694272876828294194, -40.00000000000002132 ) ) ;
#15620=CARTESIAN_POINT ( 'NONE',  ( 170.0000000000001421, 9.369682556672135121, 22.62041470344889760 ) ) ;
#15621=CARTESIAN_POINT ( 'NONE',  ( 14.38125909742180752, 10.73282306404735387, -10.73282306404708919 ) ) ;
#15622=CARTESIAN_POINT ( 'NONE',  ( 91.82158438592156813, 40.45024623143973486, -16.11829626348390931 ) ) ;
#15623=CARTESIAN_POINT ( 'NONE',  ( 57.59792236341147031, 1.722363176415065089, -1.722363176415036445 ) ) ;
#15624=CARTESIAN_POINT ( 'NONE',  ( -86.95438060894043986, 9.637778285144355195, -19.12135828296647588 ) ) ;
#15625=CARTESIAN_POINT ( 'NONE',  ( 184.8905102610680444, 14.79361573936424890, -41.77492675555986068 ) ) ;
#15626=CARTESIAN_POINT ( 'NONE',  ( 192.4448373802101173, 42.42640687122089815, -14.14213562370272470 ) ) ;
#15627=CARTESIAN_POINT ( 'NONE',  ( 184.8905102610680444, -43.07788698682556827, -13.49065550809859104 ) ) ;
#15628=CARTESIAN_POINT ( 'NONE',  ( 0.2972598230769938343, 10.13633138497486286, -10.13633138497461594 ) ) ;
#15629=CARTESIAN_POINT ( 'NONE',  ( 14.38125909742180752, 15.17850393972634038, 0.000000000000000000 ) ) ;
#15631=CARTESIAN_POINT ( 'NONE',  ( 19.06497207195981858, -40.00000000000007105, 14.19242893257826665 ) ) ;
#15632=CARTESIAN_POINT ( 'NONE',  ( -192.9588430854690273, 18.05360324515418924, 38.51493924976949756 ) ) ;
#15634=CARTESIAN_POINT ( 'NONE',  ( 200.0000000000000000, -20.00000000000006750, 40.00000000000002132 ) ) ;
#15635=ORIENTED_EDGE ( 'NONE', *, *, #20542, .T. ) ;
#15636=CARTESIAN_POINT ( 'NONE',  ( 19.06497207195979726, 38.31983398719629719, -18.24870850772750686 ) ) ;
#15637=CARTESIAN_POINT ( 'NONE',  ( 40.56892791155959088, 37.51946456477319458, 15.54107107570585455 ) ) ;
#15639=CARTESIAN_POINT ( 'NONE',  ( -105.2054292635175869, -1.366713675291838737, 21.49321519473981468 ) ) ;
#15641=CARTESIAN_POINT ( 'NONE',  ( -189.6939181379304955, -43.50327460064440999, 18.01964634722552461 ) ) ;
#15642=B_SPLINE_CURVE_WITH_KNOTS ( 'NONE', 3,
 ( #22318, #9530, #16046, #13917, #25781, #22052, #15639, #1830 ),
 .UNSPECIFIED., .F., .F.,
 ( 4, 2, 2, 4 ),
 ( 0.0002291728420604105022, 0.002290361214547608718, 0.004351549587034806744, 0.008473926332009199328 ),
 .UNSPECIFIED. ) ;
#15644=CARTESIAN_POINT ( 'NONE',  ( 23.39921416754915739, -23.33452606844846500, 42.84940400815675332 ) ) ;
#15645=B_SPLINE_CURVE_WITH_KNOTS ( 'NONE', 3,
 ( #22250, #6271, #24241, #4165, #21979, #2158 ),
 .UNSPECIFIED., .F., .F.,
 ( 4, 2, 4 ),
 ( 7.757919228897728493E-18, 0.004202846899763157743, 0.008405693799526306811 ),
 .UNSPECIFIED. ) ;
#15648=CARTESIAN_POINT ( 'NONE',  ( 27.79909650598017379, 13.47302921524990538, -45.20561170652695893 ) ) ;
#15651=CARTESIAN_POINT ( 'NONE',  ( -87.13361725327071383, 21.49321519333427233, 0.6985161928263129427 ) ) ;
#15652=CARTESIAN_POINT ( 'NONE',  ( -198.0356074513804572, -9.007331120208026888E-14, 15.37879056873070560 ) ) ;
#15655=CARTESIAN_POINT ( 'NONE',  ( -259.2033419157646676, 9.517827891722582478, 40.00000000000002132 ) ) ;
#15657=CARTESIAN_POINT ( 'NONE',  ( 98.29820294268191105, -7.653668647302824368, -18.47759065022797031 ) ) ;
#15658=CARTESIAN_POINT ( 'NONE',  ( -100.7734535825088500, -17.32597176626812185, -40.00000000000002132 ) ) ;
#15659=CARTESIAN_POINT ( 'NONE',  ( 146.6084372240433709, -34.62501878078303008, 40.00000000000002132 ) ) ;
#15660=CARTESIAN_POINT ( 'NONE',  ( 192.4448373802100889, 2.472897170449861688E-13, -19.99999999996060751 ) ) ;
#15661=CARTESIAN_POINT ( 'NONE',  ( -100.7734535825088358, -2.560096224687585342E-13, 22.67402823373191723 ) ) ;
#15662=CARTESIAN_POINT ( 'NONE',  ( 14.38125909742181285, -10.73282306404712472, -10.73282306404731301 ) ) ;
#15663=ORIENTED_EDGE ( 'NONE', *, *, #11565, .T. ) ;
#15665=CARTESIAN_POINT ( 'NONE',  ( -135.8532207217289738, 9.153146818113546246, -0.000000000000000000 ) ) ;
#15666=CARTESIAN_POINT ( 'NONE',  ( -4.039451493210489019, 13.82811171175440812, 46.99046209229809534 ) ) ;
#15667=CARTESIAN_POINT ( 'NONE',  ( -93.01854144616076780, -8.553566904025881712, 20.65013722625350567 ) ) ;
#15671=CARTESIAN_POINT ( 'NONE',  ( -91.56559293963836410, 16.03295912088714203, -16.03295912088699282 ) ) ;
#15674=VERTEX_POINT ( 'NONE', #15747 ) ;
#15675=CARTESIAN_POINT ( 'NONE',  ( -30.26275506840324425, 1.694272468446254232, -40.00000000000002132 ) ) ;
#15676=CARTESIAN_POINT ( 'NONE',  ( -100.0957100000493512, -20.56213589465292912, 8.517115558914053253 ) ) ;
#15680=CARTESIAN_POINT ( 'NONE',  ( 192.4448373802101173, 42.42640687116508502, -14.14213562375874567 ) ) ;
#15682=CARTESIAN_POINT ( 'NONE',  ( -86.96347745069644475, 5.999880687339585546E-14, -21.75974354311649961 ) ) ;
#15683=CARTESIAN_POINT ( 'NONE',  ( 22.27434459963462388, -13.86259002493217096, 47.22399357567389444 ) ) ;
#15686=CARTESIAN_POINT ( 'NONE',  ( 91.82158438592158234, -1.633484621919921769E-13, 17.20528682183300262 ) ) ;
#15687=CARTESIAN_POINT ( 'NONE',  ( -238.4067589809705794, -3.369206980223063916E-14, -0.9644942799825824142 ) ) ;
#15688=CARTESIAN_POINT ( 'NONE',  ( -199.9999999999999716, -47.95319408140863260, -15.63350978565342153 ) ) ;
#15689=CARTESIAN_POINT ( 'NONE',  ( -213.1075012329537230, -9.698598906450557777, 9.698598906450415669 ) ) ;
#15690=CARTESIAN_POINT ( 'NONE',  ( 163.1118516004056573, 1.251511021549353291E-13, -27.26290988616872824 ) ) ;
#15691=CARTESIAN_POINT ( 'NONE',  ( 136.1360204305621266, -3.511608612530379592, -53.05693388239318153 ) ) ;
#15692=CARTESIAN_POINT ( 'NONE',  ( -97.72675010090215153, 8.185591577777120875, 20.89622088363376307 ) ) ;
#15694=CARTESIAN_POINT ( 'NONE',  ( -77.59212294118380271, 13.55867551896204937, -17.46520578609249696 ) ) ;
#15695=CARTESIAN_POINT ( 'NONE',  ( 19.06497207195979726, 40.00000000000017053, -14.19242893257798599 ) ) ;
#15696=CARTESIAN_POINT ( 'NONE',  ( -238.4067589809705794, -40.00000000000021316, 40.96449427990166470 ) ) ;
#15697=CARTESIAN_POINT ( 'NONE',  ( 163.1118516004056573, -19.27778845539233998, 37.29075403953149959 ) ) ;
#15698=CARTESIAN_POINT ( 'NONE',  ( -198.0356074513804572, -10.87444709759714634, -10.87444709759729911 ) ) ;
#15700=CARTESIAN_POINT ( 'NONE',  ( -100.7734535825088500, -12.25131212657462498, -44.31723036834905827 ) ) ;
#15702=CARTESIAN_POINT ( 'NONE',  ( 184.8905102610680444, 13.49065550809826952, -13.49065550809790359 ) ) ;
#15705=CARTESIAN_POINT ( 'NONE',  ( -30.26275506840324070, 1.198031551616724366, -57.76657404653984429 ) ) ;
#15706=CARTESIAN_POINT ( 'NONE',  ( -82.28159816621803202, 6.254964767126788949, 19.22531893665605196 ) ) ;
#15710=CARTESIAN_POINT ( 'NONE',  ( -24.88648382749770605, 12.31763033300769195, 39.69105101992045093 ) ) ;
#15711=ORIENTED_EDGE ( 'NONE', *, *, #18093, .T. ) ;
#15713=CARTESIAN_POINT ( 'NONE',  ( -30.26275506840324425, 41.69427246844628598, -40.00000000000002132 ) ) ;
#15714=CARTESIAN_POINT ( 'NONE',  ( -208.1127848780265026, -10.60833733269551971, 10.60833733269537049 ) ) ;
#15715=CARTESIAN_POINT ( 'NONE',  ( -192.9588430854690273, 39.99999999999980105, 54.46834944098235809 ) ) ;
#15716=CARTESIAN_POINT ( 'NONE',  ( -86.86493150571119770, -19.60045294882755584, -8.366608963954130118 ) ) ;
#15720=SHAPE_REPRESENTATION ( 'Stator', ( #21058 ), #17620 ) ;
#15721=CARTESIAN_POINT ( 'NONE',  ( -238.4067589809705794, 39.99999999999999289, -0.9644942799821634161 ) ) ;
#15723=CARTESIAN_POINT ( 'NONE',  ( 170.2234770963711128, 40.00000000000014211, -24.55285855007172913 ) ) ;
#15724=CARTESIAN_POINT ( 'NONE',  ( -149.5198336001615189, 31.65188091022390893, 13.11063834760882152 ) ) ;
#15725=CARTESIAN_POINT ( 'NONE',  ( -0.5869797817569126774, -18.21245090263647981, -43.96874597320456957 ) ) ;
#15726=CARTESIAN_POINT ( 'NONE',  ( -198.0356074513804572, 17.40982414986501325, -39.15871834505897198 ) ) ;
#15728=CARTESIAN_POINT ( 'NONE',  ( -208.1127848780264742, -39.99999999999990763, -15.00245453012711394 ) ) ;
#15729=CARTESIAN_POINT ( 'NONE',  ( -105.4741150117382773, -19.77569912955116749, -7.943527260750395946 ) ) ;
#15730=CARTESIAN_POINT ( 'NONE',  ( -86.96347745069645896, 21.75974354311648895, 40.00000000000002132 ) ) ;
#15731=CARTESIAN_POINT ( 'NONE',  ( 4.995406935893294431, -15.24977328854832415, -40.00000000000002132 ) ) ;
#15732=CARTESIAN_POINT ( 'NONE',  ( 184.8905102610680444, 43.07788698682572459, 13.49065550809829439 ) ) ;
#15733=CARTESIAN_POINT ( 'NONE',  ( 136.1360204305621266, 35.03383547441298163, -40.00000000000002132 ) ) ;
#15734=CARTESIAN_POINT ( 'NONE',  ( -105.4741150117389168, 7.943527260764259523, 19.77569912954497866 ) ) ;
#15735=CARTESIAN_POINT ( 'NONE',  ( 146.6084372240433993, -3.357462877844280890E-13, 34.62501878078305850 ) ) ;
#15736=CARTESIAN_POINT ( 'NONE',  ( 91.82158438592158234, 44.40256751092336884, -12.16597498400043342 ) ) ;
#15737=CARTESIAN_POINT ( 'NONE',  ( 14.38125909742180752, 55.17850393972636880, 2.449293598294708485E-15 ) ) ;
#15739=CARTESIAN_POINT ( 'NONE',  ( 98.29820294267354086, -18.47759065023112157, 7.653668647303947914 ) ) ;
#15740=CARTESIAN_POINT ( 'NONE',  ( 57.59792236341147031, 26.56190807104693619, -30.00663442387692115 ) ) ;
#15741=CARTESIAN_POINT ( 'NONE',  ( -280.0000000000000000, -1.237140859393462838E-13, 20.00000000000001421 ) ) ;
#15742=CARTESIAN_POINT ( 'NONE',  ( -198.0356074513804572, 39.15871834505887250, 17.40982414986519089 ) ) ;
#15743=CARTESIAN_POINT ( 'NONE',  ( 130.8568914410475372, -3.326198072800416995E-13, 34.05028731879788495 ) ) ;
#15745=CARTESIAN_POINT ( 'NONE',  ( -198.0356074513804572, 15.37879056873067007, 0.000000000000000000 ) ) ;
#15747=CARTESIAN_POINT ( 'NONE',  ( -87.13361725327075646, -15.19799821270861706, 15.19799821270823159 ) ) ;
#15749=CARTESIAN_POINT ( 'NONE',  ( -87.08883489506207809, 3.402281996148261101, -21.20173182216571917 ) ) ;
#15750=CARTESIAN_POINT ( 'NONE',  ( 136.1360204305621266, -24.77266263493151044, 24.77266263493093135 ) ) ;
#15751=CARTESIAN_POINT ( 'NONE',  ( 57.59792236341148453, 1.722363176415528940, -54.84617931850878136 ) ) ;
#15752=CARTESIAN_POINT ( 'NONE',  ( -77.55640685876511498, -22.13135000837103661, -4.964495286674871776E-15 ) ) ;
#15753=CARTESIAN_POINT ( 'NONE',  ( -87.13348102036110276, 16.17099723932746258, -14.22374190074556033 ) ) ;
#15754=CARTESIAN_POINT ( 'NONE',  ( -259.2033419157646676, -21.55415060305824326, -21.55415060305857367 ) ) ;
#15755=CARTESIAN_POINT ( 'NONE',  ( -30.26275506840322649, -29.48230279907769358, -29.48230279907820162 ) ) ;
#15756=CARTESIAN_POINT ( 'NONE',  ( -162.0762913951021176, -27.08623940707584055, -29.48230308784799547 ) ) ;
#15757=CARTESIAN_POINT ( 'NONE',  ( 192.4448373802101173, -14.14213562375826605, -42.42640687116518450 ) ) ;
#15758=CARTESIAN_POINT ( 'NONE',  ( -114.7826396787322665, 2.171560191748074081E-13, -22.13135001986799111 ) ) ;
#15761=CARTESIAN_POINT ( 'NONE',  ( 130.8568914410475088, -40.00000000000001421, 5.949712681206549725 ) ) ;
#15762=CARTESIAN_POINT ( 'NONE',  ( -259.2033419157646676, 6.730120644403214669, 49.83842185052034068 ) ) ;
#15765=CARTESIAN_POINT ( 'NONE',  ( -208.1127848780264742, 15.00245453012665742, 40.00000000000002132 ) ) ;
#15766=VERTEX_POINT ( 'NONE', #17748 ) ;
#15767=CARTESIAN_POINT ( 'NONE',  ( -208.1127848780264742, 38.89260858015732936, -17.67593391476642140 ) ) ;
#15768=CARTESIAN_POINT ( 'NONE',  ( 91.16600911855444167, 21.07464282850845905, 8.729402881737186704 ) ) ;
#15769=CARTESIAN_POINT ( 'NONE',  ( 22.86726691379304199, 17.87269271907674195, 43.14849715852160728 ) ) ;
#15770=CARTESIAN_POINT ( 'NONE',  ( -30.26275506840324425, 1.694272468446254232, 40.00000000000002132 ) ) ;
#15772=CARTESIAN_POINT ( 'NONE',  ( -192.9370391625990919, -44.11033075278038496, 24.26711063095388710 ) ) ;
#15774=CARTESIAN_POINT ( 'NONE',  ( -1.624577210500880220, -18.12534649861199654, 43.75845733969866558 ) ) ;
#15775=CARTESIAN_POINT ( 'NONE',  ( 22.33254948916862404, 17.93222939140627403, -43.29223140031697170 ) ) ;
#15778=CARTESIAN_POINT ( 'NONE',  ( 126.3230993689412855, -28.30579214049056347, 11.72464299830478218 ) ) ;
#15779=SPHERICAL_SURFACE ( 'NONE', #23324, 15.00000000000000000 ) ;
#15782=CARTESIAN_POINT ( 'NONE',  ( -162.0762913951020892, 1.198031840456041497, -57.76657433537918251 ) ) ;
#15783=CARTESIAN_POINT ( 'NONE',  ( -105.3755690713226585, 21.75974354311648185, 40.00000000000002132 ) ) ;
#15784=CARTESIAN_POINT ( 'NONE',  ( -151.7004448982690974, 13.46262099571027981, -32.50164219281900557 ) ) ;
#15787=CARTESIAN_POINT ( 'NONE',  ( -213.1075012329537230, 9.698598906450543566, -9.698598906450348167 ) ) ;
#15788=CARTESIAN_POINT ( 'NONE',  ( 146.6084372240433709, 34.62501878078307982, -40.00000000000002132 ) ) ;
#15789=CARTESIAN_POINT ( 'NONE',  ( -208.1127848780264742, 55.00245453014418473, 40.00000000000002132 ) ) ;
#15790=CARTESIAN_POINT ( 'NONE',  ( 184.8905102610680444, 2.362515690532070066E-13, -19.07866798485558490 ) ) ;
#15791=CARTESIAN_POINT ( 'NONE',  ( 170.2234770963711128, -2.259079968736224833E-13, 24.55285855007187124 ) ) ;
#15792=CARTESIAN_POINT ( 'NONE',  ( -192.9588430854690273, 18.05360324515473280, -38.51493924976924177 ) ) ;
#15797=CARTESIAN_POINT ( 'NONE',  ( -86.96347745069645896, 21.75974354311648895, -0.000000000000000000 ) ) ;
#15799=CARTESIAN_POINT ( 'NONE',  ( -103.9663809734266806, -8.574562934117741619, 19.92521373309844535 ) ) ;
#15802=CARTESIAN_POINT ( 'NONE',  ( 130.8568914410475088, -4.207082182989324792, -52.36146031193423056 ) ) ;
#15803=CARTESIAN_POINT ( 'NONE',  ( 27.79909650603157090, -45.20561170655300032, -13.47302921519561991 ) ) ;
#15805=CARTESIAN_POINT ( 'NONE',  ( -192.9588430854690273, 14.46834944099966336, -40.00000000000002132 ) ) ;
#15806=CARTESIAN_POINT ( 'NONE',  ( -86.86493150571010347, -19.60045294882735334, 8.366608963953911626 ) ) ;
#15807=EDGE_LOOP ( 'NONE', ( #1210, #25880, #25433, #4260, #7962, #9442 ) ) ;
#15810=CARTESIAN_POINT ( 'NONE',  ( -135.8532207217289738, 21.81201906317767936, 21.81201906317778239 ) ) ;
#15811=FACE_OUTER_BOUND ( 'NONE', #12395, .T. ) ;
#15812=CARTESIAN_POINT ( 'NONE',  ( 192.4448373802100889, 1.051811698935164031E-13, -20.00000000003942091 ) ) ;
#15813=CARTESIAN_POINT ( 'NONE',  ( -86.96347745069644475, -21.75974354311652093, 40.00000000000002132 ) ) ;
#15817=CARTESIAN_POINT ( 'NONE',  ( 91.82158438592159655, -39.99999999999976552, -22.79471317813512599 ) ) ;
#15818=CARTESIAN_POINT ( 'NONE',  ( -110.1003821002711760, -15.15067674037973688, 13.36729751626187301 ) ) ;
#15819=CARTESIAN_POINT ( 'NONE',  ( 130.8568914410475372, -4.207082182992846420, 4.207082182992822439 ) ) ;
#15820=CARTESIAN_POINT ( 'NONE',  ( 163.1118516004056573, 27.26290988616875310, 0.000000000000000000 ) ) ;
#15821=CARTESIAN_POINT ( 'NONE',  ( 170.2234770963711128, -10.92277846919171935, -45.64576402573189995 ) ) ;
#15823=CARTESIAN_POINT ( 'NONE',  ( -3.071327051952942089, -47.32824404903815463, 13.87830843099601275 ) ) ;
#15824=CARTESIAN_POINT ( 'NONE',  ( -135.8532207217289738, -1.208299557080134822E-13, 9.153146818113572891 ) ) ;
#15825=CARTESIAN_POINT ( 'NONE',  ( -280.0000000000000568, -40.00000000000000000, -20.00000000000015277 ) ) ;
#15826=CARTESIAN_POINT ( 'NONE',  ( -238.4067589809705794, 28.96627169325324758, -27.60227080167054581 ) ) ;
#15827=CARTESIAN_POINT ( 'NONE',  ( -114.7844311315812149, 14.74981244961873728, 16.56244415773397805 ) ) ;
#15828=CARTESIAN_POINT ( 'NONE',  ( -197.6433718612336747, -18.53520099267758425, -44.74793361791282820 ) ) ;
#15829=CARTESIAN_POINT ( 'NONE',  ( 151.7948205124836250, 23.49921654116361225, -23.49921654116333514 ) ) ;
#15831=CARTESIAN_POINT ( 'NONE',  ( 57.59792236341147031, -1.722363176415055985, 1.722363176415024677 ) ) ;
#15832=CARTESIAN_POINT ( 'NONE',  ( 170.2234770963711128, 45.64576402573181468, 10.92277846919223627 ) ) ;
#15833=CARTESIAN_POINT ( 'NONE',  ( 4.995406935893294431, -15.24977328854832415, -40.00000000000002132 ) ) ;
#15835=CARTESIAN_POINT ( 'NONE',  ( 130.8568914410475088, -52.36146031193413108, -4.207082182990267150 ) ) ;
#15837=CARTESIAN_POINT ( 'NONE',  ( -77.56353172722820943, 1.385506815401374769, 22.09247646618768712 ) ) ;
#15839=CARTESIAN_POINT ( 'NONE',  ( 0.2972598230770030492, -39.99999999999987210, -14.33493731733975451 ) ) ;
#15841=CARTESIAN_POINT ( 'NONE',  ( -5.304449574951913604, 17.72890873421401992, 42.80137191221402304 ) ) ;
#15843=VERTEX_POINT ( 'NONE', #11498 ) ;
#15844=CARTESIAN_POINT ( 'NONE',  ( -192.9588430854690273, 54.46834944098218756, -40.00000000000002132 ) ) ;
#15845=CARTESIAN_POINT ( 'NONE',  ( -198.9233928134952976, -49.24835219437316169, -14.16707757978289806 ) ) ;
#15846=CARTESIAN_POINT ( 'NONE',  ( 0.2972598230769883387, 39.99999999999997158, 14.33493731733947563 ) ) ;
#15847=CARTESIAN_POINT ( 'NONE',  ( -83.21262154144231715, -33.12752917117752105, 13.72187187063024183 ) ) ;
#15849=CARTESIAN_POINT ( 'NONE',  ( -135.8532207217289738, -1.208299557080134822E-13, 9.153146818113572891 ) ) ;
#15853=CARTESIAN_POINT ( 'NONE',  ( -3.615356597029639296, -17.91804473398299535, -43.25798660799100048 ) ) ;
#15854=B_SPLINE_CURVE_WITH_KNOTS ( 'NONE', 3,
 ( #15007, #5170, #11390, #23011, #13274, #4911, #21396, #23268, #21520, #4786, #3294, #19264 ),
 .UNSPECIFIED., .F., .F.,
 ( 4, 2, 2, 2, 2, 4 ),
 ( 5.597004042492164534E-17, 0.004680202113614274732, 0.009360404227228492219, 0.01170050528403562135, 0.01404060634084275221, 0.01872080845445705383 ),
 .UNSPECIFIED. ) ;
#15855=CARTESIAN_POINT ( 'NONE',  ( 130.8568914410475088, -32.49135343045495006, 24.07718906446878648 ) ) ;
#15856=CARTESIAN_POINT ( 'NONE',  ( 160.7895100361087088, -20.14405787076046295, 20.14405787076000465 ) ) ;
#15857=CARTESIAN_POINT ( 'NONE',  ( -56.48582580120559982, -21.81201906317755501, -34.75652343174621706 ) ) ;
#15858=CARTESIAN_POINT ( 'NONE',  ( 192.4448373802101173, -40.00000000000019185, 20.00000000003900524 ) ) ;
#15861=CARTESIAN_POINT ( 'NONE',  ( -56.48582580120558561, -30.84685318188645908, 40.00000000000002132 ) ) ;
#15862=CARTESIAN_POINT ( 'NONE',  ( 192.4448373802101173, 14.14213562375862665, 42.42640687116509213 ) ) ;
#15863=CARTESIAN_POINT ( 'NONE',  ( 91.82158438592159655, -22.79471317813468545, -2.449293598294708485E-15 ) ) ;
#15864=CARTESIAN_POINT ( 'NONE',  ( 18.90082831370066785, -43.99399836018038457, -24.18116416851802342 ) ) ;
#15865=EDGE_CURVE ( 'NONE', #6051, #12893, #12564, .T. ) ;
#15866=CARTESIAN_POINT ( 'NONE',  ( -114.4364955367327354, 8.064892380842190178, 20.29001642038852182 ) ) ;
#15867=CARTESIAN_POINT ( 'NONE',  ( -259.2033419157646676, 21.55415060305830366, 21.55415060305842800 ) ) ;
#15868=CARTESIAN_POINT ( 'NONE',  ( 130.8568914410475088, -34.05028731879786363, -40.00000000000002132 ) ) ;
#15870=CARTESIAN_POINT ( 'NONE',  ( 98.29820294267354086, -18.47759065023111447, 7.653668647303970118 ) ) ;
#15871=CARTESIAN_POINT ( 'NONE',  ( -199.9999999999998863, -44.86878812508856385, -24.82633483071075986 ) ) ;
#15872=( BOUNDED_CURVE ( )  B_SPLINE_CURVE ( 3, ( #14541, #22138, #2440, #6819 ),
 .UNSPECIFIED., .F., .T. ) 
 B_SPLINE_CURVE_WITH_KNOTS ( ( 4, 4 ),
 ( 0.007854122480158971450, 0.01576650722537254259 ),
 .UNSPECIFIED. ) 
 CURVE ( )  GEOMETRIC_REPRESENTATION_ITEM ( )  RATIONAL_B_SPLINE_CURVE ( ( 0.9999999999999523714, 0.8893928793063825555, 0.7971366613349984975, 0.7232313460858235121 ) ) 
 REPRESENTATION_ITEM ( '' )  );
#15873=CARTESIAN_POINT ( 'NONE',  ( 136.1360204305621551, 31.79587985999267374, -24.77266263493117293 ) ) ;
#15874=CARTESIAN_POINT ( 'NONE',  ( 184.8905102610680444, -40.00000000000005684, 19.07866798485543569 ) ) ;
#15876=CARTESIAN_POINT ( 'NONE',  ( -83.21262154144254453, -13.72187187061479108, 33.12752917118424989 ) ) ;
#15877=EDGE_CURVE ( 'NONE', #3931, #23238, #25092, .T. ) ;
#15878=CARTESIAN_POINT ( 'NONE',  ( -192.9588430854689989, 14.46834944099965981, 0.000000000000000000 ) ) ;
#15884=CARTESIAN_POINT ( 'NONE',  ( -213.1075012329537230, 66.26714140138673770, -9.698598906462034819 ) ) ;
#15885=CARTESIAN_POINT ( 'NONE',  ( 151.7948205124836534, 23.49921654116056047, -33.06932595376338213 ) ) ;
#15886=CARTESIAN_POINT ( 'NONE',  ( 190.0000000000000000, 7.164183775012018789E-14, 0.000000000000000000 ) ) ;
#15887=CARTESIAN_POINT ( 'NONE',  ( -82.23724611275160612, 13.84097227486004655, -14.71983334135863508 ) ) ;
#15888=CARTESIAN_POINT ( 'NONE',  ( 4.995406935893287326, 17.50105314357225694, -39.06748935135176026 ) ) ;
#15889=CARTESIAN_POINT ( 'NONE',  ( 151.7948205124836250, -4.785054706301600902, -4.785054706301715477 ) ) ;
#15890=CARTESIAN_POINT ( 'NONE',  ( -86.96347745069644475, -15.38646221621807442, 15.38646221621768184 ) ) ;
#15891=CARTESIAN_POINT ( 'NONE',  ( 19.06497207195980792, -18.24870850772710540, -38.31983398719647482 ) ) ;
#15892=CARTESIAN_POINT ( 'NONE',  ( -162.0762913951020892, -1.198031840385783919, 1.198031840385741731 ) ) ;
#15894=EDGE_CURVE ( 'NONE', #9227, #19209, #18334, .T. ) ;
#15896=CARTESIAN_POINT ( 'NONE',  ( -259.2033419157646676, -40.00000000000017764, 30.48217210827725054 ) ) ;
#15897=CARTESIAN_POINT ( 'NONE',  ( 4.995406935893287326, 17.50105314357170627, 39.06748935135200895 ) ) ;
#15898=CARTESIAN_POINT ( 'NONE',  ( 91.82158438592158234, 12.16597498397756993, 12.16597498397776356 ) ) ;
#15899=CARTESIAN_POINT ( 'NONE',  ( 146.6084372240433709, 5.374981219216996564, 40.00000000000002132 ) ) ;
#15900=ORIENTED_EDGE ( 'NONE', *, *, #6614, .T. ) ;
#15901=CARTESIAN_POINT ( 'NONE',  ( 130.8568914410475088, 4.207082182989741348, -52.36146031193420924 ) ) ;
#15902=CARTESIAN_POINT ( 'NONE',  ( 31.39166500904787327, 40.05004873988723801, 16.58927336176482470 ) ) ;
#15903=CARTESIAN_POINT ( 'NONE',  ( 27.00968939610489983, 17.38581019149919626, 41.97305875713701084 ) ) ;
#15904=CARTESIAN_POINT ( 'NONE',  ( -208.1127848780265026, 15.00245453012665564, 0.000000000000000000 ) ) ;
#15905=ORIENTED_EDGE ( 'NONE', *, *, #16629, .F. ) ;
#15906=CARTESIAN_POINT ( 'NONE',  ( -198.9234529669416816, -44.84148137680988810, 24.80620787426756735 ) ) ;
#15908=CARTESIAN_POINT ( 'NONE',  ( 20.16956056500655237, -13.95858718337597892, 47.86583268170348759 ) ) ;
#15909=B_SPLINE_CURVE_WITH_KNOTS ( 'NONE', 3,
 ( #2689, #11053, #10795, #949, #25169, #23168, #6920, #1072 ),
 .UNSPECIFIED., .F., .F.,
 ( 4, 2, 2, 4 ),
 ( 0.008396858476694638723, 0.01250098582284328574, 0.01455304949591760752, 0.01660511316899192930 ),
 .UNSPECIFIED. ) ;
#15910=CARTESIAN_POINT ( 'NONE',  ( 27.26078259662905268, 17.35591035711511410, -41.90087417141796777 ) ) ;
#15913=CARTESIAN_POINT ( 'NONE',  ( -129.2920262388371668, -10.46331600586649202, 25.26067940862601091 ) ) ;
#15914=CARTESIAN_POINT ( 'NONE',  ( 4.995406935893290878, 39.06748935135239265, -39.06748935135144762 ) ) ;
#15915=CARTESIAN_POINT ( 'NONE',  ( 136.1360204305621266, 35.03383547441298163, 40.00000000000002132 ) ) ;
#15919=CARTESIAN_POINT ( 'NONE',  ( 19.06497207195979726, 38.31983398719604139, 18.24870850772803976 ) ) ;
#15920=CARTESIAN_POINT ( 'NONE',  ( 14.38125909742181285, -15.17850393972633505, 0.000000000000000000 ) ) ;
#15921=CARTESIAN_POINT ( 'NONE',  ( -86.96347745069643054, -18.24025645688353947, -40.00000000000002132 ) ) ;
#15922=CARTESIAN_POINT ( 'NONE',  ( 136.1360204305621551, -35.03383547441293899, 40.00000000000002132 ) ) ;
#15923=CARTESIAN_POINT ( 'NONE',  ( 163.1118516004056573, 40.00000000000017764, -12.73709011382432976 ) ) ;
#15924=CARTESIAN_POINT ( 'NONE',  ( -280.0000000000000000, -2.609240458947769655E-13, 20.00000000000001421 ) ) ;
#15925=CARTESIAN_POINT ( 'NONE',  ( -213.1075012329537230, -9.698598906450422774, -9.698598906450550672 ) ) ;
#15927=CARTESIAN_POINT ( 'NONE',  ( -87.01701082927733921, 20.73853774319881538, -5.374668562258758442 ) ) ;
#15928=CARTESIAN_POINT ( 'NONE',  ( -259.2033419157646676, 9.517827891722584255, -0.000000000000000000 ) ) ;
#15933=CARTESIAN_POINT ( 'NONE',  ( 184.8905102610680444, 14.79361573936396113, -14.79361573936377461 ) ) ;
#15934=CARTESIAN_POINT ( 'NONE',  ( 23.39921416754913253, -42.84940400815667516, -23.33452606844848631 ) ) ;
#15936=CARTESIAN_POINT ( 'NONE',  ( -91.56559293963834989, -22.67402823373193499, -40.00000000000002132 ) ) ;
#15937=CARTESIAN_POINT ( 'NONE',  ( -103.9663809733227282, -20.15238534249515823, 8.026122153668060477 ) ) ;
#15939=EDGE_LOOP ( 'NONE', ( #15905, #9961, #5778, #864 ) ) ;
#15943=CARTESIAN_POINT ( 'NONE',  ( 169.9999999999999432, 19.80854622259133890, 15.47746304364925685 ) ) ;
#15944=CARTESIAN_POINT ( 'NONE',  ( 91.82158438592158234, -12.16597498397761967, -12.16597498397768007 ) ) ;
#15946=CARTESIAN_POINT ( 'NONE',  ( -183.1091233172528234, -45.18843800008796308, -13.45963571008054238 ) ) ;
#15947=CARTESIAN_POINT ( 'NONE',  ( -105.3755690713226585, -40.00000000000010658, 18.24025645688337249 ) ) ;
#15948=CARTESIAN_POINT ( 'NONE',  ( -208.1127848780264742, 15.00245453012665742, 40.00000000000002132 ) ) ;
#15952=EDGE_CURVE ( 'NONE', #19812, #4726, #5824, .T. ) ;
#15955=CARTESIAN_POINT ( 'NONE',  ( -280.0000000000000568, -40.00000000000000000, -20.00000000000015277 ) ) ;
#15957=CARTESIAN_POINT ( 'NONE',  ( -192.9588430854690273, -39.99999999999991473, -14.46834944100011633 ) ) ;
#15959=CARTESIAN_POINT ( 'NONE',  ( -200.0000000000000000, -46.41341197396108953, -18.14835560307970397 ) ) ;
#15960=CARTESIAN_POINT ( 'NONE',  ( 4.995406935893305977, -39.06748935135212264, 39.06748935135171763 ) ) ;
#15961=CARTESIAN_POINT ( 'NONE',  ( 146.6084372240433709, 34.62501878078307982, -40.00000000000002132 ) ) ;
#15962=CARTESIAN_POINT ( 'NONE',  ( 4.995406935893297984, -39.06748935135182421, -17.50105314357212549 ) ) ;
#15965=CARTESIAN_POINT ( 'NONE',  ( -259.2033419157646676, 39.99999999999987921, 9.517827891723049660 ) ) ;
#15966=CARTESIAN_POINT ( 'NONE',  ( 163.1118516004056573, -39.99999999999990052, -27.26290988616886679 ) ) ;
#15967=CARTESIAN_POINT ( 'NONE',  ( 170.2234770963711128, 39.20704971665398375, -17.36149277826984871 ) ) ;
#15968=CARTESIAN_POINT ( 'NONE',  ( -56.48582580120559271, 6.472252184284121412, 6.472252184284244869 ) ) ;
#15969=CARTESIAN_POINT ( 'NONE',  ( -192.1964066537985332, -14.00508515768846252, -48.17614796926347509 ) ) ;
#15970=CARTESIAN_POINT ( 'NONE',  ( 19.06497207195981147, -10.03556273973439517, 10.03556273973429214 ) ) ;
#15971=VERTEX_POINT ( 'NONE', #23875 ) ;
#15972=CARTESIAN_POINT ( 'NONE',  ( -208.1127848780265026, 10.60833733269551615, -10.60833733269529766 ) ) ;
#15973=CARTESIAN_POINT ( 'NONE',  ( 4.995406935893287326, 17.50105314357170627, 39.06748935135200895 ) ) ;
#15975=CARTESIAN_POINT ( 'NONE',  ( 48.46027384457359943, 18.19770403991907415, 35.02097776273673446 ) ) ;
#15976=CARTESIAN_POINT ( 'NONE',  ( -91.56559293963834989, -16.03295912088659492, -40.53558337403696044 ) ) ;
#15977=DIRECTION ( 'NONE',  ( 1.000000000000000000, 0.000000000000000000, 0.000000000000000000 ) ) ;
#15978=CARTESIAN_POINT ( 'NONE',  ( -82.25136756410482519, 3.474794711389625146, 19.89060514491995590 ) ) ;
#15979=ORIENTED_EDGE ( 'NONE', *, *, #25230, .T. ) ;
#15982=CARTESIAN_POINT ( 'NONE',  ( -5.152948516938707257, 23.23217004669232111, 42.67688069069163248 ) ) ;
#15985=EDGE_LOOP ( 'NONE', ( #13724, #8971, #10354, #25685, #10669 ) ) ;
#15986=CARTESIAN_POINT ( 'NONE',  ( -280.0000000000000000, -14.14213562373098831, -14.14213562373098654 ) ) ;
#15988=CARTESIAN_POINT ( 'NONE',  ( -110.0574180503309805, 6.256710540492572470, 19.22461201371535822 ) ) ;
#15989=CARTESIAN_POINT ( 'NONE',  ( -114.6379801953813455, -18.98756686744332001, -11.20591363448406597 ) ) ;
#15991=EDGE_CURVE ( 'NONE', #21267, #19077, #25656, .T. ) ;
#15993=CARTESIAN_POINT ( 'NONE',  ( 192.4448373802100889, -1.741373372144848397E-13, 20.00000000003942091 ) ) ;
#15995=( BOUNDED_SURFACE ( )  B_SPLINE_SURFACE ( 3, 2, ( 
 ( #19040, #21171, #6394 ),
 ( #23169, #11054, #16906 ),
 ( #14635, #8661, #6658 ),
 ( #12510, #13053, #14903 ),
 ( #16769, #20638, #12784 ),
 ( #2414, #20911, #18906 ),
 ( #23043, #4818, #8525 ),
 ( #4416, #21037, #8389 ),
 ( #2820, #10929, #819 ),
 ( #8926, #17035, #25170 ),
 ( #6921, #15038, #2944 ),
 ( #16511, #24637, #10523 ),
 ( #18637, #13178, #23296 ),
 ( #16039, #5072, #950 ),
 ( #7301, #15171, #15537 ),
 ( #9307, #11420, #1326 ),
 ( #26184, #3192, #7922 ),
 ( #15415, #17163, #21299 ),
 ( #24165, #23541, #5312 ),
 ( #9182, #11544, #17413 ),
 ( #1204, #15291, #25553 ),
 ( #11301, #19540, #13423 ),
 ( #9431, #5940, #9058 ),
 ( #3448, #3074, #7174 ),
 ( #17538, #23421, #5445 ),
 ( #7422, #14048, #23665 ),
 ( #21546, #19668, #1455 ),
 ( #13546, #3320, #18032 ),
 ( #7056, #21674, #25297 ),
 ( #22182, #11175, #25676 ),
 ( #12053, #19418, #9926 ),
 ( #3955, #5196, #19290 ),
 ( #1073, #17295, #25427 ),
 ( #13299, #21420, #20443 ),
 ( #16575, #26315, #6202 ),
 ( #213, #12583, #22705 ),
 ( #24706, #2088, #18438 ),
 ( #18168, #10062, #24310 ),
 ( #8058, #16705, #20712 ),
 ( #22842, #14313, #2221 ),
 ( #1956, #12447, #24434 ),
 ( #14576, #10195, #6076 ),
 ( #2478, #4481, #10329 ),
 ( #6461, #16174, #22447 ),
 ( #8323, #10590, #18705 ),
 ( #18298, #16447, #4090 ),
 ( #488, #6588, #14178 ),
 ( #8595, #4617, #20575 ),
 ( #85, #4227, #24571 ),
 ( #22313, #24837, #2347 ),
 ( #12316, #12189, #20311 ),
 ( #14710, #8194, #6327 ),
 ( #20173, #16310, #14449 ),
 ( #22576, #4355, #10460 ),
 ( #18572, #352, #8456 ),
 ( #24976, #619, #12713 ),
 ( #16843, #22970, #2616 ),
 ( #18841, #20841, #14837 ),
 ( #8725, #10730, #6725 ),
 ( #8844, #333, #2736 ),
 ( #8574, #18685, #6442 ),
 ( #24684, #2460, #2599 ) ),
 .UNSPECIFIED., .F., .F., .T. ) 
 B_SPLINE_SURFACE_WITH_KNOTS ( ( 4, 2, 2, 2, 2, 2, 2, 2, 2, 2, 2, 2, 2, 2, 2, 2, 2, 2, 2, 2, 2, 2, 2, 2, 2, 2, 2, 2, 2, 2, 4 ),
 ( 3, 3 ),
 ( 0.005118828937694740178, 0.02956064127319283155, 0.05400245360869092293, 0.07844426594418901777, 0.08149949248612628483, 0.08302710575709490448, 0.08379091239257921431, 0.08417281571032136922, 0.08436376736919246055, 0.08445924319862799234, 0.08450698111334575824, 0.08455471902806353801, 0.09066517211193805825, 0.09677562519581259237, 0.09983085173774985943, 0.1028860782796871126, 0.1089965313635616329, 0.1151069844474361670, 0.1181622109893734340, 0.1196898242603420537, 0.1204536308958263635, 0.1208355342135685184, 0.1208594031709274014, 0.1208832721282862843, 0.1209310100430040641, 0.1210264858724396098, 0.1212174375313106872, 0.1273278906151852075, 0.1517697029506832884, 0.1762115152861813971, 0.2006533276216794781 ),
 ( 0.000000000000000000, 1.000000000000000000 ),
 .UNSPECIFIED. ) 
 GEOMETRIC_REPRESENTATION_ITEM ( )  RATIONAL_B_SPLINE_SURFACE ( (
 ( 1.000000000000000000, 0.9997813423572990965, 1.000000000000000000),
 ( 1.000000000000000000, 0.9990919206322235180, 1.000000000000000000),
 ( 1.000000000000000000, 0.9967874177836947291, 1.000000000000000000),
 ( 1.000000000000000000, 0.9887544623284948431, 1.000000000000000000),
 ( 1.000000000000000000, 0.9830290792199358751, 1.000000000000000000),
 ( 1.000000000000000000, 0.9678345454221568556, 1.000000000000000000),
 ( 1.000000000000000000, 0.9583650305405057024, 1.000000000000000000),
 ( 1.000000000000000000, 0.9453335293271457607, 1.000000000000000000),
 ( 1.000000000000000000, 0.9438523872744090104, 1.000000000000000000),
 ( 1.000000000000000000, 0.9415799504612152315, 1.000000000000000000),
 ( 1.000000000000000000, 0.9408140170424226234, 1.000000000000000000),
 ( 1.000000000000000000, 0.9396523143998946059, 1.000000000000000000),
 ( 1.000000000000000000, 0.9392629463989466965, 1.000000000000000000),
 ( 1.000000000000000000, 0.9386756783046048547, 1.000000000000000000),
 ( 1.000000000000000000, 0.9384793862554827726, 1.000000000000000000),
 ( 1.000000000000000000, 0.9381841422086968363, 1.000000000000000000),
 ( 1.000000000000000000, 0.9380855931974630968, 1.000000000000000000),
 ( 1.000000000000000000, 0.9379375679425695500, 1.000000000000000000),
 ( 1.000000000000000000, 0.9378881925679208864, 1.000000000000000000),
 ( 1.000000000000000000, 0.9378140790407644145, 1.000000000000000000),
 ( 1.000000000000000000, 0.9377896949153101680, 1.000000000000000000),
 ( 1.000000000000000000, 0.9377409313169018379, 1.000000000000000000),
 ( 1.000000000000000000, 0.9377165729686782747, 1.000000000000000000),
 ( 1.000000000000000000, 0.9345773786259867766, 1.000000000000000000),
 ( 1.000000000000000000, 0.9318492984274235891, 1.000000000000000000),
 ( 1.000000000000000000, 0.9273872927429864799, 1.000000000000000000),
 ( 1.000000000000000000, 0.9256532593473387749, 1.000000000000000000),
 ( 1.000000000000000000, 0.9239357372749489317, 1.000000000000000000),
 ( 1.000000000000000000, 0.9235102113426452153, 1.000000000000000000),
 ( 1.000000000000000000, 0.9229728558030405594, 1.000000000000000000),
 ( 1.000000000000000000, 0.9228633126625513938, 1.000000000000000000),
 ( 1.000000000000000000, 0.9230139704738934414, 1.000000000000000000),
 ( 1.000000000000000000, 0.9237531682200406102, 1.000000000000000000),
 ( 1.000000000000000000, 0.9264156051934446801, 1.000000000000000000),
 ( 1.000000000000000000, 0.9283388455998538014, 1.000000000000000000),
 ( 1.000000000000000000, 0.9320050037531960596, 1.000000000000000000),
 ( 1.000000000000000000, 0.9333574575349539160, 1.000000000000000000),
 ( 1.000000000000000000, 0.9355411998008593688, 1.000000000000000000),
 ( 1.000000000000000000, 0.9362956009276561797, 1.000000000000000000),
 ( 1.000000000000000000, 0.9374637148016045085, 1.000000000000000000),
 ( 1.000000000000000000, 0.9378591705544803148, 1.000000000000000000),
 ( 1.000000000000000000, 0.9384610703419883349, 1.000000000000000000),
 ( 1.000000000000000000, 0.9386631562400679085, 1.000000000000000000),
 ( 1.000000000000000000, 0.9388793792114360492, 1.000000000000000000),
 ( 1.000000000000000000, 0.9388921037490475241, 1.000000000000000000),
 ( 1.000000000000000000, 0.9389175638858683337, 1.000000000000000000),
 ( 1.000000000000000000, 0.9389305010154731512, 1.000000000000000000),
 ( 1.000000000000000000, 0.9389691441648032599, 1.000000000000000000),
 ( 1.000000000000000000, 0.9389948969011605584, 1.000000000000000000),
 ( 1.000000000000000000, 0.9390721270300055323, 1.000000000000000000),
 ( 1.000000000000000000, 0.9391235763422360883, 1.000000000000000000),
 ( 1.000000000000000000, 0.9392778120326598090, 1.000000000000000000),
 ( 1.000000000000000000, 0.9393804861645954629, 1.000000000000000000),
 ( 1.000000000000000000, 0.9427638002342189072, 1.000000000000000000),
 ( 1.000000000000000000, 0.9458915987232036082, 1.000000000000000000),
 ( 1.000000000000000000, 0.9607963039211067091, 1.000000000000000000),
 ( 1.000000000000000000, 0.9703812854709542579, 1.000000000000000000),
 ( 1.000000000000000000, 0.9854660764533734740, 1.000000000000000000),
 ( 1.000000000000000000, 0.9909632567906729861, 1.000000000000000000),
 ( 1.000000000000000000, 0.9982308762622305043, 1.000000000000000000),
 ( 1.000000000000000000, 0.9999976772054812724, 1.000000000000000000),
 ( 1.000000000000000000, 1.000000000000000000, 1.000000000000000000) ) ) 
 REPRESENTATION_ITEM ( '' )  SURFACE ( )  );
#15996=CARTESIAN_POINT ( 'NONE',  ( -87.13361725327072804, -21.49321519333431141, -7.703719777548943412E-31 ) ) ;
#15999=CARTESIAN_POINT ( 'NONE',  ( -181.5938152729462729, 40.59897145788209372, 16.81664459624710162 ) ) ;
#16000=CARTESIAN_POINT ( 'NONE',  ( 11.38508063393983250, -24.83994849154103690, -44.88728980639532296 ) ) ;
#16001=CARTESIAN_POINT ( 'NONE',  ( -162.0762913951020892, -29.48230308784744125, -29.48230308784792442 ) ) ;
#16003=CARTESIAN_POINT ( 'NONE',  ( -105.4741150117383057, 7.943527260750631314, -19.77569912955104670 ) ) ;
#16004=CARTESIAN_POINT ( 'NONE',  ( 170.2234770963711128, -10.92277846919171935, -45.64576402573189995 ) ) ;
#16005=CARTESIAN_POINT ( 'NONE',  ( 170.2234770963711128, -2.259079968736224833E-13, 24.55285855007187124 ) ) ;
#16006=CARTESIAN_POINT ( 'NONE',  ( 192.4448373802100889, 20.00000000003945644, 0.000000000000000000 ) ) ;
#16007=CARTESIAN_POINT ( 'NONE',  ( -56.48582580120557850, -30.84685318188645198, -2.449293598294708485E-15 ) ) ;
#16009=CARTESIAN_POINT ( 'NONE',  ( 136.1360204305621266, -4.966164525587039691, -2.449293598294708485E-15 ) ) ;
#16010=CARTESIAN_POINT ( 'NONE',  ( -110.0700150100807519, 17.57514348718454045, 10.00661953090928691 ) ) ;
#16011=CARTESIAN_POINT ( 'NONE',  ( 4.995406935893283773, 40.00000000000017764, -15.24977328854790848 ) ) ;
#16012=CARTESIAN_POINT ( 'NONE',  ( -213.1075012329537230, 37.98287015391236565, -18.58567234101138510 ) ) ;
#16013=CARTESIAN_POINT ( 'NONE',  ( 192.4448373802101173, 19.99999999996065014, -40.00000000000002132 ) ) ;
#16015=CARTESIAN_POINT ( 'NONE',  ( 23.46661716383121288, -46.77475180958801815, 13.79413593526245840 ) ) ;
#16016=CARTESIAN_POINT ( 'NONE',  ( -199.9999999999999432, -39.01096890182021326, -39.01096890182085986 ) ) ;
#16017=AXIS2_PLACEMENT_3D ( 'NONE', #14529, #16660, #18654 ) ;
#16018=CARTESIAN_POINT ( 'NONE',  ( 130.8568914410475088, 4.207082182989741348, -52.36146031193420924 ) ) ;
#16019=CARTESIAN_POINT ( 'NONE',  ( 57.59792236341149163, -40.00000000000014211, 37.56421063658172699 ) ) ;
#16020=CARTESIAN_POINT ( 'NONE',  ( 57.59792236341147031, 26.56190807104652052, 30.00663442387728708 ) ) ;
#16021=CARTESIAN_POINT ( 'NONE',  ( -91.56559293963834989, -22.67402823373193499, 0.000000000000000000 ) ) ;
#16022=CARTESIAN_POINT ( 'NONE',  ( -86.96347745069644475, -21.75974354311652093, -40.00000000000002132 ) ) ;
#16026=CARTESIAN_POINT ( 'NONE',  ( 14.38125909742180397, 67.30136555898270956, -10.73282306405792319 ) ) ;
#16027=CARTESIAN_POINT ( 'NONE',  ( -91.56559293963834989, -40.53558337403692491, 16.03295912088671571 ) ) ;
#16028=CARTESIAN_POINT ( 'NONE',  ( -192.1131556193064682, -14.00853984552904485, 48.19965519933757747 ) ) ;
#16030=CARTESIAN_POINT ( 'NONE',  ( -208.1127848780264742, -67.17687982760682530, -10.60833733268364298 ) ) ;
#16032=CARTESIAN_POINT ( 'NONE',  ( 4.995406935893289102, 10.78321810389013002, -10.78321810388986712 ) ) ;
#16033=CARTESIAN_POINT ( 'NONE',  ( -56.48582580120559271, 6.472252184284211118, -6.472252184284153387 ) ) ;
#16036=CARTESIAN_POINT ( 'NONE',  ( -213.1075012329537230, -40.00000000000011369, 13.71589010951897691 ) ) ;
#16037=CARTESIAN_POINT ( 'NONE',  ( 163.1118516004056573, 47.56205970284957374, 9.006482792074494981 ) ) ;
#16039=CARTESIAN_POINT ( 'NONE',  ( -4.558244102846631840, 42.85231560262757711, -23.34817229226003832 ) ) ;
#16040=CARTESIAN_POINT ( 'NONE',  ( -213.1075012329537230, 13.71589010951907817, -40.00000000000002132 ) ) ;
#16042=FACE_OUTER_BOUND ( 'NONE', #14779, .T. ) ;
#16043=( BOUNDED_SURFACE ( )  B_SPLINE_SURFACE ( 3, 3, ( 
 ( #26191, #7930, #6081, #3685, #15904, #21910, #13780, #7788, #11927, #24033, #9801, #11793, #4095, #5946, #9668, #17906, #5812, #23765, #5674, #3550, #14054, #24316, #16180, #12061, #22188, #1696, #3962, #20179, #17638, #20052 ),
 ( #5545, #1961, #20317, #14185, #10068, #18173, #7656, #12195, #26321, #17772, #11651, #19912, #19774, #25915, #15770, #6732, #2225, #2353, #14844, #8462, #2093, #4622, #6466, #10466, #22977, #24842, #14715, #16849, #12721, #14581 ),
 ( #90, #24440, #494, #6207, #22710, #8601, #6332, #14454, #4755, #22582, #4487, #4361, #18442, #20846, #625, #12860, #12588, #24712, #16580, #18578, #20719, #217, #6595, #22847, #24982, #2484, #10597, #18710, #16315, #16710 ),
 ( #2623, #10333, #10202, #10736, #18847, #18304, #8732, #8199, #14319, #22453, #4232, #12321, #20448, #8328, #358, #16452, #24576, #12452, #20579, #5620, #7125, #3623, #7601, #1636, #15106, #7732, #20978, #1504, #25372, #10864 ),
 ( #6991, #15235, #23240, #10999, #13726, #19851, #15844, #23367, #17232, #9120, #21243, #1018, #19108, #25857, #15713, #9745, #5490, #3496, #13590, #8865, #21721, #21851, #11595, #2891, #17845, #25995, #9610, #19716, #892, #18981 ),
 ( #17715, #23840, #23974, #11733, #5750, #2759, #760, #16977, #25113, #6863, #9002, #14979, #23113, #4885, #5016, #13122, #12992, #17106, #21112, #11125, #25238, #3017, #19237, #8269, #22399, #12268, #10402, #8003, #20260, #26267 ),
 ( #16523, #22527, #2168, #24651, #30, #2292, #8141, #2039, #24522, #26124, #4174, #4307, #1904, #11865, #4037, #5886, #17978, #16257, #12136, #18116, #24385, #14260, #6024, #6150, #10142, #20125, #12396, #7866, #10008, #24250 ) ),
 .UNSPECIFIED., .T., .F., .F. ) 
 B_SPLINE_SURFACE_WITH_KNOTS ( ( 4, 3, 4 ),
 ( 4, 2, 2, 2, 2, 2, 2, 2, 2, 2, 2, 2, 2, 2, 4 ),
 ( 0.000000000000000000, 0.5000000000000000000, 1.000000000000000000 ),
 ( 0.000000000000000000, 0.1357259735107005372, 0.1651108541090157700, 0.1944957347073310028, 0.3598804999793158710, 0.3867117631979620773, 0.4135430264166082281, 0.5789277916885930964, 0.6062785021374117456, 0.6336292125862302838, 0.8508620842112317728, 0.8814014469398914198, 0.9119408096685510667, 0.9559704048342755334, 1.000000000000000000 ),
 .UNSPECIFIED. ) 
 GEOMETRIC_REPRESENTATION_ITEM ( )  RATIONAL_B_SPLINE_SURFACE ( (
 ( 1.000000000000000000, 1.000000000000000000, 1.000000000000000000, 1.000000000000000000, 1.000000000000000000, 1.000000000000000000, 1.000000000000000000, 1.000000000000000000, 1.000000000000000000, 1.000000000000000000, 1.000000000000000000, 1.000000000000000000, 1.000000000000000000, 1.000000000000000000, 1.000000000000000000, 1.000000000000000000, 1.000000000000000000, 1.000000000000000000, 1.000000000000000000, 1.000000000000000000, 1.000000000000000000, 1.000000000000000000, 1.000000000000000000, 1.000000000000000000, 1.000000000000000000, 1.000000000000000000, 1.000000000000000000, 1.000000000000000000, 1.000000000000000000, 1.000000000000000000),
 ( 0.3333333333333333703, 0.3333333333333333703, 0.3333333333333333703, 0.3333333333333333703, 0.3333333333333333703, 0.3333333333333333703, 0.3333333333333333703, 0.3333333333333333703, 0.3333333333333333703, 0.3333333333333333703, 0.3333333333333333703, 0.3333333333333333703, 0.3333333333333333703, 0.3333333333333333703, 0.3333333333333333703, 0.3333333333333333703, 0.3333333333333333703, 0.3333333333333333703, 0.3333333333333333703, 0.3333333333333333703, 0.3333333333333333703, 0.3333333333333333703, 0.3333333333333333703, 0.3333333333333333703, 0.3333333333333333703, 0.3333333333333333703, 0.3333333333333333703, 0.3333333333333333703, 0.3333333333333333703, 0.3333333333333333703),
 ( 0.3333333333333333703, 0.3333333333333333703, 0.3333333333333333703, 0.3333333333333333703, 0.3333333333333333703, 0.3333333333333333703, 0.3333333333333333703, 0.3333333333333333703, 0.3333333333333333703, 0.3333333333333333703, 0.3333333333333333703, 0.3333333333333333703, 0.3333333333333333703, 0.3333333333333333703, 0.3333333333333333703, 0.3333333333333333703, 0.3333333333333333703, 0.3333333333333333703, 0.3333333333333333703, 0.3333333333333333703, 0.3333333333333333703, 0.3333333333333333703, 0.3333333333333333703, 0.3333333333333333703, 0.3333333333333333703, 0.3333333333333333703, 0.3333333333333333703, 0.3333333333333333703, 0.3333333333333333703, 0.3333333333333333703),
 ( 1.000000000000000000, 1.000000000000000000, 1.000000000000000000, 1.000000000000000000, 1.000000000000000000, 1.000000000000000000, 1.000000000000000000, 1.000000000000000000, 1.000000000000000000, 1.000000000000000000, 1.000000000000000000, 1.000000000000000000, 1.000000000000000000, 1.000000000000000000, 1.000000000000000000, 1.000000000000000000, 1.000000000000000000, 1.000000000000000000, 1.000000000000000000, 1.000000000000000000, 1.000000000000000000, 1.000000000000000000, 1.000000000000000000, 1.000000000000000000, 1.000000000000000000, 1.000000000000000000, 1.000000000000000000, 1.000000000000000000, 1.000000000000000000, 1.000000000000000000),
 ( 0.3333333333333333703, 0.3333333333333333703, 0.3333333333333333703, 0.3333333333333333703, 0.3333333333333333703, 0.3333333333333333703, 0.3333333333333333703, 0.3333333333333333703, 0.3333333333333333703, 0.3333333333333333703, 0.3333333333333333703, 0.3333333333333333703, 0.3333333333333333703, 0.3333333333333333703, 0.3333333333333333703, 0.3333333333333333703, 0.3333333333333333703, 0.3333333333333333703, 0.3333333333333333703, 0.3333333333333333703, 0.3333333333333333703, 0.3333333333333333703, 0.3333333333333333703, 0.3333333333333333703, 0.3333333333333333703, 0.3333333333333333703, 0.3333333333333333703, 0.3333333333333333703, 0.3333333333333333703, 0.3333333333333333703),
 ( 0.3333333333333333703, 0.3333333333333333703, 0.3333333333333333703, 0.3333333333333333703, 0.3333333333333333703, 0.3333333333333333703, 0.3333333333333333703, 0.3333333333333333703, 0.3333333333333333703, 0.3333333333333333703, 0.3333333333333333703, 0.3333333333333333703, 0.3333333333333333703, 0.3333333333333333703, 0.3333333333333333703, 0.3333333333333333703, 0.3333333333333333703, 0.3333333333333333703, 0.3333333333333333703, 0.3333333333333333703, 0.3333333333333333703, 0.3333333333333333703, 0.3333333333333333703, 0.3333333333333333703, 0.3333333333333333703, 0.3333333333333333703, 0.3333333333333333703, 0.3333333333333333703, 0.3333333333333333703, 0.3333333333333333703),
 ( 1.000000000000000000, 1.000000000000000000, 1.000000000000000000, 1.000000000000000000, 1.000000000000000000, 1.000000000000000000, 1.000000000000000000, 1.000000000000000000, 1.000000000000000000, 1.000000000000000000, 1.000000000000000000, 1.000000000000000000, 1.000000000000000000, 1.000000000000000000, 1.000000000000000000, 1.000000000000000000, 1.000000000000000000, 1.000000000000000000, 1.000000000000000000, 1.000000000000000000, 1.000000000000000000, 1.000000000000000000, 1.000000000000000000, 1.000000000000000000, 1.000000000000000000, 1.000000000000000000, 1.000000000000000000, 1.000000000000000000, 1.000000000000000000, 1.000000000000000000) ) ) 
 REPRESENTATION_ITEM ( '' )  SURFACE ( )  );
#16046=CARTESIAN_POINT ( 'NONE',  ( -105.3895334812053193, -6.678845697753541089, 20.30817960291332369 ) ) ;
#16048=CARTESIAN_POINT ( 'NONE',  ( -188.9524464571102556, -43.19209889639846978, 23.58788642769247090 ) ) ;
#16050=CARTESIAN_POINT ( 'NONE',  ( 6.984886629847075312, -14.16808340396305255, 49.25486234615101466 ) ) ;
#16051=EDGE_CURVE ( 'NONE', #61, #7472, #10091, .T. ) ;
#16052=EDGE_CURVE ( 'NONE', #22053, #13885, #16832, .T. ) ;
#16053=CARTESIAN_POINT ( 'NONE',  ( 22.72611120194095236, 17.88893075486401329, -43.18769924474474919 ) ) ;
#16056=CARTESIAN_POINT ( 'NONE',  ( -187.7699188115425102, -23.34606611631818751, 42.84915433766021664 ) ) ;
#16057=CARTESIAN_POINT ( 'NONE',  ( 14.38125909742180397, 67.30136555898270956, -10.73282306405792319 ) ) ;
#16058=CARTESIAN_POINT ( 'NONE',  ( 200.0000000000000000, 20.00000000000013856, 40.00000000000002132 ) ) ;
#16059=CARTESIAN_POINT ( 'NONE',  ( -188.3120606736140417, 13.82878088495430191, -46.99497558484331705 ) ) ;
#16060=CARTESIAN_POINT ( 'NONE',  ( 4.995406935893289102, 10.78321810389013002, -10.78321810388986712 ) ) ;
#16062=CARTESIAN_POINT ( 'NONE',  ( 130.8568914410475372, 34.05028731879791337, 0.000000000000000000 ) ) ;
#16063=CARTESIAN_POINT ( 'NONE',  ( -280.0000000000000568, -20.00000000000006750, 40.00000000000002132 ) ) ;
#16064=CARTESIAN_POINT ( 'NONE',  ( 199.9999999999999432, 2.486775779033024914E-13, -19.99999999999992539 ) ) ;
#16065=CARTESIAN_POINT ( 'NONE',  ( -238.4067589809705794, 57.25054294077225592, 0.6820004458485544596 ) ) ;
#16067=CARTESIAN_POINT ( 'NONE',  ( 146.6084372240433709, 52.76785682606523409, -3.800685668858194255 ) ) ;
#16069=CARTESIAN_POINT ( 'NONE',  ( 4.995406935893294431, -17.50105314357198694, 39.06748935135188816 ) ) ;
#16070=CARTESIAN_POINT ( 'NONE',  ( -238.4067589809705794, -0.9644942799826262680, 0.000000000000000000 ) ) ;
#16071=CARTESIAN_POINT ( 'NONE',  ( -105.4741150117391300, -8.366608964594041353, 19.60045294982699460 ) ) ;
#16074=ORIENTED_EDGE ( 'NONE', *, *, #21445, .T. ) ;
#16075=CARTESIAN_POINT ( 'NONE',  ( 170.2234770963711128, -10.92277846919171935, -45.64576402573189995 ) ) ;
#16076=CARTESIAN_POINT ( 'NONE',  ( 23.10188454848739070, -46.91040837923751639, -13.81611343686933502 ) ) ;
#16077=ORIENTED_EDGE ( 'NONE', *, *, #20019, .T. ) ;
#16078=CARTESIAN_POINT ( 'NONE',  ( 184.8905102610680444, 19.07866798485562398, -40.00000000000002132 ) ) ;
#16079=CARTESIAN_POINT ( 'NONE',  ( -88.38011430172180383, -20.03522014374173210, 8.298859908482608461 ) ) ;
#16080=AXIS2_PLACEMENT_3D ( 'NONE', #6545, #13196, #25059 ) ;
#16081=ORIENTED_EDGE ( 'NONE', *, *, #2836, .F. ) ;
#16083=CARTESIAN_POINT ( 'NONE',  ( -109.1264249741454933, -33.12752917269487796, -13.72187187123350327 ) ) ;
#16084=CARTESIAN_POINT ( 'NONE',  ( 146.6084372240433993, -24.48358557860319706, -24.48358557860330720 ) ) ;
#16085=CARTESIAN_POINT ( 'NONE',  ( -188.3120606736019340, -43.00889065702904190, -23.45204117844409453 ) ) ;
#16086=CARTESIAN_POINT ( 'NONE',  ( 200.0000000000000000, -40.00000000000005684, 19.99999999999978328 ) ) ;
#16087=CARTESIAN_POINT ( 'NONE',  ( -213.1075012329537230, 53.71589010953660193, 40.00000000000002132 ) ) ;
#16090=CARTESIAN_POINT ( 'NONE',  ( -162.0762913951020892, -3.568845385355699554E-14, 1.694272876828323948 ) ) ;
#16091=CARTESIAN_POINT ( 'NONE',  ( 200.0000000000000000, -39.99999999999991473, -20.00000000000024514 ) ) ;
#16092=CARTESIAN_POINT ( 'NONE',  ( -192.9588430854689989, 1.161019517985663313E-13, -14.46834944099969533 ) ) ;
#16093=CARTESIAN_POINT ( 'NONE',  ( -200.0000000000000000, -47.13392792189006286, -16.85576820966595335 ) ) ;
#16094=CARTESIAN_POINT ( 'NONE',  ( 136.1360204305621551, -31.79587985999244282, -24.77266263493140386 ) ) ;
#16095=CARTESIAN_POINT ( 'NONE',  ( -192.9588430854689989, -14.46834944099973086, 0.000000000000000000 ) ) ;
#16096=CARTESIAN_POINT ( 'NONE',  ( 57.59792236341147031, -26.56190807104670171, -30.00663442387710234 ) ) ;
#16098=CARTESIAN_POINT ( 'NONE',  ( 21.99343714674520811, -47.30053030063386643, 13.87412077874992278 ) ) ;
#16099=CARTESIAN_POINT ( 'NONE',  ( 116.7964245048539169, 19.78678521258989065, 19.78678521259021039 ) ) ;
#16100=CARTESIAN_POINT ( 'NONE',  ( -192.9588430854690273, -40.00000000000011369, 14.46834944099955855 ) ) ;
#16101=CARTESIAN_POINT ( 'NONE',  ( 19.06497207195979726, 38.31983398719629719, -18.24870850772750686 ) ) ;
#16102=CARTESIAN_POINT ( 'NONE',  ( 184.8905102610680444, 14.79361573936375507, 14.79361573936398067 ) ) ;
#16103=CARTESIAN_POINT ( 'NONE',  ( -188.9524938556044162, -23.58789616778188147, -43.19211203807876132 ) ) ;
#16104=CARTESIAN_POINT ( 'NONE',  ( -213.1075012329537230, -37.98287015391232302, -18.58567234101164800 ) ) ;
#16107=CARTESIAN_POINT ( 'NONE',  ( -162.0762913951021176, -27.08623940707584055, -29.48230308784799547 ) ) ;
#16108=EDGE_CURVE ( 'NONE', #19940, #11892, #1117, .T. ) ;
#16109=CARTESIAN_POINT ( 'NONE',  ( 98.29820294267871361, -20.00000000000369837, 2.581272653893885938 ) ) ;
#16110=CARTESIAN_POINT ( 'NONE',  ( 146.6084372240433993, 34.62501878078308692, 0.000000000000000000 ) ) ;
#16112=CARTESIAN_POINT ( 'NONE',  ( 184.8905102610680444, -14.79361573936330565, -41.77492675556016621 ) ) ;
#16113=CARTESIAN_POINT ( 'NONE',  ( -90.07798792367798058, 22.27377874500493604, -0.000000000000000000 ) ) ;
#16117=CARTESIAN_POINT ( 'NONE',  ( -4.915070467883093208, 13.76630780994167580, 46.68718905934800034 ) ) ;
#16120=CARTESIAN_POINT ( 'NONE',  ( -208.1127848780265026, 10.60833733269537049, 10.60833733269544510 ) ) ;
#16122=CARTESIAN_POINT ( 'NONE',  ( -105.2502192156942868, 3.402547493085597896, 21.20168261175021129 ) ) ;
#16123=CARTESIAN_POINT ( 'NONE',  ( -198.0356074513804572, 10.87444709759714989, 10.87444709759722450 ) ) ;
#16126=CARTESIAN_POINT ( 'NONE',  ( -280.0000000000000000, -2.609240458947769655E-13, 20.00000000000001421 ) ) ;
#16131=CARTESIAN_POINT ( 'NONE',  ( -186.9957605999037753, 41.92394832788998826, 17.36546798563979976 ) ) ;
#16132=CARTESIAN_POINT ( 'NONE',  ( -3.993758944536758726, -13.83056263162038135, -47.00698038897023423 ) ) ;
#16133=CARTESIAN_POINT ( 'NONE',  ( -86.96347745069643054, -41.18208027870611687, 15.38646221621750954 ) ) ;
#16135=CARTESIAN_POINT ( 'NONE',  ( -114.7826396787322238, 2.131776515495821831E-13, -22.13135001986798400 ) ) ;
#16136=CARTESIAN_POINT ( 'NONE',  ( 4.995406935893305977, -39.06748935135212264, 39.06748935135171763 ) ) ;
#16137=CARTESIAN_POINT ( 'NONE',  ( 130.8568914410475372, -3.326198072800416995E-13, 34.05028731879788495 ) ) ;
#16138=CARTESIAN_POINT ( 'NONE',  ( -259.2033419157646676, 35.01439189186559275, -21.55415060305807984 ) ) ;
#16140=CARTESIAN_POINT ( 'NONE',  ( 130.8568914410475372, -5.949712681206667853, -2.449293598294708485E-15 ) ) ;
#16142=CARTESIAN_POINT ( 'NONE',  ( 151.7948205124836534, -6.767089262349000656, -40.00000000000002132 ) ) ;
#16143=CARTESIAN_POINT ( 'NONE',  ( -105.2709636321762616, 17.75029751208181139, 12.04384390868683496 ) ) ;
#16144=CARTESIAN_POINT ( 'NONE',  ( -238.4067589809705794, 3.877349844572403567E-13, -40.96449427998260973 ) ) ;
#16146=CARTESIAN_POINT ( 'NONE',  ( -162.0762913951020892, 1.198031840385716418, 1.198031840385750169 ) ) ;
#16148=CARTESIAN_POINT ( 'NONE',  ( -30.26275506840324425, 1.694272468446254232, -40.00000000000002132 ) ) ;
#16149=ORIENTED_EDGE ( 'NONE', *, *, #18004, .F. ) ;
#16151=ORIENTED_EDGE ( 'NONE', *, *, #12049, .F. ) ;
#16152=CARTESIAN_POINT ( 'NONE',  ( 57.59792236341147031, -2.435789363418150000, 40.00000000000002132 ) ) ;
#16154=CARTESIAN_POINT ( 'NONE',  ( -100.7734535825088358, -8.145438380286941744E-14, 17.32597176626811120 ) ) ;
#16155=CARTESIAN_POINT ( 'NONE',  ( -259.2033419157646676, 21.55415060305790931, 35.01439189186571355 ) ) ;
#16156=CARTESIAN_POINT ( 'NONE',  ( 91.82158438592158234, -17.20528682183298486, 0.000000000000000000 ) ) ;
#16157=CARTESIAN_POINT ( 'NONE',  ( -188.2995950289364373, 13.82811170417284075, -46.99046209955416487 ) ) ;
#16158=CARTESIAN_POINT ( 'NONE',  ( 170.0000000000000000, 24.25569233607185282, -6.285860131565223163 ) ) ;
#16161=CARTESIAN_POINT ( 'NONE',  ( 146.6084372240433993, 3.800685668858732935, -3.800685668858610367 ) ) ;
#16162=CARTESIAN_POINT ( 'NONE',  ( 91.82158438592159655, -44.40256751092341858, 12.16597498400012434 ) ) ;
#16165=CARTESIAN_POINT ( 'NONE',  ( -82.24432634623720162, 12.38461122507612089, -15.96101146153671912 ) ) ;
#16166=CARTESIAN_POINT ( 'NONE',  ( 163.1118516004056573, -9.006482792069506971, -9.006482792069697041 ) ) ;
#16167=CARTESIAN_POINT ( 'NONE',  ( -65.65550967526027648, 9.107276986624018633, 24.89650881518432968 ) ) ;
#16168=CARTESIAN_POINT ( 'NONE',  ( 200.0000000000000000, -42.42640687119272513, -14.14213562373140753 ) ) ;
#16169=CARTESIAN_POINT ( 'NONE',  ( 192.4448373802100889, 14.14213562375893574, -14.14213562375874922 ) ) ;
#16172=CARTESIAN_POINT ( 'NONE',  ( 151.7948205124836534, 40.00000000000002842, 6.767089262349174739 ) ) ;
#16174=CARTESIAN_POINT ( 'NONE',  ( 22.75856136761854387, 43.17893233522199381, -17.88529938203877379 ) ) ;
#16175=CARTESIAN_POINT ( 'NONE',  ( 91.82158438592158234, 22.79471317813472453, -40.00000000000002132 ) ) ;
#16177=CARTESIAN_POINT ( 'NONE',  ( 199.9999999999999432, -14.14213562373096345, -14.14213562373104871 ) ) ;
#16178=CARTESIAN_POINT ( 'NONE',  ( -47.65341557551126073, -29.74088027401770518, 14.80716566690741409 ) ) ;
#16180=CARTESIAN_POINT ( 'NONE',  ( 136.1360204305621266, -35.03383547441293899, 0.000000000000000000 ) ) ;
#16181=EDGE_LOOP ( 'NONE', ( #21805, #10139, #20123, #7789 ) ) ;
#16182=CARTESIAN_POINT ( 'NONE',  ( -188.9266304146012203, -43.31220791188976449, 17.94050393342803673 ) ) ;
#16187=CARTESIAN_POINT ( 'NONE',  ( 20.16956056503475736, -23.97604322319281422, 43.71646652951534406 ) ) ;
#16188=CARTESIAN_POINT ( 'NONE',  ( 22.37977766478910979, 13.85469381971835290, -47.17011059971203224 ) ) ;
#16190=CARTESIAN_POINT ( 'NONE',  ( -91.56559293963834989, -2.543181659092656077E-13, 22.67402823373191723 ) ) ;
#16191=CARTESIAN_POINT ( 'NONE',  ( 133.2080217031554525, -29.90338805389125199, 12.38638889282714928 ) ) ;
#16192=CARTESIAN_POINT ( 'NONE',  ( -114.4364955367308454, -8.644468109209068274, 20.04994829327590011 ) ) ;
#16193=CARTESIAN_POINT ( 'NONE',  ( 170.2234770963711128, 10.92277846919216522, -10.92277846919186501 ) ) ;
#16194=CARTESIAN_POINT ( 'NONE',  ( 151.7948205124836250, 33.23291073765556547, 0.000000000000000000 ) ) ;
#16195=CIRCLE ( 'NONE', #1779, 15.00000000000000178 ) ;
#16196=CARTESIAN_POINT ( 'NONE',  ( -190.7346372394923151, 13.94676542150583742, -47.78727444208931274 ) ) ;
#16197=CARTESIAN_POINT ( 'NONE',  ( -30.26275506840324070, 1.198031551616030033, -1.198031551616006496 ) ) ;
#16198=CARTESIAN_POINT ( 'NONE',  ( 14.38125909742182884, -55.17850393972636169, -2.449293598294708485E-15 ) ) ;
#16199=CIRCLE ( 'NONE', #4758, 14.99999999999999645 ) ;
#16200=CARTESIAN_POINT ( 'NONE',  ( 192.4448373802101173, 19.99999999996063949, 40.00000000000002132 ) ) ;
#16201=CARTESIAN_POINT ( 'NONE',  ( 200.0000000000000000, 40.00000000000026290, -19.99999999999950617 ) ) ;
#16202=CARTESIAN_POINT ( 'NONE',  ( 192.4448373802101173, -14.14213562375886291, 42.42640687116498555 ) ) ;
#16203=( BOUNDED_SURFACE ( )  B_SPLINE_SURFACE ( 3, 3, ( 
 ( #14703, #25102, #613, #8719, #18970, #22963, #20966, #2747, #750, #21101, #18697, #8854, #14568, #25227, #23228, #6851, #18565, #2881, #10989, #6980, #20567, #344, #8448, #22698, #4473, #12573, #10581, #17221, #1261, #17351 ),
 ( #7616, #23602, #25487, #15357, #5507, #25359, #5381, #9110, #1522, #13486, #3380, #7236, #7114, #5133, #19351, #1393, #15731, #19735, #17731, #23481, #5006, #11111, #15225, #1007, #11358, #23356, #3005, #21737, #13238, #13608 ),
 ( #19607, #21607, #13357, #15473, #11479, #9494, #3513, #5253, #11613, #25872, #19474, #21232, #21361, #7490, #17599, #25738, #13111, #19227, #3130, #15601, #21479, #3254, #11233, #1140, #9244, #9365, #17475, #7363, #25617, #23726 ),
 ( #9628, #1920, #18135, #16274, #48, #13878, #2057, #5769, #22142, #12285, #21867, #13741, #1653, #16007, #11884, #9762, #23856, #8161, #179, #9894, #24133, #16140, #5634, #24270, #1790, #17862, #6169, #18266, #22011, #26013 ),
 ( #5905, #7749, #2188, #8286, #26284, #3643, #10025, #8023, #24403, #22416, #4054, #20004, #6043, #15861, #14013, #17998, #23990, #20142, #26142, #3780, #18403, #11750, #10296, #4192, #7886, #20413, #3924, #12022, #14148, #22280 ),
 ( #12155, #20278, #10163, #14279, #19869, #852, #4848, #2856, #8560, #16412, #22544, #2312, #12415, #22808, #18538, #14414, #6824, #10421, #16938, #320, #24540, #20945, #4585, #6296, #25073, #10698, #23077, #8421, #12954, #12544 ),
 ( #4324, #20541, #18943, #8696, #2723, #16542, #24672, #6428, #723, #24806, #6558, #10964, #22676, #14546, #16675, #14672, #4449, #12682, #20812, #20676, #589, #2445, #10557, #18669, #24944, #456, #18809, #2583, #19071, #16807 ) ),
 .UNSPECIFIED., .T., .F., .F. ) 
 B_SPLINE_SURFACE_WITH_KNOTS ( ( 4, 3, 4 ),
 ( 4, 2, 2, 2, 2, 2, 2, 2, 2, 2, 2, 2, 2, 2, 4 ),
 ( 0.000000000000000000, 0.5000000000000000000, 1.000000000000000000 ),
 ( 0.000000000000000000, 0.1357259735107005372, 0.1651108541090157700, 0.1944957347073310028, 0.3598804999793158710, 0.3867117631979620773, 0.4135430264166082281, 0.5789277916885930964, 0.6062785021374117456, 0.6336292125862302838, 0.8508620842112317728, 0.8814014469398914198, 0.9119408096685510667, 0.9559704048342755334, 1.000000000000000000 ),
 .UNSPECIFIED. ) 
 GEOMETRIC_REPRESENTATION_ITEM ( )  RATIONAL_B_SPLINE_SURFACE ( (
 ( 1.000000000000000000, 1.000000000000000000, 1.000000000000000000, 1.000000000000000000, 1.000000000000000000, 1.000000000000000000, 1.000000000000000000, 1.000000000000000000, 1.000000000000000000, 1.000000000000000000, 1.000000000000000000, 1.000000000000000000, 1.000000000000000000, 1.000000000000000000, 1.000000000000000000, 1.000000000000000000, 1.000000000000000000, 1.000000000000000000, 1.000000000000000000, 1.000000000000000000, 1.000000000000000000, 1.000000000000000000, 1.000000000000000000, 1.000000000000000000, 1.000000000000000000, 1.000000000000000000, 1.000000000000000000, 1.000000000000000000, 1.000000000000000000, 1.000000000000000000),
 ( 0.3333333333333333703, 0.3333333333333333703, 0.3333333333333333703, 0.3333333333333333703, 0.3333333333333333703, 0.3333333333333333703, 0.3333333333333333703, 0.3333333333333333703, 0.3333333333333333703, 0.3333333333333333703, 0.3333333333333333703, 0.3333333333333333703, 0.3333333333333333703, 0.3333333333333333703, 0.3333333333333333703, 0.3333333333333333703, 0.3333333333333333703, 0.3333333333333333703, 0.3333333333333333703, 0.3333333333333333703, 0.3333333333333333703, 0.3333333333333333703, 0.3333333333333333703, 0.3333333333333333703, 0.3333333333333333703, 0.3333333333333333703, 0.3333333333333333703, 0.3333333333333333703, 0.3333333333333333703, 0.3333333333333333703),
 ( 0.3333333333333333703, 0.3333333333333333703, 0.3333333333333333703, 0.3333333333333333703, 0.3333333333333333703, 0.3333333333333333703, 0.3333333333333333703, 0.3333333333333333703, 0.3333333333333333703, 0.3333333333333333703, 0.3333333333333333703, 0.3333333333333333703, 0.3333333333333333703, 0.3333333333333333703, 0.3333333333333333703, 0.3333333333333333703, 0.3333333333333333703, 0.3333333333333333703, 0.3333333333333333703, 0.3333333333333333703, 0.3333333333333333703, 0.3333333333333333703, 0.3333333333333333703, 0.3333333333333333703, 0.3333333333333333703, 0.3333333333333333703, 0.3333333333333333703, 0.3333333333333333703, 0.3333333333333333703, 0.3333333333333333703),
 ( 1.000000000000000000, 1.000000000000000000, 1.000000000000000000, 1.000000000000000000, 1.000000000000000000, 1.000000000000000000, 1.000000000000000000, 1.000000000000000000, 1.000000000000000000, 1.000000000000000000, 1.000000000000000000, 1.000000000000000000, 1.000000000000000000, 1.000000000000000000, 1.000000000000000000, 1.000000000000000000, 1.000000000000000000, 1.000000000000000000, 1.000000000000000000, 1.000000000000000000, 1.000000000000000000, 1.000000000000000000, 1.000000000000000000, 1.000000000000000000, 1.000000000000000000, 1.000000000000000000, 1.000000000000000000, 1.000000000000000000, 1.000000000000000000, 1.000000000000000000),
 ( 0.3333333333333333703, 0.3333333333333333703, 0.3333333333333333703, 0.3333333333333333703, 0.3333333333333333703, 0.3333333333333333703, 0.3333333333333333703, 0.3333333333333333703, 0.3333333333333333703, 0.3333333333333333703, 0.3333333333333333703, 0.3333333333333333703, 0.3333333333333333703, 0.3333333333333333703, 0.3333333333333333703, 0.3333333333333333703, 0.3333333333333333703, 0.3333333333333333703, 0.3333333333333333703, 0.3333333333333333703, 0.3333333333333333703, 0.3333333333333333703, 0.3333333333333333703, 0.3333333333333333703, 0.3333333333333333703, 0.3333333333333333703, 0.3333333333333333703, 0.3333333333333333703, 0.3333333333333333703, 0.3333333333333333703),
 ( 0.3333333333333333703, 0.3333333333333333703, 0.3333333333333333703, 0.3333333333333333703, 0.3333333333333333703, 0.3333333333333333703, 0.3333333333333333703, 0.3333333333333333703, 0.3333333333333333703, 0.3333333333333333703, 0.3333333333333333703, 0.3333333333333333703, 0.3333333333333333703, 0.3333333333333333703, 0.3333333333333333703, 0.3333333333333333703, 0.3333333333333333703, 0.3333333333333333703, 0.3333333333333333703, 0.3333333333333333703, 0.3333333333333333703, 0.3333333333333333703, 0.3333333333333333703, 0.3333333333333333703, 0.3333333333333333703, 0.3333333333333333703, 0.3333333333333333703, 0.3333333333333333703, 0.3333333333333333703, 0.3333333333333333703),
 ( 1.000000000000000000, 1.000000000000000000, 1.000000000000000000, 1.000000000000000000, 1.000000000000000000, 1.000000000000000000, 1.000000000000000000, 1.000000000000000000, 1.000000000000000000, 1.000000000000000000, 1.000000000000000000, 1.000000000000000000, 1.000000000000000000, 1.000000000000000000, 1.000000000000000000, 1.000000000000000000, 1.000000000000000000, 1.000000000000000000, 1.000000000000000000, 1.000000000000000000, 1.000000000000000000, 1.000000000000000000, 1.000000000000000000, 1.000000000000000000, 1.000000000000000000, 1.000000000000000000, 1.000000000000000000, 1.000000000000000000, 1.000000000000000000, 1.000000000000000000) ) ) 
 REPRESENTATION_ITEM ( '' )  SURFACE ( )  );
#16205=CARTESIAN_POINT ( 'NONE',  ( 136.1360204305621266, 24.77266263493104148, 24.77266263493145004 ) ) ;
#16206=EDGE_LOOP ( 'NONE', ( #18196, #329, #6931, #25776 ) ) ;
#16208=CARTESIAN_POINT ( 'NONE',  ( -96.94475454966692496, -9.001119816639596038, 20.58449551010044587 ) ) ;
#16212=CARTESIAN_POINT ( 'NONE',  ( 146.6084372240433709, -32.08495691632041513, -24.48358557860343154 ) ) ;
#16213=CARTESIAN_POINT ( 'NONE',  ( 22.92196489051161024, -46.97629733300992427, -13.82589419143533327 ) ) ;
#16215=CARTESIAN_POINT ( 'NONE',  ( -208.1127848780265026, 15.00245453012665564, 0.000000000000000000 ) ) ;
#16216=CARTESIAN_POINT ( 'NONE',  ( -96.94475454971259865, -20.92018922313259921, 8.190683501837476399 ) ) ;
#16221=B_SPLINE_CURVE_WITH_KNOTS ( 'NONE', 3,
 ( #5797, #18291, #22304, #77, #10054, #14306, #20165, #10322 ),
 .UNSPECIFIED., .F., .F.,
 ( 4, 2, 2, 4 ),
 ( 0.0002282271112602323728, 0.004312542793977438421, 0.006354700635336038572, 0.008396858476694638723 ),
 .UNSPECIFIED. ) ;
#16222=CARTESIAN_POINT ( 'NONE',  ( -192.9588430854690273, 38.51493924976939098, -18.05360324515436687 ) ) ;
#16223=CARTESIAN_POINT ( 'NONE',  ( -144.1957134274819907, -30.13185274855893780, -12.48102206796960267 ) ) ;
#16224=CARTESIAN_POINT ( 'NONE',  ( -280.0000000000000568, -40.00000000000014211, 19.99999999999987210 ) ) ;
#16225=CARTESIAN_POINT ( 'NONE',  ( -238.4067589809705794, 0.9644942799825385604, 40.00000000000002132 ) ) ;
#16227=CARTESIAN_POINT ( 'NONE',  ( 192.4448373802100889, 1.051811698935164031E-13, -20.00000000003942091 ) ) ;
#16228=CARTESIAN_POINT ( 'NONE',  ( -162.0762913951020892, -1.777970010055771463E-13, 41.69427287682835015 ) ) ;
#16229=CARTESIAN_POINT ( 'NONE',  ( 151.7948205124836534, -40.00000000000034817, 33.23291073765511072 ) ) ;
#16230=CARTESIAN_POINT ( 'NONE',  ( 184.8905102610680444, 39.99999999999999289, 19.07866798485573057 ) ) ;
#16232=CARTESIAN_POINT ( 'NONE',  ( -192.9588430854689705, -38.51493924976963967, 38.51493924976919914 ) ) ;
#16233=CARTESIAN_POINT ( 'NONE',  ( 130.8568914410475088, 34.05028731879790627, -40.00000000000002132 ) ) ;
#16235=CARTESIAN_POINT ( 'NONE',  ( -280.0000000000000568, -14.14213562373078226, -42.42640687119295251 ) ) ;
#16237=CARTESIAN_POINT ( 'NONE',  ( 18.89824444022308114, -48.20791849611961766, 14.00990882958429751 ) ) ;
#16238=CARTESIAN_POINT ( 'NONE',  ( 4.995406935893290878, 1.606505379428369110E-13, -15.24977328854832592 ) ) ;
#16239=CARTESIAN_POINT ( 'NONE',  ( -238.4067589809705794, 39.99999999999983658, 40.96449428006354765 ) ) ;
#16240=CARTESIAN_POINT ( 'NONE',  ( -86.96347745069644475, 41.18208027870598187, -15.38646221621779731 ) ) ;
#16241=CARTESIAN_POINT ( 'NONE',  ( 57.59792236341147031, -26.56190807104712448, 30.00663442387673285 ) ) ;
#16242=CARTESIAN_POINT ( 'NONE',  ( -192.9370379451513884, -14.03127537977493411, -48.35015161800508565 ) ) ;
#16243=CARTESIAN_POINT ( 'NONE',  ( 57.59792236341147031, 1.722363176415065089, -1.722363176415036445 ) ) ;
#16245=CARTESIAN_POINT ( 'NONE',  ( -208.1127848780264742, -17.67593391476605547, -38.89260858015755673 ) ) ;
#16246=CARTESIAN_POINT ( 'NONE',  ( 98.29820294270304259, -18.47759065022024672, 7.653668647299475047 ) ) ;
#16247=CARTESIAN_POINT ( 'NONE',  ( -86.96347745069645896, 21.75974354311648895, -0.000000000000000000 ) ) ;
#16249=CARTESIAN_POINT ( 'NONE',  ( 14.38125909742181463, 10.73282306403652875, -67.30136555895941797 ) ) ;
#16250=CARTESIAN_POINT ( 'NONE',  ( -77.55640685876512919, -9.396736996787159758E-14, 22.13135000837102595 ) ) ;
#16253=CARTESIAN_POINT ( 'NONE',  ( 23.30631261065773430, -23.35506702541406554, 42.87793822514953490 ) ) ;
#16254=CARTESIAN_POINT ( 'NONE',  ( -3.524834090819536137, 17.92814044289615794, 43.28235980537024830 ) ) ;
#16255=VERTEX_POINT ( 'NONE', #14163 ) ;
#16257=CARTESIAN_POINT ( 'NONE',  ( 14.38125909742180752, 15.17850393972634038, 0.000000000000000000 ) ) ;
#16260=FACE_OUTER_BOUND ( 'NONE', #11299, .T. ) ;
#16261=CARTESIAN_POINT ( 'NONE',  ( 19.06497207195979726, 40.00000000000017053, -14.19242893257798599 ) ) ;
#16262=B_SPLINE_CURVE_WITH_KNOTS ( 'NONE', 3,
 ( #6999, #18590, #14724, #21125, #22856, #2901, #12734, #20729 ),
 .UNSPECIFIED., .F., .F.,
 ( 4, 2, 2, 4 ),
 ( 0.0002278873370240370642, 0.004309043385737469124, 0.006349621410094185778, 0.008390199434450903299 ),
 .UNSPECIFIED. ) ;
#16268=CARTESIAN_POINT ( 'NONE',  ( 12.96694272559235195, -14.15914421027394354, -49.19577900140984639 ) ) ;
#16269=CARTESIAN_POINT ( 'NONE',  ( -259.2033419157646676, -49.83842185052040463, 6.730120644403092101 ) ) ;
#16270=CARTESIAN_POINT ( 'NONE',  ( -110.1017833366170748, 9.975556358476777704E-14, -20.19517362627949453 ) ) ;
#16271=CARTESIAN_POINT ( 'NONE',  ( -86.96347745069643054, -41.18208027870589660, -15.38646221621809040 ) ) ;
#16272=CARTESIAN_POINT ( 'NONE',  ( -77.92915424793434909, 20.15198149301296482, 8.347224043097730473 ) ) ;
#16273=CARTESIAN_POINT ( 'NONE',  ( -56.48582580120559271, 6.472252184284121412, 6.472252184284244869 ) ) ;
#16274=CARTESIAN_POINT ( 'NONE',  ( -213.1075012329536946, -53.71589010951918652, -2.449293598294708485E-15 ) ) ;
#16276=CARTESIAN_POINT ( 'NONE',  ( 192.4448373802100889, -19.99999999996057198, -2.449293598294708485E-15 ) ) ;
#16279=CARTESIAN_POINT ( 'NONE',  ( -198.0356074513804572, 5.461327841961909642E-13, -55.37879056873073580 ) ) ;
#16280=CARTESIAN_POINT ( 'NONE',  ( 163.1118516004056573, -19.27778845538761132, -19.27778845538770724 ) ) ;
#16281=CARTESIAN_POINT ( 'NONE',  ( 151.7948205124836250, -33.23291073765550863, 0.000000000000000000 ) ) ;
#16282=ORIENTED_EDGE ( 'NONE', *, *, #21658, .T. ) ;
#16285=CARTESIAN_POINT ( 'NONE',  ( -30.26275506840324070, 1.694272468446254232, 0.000000000000000000 ) ) ;
#16288=CARTESIAN_POINT ( 'NONE',  ( -135.8532207217289738, 40.00000000000002842, -9.153146818113432559 ) ) ;
#16289=CARTESIAN_POINT ( 'NONE',  ( 4.995406935893286438, 67.35176059880245703, -10.78321810387767066 ) ) ;
#16290=CARTESIAN_POINT ( 'NONE',  ( -162.0762913951020892, 1.694272876828294194, 0.000000000000000000 ) ) ;
#16291=EDGE_CURVE ( 'NONE', #858, #20449, #24101, .T. ) ;
#16292=CARTESIAN_POINT ( 'NONE',  ( -175.9235640272266039, 12.95568063362427047, -42.70623598722775682 ) ) ;
#16293=CARTESIAN_POINT ( 'NONE',  ( -86.86493150571116928, 8.366608963953661160, 19.60045294882771572 ) ) ;
#16296=EDGE_CURVE ( 'NONE', #19940, #23643, #22560, .T. ) ;
#16298=CARTESIAN_POINT ( 'NONE',  ( 163.1118516004056573, 37.29075403953132906, 19.27778845539275565 ) ) ;
#16299=CARTESIAN_POINT ( 'NONE',  ( -208.1127848780264742, -67.17687982760682530, -10.60833733268364298 ) ) ;
#16301=CARTESIAN_POINT ( 'NONE',  ( -86.99952317291106851, 18.62540174577003427, -10.54562204237578271 ) ) ;
#16302=CARTESIAN_POINT ( 'NONE',  ( -280.0000000000000568, -14.14213562373137556, 42.42640687119276066 ) ) ;
#16304=CARTESIAN_POINT ( 'NONE',  ( -192.9588430854690273, -18.05360324515454096, 38.51493924976936967 ) ) ;
#16305=CARTESIAN_POINT ( 'NONE',  ( -238.4067589809705794, -57.25054294065807881, 0.6820004457338858517 ) ) ;
#16308=CARTESIAN_POINT ( 'NONE',  ( 199.9999999999999432, -3.553951640073651008E-14, 19.99999999999992539 ) ) ;
#16310=CARTESIAN_POINT ( 'NONE',  ( 23.05038679986473937, 43.09692730306933584, -17.85133178553897793 ) ) ;
#16311=CARTESIAN_POINT ( 'NONE',  ( -135.8532207217289738, 30.84685318188643066, 2.449293598294708485E-15 ) ) ;
#16313=CARTESIAN_POINT ( 'NONE',  ( -105.3755690713226727, -21.75974354311652093, 0.000000000000000000 ) ) ;
#16314=CARTESIAN_POINT ( 'NONE',  ( -7.769366557095455761, -41.90323276218102677, 22.72119856430033380 ) ) ;
#16315=CARTESIAN_POINT ( 'NONE',  ( 192.4448373802101173, 19.99999999996063949, 40.00000000000002132 ) ) ;
#16316=VERTEX_POINT ( 'NONE', #16293 ) ;
#16317=FACE_OUTER_BOUND ( 'NONE', #6988, .T. ) ;
#16320=CARTESIAN_POINT ( 'NONE',  ( 7.112934525951993159, -18.57375239869932670, 44.84100494512510693 ) ) ;
#16321=CARTESIAN_POINT ( 'NONE',  ( 9.345847406432913118, 14.17927947630575325, -49.32890504403901843 ) ) ;
#16323=CARTESIAN_POINT ( 'NONE',  ( 130.8568914410475372, -3.326198072800416995E-13, 34.05028731879788495 ) ) ;
#16325=CARTESIAN_POINT ( 'NONE',  ( 199.9999999999999432, 1.065690307512836407E-13, -20.00000000000010303 ) ) ;
#16326=CARTESIAN_POINT ( 'NONE',  ( -259.2033419157646676, -6.730120644402966867, -49.83842185052038332 ) ) ;
#16327=CARTESIAN_POINT ( 'NONE',  ( 192.4448373802101173, 20.00000000003945644, 40.00000000000002132 ) ) ;
#16328=CARTESIAN_POINT ( 'NONE',  ( -188.3611024622149728, 23.46270902204793529, -43.02327292322510033 ) ) ;
#16329=CARTESIAN_POINT ( 'NONE',  ( 0.2972598230769886718, 38.42060263243643448, 18.14793986248763957 ) ) ;
#16330=CARTESIAN_POINT ( 'NONE',  ( 0.2972598230769886718, 38.42060263243643448, 18.14793986248763957 ) ) ;
#16331=CARTESIAN_POINT ( 'NONE',  ( -198.0356074513804572, -55.37879056874826489, 40.00000000000002132 ) ) ;
#16332=CARTESIAN_POINT ( 'NONE',  ( -162.0762913951020892, 41.69427287692678163, -40.00000000000002132 ) ) ;
#16333=CARTESIAN_POINT ( 'NONE',  ( 136.1360204305621551, -40.00000000000036238, 35.03383547441254109 ) ) ;
#16334=CARTESIAN_POINT ( 'NONE',  ( -259.2033419157646676, 21.55415060305830366, 21.55415060305842800 ) ) ;
#16335=CARTESIAN_POINT ( 'NONE',  ( 98.29820294268670011, 19.44947291833535630, -5.307337294604018929 ) ) ;
#16336=CARTESIAN_POINT ( 'NONE',  ( 4.995406935893300648, -10.78321810387790514, -67.35176059880241439 ) ) ;
#16338=CARTESIAN_POINT ( 'NONE',  ( 184.8905102610680444, -14.79361573936379415, -14.79361573936387941 ) ) ;
#16339=CARTESIAN_POINT ( 'NONE',  ( -96.94475454971953354, 9.001119816637983106, 20.58449551010110667 ) ) ;
#16342=ORIENTED_EDGE ( 'NONE', *, *, #24271, .T. ) ;
#16343=CARTESIAN_POINT ( 'NONE',  ( -135.8532207217289738, -50.09629031063965243, -6.472252184284438492 ) ) ;
#16344=CARTESIAN_POINT ( 'NONE',  ( 22.37977766479031771, -47.17011059971120090, -13.85469381971834402 ) ) ;
#16346=CARTESIAN_POINT ( 'NONE',  ( -97.72675010090144099, -20.89622088363380925, 8.185591577777151073 ) ) ;
#16351=CARTESIAN_POINT ( 'NONE',  ( 0.2972598230769938343, 10.13633138497472252, 10.13633138497475628 ) ) ;
#16352=CARTESIAN_POINT ( 'NONE',  ( -188.4702232936898554, -47.05182887786696710, -13.83721295434361487 ) ) ;
#16353=CARTESIAN_POINT ( 'NONE',  ( 130.8568914410475088, -40.00000000000001421, 5.949712681206549725 ) ) ;
#16354=CARTESIAN_POINT ( 'NONE',  ( 151.7948205124836250, -33.23291073765550863, 0.000000000000000000 ) ) ;
#16357=CARTESIAN_POINT ( 'NONE',  ( -259.2033419157646676, -40.00000000000017764, 30.48217210827725054 ) ) ;
#16358=CARTESIAN_POINT ( 'NONE',  ( -259.2033419157646676, -1.564921101325656229E-13, 30.48217210827739621 ) ) ;
#16359=CARTESIAN_POINT ( 'NONE',  ( -280.0000000000000000, 1.839446121267387017E-14, -20.00000000000001421 ) ) ;
#16361=CARTESIAN_POINT ( 'NONE',  ( -208.1127848780264742, -38.89260858015758515, 38.89260858015713751 ) ) ;
#16362=CARTESIAN_POINT ( 'NONE',  ( -192.9588430854690273, -14.46834944099973264, -40.00000000000002132 ) ) ;
#16363=CARTESIAN_POINT ( 'NONE',  ( 170.2234770963711128, 17.36149277826973503, 39.20704971665401217 ) ) ;
#16365=CARTESIAN_POINT ( 'NONE',  ( 8.517493190815677906, -49.32792454093240764, 14.17913040910394429 ) ) ;
#16366=CARTESIAN_POINT ( 'NONE',  ( -100.7734535825088358, 1.654174317907124744E-13, -17.32597176626811120 ) ) ;
#16367=CARTESIAN_POINT ( 'NONE',  ( -91.56559293963834989, -40.00000000000009948, 17.32597176626796553 ) ) ;
#16369=CARTESIAN_POINT ( 'NONE',  ( -192.9588430854690273, 38.51493924976939098, -18.05360324515436687 ) ) ;
#16371=CARTESIAN_POINT ( 'NONE',  ( -94.58366989427317151, -9.000605044545517686, -20.58370269626833604 ) ) ;
#16372=CARTESIAN_POINT ( 'NONE',  ( 136.1360204305621551, -31.79587985999244282, -24.77266263493140386 ) ) ;
#16373=ORIENTED_EDGE ( 'NONE', *, *, #25592, .F. ) ;
#16374=CARTESIAN_POINT ( 'NONE',  ( 130.8568914410475088, -52.36146031193413108, -4.207082182990267150 ) ) ;
#16376=CARTESIAN_POINT ( 'NONE',  ( 14.38125909742182884, -55.17850393974264733, -40.00000000000002132 ) ) ;
#16377=CARTESIAN_POINT ( 'NONE',  ( -30.26275506840324070, 1.198031551616030033, -1.198031551616006496 ) ) ;
#16381=ORIENTED_EDGE ( 'NONE', *, *, #13762, .F. ) ;
#16384=CARTESIAN_POINT ( 'NONE',  ( -28.75808802781980944, -18.59445401971578704, -35.61482992978298512 ) ) ;
#16386=CARTESIAN_POINT ( 'NONE',  ( -3.856733984653986980, 17.89110409353202158, 43.19294614843431646 ) ) ;
#16387=VERTEX_POINT ( 'NONE', #21352 ) ;
#16388=ORIENTED_EDGE ( 'NONE', *, *, #25739, .F. ) ;
#16390=CARTESIAN_POINT ( 'NONE',  ( -238.4067589809705794, 0.6820004457912757223, 0.6820004457913219076 ) ) ;
#16394=CARTESIAN_POINT ( 'NONE',  ( -56.48582580120559271, -6.472252184284187138, -6.472252184284199572 ) ) ;
#16397=CARTESIAN_POINT ( 'NONE',  ( -100.0957100001246687, -8.517115559311239537, -20.56213589529557240 ) ) ;
#16398=ADVANCED_FACE ( 'NONE', ( #23219 ), #17742, .T. ) ;
#16399=CARTESIAN_POINT ( 'NONE',  ( -91.56559293963834989, 1.671088883502053755E-13, -17.32597176626811120 ) ) ;
#16400=CARTESIAN_POINT ( 'NONE',  ( -238.4067589809705794, -3.369206980223063916E-14, -0.9644942799825824142 ) ) ;
#16401=CARTESIAN_POINT ( 'NONE',  ( -114.4364955367328349, 20.29001642038852538, -8.064892380842216824 ) ) ;
#16402=CIRCLE ( 'NONE', #8322, 40.00000000000003553 ) ;
#16405=CARTESIAN_POINT ( 'NONE',  ( -188.4265004370476504, 23.47686928852973764, 43.04236487214772922 ) ) ;
#16406=CARTESIAN_POINT ( 'NONE',  ( 23.38399212876534961, -23.33762193384630379, -42.85408588822686227 ) ) ;
#16407=CARTESIAN_POINT ( 'NONE',  ( 192.4448373802101173, 14.14213562375922884, -42.42640687116488607 ) ) ;
#16408=CARTESIAN_POINT ( 'NONE',  ( -97.72675010090189573, 20.56394680065915637, -8.987772175319548751 ) ) ;
#16409=CARTESIAN_POINT ( 'NONE',  ( -208.1127848780264742, -38.89260858015758515, 38.89260858015713751 ) ) ;
#16411=CARTESIAN_POINT ( 'NONE',  ( -192.9588430854689989, -10.23066800230742501, -10.23066800230756712 ) ) ;
#16412=CARTESIAN_POINT ( 'NONE',  ( -105.3755690713226585, 21.75974354311648185, 40.00000000000002132 ) ) ;
#16414=FACE_BOUND ( 'NONE', #24514, .T. ) ;
#16415=CARTESIAN_POINT ( 'NONE',  ( -162.0762913951020607, -41.69427287692683848, 40.00000000000002132 ) ) ;
#16416=CARTESIAN_POINT ( 'NONE',  ( -114.5469942457206116, 9.971021741842124086, 19.54051464164524887 ) ) ;
#16417=CARTESIAN_POINT ( 'NONE',  ( -198.0356074513804572, 40.00000000000014921, -15.37879056873028816 ) ) ;
#16418=CARTESIAN_POINT ( 'NONE',  ( -259.2033419157646676, 21.55415060305839958, -35.01439189186541512 ) ) ;
#16419=CARTESIAN_POINT ( 'NONE',  ( 163.1118516004056573, -27.26290988616869626, -40.00000000000002132 ) ) ;
#16423=CARTESIAN_POINT ( 'NONE',  ( -280.0000000000000568, -20.00000000000006750, 40.00000000000002132 ) ) ;
#16425=CARTESIAN_POINT ( 'NONE',  ( 144.1620285550793312, 12.51613133675833822, 30.21661402164571797 ) ) ;
#16426=CARTESIAN_POINT ( 'NONE',  ( -280.0000000000000000, 14.14213562373108246, -14.14213562373078581 ) ) ;
#16427=CARTESIAN_POINT ( 'NONE',  ( -114.6297772182882397, -21.30737554388467814, -5.474609583126212264 ) ) ;
#16429=CARTESIAN_POINT ( 'NONE',  ( -199.9999999999999716, -53.44529986889247652, -10.02640517461732372 ) ) ;
#16433=CARTESIAN_POINT ( 'NONE',  ( 200.0000000000000000, 14.14213562373041455, 42.42640687119311593 ) ) ;
#16434=CARTESIAN_POINT ( 'NONE',  ( -280.0000000000000568, -42.42640687119305198, 14.14213562373058686 ) ) ;
#16435=CARTESIAN_POINT ( 'NONE',  ( -190.0000000000001705, -69.99999999999994316, 8.572527594031469837E-15 ) ) ;
#16436=CARTESIAN_POINT ( 'NONE',  ( -135.8532207217289738, 40.00000000000031974, -30.84685318188603986 ) ) ;
#16437=CARTESIAN_POINT ( 'NONE',  ( -86.96347745069645896, -12.89780903124443689, 43.67073346367968156 ) ) ;
#16439=CARTESIAN_POINT ( 'NONE',  ( 130.8568914410475372, -24.07718906447222551, -24.07718906447233209 ) ) ;
#16440=CARTESIAN_POINT ( 'NONE',  ( -105.3755690713226585, -41.18208027870589660, -15.38646221621809040 ) ) ;
#16441=CARTESIAN_POINT ( 'NONE',  ( -190.0000000000001705, 1.836970198721007106E-15, 0.000000000000000000 ) ) ;
#16443=( BOUNDED_SURFACE ( )  B_SPLINE_SURFACE ( 3, 2, ( 
 ( #6619, #4118, #18329 ),
 ( #25003, #12342, #18868 ),
 ( #12214, #649, #20470 ),
 ( #8622, #14602, #14737 ),
 ( #20336, #22868, #2245 ),
 ( #18462, #10352, #8353 ),
 ( #110, #12612, #8217 ),
 ( #20740, #240, #16474 ),
 ( #24598, #18601, #6353 ),
 ( #4645, #12747, #8756 ),
 ( #10488, #380, #14472 ),
 ( #4381, #2509, #2651 ) ),
 .UNSPECIFIED., .F., .F., .F. ) 
 B_SPLINE_SURFACE_WITH_KNOTS ( ( 4, 2, 2, 2, 2, 4 ),
 ( 3, 3 ),
 ( 0.006022589392327087551, 0.01254516766564490668, 0.01580645680230381711, 0.01906774593896272754, 0.02559032421228054494, 0.03211290248559836580 ),
 ( 0.000000000000000000, 1.000000000000000000 ),
 .UNSPECIFIED. ) 
 GEOMETRIC_REPRESENTATION_ITEM ( )  RATIONAL_B_SPLINE_SURFACE ( (
 ( 1.000000000000000000, 0.9998834880171258988, 1.000000000000000000),
 ( 1.000000000000000000, 0.9998139205011338237, 1.000000000000000000),
 ( 1.000000000000000000, 0.9997315632445886724, 1.000000000000000000),
 ( 1.000000000000000000, 0.9996405464946352959, 1.000000000000000000),
 ( 1.000000000000000000, 0.9996155081776924023, 1.000000000000000000),
 ( 1.000000000000000000, 0.9995814087511104562, 1.000000000000000000),
 ( 1.000000000000000000, 0.9995724100939920032, 1.000000000000000000),
 ( 1.000000000000000000, 0.9995726760936896049, 1.000000000000000000),
 ( 1.000000000000000000, 0.9996103361816741639, 1.000000000000000000),
 ( 1.000000000000000000, 0.9997312749796802844, 1.000000000000000000),
 ( 1.000000000000000000, 0.9998135910914284219, 1.000000000000000000),
 ( 1.000000000000000000, 0.9998834880173383954, 1.000000000000000000) ) ) 
 REPRESENTATION_ITEM ( '' )  SURFACE ( )  );
#16445=CARTESIAN_POINT ( 'NONE',  ( 4.995406935893292655, 39.99999999999982947, 55.24977328856478209 ) ) ;
#16447=CARTESIAN_POINT ( 'NONE',  ( 22.77497178454824223, 43.17449153292937325, -17.88345994150133578 ) ) ;
#16448=CARTESIAN_POINT ( 'NONE',  ( 14.38125909742180752, 55.17850393972636880, 2.449293598294708485E-15 ) ) ;
#16449=CARTESIAN_POINT ( 'NONE',  ( -100.7734535825088358, -16.03295912088706743, -16.03295912088710296 ) ) ;
#16451=CARTESIAN_POINT ( 'NONE',  ( -4.027137536849560107, -43.00884733904522506, 23.45200847982325598 ) ) ;
#16452=CARTESIAN_POINT ( 'NONE',  ( 0.2972598230769930572, 54.33493731733936016, 2.449293598294708485E-15 ) ) ;
#16455=SPHERICAL_SURFACE ( 'NONE', #13070, 15.00000000000000000 ) ;
#16457=CARTESIAN_POINT ( 'NONE',  ( 130.8568914410475088, -52.36146031193419503, 4.207082182989537955 ) ) ;
#16458=CARTESIAN_POINT ( 'NONE',  ( -47.45115950043103226, -10.57586762654845280, 31.57405104340034541 ) ) ;
#16459=CARTESIAN_POINT ( 'NONE',  ( -3.205219349397945283, 17.96245967913786856, -43.36521377095283469 ) ) ;
#16461=CARTESIAN_POINT ( 'NONE',  ( 48.46046615278683589, -37.63122026539700471, 11.89583623203270157 ) ) ;
#16462=CARTESIAN_POINT ( 'NONE',  ( 132.4338126186516149, -29.78211700502427917, 12.33615677966322721 ) ) ;
#16463=CARTESIAN_POINT ( 'NONE',  ( -188.2507053403079738, -13.82466505297404247, 46.97353740712713233 ) ) ;
#16464=CARTESIAN_POINT ( 'NONE',  ( 57.59792236341147031, -30.00663442387662627, -26.56190807104723461 ) ) ;
#16465=CARTESIAN_POINT ( 'NONE',  ( 163.1118516004056573, 27.26290988616875310, 0.000000000000000000 ) ) ;
#16466=CARTESIAN_POINT ( 'NONE',  ( -188.2957210513887674, 13.82790368522472946, -46.98905903629629677 ) ) ;
#16467=CARTESIAN_POINT ( 'NONE',  ( 192.4448373802100889, -14.14213562375896061, 14.14213562375865330 ) ) ;
#16468=CARTESIAN_POINT ( 'NONE',  ( -208.1127848780264742, 38.89260858015707356, 17.67593391476696141 ) ) ;
#16469=CARTESIAN_POINT ( 'NONE',  ( -238.4067589809705510, -40.96449427998265946, -2.449293598294708485E-15 ) ) ;
#16470=CARTESIAN_POINT ( 'NONE',  ( -86.96347745069644475, 18.24025645688351105, 2.449293598294708485E-15 ) ) ;
#16471=CARTESIAN_POINT ( 'NONE',  ( -100.7734535825088500, -40.00000000000027711, 22.67402823373149801 ) ) ;
#16472=CARTESIAN_POINT ( 'NONE',  ( 184.8905102610680444, 13.49065550809807945, 13.49065550809809544 ) ) ;
#16474=CARTESIAN_POINT ( 'NONE',  ( -94.58360650935111380, 20.91945674502911956, -8.190527749670891922 ) ) ;
#16475=CARTESIAN_POINT ( 'NONE',  ( 163.1118516004056573, 19.27778845539265618, -37.29075403953135037 ) ) ;
#16476=CARTESIAN_POINT ( 'NONE',  ( -114.6679276626351509, -4.801621139947936712, 21.51116696530568362 ) ) ;
#16477=VERTEX_POINT ( 'NONE', #7540 ) ;
#16478=CARTESIAN_POINT ( 'NONE',  ( 200.0000000000000000, -42.42640687119293119, 14.14213562373082134 ) ) ;
#16479=CARTESIAN_POINT ( 'NONE',  ( -103.9650464692577998, 8.298274099270956938, 20.03380587467329832 ) ) ;
#16480=CARTESIAN_POINT ( 'NONE',  ( 4.995406935893305977, -39.06748935135212264, 39.06748935135171763 ) ) ;
#16481=CARTESIAN_POINT ( 'NONE',  ( -4.061681315507636114, -46.98276670624674267, -13.82654462146565777 ) ) ;
#16483=EDGE_CURVE ( 'NONE', #10709, #19077, #3696, .T. ) ;
#16485=CARTESIAN_POINT ( 'NONE',  ( 14.33519811653601472, -49.08818492847915849, -14.14278418308693475 ) ) ;
#16486=CARTESIAN_POINT ( 'NONE',  ( -199.9999999999999716, -44.86878812508714276, 24.82633483071253622 ) ) ;
#16487=ORIENTED_EDGE ( 'NONE', *, *, #225, .T. ) ;
#16489=CARTESIAN_POINT ( 'NONE',  ( -4.039451493210489907, 13.82811171175507603, -46.99046209229789639 ) ) ;
#16490=CARTESIAN_POINT ( 'NONE',  ( -208.1127848780265026, 10.60833733269537049, 10.60833733269544510 ) ) ;
#16491=CARTESIAN_POINT ( 'NONE',  ( -188.6890294954627905, -43.11788624869991793, -23.53287096354742403 ) ) ;
#16492=CARTESIAN_POINT ( 'NONE',  ( -208.1127848780264742, -40.00000000000011369, 15.00245453012655439 ) ) ;
#16493=CARTESIAN_POINT ( 'NONE',  ( -100.7734535825088358, 17.32597176626809343, 2.449293598294708485E-15 ) ) ;
#16496=CARTESIAN_POINT ( 'NONE',  ( 136.1360204305621266, 1.473277640373554421E-13, -35.03383547441296741 ) ) ;
#16497=CARTESIAN_POINT ( 'NONE',  ( -213.1075012329537230, 39.99999999999992895, 13.71589010951925935 ) ) ;
#16498=CARTESIAN_POINT ( 'NONE',  ( 170.2234770963711128, 1.169953928977015745E-13, -24.55285855007187124 ) ) ;
#16499=CARTESIAN_POINT ( 'NONE',  ( 146.6084372240433993, 34.62501878078308692, 0.000000000000000000 ) ) ;
#16500=CARTESIAN_POINT ( 'NONE',  ( -213.1075012329537230, -53.71589010950170717, 40.00000000000002132 ) ) ;
#16501=CARTESIAN_POINT ( 'NONE',  ( -208.1127848780264742, -10.60833733268345469, 67.17687982760682530 ) ) ;
#16502=CARTESIAN_POINT ( 'NONE',  ( -86.86493150571114086, -8.366608963953616751, 19.60045294882772993 ) ) ;
#16504=CARTESIAN_POINT ( 'NONE',  ( 136.1360204305621551, 40.00000000000009948, -4.966164525586641787 ) ) ;
#16505=CARTESIAN_POINT ( 'NONE',  ( 0.2972598230770030492, -1.921041075453695163E-13, 54.33493731733936016 ) ) ;
#16506=CARTESIAN_POINT ( 'NONE',  ( 163.1118516004056573, 9.006482792074356425, -47.56205970284957374 ) ) ;
#16509=CARTESIAN_POINT ( 'NONE',  ( -56.48582580120558561, -50.09629031063963112, -6.472252184284449150 ) ) ;
#16511=CARTESIAN_POINT ( 'NONE',  ( -5.152948516935869527, 42.67688069069274093, -23.23217004669248809 ) ) ;
#16513=CARTESIAN_POINT ( 'NONE',  ( -192.9588430854689705, -54.46834944099975928, -2.449293598294708485E-15 ) ) ;
#16514=DIRECTION ( 'NONE',  ( 0.000000000000000000, -0.9307566067079398042, -0.3656393565653475175 ) ) ;
#16515=CARTESIAN_POINT ( 'NONE',  ( 146.6084372240433993, -24.48358557860353457, 24.48358557860296258 ) ) ;
#16517=EDGE_LOOP ( 'NONE', ( #19666, #18039, #593, #962 ) ) ;
#16519=CARTESIAN_POINT ( 'NONE',  ( -96.94475454971987460, 9.001119816634455262, -20.58449551010242828 ) ) ;
#16520=CARTESIAN_POINT ( 'NONE',  ( 6.011245401487562923, 18.54985650214280923, 44.78331514754981413 ) ) ;
#16521=EDGE_LOOP ( 'NONE', ( #4559, #25950, #6356, #3716 ) ) ;
#16523=CARTESIAN_POINT ( 'NONE',  ( -280.0000000000000000, -20.00000000000006750, 0.000000000000000000 ) ) ;
#16526=CARTESIAN_POINT ( 'NONE',  ( -238.4067589809705794, 0.6820004457912757223, 0.6820004457913219076 ) ) ;
#16527=CARTESIAN_POINT ( 'NONE',  ( -238.4067589809705794, 28.96627169325324758, -27.60227080167054581 ) ) ;
#16528=CARTESIAN_POINT ( 'NONE',  ( -199.9999999999999432, -15.63350978565347660, 47.95319408140866813 ) ) ;
#16530=CARTESIAN_POINT ( 'NONE',  ( -93.01741312765729219, -8.946232117619631552, -20.50009083229717533 ) ) ;
#16531=CARTESIAN_POINT ( 'NONE',  ( -30.26275506840324425, 40.00000000000044764, -41.69427246844585255 ) ) ;
#16532=CARTESIAN_POINT ( 'NONE',  ( 57.59792236341147031, -1.493297263419786540E-14, 2.435789363418160658 ) ) ;
#16536=CARTESIAN_POINT ( 'NONE',  ( -188.8753211508389711, 17.93495349242735060, 43.29880796194883885 ) ) ;
#16537=CARTESIAN_POINT ( 'NONE',  ( -56.48582580120559271, 6.472252184284121412, 6.472252184284244869 ) ) ;
#16538=CARTESIAN_POINT ( 'NONE',  ( 170.2234770963711128, 17.36149277826973503, 39.20704971665401217 ) ) ;
#16540=CARTESIAN_POINT ( 'NONE',  ( 19.06497207195980792, 18.24870850772790831, -38.31983398719609824 ) ) ;
#16541=CARTESIAN_POINT ( 'NONE',  ( -199.9999999999999716, 46.84854965773192248, -17.28402242884627782 ) ) ;
#16542=CARTESIAN_POINT ( 'NONE',  ( -198.0356074513804572, -15.37879056873074290, 0.000000000000000000 ) ) ;
#16544=CARTESIAN_POINT ( 'NONE',  ( -198.0356074513804572, -15.37879056873074290, 0.000000000000000000 ) ) ;
#16545=CARTESIAN_POINT ( 'NONE',  ( -114.6980683190641628, 18.22973761981876706, 12.42092015837599739 ) ) ;
#16546=CARTESIAN_POINT ( 'NONE',  ( -162.0762913951021176, 40.00000000000042633, -41.69427287672947102 ) ) ;
#16548=CARTESIAN_POINT ( 'NONE',  ( 154.0339099654741517, -11.67508747798902391, 28.18615453125275394 ) ) ;
#16550=ADVANCED_FACE ( 'NONE', ( #21282 ), #25240, .T. ) ;
#16553=CARTESIAN_POINT ( 'NONE',  ( -213.1075012329537230, 13.71589010951907994, 0.000000000000000000 ) ) ;
#16554=B_SPLINE_CURVE_WITH_KNOTS ( 'NONE', 3,
 ( #8514, #16759, #2536, #24762, #24893, #23034, #6259, #21028, #4282, #2679, #2272, #12372, #6648, #12501, #10786, #4543, #4672, #10920, #20901, #20766, #18763, #16897, #14763, #19031, #18896, #6515, #14894, #675, #20500, #8784, #10381, #18491, #810, #10514 ),
 .UNSPECIFIED., .F., .F.,
 ( 4, 2, 2, 2, 2, 2, 2, 2, 2, 2, 2, 2, 2, 2, 2, 2, 4 ),
 ( -5.298243351207334109E-05, 0.01887868273877498990, 0.02834451532491851986, 0.03071097347145438500, 0.03307743161799024667, 0.03544388976452610834, 0.03781034791106197002, 0.04254326420413369336, 0.04727618049720541671, 0.04964263864374132001, 0.05200909679027721638, 0.05674201308334893973, 0.05910847122988479446, 0.06029170030315276346, 0.06147492937642073246, 0.06620784566949260153, 0.07567367825563635353 ),
 .UNSPECIFIED. ) ;
#16555=CARTESIAN_POINT ( 'NONE',  ( -56.48582580120559271, 21.81201906317798489, -21.81201906317746619 ) ) ;
#16556=B_SPLINE_CURVE_WITH_KNOTS ( 'NONE', 3,
 ( #16272, #4190, #2185, #18401, #6949, #23448, #720, #7207, #2720, #15067, #21067, #2974, #13208, #17445, #5346, #23197 ),
 .UNSPECIFIED., .F., .F.,
 ( 4, 2, 2, 2, 2, 2, 2, 4 ),
 ( 1.734723475976807094E-18, 0.004250215528541258399, 0.006375323292811887164, 0.008500431057082516798, 0.01275064658562377433, 0.01381320046775908784, 0.01487575434989440309, 0.01700086211416503013 ),
 .UNSPECIFIED. ) ;
#16557=CARTESIAN_POINT ( 'NONE',  ( -105.3239292022295075, -20.72686647363872581, -5.381957438748616873 ) ) ;
#16558=CARTESIAN_POINT ( 'NONE',  ( -188.2995950289364089, -13.82811170417104840, -46.99046209955525200 ) ) ;
#16559=CARTESIAN_POINT ( 'NONE',  ( -87.13361725327072804, 0.6795304812954694462, -21.49321519333428654 ) ) ;
#16562=CARTESIAN_POINT ( 'NONE',  ( -86.96347745069644475, -15.38646221621738164, -41.18208027870615240 ) ) ;
#16563=CARTESIAN_POINT ( 'NONE',  ( -192.9588430854689989, -10.23066800230742501, -10.23066800230756712 ) ) ;
#16564=DIRECTION ( 'NONE',  ( 0.000000000000000000, 1.000000000000000000, 0.000000000000000000 ) ) ;
#16565=CARTESIAN_POINT ( 'NONE',  ( -238.4067589809705794, 39.99999999999999289, -0.9644942799821634161 ) ) ;
#16566=CARTESIAN_POINT ( 'NONE',  ( -213.1075012329537230, -37.98287015391257881, 18.58567234101111509 ) ) ;
#16567=DIRECTION ( 'NONE',  ( -0.01051738777841135231, 0.9166396752739897069, 0.3995761382614246848 ) ) ;
#16569=CARTESIAN_POINT ( 'NONE',  ( 14.38125909742181285, -10.73282306404727393, 10.73282306404716380 ) ) ;
#16571=CIRCLE ( 'NONE', #25511, 14.99999999999999467 ) ;
#16573=CARTESIAN_POINT ( 'NONE',  ( 163.1118516004056573, -40.00000000000003553, 12.73709011382460687 ) ) ;
#16575=CARTESIAN_POINT ( 'NONE',  ( 17.65190073994223852, 44.23515346912816426, -24.35922420889879447 ) ) ;
#16576=CARTESIAN_POINT ( 'NONE',  ( 170.2234770963711128, 15.44714144992819627, -40.00000000000002132 ) ) ;
#16577=CARTESIAN_POINT ( 'NONE',  ( 130.8568914410475372, 34.05028731879791337, 0.000000000000000000 ) ) ;
#16578=CARTESIAN_POINT ( 'NONE',  ( 146.6084372240433709, -34.62501878078303008, 40.00000000000002132 ) ) ;
#16579=CARTESIAN_POINT ( 'NONE',  ( -4.112199523540559731, -42.98379141459074049, 23.43514144949434552 ) ) ;
#16580=CARTESIAN_POINT ( 'NONE',  ( 19.06497207195980792, 54.19242893257844429, 40.00000000000002132 ) ) ;
#16582=CARTESIAN_POINT ( 'NONE',  ( -3.555049149807541387, 23.55301256057208903, -43.14507846637719979 ) ) ;
#16583=CARTESIAN_POINT ( 'NONE',  ( 146.6084372240433993, -24.48358557860319706, -24.48358557860330720 ) ) ;
#16584=CARTESIAN_POINT ( 'NONE',  ( -4.031723327955644365, -13.82865651623139769, 46.99313739789381117 ) ) ;
#16586=CARTESIAN_POINT ( 'NONE',  ( 3.869409319524869773, 14.12455301876681268, -48.96737585071113585 ) ) ;
#16590=CARTESIAN_POINT ( 'NONE',  ( -188.3611024622156833, -23.46270902204734909, 43.02327292322546981 ) ) ;
#16591=( BOUNDED_SURFACE ( )  B_SPLINE_SURFACE ( 3, 3, ( 
 ( #25261, #12883, #15132, #23263, #5039, #1040, #9141, #13269, #25393, #7144, #21391, #15260, #23389, #3164, #23509, #13388, #21515, #3288, #11385, #24162, #12051, #3676, #21899, #13772, #25906, #5666, #10060, #3953, #11784, #19904 ),
 ( #26179, #7919, #21769, #16036, #22044, #25773, #17629, #21638, #3542, #9792, #1952, #1688, #17895, #13514, #1422, #25646, #7523, #24023, #15631, #7392, #9923, #15503, #23633, #26043, #5537, #5802, #5938, #1555, #7780, #9523 ),
 ( #5412, #15896, #13909, #3817, #23756, #19639, #11920, #22179, #20042, #1821, #11513, #18029, #11642, #14045, #20170, #3412, #13643, #19764, #9660, #17764, #7647, #15761, #23890, #2218, #4478, #16573, #22703, #486, #24704, #20440 ),
 ( #12580, #4352, #2086, #18703, #82, #18570, #14447, #8320, #6458, #6587, #12314, #8593, #16703, #14311, #24835, #14574, #18296, #10193, #14176, #22445, #2345, #20840, #24569, #6325, #6074, #20309, #2615, #8192, #20710, #16308 ),
 ( #4225, #350, #8454, #12187, #10327, #18436, #4616, #24432, #22310, #14708, #211, #18166, #10457, #2476, #10588, #6199, #16445, #22841, #12712, #22574, #26313, #4086, #8056, #12444, #16172, #20573, #24307, #25364, #21483, #23233 ),
 ( #13115, #3010, #18974, #7119, #16842, #15361, #15229, #9249, #21105, #23360, #5137, #2885, #13242, #19231, #23484, #4748, #5259, #1011, #19102, #18840, #21236, #886, #8995, #9114, #8858, #13361, #1144, #10856, #25491, #4879 ),
 ( #16970, #10728, #25232, #8724, #618, #25106, #12983, #21367, #11117, #11237, #6855, #24975, #3135, #14972, #6724, #23107, #10993, #17099, #6984, #14836, #17225, #22969, #5010, #19355, #15099, #17356, #12854, #7240, #20972, #2753 ) ),
 .UNSPECIFIED., .T., .F., .T. ) 
 B_SPLINE_SURFACE_WITH_KNOTS ( ( 4, 3, 4 ),
 ( 4, 2, 2, 2, 2, 2, 2, 2, 2, 2, 2, 2, 2, 2, 4 ),
 ( 0.000000000000000000, 0.5000000000000000000, 1.000000000000000000 ),
 ( 0.000000000000000000, 0.1357259735107005372, 0.1651108541090157700, 0.1944957347073310028, 0.3598804999793158710, 0.3867117631979620773, 0.4135430264166082281, 0.5789277916885930964, 0.6062785021374117456, 0.6336292125862302838, 0.8508620842112317728, 0.8814014469398914198, 0.9119408096685510667, 0.9559704048342755334, 1.000000000000000000 ),
 .UNSPECIFIED. ) 
 GEOMETRIC_REPRESENTATION_ITEM ( )  RATIONAL_B_SPLINE_SURFACE ( (
 ( 1.000000000000000000, 1.000000000000000000, 1.000000000000000000, 1.000000000000000000, 1.000000000000000000, 1.000000000000000000, 1.000000000000000000, 1.000000000000000000, 1.000000000000000000, 1.000000000000000000, 1.000000000000000000, 1.000000000000000000, 1.000000000000000000, 1.000000000000000000, 1.000000000000000000, 1.000000000000000000, 1.000000000000000000, 1.000000000000000000, 1.000000000000000000, 1.000000000000000000, 1.000000000000000000, 1.000000000000000000, 1.000000000000000000, 1.000000000000000000, 1.000000000000000000, 1.000000000000000000, 1.000000000000000000, 1.000000000000000000, 1.000000000000000000, 1.000000000000000000),
 ( 0.3333333333333333703, 0.3333333333333333703, 0.3333333333333333703, 0.3333333333333333703, 0.3333333333333333703, 0.3333333333333333703, 0.3333333333333333703, 0.3333333333333333703, 0.3333333333333333703, 0.3333333333333333703, 0.3333333333333333703, 0.3333333333333333703, 0.3333333333333333703, 0.3333333333333333703, 0.3333333333333333703, 0.3333333333333333703, 0.3333333333333333703, 0.3333333333333333703, 0.3333333333333333703, 0.3333333333333333703, 0.3333333333333333703, 0.3333333333333333703, 0.3333333333333333703, 0.3333333333333333703, 0.3333333333333333703, 0.3333333333333333703, 0.3333333333333333703, 0.3333333333333333703, 0.3333333333333333703, 0.3333333333333333703),
 ( 0.3333333333333333703, 0.3333333333333333703, 0.3333333333333333703, 0.3333333333333333703, 0.3333333333333333703, 0.3333333333333333703, 0.3333333333333333703, 0.3333333333333333703, 0.3333333333333333703, 0.3333333333333333703, 0.3333333333333333703, 0.3333333333333333703, 0.3333333333333333703, 0.3333333333333333703, 0.3333333333333333703, 0.3333333333333333703, 0.3333333333333333703, 0.3333333333333333703, 0.3333333333333333703, 0.3333333333333333703, 0.3333333333333333703, 0.3333333333333333703, 0.3333333333333333703, 0.3333333333333333703, 0.3333333333333333703, 0.3333333333333333703, 0.3333333333333333703, 0.3333333333333333703, 0.3333333333333333703, 0.3333333333333333703),
 ( 1.000000000000000000, 1.000000000000000000, 1.000000000000000000, 1.000000000000000000, 1.000000000000000000, 1.000000000000000000, 1.000000000000000000, 1.000000000000000000, 1.000000000000000000, 1.000000000000000000, 1.000000000000000000, 1.000000000000000000, 1.000000000000000000, 1.000000000000000000, 1.000000000000000000, 1.000000000000000000, 1.000000000000000000, 1.000000000000000000, 1.000000000000000000, 1.000000000000000000, 1.000000000000000000, 1.000000000000000000, 1.000000000000000000, 1.000000000000000000, 1.000000000000000000, 1.000000000000000000, 1.000000000000000000, 1.000000000000000000, 1.000000000000000000, 1.000000000000000000),
 ( 0.3333333333333333703, 0.3333333333333333703, 0.3333333333333333703, 0.3333333333333333703, 0.3333333333333333703, 0.3333333333333333703, 0.3333333333333333703, 0.3333333333333333703, 0.3333333333333333703, 0.3333333333333333703, 0.3333333333333333703, 0.3333333333333333703, 0.3333333333333333703, 0.3333333333333333703, 0.3333333333333333703, 0.3333333333333333703, 0.3333333333333333703, 0.3333333333333333703, 0.3333333333333333703, 0.3333333333333333703, 0.3333333333333333703, 0.3333333333333333703, 0.3333333333333333703, 0.3333333333333333703, 0.3333333333333333703, 0.3333333333333333703, 0.3333333333333333703, 0.3333333333333333703, 0.3333333333333333703, 0.3333333333333333703),
 ( 0.3333333333333333703, 0.3333333333333333703, 0.3333333333333333703, 0.3333333333333333703, 0.3333333333333333703, 0.3333333333333333703, 0.3333333333333333703, 0.3333333333333333703, 0.3333333333333333703, 0.3333333333333333703, 0.3333333333333333703, 0.3333333333333333703, 0.3333333333333333703, 0.3333333333333333703, 0.3333333333333333703, 0.3333333333333333703, 0.3333333333333333703, 0.3333333333333333703, 0.3333333333333333703, 0.3333333333333333703, 0.3333333333333333703, 0.3333333333333333703, 0.3333333333333333703, 0.3333333333333333703, 0.3333333333333333703, 0.3333333333333333703, 0.3333333333333333703, 0.3333333333333333703, 0.3333333333333333703, 0.3333333333333333703),
 ( 1.000000000000000000, 1.000000000000000000, 1.000000000000000000, 1.000000000000000000, 1.000000000000000000, 1.000000000000000000, 1.000000000000000000, 1.000000000000000000, 1.000000000000000000, 1.000000000000000000, 1.000000000000000000, 1.000000000000000000, 1.000000000000000000, 1.000000000000000000, 1.000000000000000000, 1.000000000000000000, 1.000000000000000000, 1.000000000000000000, 1.000000000000000000, 1.000000000000000000, 1.000000000000000000, 1.000000000000000000, 1.000000000000000000, 1.000000000000000000, 1.000000000000000000, 1.000000000000000000, 1.000000000000000000, 1.000000000000000000, 1.000000000000000000, 1.000000000000000000) ) ) 
 REPRESENTATION_ITEM ( '' )  SURFACE ( )  );
#16592=CARTESIAN_POINT ( 'NONE',  ( -100.7734535825088358, -16.03295912088728770, 16.03295912088687913 ) ) ;
#16593=CARTESIAN_POINT ( 'NONE',  ( -162.0762913951020892, -1.694272876828353702, 0.000000000000000000 ) ) ;
#16594=CARTESIAN_POINT ( 'NONE',  ( -188.2652746676673701, 13.82569223136002279, -46.97858116095154202 ) ) ;
#16595=CARTESIAN_POINT ( 'NONE',  ( 163.1118516004056573, 9.006482792069759213, -9.006482792069505194 ) ) ;
#16596=CARTESIAN_POINT ( 'NONE',  ( 4.995406935893289102, 10.78321810389013002, -10.78321810388986712 ) ) ;
#16597=CARTESIAN_POINT ( 'NONE',  ( -192.9588430854689705, -54.46834944099975928, -2.449293598294708485E-15 ) ) ;
#16598=CARTESIAN_POINT ( 'NONE',  ( -198.0356074513804572, 55.37879056873070027, 2.449293598294708485E-15 ) ) ;
#16599=CARTESIAN_POINT ( 'NONE',  ( 170.2234770963711128, -40.00000000000024158, 24.55285855007145202 ) ) ;
#16600=CARTESIAN_POINT ( 'NONE',  ( 91.82158438592158234, 16.11829626346139577, 16.11829626346143840 ) ) ;
#16601=CARTESIAN_POINT ( 'NONE',  ( 98.29820294267349823, -4.524526698162719462, 19.49240851342997161 ) ) ;
#16602=CARTESIAN_POINT ( 'NONE',  ( 170.2234770963711128, 45.64576402573196390, -10.92277846919159856 ) ) ;
#16603=CARTESIAN_POINT ( 'NONE',  ( -238.4067589809705794, -0.6820004457913680929, 0.6820004457913170226 ) ) ;
#16604=ORIENTED_EDGE ( 'NONE', *, *, #17195, .T. ) ;
#16605=CARTESIAN_POINT ( 'NONE',  ( -280.0000000000000000, -14.14213562373098831, -14.14213562373098654 ) ) ;
#16607=CARTESIAN_POINT ( 'NONE',  ( -189.2428623074473535, -13.87687453620301348, -47.31877164625541354 ) ) ;
#16608=CARTESIAN_POINT ( 'NONE',  ( -208.1127848780264742, -10.60833733268345469, 67.17687982760682530 ) ) ;
#16609=CARTESIAN_POINT ( 'NONE',  ( -0.6848998192525614925, -43.87669161505422721, -24.09453515736277041 ) ) ;
#16611=CARTESIAN_POINT ( 'NONE',  ( 146.6084372240433993, -34.62501878078303008, 0.000000000000000000 ) ) ;
#16616=CARTESIAN_POINT ( 'NONE',  ( -192.6563370916107374, -44.11756948123341715, -18.27409561805956173 ) ) ;
#16618=CARTESIAN_POINT ( 'NONE',  ( -86.96347745069644475, -8.210974027862429531E-14, 18.24025645688352881 ) ) ;
#16619=CARTESIAN_POINT ( 'NONE',  ( 146.6084372240433993, 5.374981219216999229, 2.449293598294708485E-15 ) ) ;
#16625=CARTESIAN_POINT ( 'NONE',  ( 0.2972598230770030492, -1.921041075453695163E-13, 54.33493731733936016 ) ) ;
#16626=CARTESIAN_POINT ( 'NONE',  ( -86.96347745069645896, 39.99999999999994316, 18.24025645688366737 ) ) ;
#16628=CARTESIAN_POINT ( 'NONE',  ( -259.2033419157646676, 9.517827891722582478, -40.00000000000002132 ) ) ;
#16629=EDGE_CURVE ( 'NONE', #12261, #21267, #6746, .T. ) ;
#16630=CARTESIAN_POINT ( 'NONE',  ( 4.995406935893307754, -55.24977328853207581, -40.00000000000002132 ) ) ;
#16632=CARTESIAN_POINT ( 'NONE',  ( -100.7734535825088500, 16.03295912088683295, 40.53558337403684675 ) ) ;
#16633=CARTESIAN_POINT ( 'NONE',  ( -86.96347745069644475, -2.438961472018186339E-13, 21.75974354311649961 ) ) ;
#16634=CARTESIAN_POINT ( 'NONE',  ( -114.4364955367320249, 20.04994829327449679, -8.644468109213075735 ) ) ;
#16635=CARTESIAN_POINT ( 'NONE',  ( -192.9588430854689989, 5.375290060580374156E-13, -54.46834944099972375 ) ) ;
#16636=CARTESIAN_POINT ( 'NONE',  ( -162.0762913951021176, -40.00000000000019895, 41.69427287672974813 ) ) ;
#16639=CARTESIAN_POINT ( 'NONE',  ( -114.4944481313176112, -9.302331659126325647, 19.81806240209552783 ) ) ;
#16640=CARTESIAN_POINT ( 'NONE',  ( 184.8905102610680444, -13.49065550809780412, -43.07788698682583828 ) ) ;
#16642=CARTESIAN_POINT ( 'NONE',  ( -86.86493150571118349, -7.943527260495776510, -19.77569912839190280 ) ) ;
#16643=CARTESIAN_POINT ( 'NONE',  ( 121.8740240556054459, 26.81399039734628076, -11.10671848392266092 ) ) ;
#16644=CARTESIAN_POINT ( 'NONE',  ( -91.56559293963834989, -17.32597176626812896, -2.449293598294708485E-15 ) ) ;
#16646=CARTESIAN_POINT ( 'NONE',  ( -192.9588430854689989, 14.46834944099965981, 0.000000000000000000 ) ) ;
#16648=ORIENTED_EDGE ( 'NONE', *, *, #3372, .T. ) ;
#16650=CARTESIAN_POINT ( 'NONE',  ( -109.1264249741457348, 13.72187187126464991, 33.12752917268250741 ) ) ;
#16651=CARTESIAN_POINT ( 'NONE',  ( -94.58360650938178082, 9.000712009840871275, -20.58386743644488703 ) ) ;
#16652=CARTESIAN_POINT ( 'NONE',  ( 8.209392600932645223, 24.84362085273527043, 44.89226883836252568 ) ) ;
#16653=EDGE_LOOP ( 'NONE', ( #8463, #15327, #5323, #20342 ) ) ;
#16655=CARTESIAN_POINT ( 'NONE',  ( 136.1360204305621266, -24.77266263493116583, -24.77266263493127951 ) ) ;
#16657=CARTESIAN_POINT ( 'NONE',  ( -110.0471271033544269, -6.849398635777247613, 18.98461286765427758 ) ) ;
#16658=FACE_OUTER_BOUND ( 'NONE', #328, .T. ) ;
#16659=DIRECTION ( 'NONE',  ( 0.9698969544100265461, -0.09318942522532003281, -0.2249791742635964820 ) ) ;
#16660=DIRECTION ( 'NONE',  ( 0.000000000000000000, 1.000000000000000000, 0.000000000000000000 ) ) ;
#16662=CARTESIAN_POINT ( 'NONE',  ( 151.7948205124836534, 39.99999999999970157, 33.23291073765595627 ) ) ;
#16663=CARTESIAN_POINT ( 'NONE',  ( -56.48582580120560692, 39.99999999999991473, 9.153146818114004546 ) ) ;
#16666=CARTESIAN_POINT ( 'NONE',  ( -86.86493150571116928, 8.366608963953661160, 19.60045294882771572 ) ) ;
#16668=CARTESIAN_POINT ( 'NONE',  ( -188.6889827002360960, 23.53286111060924313, 43.11787295909677908 ) ) ;
#16669=CARTESIAN_POINT ( 'NONE',  ( 14.38125909742181285, -10.73282306404712472, -10.73282306404731301 ) ) ;
#16670=CARTESIAN_POINT ( 'NONE',  ( -96.93773665439030651, 9.001171854901906855, 20.58457565566410352 ) ) ;
#16671=CARTESIAN_POINT ( 'NONE',  ( -135.8532207217289738, 6.472252184283881604, 50.09629031063969506 ) ) ;
#16672=CARTESIAN_POINT ( 'NONE',  ( 98.29820294267865677, -17.41560179325844615, 10.21753654889059781 ) ) ;
#16673=CARTESIAN_POINT ( 'NONE',  ( 136.1360204305621551, 24.77266263493153176, -31.79587985999237887 ) ) ;
#16674=CARTESIAN_POINT ( 'NONE',  ( -200.0000000000000568, 47.66874763508950963, -16.05666331275189762 ) ) ;
#16675=CARTESIAN_POINT ( 'NONE',  ( -30.26275506840324070, -1.694272468446265112, 0.000000000000000000 ) ) ;
#16676=CARTESIAN_POINT ( 'NONE',  ( 170.2234770963711128, -17.36149277827010096, 17.36149277826970660 ) ) ;
#16677=CARTESIAN_POINT ( 'NONE',  ( 14.38125909742181285, -15.17850393972633505, 0.000000000000000000 ) ) ;
#16679=CARTESIAN_POINT ( 'NONE',  ( 0.2972598230770030492, 5.716321584140269555E-13, -54.33493731733936016 ) ) ;
#16681=CARTESIAN_POINT ( 'NONE',  ( 130.8888609958233360, -12.21841679119747681, 29.49786752803523626 ) ) ;
#16684=CARTESIAN_POINT ( 'NONE',  ( -162.0762913951020892, 1.694272876828294194, 0.000000000000000000 ) ) ;
#16686=CARTESIAN_POINT ( 'NONE',  ( 130.8568914410475088, 32.49135343045448820, 24.07718906446946860 ) ) ;
#16687=CARTESIAN_POINT ( 'NONE',  ( -105.2109270643573922, -21.45728911406257922, 1.359352815171848361 ) ) ;
#16688=CARTESIAN_POINT ( 'NONE',  ( -138.9613193425325619, 10.11110876495220090, -29.42718875726376382 ) ) ;
#16692=CARTESIAN_POINT ( 'NONE',  ( 184.8905102610680444, -14.79361573936330565, -41.77492675556016621 ) ) ;
#16693=CARTESIAN_POINT ( 'NONE',  ( -135.8532207217289738, 6.472252184284096543, 6.472252184284234211 ) ) ;
#16694=DIRECTION ( 'NONE',  ( 0.000000000000000000, 0.3995982397861173041, -0.9166903767138807613 ) ) ;
#16695=CARTESIAN_POINT ( 'NONE',  ( 163.1118516004056573, -2.556006622855449647E-13, 27.26290988616872824 ) ) ;
#16696=CARTESIAN_POINT ( 'NONE',  ( 19.06497207195981147, -10.03556273973425483, -10.03556273973443247 ) ) ;
#16698=CARTESIAN_POINT ( 'NONE',  ( 22.40986519363267959, 13.85314893102515477, 47.15972762675168894 ) ) ;
#16700=CARTESIAN_POINT ( 'NONE',  ( -86.96347745069644475, -12.89780903124413491, 12.89780903124398037 ) ) ;
#16703=CARTESIAN_POINT ( 'NONE',  ( -86.96347745069644475, -8.210974027862429531E-14, 18.24025645688352881 ) ) ;
#16705=CARTESIAN_POINT ( 'NONE',  ( 21.60666276258112717, 43.47550165074678574, -18.00814241470989430 ) ) ;
#16706=CARTESIAN_POINT ( 'NONE',  ( 0.2972598230769930572, 14.33493731733933352, 0.000000000000000000 ) ) ;
#16707=CARTESIAN_POINT ( 'NONE',  ( -162.0762913951021176, -27.08623940707624911, 29.48230308784761888 ) ) ;
#16708=CARTESIAN_POINT ( 'NONE',  ( 14.38125909742180752, 55.17850393974265444, 40.00000000000002132 ) ) ;
#16709=CARTESIAN_POINT ( 'NONE',  ( -39.84211263202143272, -32.75097567523309294, 13.56589830563916088 ) ) ;
#16710=CARTESIAN_POINT ( 'NONE',  ( 200.0000000000000000, 19.99999999999995737, 40.00000000000002132 ) ) ;
#16711=EDGE_CURVE ( 'NONE', #13429, #3360, #15319, .T. ) ;
#16714=CARTESIAN_POINT ( 'NONE',  ( 184.8905102610680444, -14.79361573936379415, -14.79361573936387941 ) ) ;
#16715=CARTESIAN_POINT ( 'NONE',  ( -4.151555265633880332, -13.82020782288870109, 46.95165237382999379 ) ) ;
#16716=CARTESIAN_POINT ( 'NONE',  ( -3.921555385250235393, 13.83441994316400958, -47.03297225793206593 ) ) ;
#16718=CARTESIAN_POINT ( 'NONE',  ( -86.96347745069644475, 12.89780903124349898, 43.67073346367994446 ) ) ;
#16721=CARTESIAN_POINT ( 'NONE',  ( -190.5535808404529234, -18.10342626500561991, 43.70553721439956263 ) ) ;
#16722=CARTESIAN_POINT ( 'NONE',  ( 136.1360204305621266, -3.419521671106983309E-13, 35.03383547441296741 ) ) ;
#16723=ADVANCED_FACE ( 'NONE', ( #6413 ), #10683, .T. ) ;
#16724=CARTESIAN_POINT ( 'NONE',  ( 130.8568914410475088, -52.36146031193413108, -4.207082182990267150 ) ) ;
#16725=CARTESIAN_POINT ( 'NONE',  ( 136.1360204305621266, 24.77266263493104148, 24.77266263493145004 ) ) ;
#16726=CARTESIAN_POINT ( 'NONE',  ( -200.5022929845067949, 18.58571294254510065, -44.86988025226708743 ) ) ;
#16727=CARTESIAN_POINT ( 'NONE',  ( -56.48582580120559982, 50.09629031063956717, 6.472252184284792875 ) ) ;
#16728=CARTESIAN_POINT ( 'NONE',  ( -105.3755690713226727, -15.38646221621807619, 15.38646221621768362 ) ) ;
#16729=CARTESIAN_POINT ( 'NONE',  ( 0.2972598230770130412, -54.33493731733936016, -2.449293598294708485E-15 ) ) ;
#16730=CARTESIAN_POINT ( 'NONE',  ( 14.38125909742180752, 55.17850393974265444, 40.00000000000002132 ) ) ;
#16731=CARTESIAN_POINT ( 'NONE',  ( -208.1127848780264742, -39.99999999999990763, -15.00245453012711394 ) ) ;
#16732=CARTESIAN_POINT ( 'NONE',  ( -100.7734535825088500, 12.25131212657490209, -44.31723036834897300 ) ) ;
#16734=CARTESIAN_POINT ( 'NONE',  ( 170.2234770963711128, 17.36149277827028925, -39.20704971665377059 ) ) ;
#16735=CARTESIAN_POINT ( 'NONE',  ( 184.8905102610680444, 43.07788698682572459, 13.49065550809829439 ) ) ;
#16737=CARTESIAN_POINT ( 'NONE',  ( -213.1075012329537230, 9.698598906462684965, 66.26714140138669507 ) ) ;
#16738=CARTESIAN_POINT ( 'NONE',  ( -88.37877758188305677, 8.026456973721797894, 20.15391234940723564 ) ) ;
#16739=CARTESIAN_POINT ( 'NONE',  ( -238.4067589809705794, 27.60227080167040370, 28.96627169325338613 ) ) ;
#16740=CARTESIAN_POINT ( 'NONE',  ( -3.443169733045819303, -43.30433998020570385, -17.93724492941698401 ) ) ;
#16742=CARTESIAN_POINT ( 'NONE',  ( -1.828631717626211906, -47.79123445063621745, -13.94691770768551287 ) ) ;
#16743=FACE_OUTER_BOUND ( 'NONE', #792, .T. ) ;
#16746=CARTESIAN_POINT ( 'NONE',  ( -114.7537493279903202, -21.97305528828601595, -2.780162309559761180 ) ) ;
#16747=( BOUNDED_CURVE ( )  B_SPLINE_CURVE ( 3, ( #2328, #16429, #8177, #8439, #10439, #10572, #24686 ),
 .UNSPECIFIED., .F., .F. ) 
 B_SPLINE_CURVE_WITH_KNOTS ( ( 4, 3, 4 ),
 ( 0.007504510840757329035, 0.02318599846099227146, 0.03886748608123005710 ),
 .UNSPECIFIED. ) 
 CURVE ( )  GEOMETRIC_REPRESENTATION_ITEM ( )  RATIONAL_B_SPLINE_CURVE ( ( 0.5852718452494382051, 0.6660804010233934980, 0.8043231192735807999, 1.000000000000000000, 0.8043231192735453838, 0.6660804010233435379, 0.5852718452493943513 ) ) 
 REPRESENTATION_ITEM ( '' )  );
#16748=CARTESIAN_POINT ( 'NONE',  ( 136.1360204305621551, 4.966164525587085876, 40.00000000000002132 ) ) ;
#16751=CARTESIAN_POINT ( 'NONE',  ( -198.0356074513804572, -39.15871834505931304, 17.40982414986437377 ) ) ;
#16752=CARTESIAN_POINT ( 'NONE',  ( -208.1127848780264742, 39.99999999999979394, 55.00245453010936103 ) ) ;
#16753=CARTESIAN_POINT ( 'NONE',  ( 91.82158438592156813, 40.00000000000009948, -17.20528682183286051 ) ) ;
#16755=CARTESIAN_POINT ( 'NONE',  ( -198.0356074513804572, -15.37879056873074290, -40.00000000000002132 ) ) ;
#16757=CARTESIAN_POINT ( 'NONE',  ( -105.3755690713226727, -18.24025645688354302, -2.449293598294708485E-15 ) ) ;
#16758=CARTESIAN_POINT ( 'NONE',  ( 200.0000000000000000, 14.14213562373083022, 42.42640687119289566 ) ) ;
#16759=CARTESIAN_POINT ( 'NONE',  ( 104.1600437297060893, -8.548029202226684831, -20.63676802882099892 ) ) ;
#16760=CARTESIAN_POINT ( 'NONE',  ( -105.2833435977142500, 11.73665196259849708, -17.94452063501608663 ) ) ;
#16761=CARTESIAN_POINT ( 'NONE',  ( 130.8568914410475088, 39.99999999999969447, 34.05028731879830417 ) ) ;
#16762=CARTESIAN_POINT ( 'NONE',  ( -280.0000000000000000, -1.237140859393462838E-13, 20.00000000000001421 ) ) ;
#16764=DIRECTION ( 'NONE',  ( 0.9352143328345496887, -0.1355013631513355687, 0.3271292286619436052 ) ) ;
#16766=CARTESIAN_POINT ( 'NONE',  ( -30.26275506840322294, -57.76657404653985139, 1.198031551615709844 ) ) ;
#16767=ORIENTED_EDGE ( 'NONE', *, *, #7337, .F. ) ;
#16768=CARTESIAN_POINT ( 'NONE',  ( -77.65678946166498520, -4.464169626397992197, -21.58828686264906693 ) ) ;
#16769=CARTESIAN_POINT ( 'NONE',  ( -40.07203023074529114, 32.10811084139960059, -16.33025453620214051 ) ) ;
#16771=CARTESIAN_POINT ( 'NONE',  ( -259.2033419157646676, -30.48217210827743884, -40.00000000000002132 ) ) ;
#16773=CARTESIAN_POINT ( 'NONE',  ( -87.01701082927776554, -5.374668562248246850, -20.73853774320201637 ) ) ;
#16774=CARTESIAN_POINT ( 'NONE',  ( -280.0000000000000000, -14.14213562373118549, 14.14213562373078936 ) ) ;
#16776=ORIENTED_EDGE ( 'NONE', *, *, #22503, .F. ) ;
#16777=DIRECTION ( 'NONE',  ( 0.000000000000000000, 1.000000000000000000, 0.000000000000000000 ) ) ;
#16778=CARTESIAN_POINT ( 'NONE',  ( -105.4732637872226633, 8.153770687239410009, -19.68494377761406611 ) ) ;
#16779=CARTESIAN_POINT ( 'NONE',  ( 8.273828130718225538, 18.58906013840518057, 44.87796109789316290 ) ) ;
#16783=CARTESIAN_POINT ( 'NONE',  ( 163.1118516004056573, -47.56205970284957374, 9.006482792074162802 ) ) ;
#16785=CARTESIAN_POINT ( 'NONE',  ( -105.2053629887847421, 0.6703845944306704441, 21.49364769381508822 ) ) ;
#16787=CARTESIAN_POINT ( 'NONE',  ( 0.2972598230769990524, -18.14793986248724522, 38.42060263243662632 ) ) ;
#16789=CARTESIAN_POINT ( 'NONE',  ( 146.6084372240433709, 40.00000000000003553, 5.374981219217116468 ) ) ;
#16790=CARTESIAN_POINT ( 'NONE',  ( -90.07798792367796636, 6.122142489605069318E-14, -22.27377874500495381 ) ) ;
#16792=CARTESIAN_POINT ( 'NONE',  ( -162.0762913951020892, 4.094006889353306706E-13, -41.69427287682835015 ) ) ;
#16794=CARTESIAN_POINT ( 'NONE',  ( -213.1075012329537230, 40.00000000000012790, -13.71589010951869980 ) ) ;
#16798=CARTESIAN_POINT ( 'NONE',  ( -174.2681662550721171, 16.26527976854427493, 39.26785901291280112 ) ) ;
#16799=CARTESIAN_POINT ( 'NONE',  ( -86.96347745069645896, -12.89780903124443689, 43.67073346367968156 ) ) ;
#16801=CARTESIAN_POINT ( 'NONE',  ( 184.8905102610680444, 14.79361573936366092, 41.77492675556006674 ) ) ;
#16805=CARTESIAN_POINT ( 'NONE',  ( 184.8905102610680444, 43.07788698682591644, -13.49065550809769221 ) ) ;
#16807=CARTESIAN_POINT ( 'NONE',  ( 199.9999999999999432, 20.00000000000013856, 0.000000000000000000 ) ) ;
#16808=CARTESIAN_POINT ( 'NONE',  ( -86.96347745069644475, 12.89780903124349898, 43.67073346367994446 ) ) ;
#16809=CARTESIAN_POINT ( 'NONE',  ( 170.2234770963711128, -15.44714144992813409, 40.00000000000002132 ) ) ;
#16811=VERTEX_POINT ( 'NONE', #6544 ) ;
#16812=CARTESIAN_POINT ( 'NONE',  ( -56.48582580120558561, 3.151766524733697544E-13, -30.84685318188644132 ) ) ;
#16814=CARTESIAN_POINT ( 'NONE',  ( 156.5537079553356818, -11.28159757857240919, 27.23618587942422309 ) ) ;
#16817=CARTESIAN_POINT ( 'NONE',  ( 19.06497207195980792, 54.19242893257844429, 40.00000000000002132 ) ) ;
#16818=EDGE_CURVE ( 'NONE', #12261, #15079, #21499, .T. ) ;
#16822=CARTESIAN_POINT ( 'NONE',  ( -110.0368417077420986, -18.74474319001871336, 7.441767003031916516 ) ) ;
#16823=B_SPLINE_CURVE_WITH_KNOTS ( 'NONE', 3,
 ( #8533, #828, #19175, #6665, #959, #22911 ),
 .UNSPECIFIED., .F., .F.,
 ( 4, 2, 4 ),
 ( -0.0001324603514649706955, 0.04003639359266478182, 0.08020524753679453278 ),
 .UNSPECIFIED. ) ;
#16824=CARTESIAN_POINT ( 'NONE',  ( 165.3321726437878283, -18.76308274334254378, -18.76308274334263615 ) ) ;
#16825=CARTESIAN_POINT ( 'NONE',  ( -198.0012279766650352, 14.15883993157184761, -49.19397028317932552 ) ) ;
#16830=CARTESIAN_POINT ( 'NONE',  ( 14.38125909742181463, 10.73282306403652875, -67.30136555895941797 ) ) ;
#16831=CARTESIAN_POINT ( 'NONE',  ( 192.4448373802101173, -14.14213562370342281, 42.42640687122062104 ) ) ;
#16832=B_SPLINE_CURVE_WITH_KNOTS ( 'NONE', 3,
 ( #20426, #22296, #12699, #6444, #16825, #18824 ),
 .UNSPECIFIED., .F., .F.,
 ( 4, 2, 4 ),
 ( -5.998616621412680422E-08, 0.005995031700373287635, 0.01199012338691278837 ),
 .UNSPECIFIED. ) ;
#16833=CARTESIAN_POINT ( 'NONE',  ( -105.3174728402125453, -18.50892203404854897, -10.86052875576579346 ) ) ;
#16834=CARTESIAN_POINT ( 'NONE',  ( 151.7948205124836250, -3.202120068677277203E-13, 33.23291073765553705 ) ) ;
#16835=CIRCLE ( 'NONE', #5364, 14.99999999999999822 ) ;
#16836=CARTESIAN_POINT ( 'NONE',  ( -238.4067589809705794, -0.6820004457913585449, -0.6820004457913265705 ) ) ;
#16838=CARTESIAN_POINT ( 'NONE',  ( -188.2995950289364089, -23.44932284465861727, -43.00522595870986464 ) ) ;
#16839=CARTESIAN_POINT ( 'NONE',  ( 4.995406935893305977, -39.06748935135212264, 39.06748935135171763 ) ) ;
#16842=CARTESIAN_POINT ( 'NONE',  ( -208.1127848780264742, 39.99999999999992895, 15.00245453012683683 ) ) ;
#16843=CARTESIAN_POINT ( 'NONE',  ( 44.82887508604880367, 36.15717056697129550, -18.94256811184066081 ) ) ;
#16844=CARTESIAN_POINT ( 'NONE',  ( -280.0000000000000000, -20.00000000000006750, 0.000000000000000000 ) ) ;
#16845=CARTESIAN_POINT ( 'NONE',  ( 170.2234770963711128, -17.36149277826985937, -17.36149277826995174 ) ) ;
#16846=CARTESIAN_POINT ( 'NONE',  ( 91.82158438592158234, -17.20528682183298486, 0.000000000000000000 ) ) ;
#16848=CARTESIAN_POINT ( 'NONE',  ( 9.006212071516715767, -49.32687279762742349, 14.17897189020562188 ) ) ;
#16849=CARTESIAN_POINT ( 'NONE',  ( 184.8905102610680444, -20.92133201514440799, 40.00000000000002132 ) ) ;
#16852=CARTESIAN_POINT ( 'NONE',  ( 23.37394308801978937, 23.33966569535129310, -42.85717664514559999 ) ) ;
#16854=CARTESIAN_POINT ( 'NONE',  ( 14.38125909742181285, -17.55144818341476309, 39.01709431150910490 ) ) ;
#16855=CARTESIAN_POINT ( 'NONE',  ( -39.58644176656172675, -13.59899295350269810, 32.83087322326096569 ) ) ;
#16856=CARTESIAN_POINT ( 'NONE',  ( 8.602182264176247983, 18.59145335917338926, -44.88373884391542390 ) ) ;
#16858=CARTESIAN_POINT ( 'NONE',  ( 4.995406935893283773, 39.06748935135171052, 17.50105314357239195 ) ) ;
#16860=CARTESIAN_POINT ( 'NONE',  ( -189.0540493709916632, -17.95404051684981894, 43.34488811517340423 ) ) ;
#16861=CARTESIAN_POINT ( 'NONE',  ( 14.38125909742181108, 1.616281842095393922E-13, -15.17850393972633682 ) ) ;
#16862=CARTESIAN_POINT ( 'NONE',  ( -213.1075012329537230, -9.698598906450557777, 9.698598906450415669 ) ) ;
#16863=CARTESIAN_POINT ( 'NONE',  ( 4.995406935893297984, 10.78321810390233892, -67.35176059882522281 ) ) ;
#16864=CARTESIAN_POINT ( 'NONE',  ( 199.9999999999999432, 14.14213562373093680, 14.14213562373114641 ) ) ;
#16866=CARTESIAN_POINT ( 'NONE',  ( -30.26275506840325136, 57.76657404653985139, -1.198031551615314161 ) ) ;
#16867=CARTESIAN_POINT ( 'NONE',  ( -213.1075012329537230, 66.26714140138673770, -9.698598906462034819 ) ) ;
#16868=CARTESIAN_POINT ( 'NONE',  ( -280.0000000000000568, 19.99999999999996092, 40.00000000000002132 ) ) ;
#16869=CARTESIAN_POINT ( 'NONE',  ( -135.8532207217289738, -9.153146818113595984, -40.00000000000002132 ) ) ;
#16870=CARTESIAN_POINT ( 'NONE',  ( 0.2972598230769938343, 10.13633138497472252, 10.13633138497475628 ) ) ;
#16872=CARTESIAN_POINT ( 'NONE',  ( -135.8532207217289738, -21.81201906317757633, -21.81201906317793515 ) ) ;
#16873=CARTESIAN_POINT ( 'NONE',  ( -4.039451493210501454, 43.00522595894040734, -23.44932283416630270 ) ) ;
#16874=ORIENTED_EDGE ( 'NONE', *, *, #1024, .T. ) ;
#16875=CARTESIAN_POINT ( 'NONE',  ( -192.9588430854690273, 10.23066800231970319, 66.79921049724369198 ) ) ;
#16876=CARTESIAN_POINT ( 'NONE',  ( -87.13361725312203987, -16.15936047674203024, -14.23663594861907988 ) ) ;
#16877=CARTESIAN_POINT ( 'NONE',  ( 163.1118516004056573, -9.006482792069636645, 9.006482792069567367 ) ) ;
#16878=CARTESIAN_POINT ( 'NONE',  ( 3.869409319523309687, -48.96737585071549148, -14.12455301876188507 ) ) ;
#16880=CARTESIAN_POINT ( 'NONE',  ( 130.8568914410475372, -34.05028731879786363, 0.000000000000000000 ) ) ;
#16881=CARTESIAN_POINT ( 'NONE',  ( -105.4741150117383341, -8.366608964593364561, -19.60045294982747777 ) ) ;
#16884=CARTESIAN_POINT ( 'NONE',  ( -114.7252611291634139, -21.81972725943360913, 3.452297386453273109 ) ) ;
#16885=CARTESIAN_POINT ( 'NONE',  ( 170.2234770963711128, 15.44714144992819094, 2.449293598294708485E-15 ) ) ;
#16886=CARTESIAN_POINT ( 'NONE',  ( -106.9675868842832358, 19.33814434321038078, 8.010121658085223473 ) ) ;
#16888=CARTESIAN_POINT ( 'NONE',  ( 57.59792236341148453, -54.84617931850879557, 1.722363176414566155 ) ) ;
#16889=CARTESIAN_POINT ( 'NONE',  ( -86.96347745069645896, 39.99999999999994316, 18.24025645688366737 ) ) ;
#16890=CARTESIAN_POINT ( 'NONE',  ( -135.8532207217289738, 40.00000000000002842, -9.153146818113432559 ) ) ;
#16892=CARTESIAN_POINT ( 'NONE',  ( 4.995406935893307754, -55.24977328854835434, -2.449293598294708485E-15 ) ) ;
#16893=CARTESIAN_POINT ( 'NONE',  ( 23.64688638900294038, -13.78084749393264907, -46.70960658758787076 ) ) ;
#16895=CARTESIAN_POINT ( 'NONE',  ( -56.48582580120557850, -30.84685318188645198, -2.449293598294708485E-15 ) ) ;
#16896=CARTESIAN_POINT ( 'NONE',  ( -105.3755690713226727, -12.89780903124413847, 12.89780903124398037 ) ) ;
#16897=CARTESIAN_POINT ( 'NONE',  ( 149.5797498300189261, -12.18602109748318441, -29.41965740490883263 ) ) ;
#16898=CARTESIAN_POINT ( 'NONE',  ( -114.7538884075326564, 13.57382480621628673, -17.50182194317628515 ) ) ;
#16899=CARTESIAN_POINT ( 'NONE',  ( -100.7734535825088500, 40.00000000000017764, -17.32597176626768487 ) ) ;
#16900=CARTESIAN_POINT ( 'NONE',  ( -280.0000000000000000, -14.14213562373098831, -14.14213562373098654 ) ) ;
#16901=CARTESIAN_POINT ( 'NONE',  ( -126.6834156231682300, -24.89646324320138859, -9.107266674873804035 ) ) ;
#16903=CARTESIAN_POINT ( 'NONE',  ( -162.0762913951020892, -57.76657433524000851, 1.198031840315820329 ) ) ;
#16904=ORIENTED_EDGE ( 'NONE', *, *, #17112, .T. ) ;
#16905=CARTESIAN_POINT ( 'NONE',  ( 146.6084372240433993, 24.48358557860307272, 24.48358557860347418 ) ) ;
#16906=CARTESIAN_POINT ( 'NONE',  ( -70.35386311717272179, 23.12931224224253768, -8.707385196623391721 ) ) ;
#16907=CARTESIAN_POINT ( 'NONE',  ( -109.1264249741437027, -13.72187187123250673, 33.12752917269451558 ) ) ;
#16908=CARTESIAN_POINT ( 'NONE',  ( -280.0000000000000000, -20.00000000000006750, -2.449293598294708485E-15 ) ) ;
#16909=CARTESIAN_POINT ( 'NONE',  ( -105.4288990061682654, 9.009177719101042925, 19.35827336168831891 ) ) ;
#16914=CARTESIAN_POINT ( 'NONE',  ( -89.91498783729078070, 8.087768383257817106, -20.43892340018621212 ) ) ;
#16915=ORIENTED_EDGE ( 'NONE', *, *, #20205, .F. ) ;
#16917=( BOUNDED_CURVE ( )  B_SPLINE_CURVE ( 3, ( #18782, #829, #6929, #15046 ),
 .UNSPECIFIED., .F., .F. ) 
 B_SPLINE_CURVE_WITH_KNOTS ( ( 4, 4 ),
 ( 0.007854122480128121128, 0.01576650722534447477 ),
 .UNSPECIFIED. ) 
 CURVE ( )  GEOMETRIC_REPRESENTATION_ITEM ( )  RATIONAL_B_SPLINE_CURVE ( ( 0.5857864376268409057, 0.5560595459730206525, 0.5340584217468142825, 0.5197830649482216847 ) ) 
 REPRESENTATION_ITEM ( '' )  );
#16918=CARTESIAN_POINT ( 'NONE',  ( -100.7734535825088500, -44.31723036834903695, 12.25131212657476709 ) ) ;
#16920=CARTESIAN_POINT ( 'NONE',  ( -110.0723150831436783, -5.015078513972359708, 19.55249150545837367 ) ) ;
#16921=CARTESIAN_POINT ( 'NONE',  ( 19.06497207195980792, -18.24870850772763475, 38.31983398719622613 ) ) ;
#16923=CARTESIAN_POINT ( 'NONE',  ( 57.59792236341146321, 40.00000000000004263, -2.435789363418021214 ) ) ;
#16924=CARTESIAN_POINT ( 'NONE',  ( -198.0012279374157345, -24.77357825033869787, 44.79720170867067708 ) ) ;
#16926=CARTESIAN_POINT ( 'NONE',  ( 57.59792236341147742, 4.064940816252731242E-13, -37.56421063658186199 ) ) ;
#16927=CARTESIAN_POINT ( 'NONE',  ( -192.9588430854690273, 40.00000000000014211, -14.46834944099927966 ) ) ;
#16928=CARTESIAN_POINT ( 'NONE',  ( -87.01139150504059216, 18.62802765663150595, 10.64887401541982825 ) ) ;
#16931=CARTESIAN_POINT ( 'NONE',  ( -190.5535326094083075, 18.10342187830005400, 43.70552662395296295 ) ) ;
#16932=CARTESIAN_POINT ( 'NONE',  ( -259.2033419157646676, 6.730120644403426944, 6.730120644403592145 ) ) ;
#16934=CARTESIAN_POINT ( 'NONE',  ( -238.4067589809705794, 27.60227080167040370, 28.96627169325338613 ) ) ;
#16935=CARTESIAN_POINT ( 'NONE',  ( -86.99952317292415671, -18.62540174576058405, 10.54562204240063927 ) ) ;
#16936=CARTESIAN_POINT ( 'NONE',  ( -91.56559293963834989, -12.25131212657475466, -12.25131212657495361 ) ) ;
#16938=CARTESIAN_POINT ( 'NONE',  ( 19.06497207195980792, -14.19242893257839988, 40.00000000000002132 ) ) ;
#16939=CARTESIAN_POINT ( 'NONE',  ( -213.1075012329537230, 66.26714140138673770, -9.698598906462034819 ) ) ;
#16940=CARTESIAN_POINT ( 'NONE',  ( 146.6084372240433709, -5.374981219216948602, 40.00000000000002132 ) ) ;
#16943=CARTESIAN_POINT ( 'NONE',  ( 91.82158438592159655, -39.99999999999976552, -22.79471317813512599 ) ) ;
#16948=VERTEX_POINT ( 'NONE', #709 ) ;
#16949=CARTESIAN_POINT ( 'NONE',  ( -135.8532207217289738, 30.84685318188643421, 40.00000000000002132 ) ) ;
#16950=CARTESIAN_POINT ( 'NONE',  ( -105.4741150117383199, -19.77569912955117459, -7.943527260750404828 ) ) ;
#16952=CARTESIAN_POINT ( 'NONE',  ( -114.5514240057833462, -20.88736325016649076, 6.817200166920974524 ) ) ;
#16953=EDGE_CURVE ( 'NONE', #3360, #12515, #9288, .T. ) ;
#16954=CARTESIAN_POINT ( 'NONE',  ( -188.2995950289364941, -13.82811170417257607, 46.99046209955427855 ) ) ;
#16955=CARTESIAN_POINT ( 'NONE',  ( 136.1360204305621266, 1.473277640373554421E-13, -35.03383547441296741 ) ) ;
#16959=CARTESIAN_POINT ( 'NONE',  ( 19.06497207195981858, 10.03556273973516078, -66.60410523465806421 ) ) ;
#16960=CARTESIAN_POINT ( 'NONE',  ( 151.7948205124836250, 23.49921654116328540, 23.49921654116366554 ) ) ;
#16961=CARTESIAN_POINT ( 'NONE',  ( -105.2054292634446284, -16.15935121071317226, -14.23664521671883065 ) ) ;
#16962=CARTESIAN_POINT ( 'NONE',  ( -30.26275506840323359, 4.336144384597734078E-13, -41.69427246844629309 ) ) ;
#16963=DIRECTION ( 'NONE',  ( 0.9698969544100559670, -0.2249791742613554413, 0.09318942523042274273 ) ) ;
#16964=CARTESIAN_POINT ( 'NONE',  ( -2.654373026594472496, 13.89837698318165415, 47.46285323120913802 ) ) ;
#16965=EDGE_CURVE ( 'NONE', #13683, #11812, #10235, .T. ) ;
#16966=ADVANCED_FACE ( 'NONE', ( #13564 ), #25315, .F. ) ;
#16967=CARTESIAN_POINT ( 'NONE',  ( -238.4067589809705794, -0.6820004458488042598, 57.25054294077229855 ) ) ;
#16970=CARTESIAN_POINT ( 'NONE',  ( -280.0000000000000000, 1.839446121267387017E-14, -20.00000000000001421 ) ) ;
#16972=CARTESIAN_POINT ( 'NONE',  ( 4.995406935893297096, 10.78321810387837232, 67.35176059880234334 ) ) ;
#16973=CARTESIAN_POINT ( 'NONE',  ( -238.4067589809705794, 40.96449427990177128, 40.00000000000002132 ) ) ;
#16976=CARTESIAN_POINT ( 'NONE',  ( 1.925538622597735117, -44.35335385591510260, 24.44644315489020414 ) ) ;
#16977=CARTESIAN_POINT ( 'NONE',  ( -162.0762913951021176, 1.694272876828294194, -40.00000000000002132 ) ) ;
#16978=ORIENTED_EDGE ( 'NONE', *, *, #21180, .F. ) ;
#16980=CARTESIAN_POINT ( 'NONE',  ( -4.061681315507545520, -13.82654462146593133, 46.98276670624663609 ) ) ;
#16981=CARTESIAN_POINT ( 'NONE',  ( -87.07906654914069122, 21.13868447709362641, 3.689035289844212251 ) ) ;
#16982=CARTESIAN_POINT ( 'NONE',  ( -2.654373026594466278, -13.89837698318132198, -47.46285323120923749 ) ) ;
#16984=CARTESIAN_POINT ( 'NONE',  ( 170.2234770963711128, 10.92277846919147066, 45.64576402573197811 ) ) ;
#16985=CARTESIAN_POINT ( 'NONE',  ( -87.07756624671603163, -21.12895881757819438, 3.737545040698849963 ) ) ;
#16987=CARTESIAN_POINT ( 'NONE',  ( -193.3669098795969319, -18.32287322059158896, 44.23532903077781953 ) ) ;
#16988=CARTESIAN_POINT ( 'NONE',  ( -238.4067589809705794, 27.60227080167080160, -28.96627169325299533 ) ) ;
#16990=CARTESIAN_POINT ( 'NONE',  ( 130.8568914410475088, 52.36146031193420924, 4.207082182989907437 ) ) ;
#16991=CARTESIAN_POINT ( 'NONE',  ( -56.48582580120559982, -34.75652343174584047, -21.81201906317815187 ) ) ;
#16992=CARTESIAN_POINT ( 'NONE',  ( -213.1075012329537230, -9.698598906450422774, -9.698598906450550672 ) ) ;
#16993=CARTESIAN_POINT ( 'NONE',  ( -162.0762913951021176, 27.08623940707639477, -29.48230308784743059 ) ) ;
#16994=CARTESIAN_POINT ( 'NONE',  ( 200.0000000000000000, 42.42640687119267540, 14.14213562373153543 ) ) ;
#16995=CARTESIAN_POINT ( 'NONE',  ( 151.7948205124836250, 4.785054706301759886, -4.785054706301612448 ) ) ;
#16996=CARTESIAN_POINT ( 'NONE',  ( -259.2033419157646676, 9.517827891722582478, 40.00000000000002132 ) ) ;
#16997=CARTESIAN_POINT ( 'NONE',  ( -198.0356074513804572, 15.37879056873067007, 0.000000000000000000 ) ) ;
#16998=CARTESIAN_POINT ( 'NONE',  ( 151.7948205124836534, 4.785054706298574878, -51.78348778862537927 ) ) ;
#17000=CARTESIAN_POINT ( 'NONE',  ( -213.1075012329537230, -37.98287015391257881, 18.58567234101111509 ) ) ;
#17002=ORIENTED_EDGE ( 'NONE', *, *, #14820, .F. ) ;
#17003=CARTESIAN_POINT ( 'NONE',  ( -100.7734535825088500, -16.03295912088716335, 40.53558337403673306 ) ) ;
#17004=CARTESIAN_POINT ( 'NONE',  ( -77.70094361819319317, -18.98776814046944494, -11.20662771258744428 ) ) ;
#17005=CARTESIAN_POINT ( 'NONE',  ( 0.2972598230770100991, -38.42060263243686791, 38.42060263243645579 ) ) ;
#17006=CARTESIAN_POINT ( 'NONE',  ( -87.13361725327072804, -21.49321519333431141, 0.6860286135013640152 ) ) ;
#17007=EDGE_LOOP ( 'NONE', ( #18063, #4823, #24521, #16 ) ) ;
#17008=CARTESIAN_POINT ( 'NONE',  ( -105.3174410934715439, -10.86122935356454100, -18.50851042455845885 ) ) ;
#17009=VECTOR ( 'NONE', #5877, 1000.000000000000000 ) ;
#17011=CARTESIAN_POINT ( 'NONE',  ( -114.4944481313176396, -20.59122811151893373, -7.435744517473755089 ) ) ;
#17012=CARTESIAN_POINT ( 'NONE',  ( 4.995406935893288214, 55.24977328854835434, 2.449293598294708485E-15 ) ) ;
#17015=( BOUNDED_SURFACE ( )  B_SPLINE_SURFACE ( 3, 3, ( 
 ( #5922, #13754, #21882, #10177, #14030, #24146, #2203, #16290, #5785, #18281, #7902, #16021, #26160, #13892, #22160, #25888, #3939, #26027, #20154, #1936, #16156, #6057, #20424, #22293, #4205, #22026, #9777, #12172, #20291, #10312 ),
 ( #67, #8175, #7630, #11901, #15765, #17767, #11387, #5669, #20046, #11922, #26185, #23893, #3679, #21641, #9525, #21772, #13775, #1294, #1824, #21904, #11787, #17633, #9402, #23635, #11516, #19907, #7923, #9927, #18033, #15634 ),
 ( #3545, #9663, #7526, #9795, #23511, #19509, #5285, #25909, #11645, #17508, #1691, #17899, #5540, #7650, #26046, #7783, #22047, #25775, #3820, #13392, #19769, #21517, #25648, #15899, #1558, #24028, #3291, #13912, #5414, #5805 ),
 ( #7394, #15507, #13516, #3414, #19641, #23759, #1424, #13647, #16311, #8324, #14577, #24166, #12584, #5941, #20576, #20174, #22183, #16448, #4091, #2348, #14314, #22577, #2479, #12448, #12317, #3956, #24572, #14049, #86, #10461 ),
 ( #4482, #12054, #1957, #10063, #8195, #24311, #6328, #18169, #2222, #20713, #18299, #489, #20312, #26316, #14450, #2089, #8059, #24707, #18573, #6077, #16175, #4356, #6462, #353, #24435, #8457, #16576, #14179, #10196, #22314 ),
 ( #6203, #22448, #12190, #16040, #4228, #20444, #10330, #18439, #214, #22706, #10591, #18706, #21368, #887, #7120, #14838, #24838, #15100, #23108, #13243, #620, #19232, #25366, #8996, #23361, #6726, #17100, #2886, #22843, #25233 ),
 ( #16844, #6856, #5138, #6589, #14711, #12714, #755, #24977, #6985, #20842, #21107, #3136, #10857, #19356, #12855, #16706, #23235, #20973, #2617, #17226, #3011, #22971, #10731, #5011, #15230, #1012, #8859, #13116, #21237, #4618 ) ),
 .UNSPECIFIED., .T., .F., .F. ) 
 B_SPLINE_SURFACE_WITH_KNOTS ( ( 4, 3, 4 ),
 ( 4, 2, 2, 2, 2, 2, 2, 2, 2, 2, 2, 2, 2, 2, 4 ),
 ( 0.000000000000000000, 0.5000000000000000000, 1.000000000000000000 ),
 ( 0.000000000000000000, 0.1357259735107005372, 0.1651108541090157700, 0.1944957347073310028, 0.3598804999793158710, 0.3867117631979620773, 0.4135430264166082281, 0.5789277916885930964, 0.6062785021374117456, 0.6336292125862302838, 0.8508620842112317728, 0.8814014469398914198, 0.9119408096685510667, 0.9559704048342755334, 1.000000000000000000 ),
 .UNSPECIFIED. ) 
 GEOMETRIC_REPRESENTATION_ITEM ( )  RATIONAL_B_SPLINE_SURFACE ( (
 ( 1.000000000000000000, 1.000000000000000000, 1.000000000000000000, 1.000000000000000000, 1.000000000000000000, 1.000000000000000000, 1.000000000000000000, 1.000000000000000000, 1.000000000000000000, 1.000000000000000000, 1.000000000000000000, 1.000000000000000000, 1.000000000000000000, 1.000000000000000000, 1.000000000000000000, 1.000000000000000000, 1.000000000000000000, 1.000000000000000000, 1.000000000000000000, 1.000000000000000000, 1.000000000000000000, 1.000000000000000000, 1.000000000000000000, 1.000000000000000000, 1.000000000000000000, 1.000000000000000000, 1.000000000000000000, 1.000000000000000000, 1.000000000000000000, 1.000000000000000000),
 ( 0.3333333333333333703, 0.3333333333333333703, 0.3333333333333333703, 0.3333333333333333703, 0.3333333333333333703, 0.3333333333333333703, 0.3333333333333333703, 0.3333333333333333703, 0.3333333333333333703, 0.3333333333333333703, 0.3333333333333333703, 0.3333333333333333703, 0.3333333333333333703, 0.3333333333333333703, 0.3333333333333333703, 0.3333333333333333703, 0.3333333333333333703, 0.3333333333333333703, 0.3333333333333333703, 0.3333333333333333703, 0.3333333333333333703, 0.3333333333333333703, 0.3333333333333333703, 0.3333333333333333703, 0.3333333333333333703, 0.3333333333333333703, 0.3333333333333333703, 0.3333333333333333703, 0.3333333333333333703, 0.3333333333333333703),
 ( 0.3333333333333333703, 0.3333333333333333703, 0.3333333333333333703, 0.3333333333333333703, 0.3333333333333333703, 0.3333333333333333703, 0.3333333333333333703, 0.3333333333333333703, 0.3333333333333333703, 0.3333333333333333703, 0.3333333333333333703, 0.3333333333333333703, 0.3333333333333333703, 0.3333333333333333703, 0.3333333333333333703, 0.3333333333333333703, 0.3333333333333333703, 0.3333333333333333703, 0.3333333333333333703, 0.3333333333333333703, 0.3333333333333333703, 0.3333333333333333703, 0.3333333333333333703, 0.3333333333333333703, 0.3333333333333333703, 0.3333333333333333703, 0.3333333333333333703, 0.3333333333333333703, 0.3333333333333333703, 0.3333333333333333703),
 ( 1.000000000000000000, 1.000000000000000000, 1.000000000000000000, 1.000000000000000000, 1.000000000000000000, 1.000000000000000000, 1.000000000000000000, 1.000000000000000000, 1.000000000000000000, 1.000000000000000000, 1.000000000000000000, 1.000000000000000000, 1.000000000000000000, 1.000000000000000000, 1.000000000000000000, 1.000000000000000000, 1.000000000000000000, 1.000000000000000000, 1.000000000000000000, 1.000000000000000000, 1.000000000000000000, 1.000000000000000000, 1.000000000000000000, 1.000000000000000000, 1.000000000000000000, 1.000000000000000000, 1.000000000000000000, 1.000000000000000000, 1.000000000000000000, 1.000000000000000000),
 ( 0.3333333333333333703, 0.3333333333333333703, 0.3333333333333333703, 0.3333333333333333703, 0.3333333333333333703, 0.3333333333333333703, 0.3333333333333333703, 0.3333333333333333703, 0.3333333333333333703, 0.3333333333333333703, 0.3333333333333333703, 0.3333333333333333703, 0.3333333333333333703, 0.3333333333333333703, 0.3333333333333333703, 0.3333333333333333703, 0.3333333333333333703, 0.3333333333333333703, 0.3333333333333333703, 0.3333333333333333703, 0.3333333333333333703, 0.3333333333333333703, 0.3333333333333333703, 0.3333333333333333703, 0.3333333333333333703, 0.3333333333333333703, 0.3333333333333333703, 0.3333333333333333703, 0.3333333333333333703, 0.3333333333333333703),
 ( 0.3333333333333333703, 0.3333333333333333703, 0.3333333333333333703, 0.3333333333333333703, 0.3333333333333333703, 0.3333333333333333703, 0.3333333333333333703, 0.3333333333333333703, 0.3333333333333333703, 0.3333333333333333703, 0.3333333333333333703, 0.3333333333333333703, 0.3333333333333333703, 0.3333333333333333703, 0.3333333333333333703, 0.3333333333333333703, 0.3333333333333333703, 0.3333333333333333703, 0.3333333333333333703, 0.3333333333333333703, 0.3333333333333333703, 0.3333333333333333703, 0.3333333333333333703, 0.3333333333333333703, 0.3333333333333333703, 0.3333333333333333703, 0.3333333333333333703, 0.3333333333333333703, 0.3333333333333333703, 0.3333333333333333703),
 ( 1.000000000000000000, 1.000000000000000000, 1.000000000000000000, 1.000000000000000000, 1.000000000000000000, 1.000000000000000000, 1.000000000000000000, 1.000000000000000000, 1.000000000000000000, 1.000000000000000000, 1.000000000000000000, 1.000000000000000000, 1.000000000000000000, 1.000000000000000000, 1.000000000000000000, 1.000000000000000000, 1.000000000000000000, 1.000000000000000000, 1.000000000000000000, 1.000000000000000000, 1.000000000000000000, 1.000000000000000000, 1.000000000000000000, 1.000000000000000000, 1.000000000000000000, 1.000000000000000000, 1.000000000000000000, 1.000000000000000000, 1.000000000000000000, 1.000000000000000000) ) ) 
 REPRESENTATION_ITEM ( '' )  SURFACE ( )  );
#17016=CARTESIAN_POINT ( 'NONE',  ( 200.0000000000000000, -14.14213562373122457, 42.42640687119282461 ) ) ;
#17017=CARTESIAN_POINT ( 'NONE',  ( 163.1118516004056573, -1.695744499706194789E-14, 12.73709011382475254 ) ) ;
#17018=CARTESIAN_POINT ( 'NONE',  ( 192.4448373802101173, 39.99999999999998579, 19.99999999996075317 ) ) ;
#17019=CARTESIAN_POINT ( 'NONE',  ( -87.13361725327074225, 15.19799821270847850, -15.19799821270833284 ) ) ;
#17020=CARTESIAN_POINT ( 'NONE',  ( -198.0356074513804572, -55.37879056871328487, -40.00000000000002132 ) ) ;
#17021=CARTESIAN_POINT ( 'NONE',  ( 22.78333232259009122, -17.88247728649339052, -43.17211919388243047 ) ) ;
#17023=CARTESIAN_POINT ( 'NONE',  ( 151.7948205124836534, -6.767089262349000656, -40.00000000000002132 ) ) ;
#17024=CARTESIAN_POINT ( 'NONE',  ( 4.995406935893293543, -10.78321810389005364, 10.78321810388994173 ) ) ;
#17025=CARTESIAN_POINT ( 'NONE',  ( -100.7734535825088500, 40.00000000000017764, -17.32597176626768487 ) ) ;
#17027=CARTESIAN_POINT ( 'NONE',  ( 146.6084372240433709, -39.99999999999993605, -5.374981219217395356 ) ) ;
#17029=EDGE_CURVE ( 'NONE', #14634, #525, #1329, .T. ) ;
#17030=CARTESIAN_POINT ( 'NONE',  ( 159.7742640750898317, -25.95918014511565985, -10.75264448419334684 ) ) ;
#17032=CARTESIAN_POINT ( 'NONE',  ( 91.82158438592159655, -16.11829626346147393, 16.11829626346132116 ) ) ;
#17034=CARTESIAN_POINT ( 'NONE',  ( -77.90255099906769942, -8.064892378657791738, -20.29001641120690635 ) ) ;
#17035=CARTESIAN_POINT ( 'NONE',  ( -5.787027468457909052, 42.67020100828210616, -17.67457596682473664 ) ) ;
#17036=DIRECTION ( 'NONE',  ( 0.9698969544411999433, -0.2249791741464770845, -0.09318942518362427485 ) ) ;
#17037=CARTESIAN_POINT ( 'NONE',  ( 146.6084372240433993, -5.374981219216945938, -2.449293598294708485E-15 ) ) ;
#17038=CARTESIAN_POINT ( 'NONE',  ( -87.13361725327072804, -21.49321519333431141, -3.542586001259484843E-15 ) ) ;
#17039=CARTESIAN_POINT ( 'NONE',  ( -189.6939181379374588, 43.50327460064623608, -18.01964634722715530 ) ) ;
#17044=CARTESIAN_POINT ( 'NONE',  ( -102.4309680866260521, 8.087567261726858803, -20.43798635336598934 ) ) ;
#17046=ORIENTED_EDGE ( 'NONE', *, *, #15610, .T. ) ;
#17047=CARTESIAN_POINT ( 'NONE',  ( -280.0000000000000568, -14.14213562373108601, 42.42640687119285303 ) ) ;
#17050=CARTESIAN_POINT ( 'NONE',  ( -105.2958943010082749, -4.721182065458395805, 20.90688085069918500 ) ) ;
#17051=CARTESIAN_POINT ( 'NONE',  ( -259.2033419157646676, -6.730120644403667640, 49.83842185052029805 ) ) ;
#17053=CARTESIAN_POINT ( 'NONE',  ( 98.29820294270297154, 18.47759065022021474, -7.653668647299666894 ) ) ;
#17054=CARTESIAN_POINT ( 'NONE',  ( 14.38125909742180930, 39.99999999999982947, 55.17850393971022527 ) ) ;
#17059=CARTESIAN_POINT ( 'NONE',  ( 184.8905102610680444, -40.00000000000021316, 20.92133201514402430 ) ) ;
#17060=CARTESIAN_POINT ( 'NONE',  ( -105.3755690713226585, -39.99999999999985079, -18.24025645688394448 ) ) ;
#17061=FACE_OUTER_BOUND ( 'NONE', #1768, .T. ) ;
#17064=CARTESIAN_POINT ( 'NONE',  ( -194.4222775680326265, 14.07715774765984840, 48.65439176088747786 ) ) ;
#17065=CARTESIAN_POINT ( 'NONE',  ( 151.7948205124835681, -4.785054706298876859, 51.78348778862533663 ) ) ;
#17066=DIRECTION ( 'NONE',  ( 0.000000000000000000, 1.000000000000000000, 0.000000000000000000 ) ) ;
#17067=CARTESIAN_POINT ( 'NONE',  ( -162.0762913951021176, 27.08623940707598265, 29.48230308784781428 ) ) ;
#17068=CARTESIAN_POINT ( 'NONE',  ( -77.61421004776265420, -12.97751843348499889, 17.87698779689324979 ) ) ;
#17069=CARTESIAN_POINT ( 'NONE',  ( 136.1360204305621266, 53.05693388239320285, -3.511608612530223716 ) ) ;
#17072=VERTEX_POINT ( 'NONE', #17311 ) ;
#17073=CARTESIAN_POINT ( 'NONE',  ( -259.2033419157646676, 49.83842185052017015, 6.730120644404137487 ) ) ;
#17074=CARTESIAN_POINT ( 'NONE',  ( -86.96347745069645896, 21.75974354311648895, -0.000000000000000000 ) ) ;
#17077=CARTESIAN_POINT ( 'NONE',  ( -135.8532207217289738, -39.99999999999972289, -30.84685318188688541 ) ) ;
#17079=CARTESIAN_POINT ( 'NONE',  ( 126.3230993689413140, -11.72464299830521384, 28.30579214049032899 ) ) ;
#17082=ORIENTED_EDGE ( 'NONE', *, *, #1201, .F. ) ;
#17083=CARTESIAN_POINT ( 'NONE',  ( 146.6084372240433709, 5.374981219216996564, 40.00000000000002132 ) ) ;
#17085=CIRCLE ( 'NONE', #18799, 69.99999999999994316 ) ;
#17087=CARTESIAN_POINT ( 'NONE',  ( 163.1118516004056573, 1.251511021549353291E-13, -27.26290988616872824 ) ) ;
#17090=CARTESIAN_POINT ( 'NONE',  ( -30.26275506840324070, 1.198031551616724366, -57.76657404653984429 ) ) ;
#17091=CARTESIAN_POINT ( 'NONE',  ( 199.9999999999999432, 14.14213562373093680, 14.14213562373114641 ) ) ;
#17092=CARTESIAN_POINT ( 'NONE',  ( -105.2054292635175585, -15.19799821370228798, -15.19799821370232173 ) ) ;
#17093=CARTESIAN_POINT ( 'NONE',  ( -86.96347745069644475, 1.775309070576523494E-13, -18.24025645688352881 ) ) ;
#17094=CARTESIAN_POINT ( 'NONE',  ( -198.0356074513804572, -10.87444709759714634, -10.87444709759729911 ) ) ;
#17095=FACE_OUTER_BOUND ( 'NONE', #3015, .T. ) ;
#17096=CARTESIAN_POINT ( 'NONE',  ( 146.6084372240433993, -3.800685668858652999, 3.800685668858636568 ) ) ;
#17099=CARTESIAN_POINT ( 'NONE',  ( 14.38125909742181108, -5.035366881890652543E-14, 15.17850393972633682 ) ) ;
#17100=CARTESIAN_POINT ( 'NONE',  ( 170.2234770963711128, -24.55285855007184281, -40.00000000000002132 ) ) ;
#17101=CARTESIAN_POINT ( 'NONE',  ( -30.26275506840324070, 1.198031551615912571, 57.76657404653985139 ) ) ;
#17102=CARTESIAN_POINT ( 'NONE',  ( 57.59792236341147031, 37.56421063658187620, 40.00000000000002132 ) ) ;
#17105=CARTESIAN_POINT ( 'NONE',  ( 8.273828130744583120, -44.87796109790054544, 18.58906013840162785 ) ) ;
#17106=CARTESIAN_POINT ( 'NONE',  ( 14.38125909742180752, 15.17850393972634038, -40.00000000000002132 ) ) ;
#17109=CARTESIAN_POINT ( 'NONE',  ( -91.56559293963834989, -16.03295912088716335, 40.53558337403673306 ) ) ;
#17110=CARTESIAN_POINT ( 'NONE',  ( 136.1360204305621551, -39.99999999999987921, -35.03383547441310242 ) ) ;
#17111=CARTESIAN_POINT ( 'NONE',  ( -87.09798021405659085, 21.26125105737227372, 2.995673697387337686 ) ) ;
#17112=EDGE_CURVE ( 'NONE', #19812, #21839, #5472, .T. ) ;
#17113=EDGE_CURVE ( 'NONE', #16811, #12394, #8978, .T. ) ;
#17114=CARTESIAN_POINT ( 'NONE',  ( -77.90255099906865155, 8.064892378658621297, -20.29001641120614252 ) ) ;
#17116=CARTESIAN_POINT ( 'NONE',  ( -208.1127848780264742, 67.17687982763172272, -10.60833733270698254 ) ) ;
#17118=B_SPLINE_CURVE_WITH_KNOTS ( 'NONE', 3,
 ( #13867, #24259, #12013, #24124, #14405, #22133 ),
 .UNSPECIFIED., .F., .F.,
 ( 4, 2, 4 ),
 ( 0.000000000000000000, 0.03937794852163883919, 0.07875589704327767837 ),
 .UNSPECIFIED. ) ;
#17120=CARTESIAN_POINT ( 'NONE',  ( -105.3755690713226585, 43.67073346367988051, -12.89780903124366418 ) ) ;
#17121=CARTESIAN_POINT ( 'NONE',  ( 136.1360204305621266, 53.05693388239316022, 3.511608612530967566 ) ) ;
#17122=CARTESIAN_POINT ( 'NONE',  ( -77.90255099906853786, 8.644468104252327478, -20.04994828524281303 ) ) ;
#17123=CARTESIAN_POINT ( 'NONE',  ( 4.995406935893293543, -10.78321810388990265, -10.78321810389009272 ) ) ;
#17124=CARTESIAN_POINT ( 'NONE',  ( -198.9233928134160578, 24.80620717269982833, -44.84148042516462596 ) ) ;
#17125=CARTESIAN_POINT ( 'NONE',  ( 192.4448373802101173, 14.14213562370261279, 42.42640687122091236 ) ) ;
#17126=CARTESIAN_POINT ( 'NONE',  ( -86.96347745069644475, 12.89780903124419353, -12.89780903124389333 ) ) ;
#17127=CARTESIAN_POINT ( 'NONE',  ( -86.96347745069644475, 18.24025645688350750, -40.00000000000002132 ) ) ;
#17128=CARTESIAN_POINT ( 'NONE',  ( 163.1118516004056573, 37.29075403953160617, -19.27778845539222985 ) ) ;
#17129=FACE_OUTER_BOUND ( 'NONE', #14810, .T. ) ;
#17130=CARTESIAN_POINT ( 'NONE',  ( -238.4067589809705794, -57.25054294077233408, -0.6820004458489551391 ) ) ;
#17131=CARTESIAN_POINT ( 'NONE',  ( -151.4802849342813715, 31.86309571753157854, -16.17241510390819670 ) ) ;
#17132=ORIENTED_EDGE ( 'NONE', *, *, #9776, .T. ) ;
#17133=CARTESIAN_POINT ( 'NONE',  ( -105.3755690713226727, 12.89780903124400879, 12.89780903124407452 ) ) ;
#17134=CARTESIAN_POINT ( 'NONE',  ( -77.55640685876512919, -15.64922766773197971, -15.64922766773223906 ) ) ;
#17135=CARTESIAN_POINT ( 'NONE',  ( -105.3755690713226585, 43.67073346367970288, 12.89780903124427702 ) ) ;
#17136=CARTESIAN_POINT ( 'NONE',  ( -4.421177063219155379, -42.89273859401222211, -23.37490463203747382 ) ) ;
#17137=VERTEX_POINT ( 'NONE', #13662 ) ;
#17138=CARTESIAN_POINT ( 'NONE',  ( -188.2506440019887464, -42.99080317017353536, 23.43978047293204980 ) ) ;
#17140=CARTESIAN_POINT ( 'NONE',  ( 22.76838195347369620, -17.88421977190821011, 43.17632592580125817 ) ) ;
#17142=CARTESIAN_POINT ( 'NONE',  ( 146.6084372240433709, -34.62501878078303008, -40.00000000000002132 ) ) ;
#17145=CARTESIAN_POINT ( 'NONE',  ( -91.56559293963834989, -40.53558337403692491, 16.03295912088671571 ) ) ;
#17146=CARTESIAN_POINT ( 'NONE',  ( 146.6084372240433709, -40.00000000000001421, 5.374981219216829587 ) ) ;
#17147=CARTESIAN_POINT ( 'NONE',  ( -192.9588430854689989, -8.596193650988133061E-14, 14.46834944099969533 ) ) ;
#17149=CARTESIAN_POINT ( 'NONE',  ( 163.1118516004056573, 27.26290988616876021, -40.00000000000002132 ) ) ;
#17150=CARTESIAN_POINT ( 'NONE',  ( 22.80622392652972508, -17.87980911537404438, -43.16567765897917752 ) ) ;
#17151=CARTESIAN_POINT ( 'NONE',  ( -192.9588430854689989, -10.23066800230756890, 10.23066800230742501 ) ) ;
#17152=CARTESIAN_POINT ( 'NONE',  ( 146.6084372240433709, -5.374981219216948602, 40.00000000000002132 ) ) ;
#17153=CARTESIAN_POINT ( 'NONE',  ( 57.59792236341147031, 30.00663442387683588, 26.56190807104703211 ) ) ;
#17154=CARTESIAN_POINT ( 'NONE',  ( -198.0356074513804572, 40.00000000000056843, -55.37879056871282302 ) ) ;
#17155=CARTESIAN_POINT ( 'NONE',  ( -105.3178975792744865, 18.51275824395281333, -10.85284064411650817 ) ) ;
#17156=CARTESIAN_POINT ( 'NONE',  ( 163.1118516004056573, -39.99999999999986500, -12.73709011382517353 ) ) ;
#17158=CARTESIAN_POINT ( 'NONE',  ( 135.5348526930097250, -30.20724113681565726, -12.51224896074355009 ) ) ;
#17160=CARTESIAN_POINT ( 'NONE',  ( 130.8568914410475088, 52.36146031193420924, 4.207082182989907437 ) ) ;
#17162=CARTESIAN_POINT ( 'NONE',  ( -105.3755690713226727, 15.38646221621771737, 15.38646221621800514 ) ) ;
#17163=CARTESIAN_POINT ( 'NONE',  ( -3.524834090817577259, 43.28235980537106542, -17.92814044289665887 ) ) ;
#17164=CARTESIAN_POINT ( 'NONE',  ( 167.0466155511619775, 23.44215416552595954, -9.710058186601713714 ) ) ;
#17165=CARTESIAN_POINT ( 'NONE',  ( 19.06497207195980792, -14.19242893257839988, 40.00000000000002132 ) ) ;
#17167=CARTESIAN_POINT ( 'NONE',  ( -189.2667466962275569, 43.39859272266281920, -17.97628569363235229 ) ) ;
#17169=ORIENTED_EDGE ( 'NONE', *, *, #225, .F. ) ;
#17171=CARTESIAN_POINT ( 'NONE',  ( -208.1127848780265026, -10.60833733269551971, 10.60833733269537049 ) ) ;
#17172=CARTESIAN_POINT ( 'NONE',  ( 48.46158931187878238, -35.02055581498660075, -18.19743074333930721 ) ) ;
#17173=ORIENTED_EDGE ( 'NONE', *, *, #15877, .F. ) ;
#17176=CARTESIAN_POINT ( 'NONE',  ( -110.0685463886633926, -5.325649136221389135, 19.46857821975921965 ) ) ;
#17177=CARTESIAN_POINT ( 'NONE',  ( 0.2972598230770011618, 10.13633138497462305, 66.70487387989858519 ) ) ;
#17178=CARTESIAN_POINT ( 'NONE',  ( 57.59792236341147031, -1.722363176415032004, -1.722363176415048880 ) ) ;
#17179=CARTESIAN_POINT ( 'NONE',  ( 19.06497207195979726, 39.99999999999997158, 14.19242893257854554 ) ) ;
#17180=CARTESIAN_POINT ( 'NONE',  ( -200.0000000000000000, -47.66874763508945279, 16.05666331275199354 ) ) ;
#17181=CARTESIAN_POINT ( 'NONE',  ( -4.039451493210481026, -46.99046209229796034, -13.82811171175467102 ) ) ;
#17182=CARTESIAN_POINT ( 'NONE',  ( -198.0356074513804572, -39.99999999999990052, -15.37879056873112482 ) ) ;
#17183=CARTESIAN_POINT ( 'NONE',  ( -192.9588430854690273, 40.00000000000055422, -54.46834944101679810 ) ) ;
#17184=CARTESIAN_POINT ( 'NONE',  ( -77.55640685876515761, 15.64922766773203833, 15.64922766773210761 ) ) ;
#17185=CARTESIAN_POINT ( 'NONE',  ( -83.21262154144251610, -33.12752917118416462, -13.72187187061500779 ) ) ;
#17186=CARTESIAN_POINT ( 'NONE',  ( -200.0000000000000568, 22.35311919176605500, -45.06067021511782400 ) ) ;
#17187=CARTESIAN_POINT ( 'NONE',  ( -138.9613198122422375, 27.95779845120243934, -13.65853124629182247 ) ) ;
#17189=CARTESIAN_POINT ( 'NONE',  ( -193.0908541284702551, -48.38978395451684378, 14.03723495791117948 ) ) ;
#17190=DIRECTION ( 'NONE',  ( -1.836970198721030181E-16, 1.000000000000000000, 0.000000000000000000 ) ) ;
#17191=CARTESIAN_POINT ( 'NONE',  ( -77.56349232223320200, -14.64315958560953490, 16.60062240782924547 ) ) ;
#17192=CARTESIAN_POINT ( 'NONE',  ( -86.96347745069643054, -41.18208027870611687, 15.38646221621750954 ) ) ;
#17194=CARTESIAN_POINT ( 'NONE',  ( 170.0000000000428315, 17.64300463311351308, -17.64300463311329992 ) ) ;
#17195=EDGE_CURVE ( 'NONE', #7311, #858, #395, .T. ) ;
#17197=CARTESIAN_POINT ( 'NONE',  ( 19.06497207195979726, 38.31983398719604139, 18.24870850772803976 ) ) ;
#17199=FACE_OUTER_BOUND ( 'NONE', #20217, .T. ) ;
#17200=ORIENTED_EDGE ( 'NONE', *, *, #8930, .T. ) ;
#17201=CARTESIAN_POINT ( 'NONE',  ( -259.2033419157646676, -39.99999999999975131, -30.48217210827782608 ) ) ;
#17203=ADVANCED_FACE ( 'NONE', ( #19404 ), #18963, .F. ) ;
#17204=CARTESIAN_POINT ( 'NONE',  ( -199.9999999999999432, 10.02640517461776426, -53.44529986889236284 ) ) ;
#17207=CARTESIAN_POINT ( 'NONE',  ( -30.26275506840324070, 41.69427246844628598, 2.449293598294708485E-15 ) ) ;
#17210=CARTESIAN_POINT ( 'NONE',  ( -77.56334768864783769, -14.65129183225244169, 16.59360462362402089 ) ) ;
#17211=CARTESIAN_POINT ( 'NONE',  ( 19.06497207195981858, -40.00000000000007105, 14.19242893257826665 ) ) ;
#17213=AXIS2_PLACEMENT_3D ( 'NONE', #4900, #2774, #5032 ) ;
#17214=CARTESIAN_POINT ( 'NONE',  ( -86.86493150571118349, 8.366608963953861888, 19.60045294882763400 ) ) ;
#17215=CARTESIAN_POINT ( 'NONE',  ( -47.50817905883608461, -12.56548180746172427, -30.33575659736102281 ) ) ;
#17216=CARTESIAN_POINT ( 'NONE',  ( 192.4448373802100889, 14.14213562375873678, 14.14213562375894817 ) ) ;
#17218=CARTESIAN_POINT ( 'NONE',  ( 146.6084372240433709, -39.99999999999993605, -5.374981219217395356 ) ) ;
#17219=CARTESIAN_POINT ( 'NONE',  ( -105.4741150117366431, -7.943527260727707429, 19.77569912956141707 ) ) ;
#17220=B_SPLINE_CURVE_WITH_KNOTS ( 'NONE', 3,
 ( #13056, #10933, #6924, #25043, #688, #23046, #2417, #10666, #10393, #15041, #14513, #4821, #22645, #285 ),
 .UNSPECIFIED., .F., .F.,
 ( 4, 2, 2, 2, 2, 2, 4 ),
 ( 0.0003146819161548550822, 0.002410867973033469468, 0.004507054029912084016, 0.008699426143669313979, 0.01079561220054792853, 0.01289179825742654481, 0.01708417037118376697 ),
 .UNSPECIFIED. ) ;
#17221=CARTESIAN_POINT ( 'NONE',  ( 184.8905102610680444, 20.92133201514447549, 0.000000000000000000 ) ) ;
#17222=CARTESIAN_POINT ( 'NONE',  ( -198.0356074513804288, -39.15871834505936278, 39.15871834505892224 ) ) ;
#17223=CARTESIAN_POINT ( 'NONE',  ( -192.9588430854690273, -14.46834944099973264, -40.00000000000002132 ) ) ;
#17225=CARTESIAN_POINT ( 'NONE',  ( 91.82158438592158234, 7.693928927950222250E-14, -17.20528682183300262 ) ) ;
#17226=CARTESIAN_POINT ( 'NONE',  ( 57.59792236341147031, -2.435789363418150444, 0.000000000000000000 ) ) ;
#17227=CARTESIAN_POINT ( 'NONE',  ( 19.06497207195980792, -18.24870850772763475, 38.31983398719622613 ) ) ;
#17228=CARTESIAN_POINT ( 'NONE',  ( -86.96347745069644475, 18.24025645688351105, 2.449293598294708485E-15 ) ) ;
#17229=VERTEX_POINT ( 'NONE', #1308 ) ;
#17230=CARTESIAN_POINT ( 'NONE',  ( 8.209392600961981756, -44.89226883836379045, 24.84362085273889065 ) ) ;
#17232=CARTESIAN_POINT ( 'NONE',  ( -135.8532207217289738, 30.84685318188643777, -40.00000000000002132 ) ) ;
#17234=CARTESIAN_POINT ( 'NONE',  ( 4.995406935893290878, 39.06748935135185263, 39.06748935135198764 ) ) ;
#17235=CARTESIAN_POINT ( 'NONE',  ( -238.4067589809705794, -4.716212492215116094E-14, 0.9644942799825824142 ) ) ;
#17236=CARTESIAN_POINT ( 'NONE',  ( -82.23757706630857456, 20.18845287563442170, 0.8296373908661033303 ) ) ;
#17240=CARTESIAN_POINT ( 'NONE',  ( -77.90022806218999563, 8.352332316461417605, -20.16431395584788433 ) ) ;
#17242=CARTESIAN_POINT ( 'NONE',  ( -208.1127848780265026, 10.60833733269551615, -10.60833733269529766 ) ) ;
#17243=CARTESIAN_POINT ( 'NONE',  ( 169.9999999999999432, -21.59613885783095100, 12.70659020859084620 ) ) ;
#17244=CARTESIAN_POINT ( 'NONE',  ( -135.8532207217289738, -6.472252184284280396, 6.472252184284099208 ) ) ;
#17245=CARTESIAN_POINT ( 'NONE',  ( -198.0356074513804572, 17.40982414986501325, -39.15871834505897198 ) ) ;
#17247=CARTESIAN_POINT ( 'NONE',  ( 170.2234770963711128, 17.36149277826973503, 39.20704971665401217 ) ) ;
#17248=CARTESIAN_POINT ( 'NONE',  ( -77.90255099906769942, -20.29001641120661859, 8.064892378658379712 ) ) ;
#17249=CARTESIAN_POINT ( 'NONE',  ( -30.26275506840324070, -1.198031551616016266, -1.198031551616031587 ) ) ;
#17251=DIRECTION ( 'NONE',  ( 0.9352143323239846540, 0.3271292299042263818, -0.1355013636760585005 ) ) ;
#17252=CARTESIAN_POINT ( 'NONE',  ( -259.2033419157646676, -6.730120644403663199, 6.730120644403451813 ) ) ;
#17253=CARTESIAN_POINT ( 'NONE',  ( 192.4448373802101173, 42.42640687116487896, 14.14213562375934075 ) ) ;
#17254=CARTESIAN_POINT ( 'NONE',  ( -213.1075012329537230, 13.71589010951907994, 0.000000000000000000 ) ) ;
#17255=CARTESIAN_POINT ( 'NONE',  ( -213.1075012329537230, 37.98287015391236565, -18.58567234101138510 ) ) ;
#17257=CARTESIAN_POINT ( 'NONE',  ( -30.26275506840322294, -57.76657404653985139, -1.198031551616531853 ) ) ;
#17258=EDGE_CURVE ( 'NONE', #8490, #15233, #14046, .T. ) ;
#17259=CARTESIAN_POINT ( 'NONE',  ( -129.2303492452213334, 24.84170067253468162, -11.67678589738752670 ) ) ;
#17262=CARTESIAN_POINT ( 'NONE',  ( 170.2234770963711128, 10.92277846919201068, 10.92277846919202133 ) ) ;
#17264=CARTESIAN_POINT ( 'NONE',  ( 20.69615274311417963, 13.93598092273866840, 47.71500688528227130 ) ) ;
#17265=CARTESIAN_POINT ( 'NONE',  ( -70.28815428308283231, -22.81668038576722424, -9.450978466024738012 ) ) ;
#17267=CARTESIAN_POINT ( 'NONE',  ( -144.0562564041998712, -31.27039870039539338, 10.50946916240340201 ) ) ;
#17270=CARTESIAN_POINT ( 'NONE',  ( 22.70429368897842437, -17.89136451867717881, 43.19357487035005505 ) ) ;
#17271=B_SPLINE_CURVE_WITH_KNOTS ( 'NONE', 3,
 ( #681, #25034, #2278, #417, #16371, #8790, #279, #8521, #2816, #6787, #19036, #14507 ),
 .UNSPECIFIED., .F., .F.,
 ( 4, 2, 2, 2, 2, 4 ),
 ( 1.398578778534940505E-17, 0.004680202113614262589, 0.009360404227228511301, 0.01170050528403563696, 0.01404060634084276088, 0.01872080845445705036 ),
 .UNSPECIFIED. ) ;
#17272=CARTESIAN_POINT ( 'NONE',  ( 60.28378959960998174, 15.72633063278336785, -31.18416451506176656 ) ) ;
#17274=CARTESIAN_POINT ( 'NONE',  ( 146.6084372240433709, -32.08495691632075619, 24.48358557860298035 ) ) ;
#17275=CARTESIAN_POINT ( 'NONE',  ( -86.96347745069644475, 5.999880687339585546E-14, -21.75974354311649961 ) ) ;
#17277=AXIS2_PLACEMENT_3D ( 'NONE', #25731, #3247, #9620 ) ;
#17280=CARTESIAN_POINT ( 'NONE',  ( 184.8905102610680444, 20.92133201514447194, -40.00000000000002132 ) ) ;
#17281=CARTESIAN_POINT ( 'NONE',  ( 23.40652632868016880, -13.79856377312466975, -46.79646383233838947 ) ) ;
#17283=CARTESIAN_POINT ( 'NONE',  ( -280.0000000000000000, 19.99999999999996092, -0.000000000000000000 ) ) ;
#17284=CARTESIAN_POINT ( 'NONE',  ( -135.8532207217289738, 6.472252184284186249, -6.472252184284142729 ) ) ;
#17285=CARTESIAN_POINT ( 'NONE',  ( -192.9588430854690273, 40.00000000000014211, -14.46834944099927966 ) ) ;
#17286=CARTESIAN_POINT ( 'NONE',  ( -110.0471271032897960, 8.580892274481946913, -18.26740471933098675 ) ) ;
#17287=CARTESIAN_POINT ( 'NONE',  ( 136.1360204305621551, -39.99999999999994316, -4.966164525587488221 ) ) ;
#17288=CARTESIAN_POINT ( 'NONE',  ( 126.3221657595859568, -28.30549010001853816, -11.72451788904508696 ) ) ;
#17290=CARTESIAN_POINT ( 'NONE',  ( -208.1127848780264742, 17.67593391476624021, 38.89260858015742883 ) ) ;
#17291=EDGE_CURVE ( 'NONE', #22653, #11219, #3264, .T. ) ;
#17295=CARTESIAN_POINT ( 'NONE',  ( 12.77879914706121234, 44.80239647191536534, -18.55776024547099823 ) ) ;
#17296=CARTESIAN_POINT ( 'NONE',  ( 192.4448373802101173, -19.99999999996057554, 40.00000000000002132 ) ) ;
#17298=CARTESIAN_POINT ( 'NONE',  ( -192.9370391624948411, 48.35015248260834397, -14.03127550870980222 ) ) ;
#17302=CARTESIAN_POINT ( 'NONE',  ( -86.96347745069644475, 15.38646221621793586, -15.38646221621778842 ) ) ;
#17303=CARTESIAN_POINT ( 'NONE',  ( 98.29820294267318559, -18.47759065023121039, -7.653668647304145090 ) ) ;
#17305=ORIENTED_EDGE ( 'NONE', *, *, #3959, .F. ) ;
#17308=CARTESIAN_POINT ( 'NONE',  ( 14.38125909742181285, -17.55144818341476309, 39.01709431150910490 ) ) ;
#17310=CARTESIAN_POINT ( 'NONE',  ( -162.0762913951020892, -3.568845385355699554E-14, 1.694272876828323948 ) ) ;
#17311=CARTESIAN_POINT ( 'NONE',  ( 190.0000000000001137, -30.00000000000000711, 3.673940397442064700E-15 ) ) ;
#17313=CARTESIAN_POINT ( 'NONE',  ( -30.26275506840323359, -39.99999999999959499, -41.69427246844670520 ) ) ;
#17314=CARTESIAN_POINT ( 'NONE',  ( -162.0762913951021176, 40.00000000000042633, -41.69427287672947102 ) ) ;
#17315=FACE_OUTER_BOUND ( 'NONE', #2160, .T. ) ;
#17316=CARTESIAN_POINT ( 'NONE',  ( 57.59792236341147031, 1.722363176415065089, -1.722363176415036445 ) ) ;
#17318=CARTESIAN_POINT ( 'NONE',  ( -192.9370391625626837, 14.03127550871173668, 48.35015248262227772 ) ) ;
#17320=CARTESIAN_POINT ( 'NONE',  ( -77.55672185583976841, 16.64541244683857713, -14.65061613763128534 ) ) ;
#17322=CARTESIAN_POINT ( 'NONE',  ( -77.84504298479346573, -19.81984129311347331, 9.297284891546427232 ) ) ;
#17323=CARTESIAN_POINT ( 'NONE',  ( -105.3755690713226727, 12.89780903124400879, 12.89780903124407452 ) ) ;
#17324=CARTESIAN_POINT ( 'NONE',  ( -238.4067589809705794, -28.96627169325352469, 27.60227080167035041 ) ) ;
#17328=CARTESIAN_POINT ( 'NONE',  ( 91.82158438592158234, 44.40256751092319121, 12.16597498400105515 ) ) ;
#17329=CARTESIAN_POINT ( 'NONE',  ( 23.37394308801976450, 13.80096434448266685, 46.80823611210199431 ) ) ;
#17331=ORIENTED_EDGE ( 'NONE', *, *, #15952, .F. ) ;
#17332=CARTESIAN_POINT ( 'NONE',  ( 146.6084372240433709, -40.00000000000036238, 34.62501878078263218 ) ) ;
#17333=CARTESIAN_POINT ( 'NONE',  ( -3.069599232962567648, -23.65302469262814000, 43.28003856805346317 ) ) ;
#17334=CARTESIAN_POINT ( 'NONE',  ( 3.854700064722261565, -44.60002223906898422, 24.62824689552009261 ) ) ;
#17335=ORIENTED_EDGE ( 'NONE', *, *, #25881, .F. ) ;
#17338=CARTESIAN_POINT ( 'NONE',  ( -195.1685814578706015, -44.46431112711578493, -24.52825302094467830 ) ) ;
#17339=CARTESIAN_POINT ( 'NONE',  ( 57.59792236341146321, 40.00000000000004263, -2.435789363418021214 ) ) ;
#17341=B_SPLINE_CURVE_WITH_KNOTS ( 'NONE', 3,
 ( #8577, #4207, #16688, #24820, #16292, #16157 ),
 .UNSPECIFIED., .F., .F.,
 ( 4, 2, 4 ),
 ( 1.484016138952788438E-15, 0.03937685683732576603, 0.07875371367465004713 ),
 .UNSPECIFIED. ) ;
#17342=FACE_BOUND ( 'NONE', #6630, .T. ) ;
#17343=CARTESIAN_POINT ( 'NONE',  ( 4.995406935893297984, -40.00000000000007816, 15.24977328854818914 ) ) ;
#17346=CARTESIAN_POINT ( 'NONE',  ( 91.82158438592158234, -12.16597498397778843, 12.16597498397750954 ) ) ;
#17347=CARTESIAN_POINT ( 'NONE',  ( 0.2972598230769923355, 18.14793986248751168, -38.42060263243650553 ) ) ;
#17348=CARTESIAN_POINT ( 'NONE',  ( -89.91461477837958682, 20.29478540188764413, 8.406375358913457774 ) ) ;
#17349=CARTESIAN_POINT ( 'NONE',  ( -198.0356074513804572, 5.461327841961909642E-13, -55.37879056873073580 ) ) ;
#17350=CARTESIAN_POINT ( 'NONE',  ( 98.29820294272414571, 7.653668647302724892, 18.47759065022804137 ) ) ;
#17351=CARTESIAN_POINT ( 'NONE',  ( 199.9999999999999432, 20.00000000000013856, 0.000000000000000000 ) ) ;
#17352=CARTESIAN_POINT ( 'NONE',  ( 19.06497207195981858, -10.03556273973469715, 66.60410523465813526 ) ) ;
#17353=CARTESIAN_POINT ( 'NONE',  ( 170.2234770963711128, 24.55285855007190676, -40.00000000000002132 ) ) ;
#17355=CARTESIAN_POINT ( 'NONE',  ( 21.15138808362603839, -43.47948264999420331, -23.80076113581845831 ) ) ;
#17356=CARTESIAN_POINT ( 'NONE',  ( 163.1118516004056573, 1.251511021549353291E-13, -27.26290988616872824 ) ) ;
#17357=CARTESIAN_POINT ( 'NONE',  ( -280.0000000000000000, 14.14213562373088351, 14.14213562373098654 ) ) ;
#17358=CARTESIAN_POINT ( 'NONE',  ( 91.82158438592158234, 22.79471317813472098, 2.449293598294708485E-15 ) ) ;
#17361=CARTESIAN_POINT ( 'NONE',  ( 17.24092899316222827, -44.34059580270437095, 18.36647614520138205 ) ) ;
#17363=CARTESIAN_POINT ( 'NONE',  ( -86.96347745069644475, -15.38646221621796073, 41.18208027870593924 ) ) ;
#17364=CARTESIAN_POINT ( 'NONE',  ( 4.995406935893290878, -5.232665749138292703E-14, 15.24977328854832592 ) ) ;
#17365=CARTESIAN_POINT ( 'NONE',  ( -77.58090675230904765, 21.99687198915249908, -2.639383879333266236 ) ) ;
#17366=B_SPLINE_CURVE_WITH_KNOTS ( 'NONE', 3,
 ( #18520, #301, #2173, #8008, #12525, #20263 ),
 .UNSPECIFIED., .F., .F.,
 ( 4, 2, 4 ),
 ( -6.000000000146255584E-08, 0.04016968421219987984, 0.08033942842439978360 ),
 .UNSPECIFIED. ) ;
#17367=CARTESIAN_POINT ( 'NONE',  ( 22.40986519363266538, -13.85314893102481903, -47.15972762675180974 ) ) ;
#17370=CARTESIAN_POINT ( 'NONE',  ( -77.55632011649659319, 0.6824138086283418891, -22.13182254413152705 ) ) ;
#17371=CARTESIAN_POINT ( 'NONE',  ( 184.8905102610680444, 13.49065550809757497, 43.07788698682593065 ) ) ;
#17373=CARTESIAN_POINT ( 'NONE',  ( 136.1360204305621266, 53.05693388239320285, -3.511608612530223716 ) ) ;
#17374=CARTESIAN_POINT ( 'NONE',  ( 192.4448373802101173, 14.14213562375862665, 42.42640687116509213 ) ) ;
#17376=CARTESIAN_POINT ( 'NONE',  ( -56.48582580120558561, -21.81201906317755146, -21.81201906317792449 ) ) ;
#17377=CARTESIAN_POINT ( 'NONE',  ( 163.1118516004056573, 19.27778845539265618, -37.29075403953135037 ) ) ;
#17378=CARTESIAN_POINT ( 'NONE',  ( -280.0000000000000000, -14.14213562373118549, 14.14213562373078936 ) ) ;
#17379=CARTESIAN_POINT ( 'NONE',  ( -105.3755690713226585, -15.38646221621738164, -41.18208027870615240 ) ) ;
#17380=CARTESIAN_POINT ( 'NONE',  ( 184.8905102610680444, -20.92133201514440799, -40.00000000000002132 ) ) ;
#17383=CARTESIAN_POINT ( 'NONE',  ( 57.59792236341147031, -26.56190807104712448, 30.00663442387673285 ) ) ;
#17384=CARTESIAN_POINT ( 'NONE',  ( -188.2870673237731012, 43.00153493964115370, -23.44688076656412434 ) ) ;
#17386=CARTESIAN_POINT ( 'NONE',  ( 0.2972598230769907257, 66.70487387989857098, 10.13633138497486641 ) ) ;
#17387=CARTESIAN_POINT ( 'NONE',  ( -77.78737254111192101, -19.58908437138761727, -9.951945538203670338 ) ) ;
#17388=CARTESIAN_POINT ( 'NONE',  ( 37.15749683965372441, 12.76981037574219968, 41.79699086514150252 ) ) ;
#17389=CARTESIAN_POINT ( 'NONE',  ( -39.81953879990965817, -34.34246706537491889, -11.17638696932914932 ) ) ;
#17390=EDGE_LOOP ( 'NONE', ( #2454, #20720, #23016, #1043, #25589, #24071, #15289 ) ) ;
#17391=CARTESIAN_POINT ( 'NONE',  ( -188.8383598209452998, -43.28885971699677526, 17.93083279444634215 ) ) ;
#17393=CARTESIAN_POINT ( 'NONE',  ( 22.92196489051308816, -13.82589419143179121, 46.97629733301284460 ) ) ;
#17395=CARTESIAN_POINT ( 'NONE',  ( -112.9836683000657587, 19.65633339690261749, 8.141919879520816750 ) ) ;
#17397=CARTESIAN_POINT ( 'NONE',  ( -77.55640685876514340, -1.398619866344356533, 22.13135000837099753 ) ) ;
#17398=CARTESIAN_POINT ( 'NONE',  ( -259.2033419157646676, 40.00000000000000711, -9.517827891722491884 ) ) ;
#17399=CARTESIAN_POINT ( 'NONE',  ( 57.59792236341147031, 1.908507979671054758E-14, -2.435789363418160658 ) ) ;
#17401=CARTESIAN_POINT ( 'NONE',  ( -213.1075012329537230, -53.71589010953668719, -40.00000000000002132 ) ) ;
#17402=CARTESIAN_POINT ( 'NONE',  ( 67.67011021016655548, -12.13550330130990851, -29.29769665558049851 ) ) ;
#17404=CARTESIAN_POINT ( 'NONE',  ( -162.0762913951021176, -1.694272876828353702, 40.00000000000002132 ) ) ;
#17405=CARTESIAN_POINT ( 'NONE',  ( 192.4448373802100889, 14.14213562375893574, -14.14213562375874922 ) ) ;
#17406=CARTESIAN_POINT ( 'NONE',  ( 151.7948205124836250, -3.202120068677277203E-13, 33.23291073765553705 ) ) ;
#17407=CARTESIAN_POINT ( 'NONE',  ( -91.56559293963834989, -40.00000000000027711, 22.67402823373149801 ) ) ;
#17410=CARTESIAN_POINT ( 'NONE',  ( 105.6376868227169297, -21.14845495492350480, -8.759976865565771931 ) ) ;
#17413=CARTESIAN_POINT ( 'NONE',  ( -4.037857402784110761, 46.99101396955047250, -13.82822410908676858 ) ) ;
#17414=CARTESIAN_POINT ( 'NONE',  ( -208.1127848780264742, -15.00245453012673202, 40.00000000000002132 ) ) ;
#17416=DIRECTION ( 'NONE',  ( 0.01051738792036951628, 0.3656191332804069605, -0.9307051272721219570 ) ) ;
#17419=ORIENTED_EDGE ( 'NONE', *, *, #16483, .F. ) ;
#17421=CARTESIAN_POINT ( 'NONE',  ( 167.0466155511619490, 9.710058186601976615, -23.44215416552584230 ) ) ;
#17422=CARTESIAN_POINT ( 'NONE',  ( -89.92902785008706701, 8.088236460650101378, -20.44110050034134929 ) ) ;
#17428=CARTESIAN_POINT ( 'NONE',  ( 14.38125909742180397, 67.30136555895953165, 10.73282306403583242 ) ) ;
#17429=CARTESIAN_POINT ( 'NONE',  ( -199.9999999999999432, 42.45148791631907415, -35.57044988732096868 ) ) ;
#17430=CARTESIAN_POINT ( 'NONE',  ( -105.3755690713226727, 5.661656051307470077E-14, -21.75974354311649961 ) ) ;
#17432=CARTESIAN_POINT ( 'NONE',  ( -77.90255099906853786, 8.644468104252323926, -20.04994828524279882 ) ) ;
#17437=CARTESIAN_POINT ( 'NONE',  ( -135.8532207217289738, -40.00000000000014211, 9.153146818113153671 ) ) ;
#17438=CARTESIAN_POINT ( 'NONE',  ( -91.56559293963836410, 40.00000000000019185, -17.32597176626768487 ) ) ;
#17439=CARTESIAN_POINT ( 'NONE',  ( 170.2234770963711128, 17.36149277827004411, -17.36149277826983095 ) ) ;
#17440=CARTESIAN_POINT ( 'NONE',  ( -192.9588430854689989, -8.596193650988133061E-14, 14.46834944099969533 ) ) ;
#17441=CARTESIAN_POINT ( 'NONE',  ( -198.9234529670043798, 24.80620787431004004, 44.84148137681157209 ) ) ;
#17442=CARTESIAN_POINT ( 'NONE',  ( 137.0939645874030930, 30.33050608226186995, 12.56330697291266318 ) ) ;
#17443=CARTESIAN_POINT ( 'NONE',  ( -77.55640685876515761, -15.64922766773196905, -15.64922766773223195 ) ) ;
#17444=CARTESIAN_POINT ( 'NONE',  ( 0.2972598230769976091, -10.13633138497479180, 10.13633138497468522 ) ) ;
#17445=CARTESIAN_POINT ( 'NONE',  ( -77.79216379506679857, 20.86722748066878097, -6.767643439074305434 ) ) ;
#17446=CARTESIAN_POINT ( 'NONE',  ( 192.4448373802101173, -42.42640687122073473, 14.14213562370301780 ) ) ;
#17447=CARTESIAN_POINT ( 'NONE',  ( 170.2234770963711128, -10.92277846919187034, -10.92277846919209594 ) ) ;
#17449=CARTESIAN_POINT ( 'NONE',  ( 0.4289717129526279260, 24.25042218720268750, 44.08776571100843711 ) ) ;
#17451=CARTESIAN_POINT ( 'NONE',  ( 199.9999999999999432, 14.14213562373110911, -14.14213562373072364 ) ) ;
#17452=CARTESIAN_POINT ( 'NONE',  ( 163.1118516004056573, 27.26290988616875310, 0.000000000000000000 ) ) ;
#17453=CARTESIAN_POINT ( 'NONE',  ( -188.2995950289364089, -13.82811170417104840, -46.99046209955525200 ) ) ;
#17454=ORIENTED_EDGE ( 'NONE', *, *, #17746, .T. ) ;
#17455=CARTESIAN_POINT ( 'NONE',  ( 184.8905102610680444, -40.00000000000021316, 20.92133201514402430 ) ) ;
#17457=CARTESIAN_POINT ( 'NONE',  ( -77.90255099906772784, 8.644468104261493480, 20.04994828523958361 ) ) ;
#17458=VERTEX_POINT ( 'NONE', #24045 ) ;
#17461=CARTESIAN_POINT ( 'NONE',  ( -135.8532207217289738, -21.81201906317758343, -34.75652343174620995 ) ) ;
#17462=CARTESIAN_POINT ( 'NONE',  ( 91.82158438592158234, -6.516925787240506436E-14, 22.79471317813470321 ) ) ;
#17465=CARTESIAN_POINT ( 'NONE',  ( -56.48582580120558561, -1.205267837095813407E-13, 30.84685318188644132 ) ) ;
#17468=CARTESIAN_POINT ( 'NONE',  ( -77.55640685876515761, 15.64922766773205254, 15.64922766773212182 ) ) ;
#17469=CARTESIAN_POINT ( 'NONE',  ( 4.995406935893289102, 10.78321810389013002, -10.78321810388986712 ) ) ;
#17470=CARTESIAN_POINT ( 'NONE',  ( 14.38125909742180752, 17.55144818341503665, -39.01709431150898411 ) ) ;
#17471=CARTESIAN_POINT ( 'NONE',  ( -105.3175882261758147, -20.76660717853137683, 5.408274864390659076 ) ) ;
#17472=CARTESIAN_POINT ( 'NONE',  ( -213.1075012329537230, 5.259461644596141978E-13, -53.71589010951915100 ) ) ;
#17474=CARTESIAN_POINT ( 'NONE',  ( 0.2972598230769983307, -14.33493731733933352, 0.000000000000000000 ) ) ;
#17475=CARTESIAN_POINT ( 'NONE',  ( 170.2234770963711128, -15.44714144992812699, -40.00000000000002132 ) ) ;
#17476=CARTESIAN_POINT ( 'NONE',  ( 146.6084372240433709, 24.48358557860311180, 32.08495691632071356 ) ) ;
#17477=CARTESIAN_POINT ( 'NONE',  ( -198.0356074513804572, -55.37879056871328487, -40.00000000000002132 ) ) ;
#17479=CARTESIAN_POINT ( 'NONE',  ( -109.1264249741438448, 13.72187187124579211, 33.12752917268907993 ) ) ;
#17480=CARTESIAN_POINT ( 'NONE',  ( -100.7734535825088358, -2.560096224687585342E-13, 22.67402823373191723 ) ) ;
#17481=CARTESIAN_POINT ( 'NONE',  ( 136.1360204305621551, -24.77266263493126885, 31.79587985999256006 ) ) ;
#17482=CARTESIAN_POINT ( 'NONE',  ( 0.2972598230769930017, 54.33493731733938148, -40.00000000000002132 ) ) ;
#17484=CARTESIAN_POINT ( 'NONE',  ( 23.35901252181239229, -46.81387818480112628, 13.80180065670254663 ) ) ;
#17487=CARTESIAN_POINT ( 'NONE',  ( -135.8532207217289738, 21.81201906317767936, 21.81201906317778239 ) ) ;
#17489=CARTESIAN_POINT ( 'NONE',  ( -77.55380018288633437, 22.14554968447874472, -1.229295861724395866 ) ) ;
#17490=CARTESIAN_POINT ( 'NONE',  ( -7.297127544328012583, 13.59739983758589865, -45.86058602274966489 ) ) ;
#17494=CARTESIAN_POINT ( 'NONE',  ( -77.67315633212632520, -4.804802313621894250, -21.50043107020669098 ) ) ;
#17495=CARTESIAN_POINT ( 'NONE',  ( 146.6084372240433993, -24.48358557860353457, 24.48358557860296258 ) ) ;
#17496=CARTESIAN_POINT ( 'NONE',  ( -56.48582580120558561, 6.472252184284607246, -50.09629031063960269 ) ) ;
#17498=DIRECTION ( 'NONE',  ( 0.000000000000000000, 0.7071067811865443531, 0.7071067811865507924 ) ) ;
#17499=CARTESIAN_POINT ( 'NONE',  ( 19.06497207195982568, -38.31983398719592770, -38.31983398719660272 ) ) ;
#17501=CARTESIAN_POINT ( 'NONE',  ( 91.82158438592156813, 40.45024623143973486, -16.11829626348390931 ) ) ;
#17502=CARTESIAN_POINT ( 'NONE',  ( -105.3755690713226585, -43.67073346367964604, -12.89780903124457545 ) ) ;
#17503=CARTESIAN_POINT ( 'NONE',  ( 170.2234770963711128, 39.20704971665372796, 17.36149277827039583 ) ) ;
#17505=CARTESIAN_POINT ( 'NONE',  ( 199.9999999999999432, -14.14213562373096345, -14.14213562373104871 ) ) ;
#17507=CARTESIAN_POINT ( 'NONE',  ( -238.4067589809705794, -0.6820004457913585449, -0.6820004457913265705 ) ) ;
#17508=CARTESIAN_POINT ( 'NONE',  ( -105.3755690713226585, 18.24025645688349684, 40.00000000000002132 ) ) ;
#17509=VERTEX_POINT ( 'NONE', #12331 ) ;
#17511=CARTESIAN_POINT ( 'NONE',  ( 4.995406935893283773, 39.06748935135195211, -17.50105314357185193 ) ) ;
#17512=CARTESIAN_POINT ( 'NONE',  ( 26.79002001241197561, 41.25333065883494044, 17.08768905195128340 ) ) ;
#17513=CARTESIAN_POINT ( 'NONE',  ( 83.06440094970915311, 10.91839312111565263, 23.65491511366958832 ) ) ;
#17514=CARTESIAN_POINT ( 'NONE',  ( -4.660840668352645544, -42.82207049670927290, -23.32816686155640440 ) ) ;
#17517=CARTESIAN_POINT ( 'NONE',  ( -188.8948201289225608, -43.30398576617490392, 17.93709820916094699 ) ) ;
#17519=CARTESIAN_POINT ( 'NONE',  ( 22.79879570922440024, -17.88067497375698522, 43.16776802602890228 ) ) ;
#17520=EDGE_CURVE ( 'NONE', #2033, #20449, #16262, .T. ) ;
#17521=CARTESIAN_POINT ( 'NONE',  ( 36.88256715627346694, 16.19941669821687569, -39.10885149560213847 ) ) ;
#17523=CARTESIAN_POINT ( 'NONE',  ( -97.72675010090307524, -20.56394680065911729, -8.987772175319559409 ) ) ;
#17524=CARTESIAN_POINT ( 'NONE',  ( 151.7948205124836534, 40.00000000000017053, -33.23291073765538783 ) ) ;
#17525=CARTESIAN_POINT ( 'NONE',  ( -77.90255099906771363, -8.064892378658779393, 20.29001641120648003 ) ) ;
#17527=CARTESIAN_POINT ( 'NONE',  ( 151.7948205124836534, -6.767089262349006873, 40.00000000000002132 ) ) ;
#17529=DIRECTION ( 'NONE',  ( 1.000000000000000000, 1.836970198721030181E-16, -0.000000000000000000 ) ) ;
#17530=CARTESIAN_POINT ( 'NONE',  ( 19.06497207195982924, -54.19242893257843008, 40.00000000000002132 ) ) ;
#17531=CARTESIAN_POINT ( 'NONE',  ( -280.0000000000000000, 19.99999999999996092, -0.000000000000000000 ) ) ;
#17532=CARTESIAN_POINT ( 'NONE',  ( 91.82158438592158234, -17.20528682183298486, 0.000000000000000000 ) ) ;
#17533=CARTESIAN_POINT ( 'NONE',  ( 91.82158438592156813, 39.99999999999986500, 17.20528682183341473 ) ) ;
#17534=CARTESIAN_POINT ( 'NONE',  ( -86.96347745069643054, -39.99999999999985079, -18.24025645688394448 ) ) ;
#17535=CARTESIAN_POINT ( 'NONE',  ( 146.5085219967539842, -29.94471555035083199, -12.40350730235989829 ) ) ;
#17538=CARTESIAN_POINT ( 'NONE',  ( -1.087763065927251471, 43.78960619332519855, -24.03018639662559508 ) ) ;
#17539=CARTESIAN_POINT ( 'NONE',  ( -86.96347745069643054, -18.24025645688353947, 40.00000000000002132 ) ) ;
#17541=CARTESIAN_POINT ( 'NONE',  ( -190.7345856381636793, 43.65254615102346492, -23.92884448221996152 ) ) ;
#17544=ORIENTED_EDGE ( 'NONE', *, *, #4556, .T. ) ;
#17546=CARTESIAN_POINT ( 'NONE',  ( 149.5797498300189545, 12.18602109748342777, -29.41965740490875802 ) ) ;
#17549=EDGE_LOOP ( 'NONE', ( #24868, #11788, #6143, #21648 ) ) ;
#17552=CARTESIAN_POINT ( 'NONE',  ( 151.7948205124836534, 33.06932595376365924, -23.49921654116018743 ) ) ;
#17553=CARTESIAN_POINT ( 'NONE',  ( -199.9999999999999716, 35.57044988732193502, -42.45148791632000496 ) ) ;
#17554=CARTESIAN_POINT ( 'NONE',  ( -238.4067589809705794, -4.716212492215116094E-14, 0.9644942799825824142 ) ) ;
#17555=CARTESIAN_POINT ( 'NONE',  ( 23.37394308801977871, -13.80096434448300613, 46.80823611210190904 ) ) ;
#17557=CARTESIAN_POINT ( 'NONE',  ( -238.4067589809705794, -4.716212492215116094E-14, 0.9644942799825824142 ) ) ;
#17558=CARTESIAN_POINT ( 'NONE',  ( -53.37717264285771535, -29.42738956023914199, -10.11115224722892769 ) ) ;
#17559=CARTESIAN_POINT ( 'NONE',  ( -213.1075012329537230, -39.99999999999948841, -53.71589010950208376 ) ) ;
#17560=CARTESIAN_POINT ( 'NONE',  ( -114.5444905533725262, -9.939131763645404405, 19.55376799570613500 ) ) ;
#17561=CARTESIAN_POINT ( 'NONE',  ( 146.6084372240433993, 24.48358557860341733, -24.48358557860313311 ) ) ;
#17562=CARTESIAN_POINT ( 'NONE',  ( -259.2033419157646676, -1.438356298054549103E-14, -9.517827891722632216 ) ) ;
#17563=CARTESIAN_POINT ( 'NONE',  ( 146.6084372240433993, 24.48358557860341733, -24.48358557860313311 ) ) ;
#17564=CARTESIAN_POINT ( 'NONE',  ( 153.3020327024398171, 28.42252382389414933, 11.77299484472951541 ) ) ;
#17567=CARTESIAN_POINT ( 'NONE',  ( 19.06497207195981147, -10.03556273973439517, 10.03556273973429214 ) ) ;
#17568=CARTESIAN_POINT ( 'NONE',  ( 0.2972598230769957217, -4.999556039334937811E-14, 14.33493731733933352 ) ) ;
#17569=CARTESIAN_POINT ( 'NONE',  ( -100.7734535825088500, -16.03295912088716335, 40.53558337403673306 ) ) ;
#17570=CARTESIAN_POINT ( 'NONE',  ( 91.82158438592159655, -44.40256751092341858, 12.16597498400012434 ) ) ;
#17571=CARTESIAN_POINT ( 'NONE',  ( -129.2303573020097645, -11.67678754046080591, -24.84170325987118133 ) ) ;
#17572=CARTESIAN_POINT ( 'NONE',  ( 170.0000000000000853, 9.369682556672316309, -22.62041470344884075 ) ) ;
#17574=CARTESIAN_POINT ( 'NONE',  ( 0.2972598230769959993, 38.42060263243713081, -38.42060263243619289 ) ) ;
#17578=CARTESIAN_POINT ( 'NONE',  ( 19.06497207195981858, -39.99999999999987210, -14.19242893257882621 ) ) ;
#17579=EDGE_CURVE ( 'NONE', #14912, #3577, #2396, .T. ) ;
#17581=CARTESIAN_POINT ( 'NONE',  ( -47.50817905881373804, 12.56548180736879772, 30.33575659748668940 ) ) ;
#17582=ORIENTED_EDGE ( 'NONE', *, *, #24937, .T. ) ;
#17584=CARTESIAN_POINT ( 'NONE',  ( 170.2234770963711128, 17.36149277827004411, -17.36149277826983095 ) ) ;
#17585=CARTESIAN_POINT ( 'NONE',  ( 136.1360204305621266, 5.219216885335291329E-15, 4.966164525587064560 ) ) ;
#17586=CARTESIAN_POINT ( 'NONE',  ( -88.37877758187804034, -20.15391234954027055, -8.026456973411162821 ) ) ;
#17588=CARTESIAN_POINT ( 'NONE',  ( 14.38125909742181818, -1.924622159709266762E-13, 55.17850393972636880 ) ) ;
#17590=CARTESIAN_POINT ( 'NONE',  ( -259.2033419157646676, -1.438356298054549103E-14, -9.517827891722632216 ) ) ;
#17592=CARTESIAN_POINT ( 'NONE',  ( -4.580761711675023662, -17.81010960708106339, -42.99740816077124350 ) ) ;
#17593=CARTESIAN_POINT ( 'NONE',  ( 192.4448373802101173, 42.42640687122089815, -14.14213562370272470 ) ) ;
#17595=CARTESIAN_POINT ( 'NONE',  ( -199.9999999999998579, 44.86878812508723513, -24.82633483071237634 ) ) ;
#17596=CARTESIAN_POINT ( 'NONE',  ( -91.56559293963834989, -2.543181659092656077E-13, 22.67402823373191723 ) ) ;
#17597=CARTESIAN_POINT ( 'NONE',  ( 85.88498456118406921, 8.769910164384999263, 23.37206003906720397 ) ) ;
#17598=CARTESIAN_POINT ( 'NONE',  ( -238.4067589809705794, -0.9644942799826262680, 0.000000000000000000 ) ) ;
#17599=CARTESIAN_POINT ( 'NONE',  ( -30.26275506840323004, -41.69427246844627888, -40.00000000000002132 ) ) ;
#17600=CARTESIAN_POINT ( 'NONE',  ( -280.0000000000000568, 42.42640687119274645, 14.14213562373118194 ) ) ;
#17601=CARTESIAN_POINT ( 'NONE',  ( 4.995406935893294431, -15.24977328854832415, -40.00000000000002132 ) ) ;
#17602=CARTESIAN_POINT ( 'NONE',  ( 22.68416413276407795, -43.06288726621011875, -23.49220544186193038 ) ) ;
#17603=CARTESIAN_POINT ( 'NONE',  ( -86.95492397413735830, -9.645500094587582396, -19.11844798802007617 ) ) ;
#17604=CARTESIAN_POINT ( 'NONE',  ( -91.56559293963834989, -2.543181659092656077E-13, 22.67402823373191723 ) ) ;
#17605=CARTESIAN_POINT ( 'NONE',  ( -86.96347745069644475, 12.89780903124401057, 12.89780903124407629 ) ) ;
#17607=CARTESIAN_POINT ( 'NONE',  ( -135.8532207217289738, 30.84685318188643066, 2.449293598294708485E-15 ) ) ;
#17609=CARTESIAN_POINT ( 'NONE',  ( 23.35901252181232479, -42.86175755505330898, 23.34306388117434139 ) ) ;
#17610=CARTESIAN_POINT ( 'NONE',  ( -77.90255099906767100, -8.064892378658175431, 20.29001641120675004 ) ) ;
#17611=CARTESIAN_POINT ( 'NONE',  ( 200.0000000000000000, -14.14213562373106114, 42.42640687119278908 ) ) ;
#17612=CARTESIAN_POINT ( 'NONE',  ( -30.26275506840324070, -40.00000000000003553, 1.694272468446120117 ) ) ;
#17613=CARTESIAN_POINT ( 'NONE',  ( 0.2972598230769938343, 10.13633138497486286, -10.13633138497461594 ) ) ;
#17614=CARTESIAN_POINT ( 'NONE',  ( 19.06497207195980792, 14.19242893257840699, -40.00000000000002132 ) ) ;
#17615=CARTESIAN_POINT ( 'NONE',  ( -114.4364955367327497, -20.04994829327637262, -8.644468109209869411 ) ) ;
#17617=CARTESIAN_POINT ( 'NONE',  ( -77.70933353446504555, -5.475739710260814519, -21.30703284266700592 ) ) ;
#17618=CARTESIAN_POINT ( 'NONE',  ( -208.1127848780265026, 10.60833733269551615, -10.60833733269529766 ) ) ;
#17619=CARTESIAN_POINT ( 'NONE',  ( -208.1127848780264742, -38.89260858015704514, -38.89260858015768463 ) ) ;
#17620=( GEOMETRIC_REPRESENTATION_CONTEXT ( 3 ) GLOBAL_UNCERTAINTY_ASSIGNED_CONTEXT ( ( #11221 ) ) GLOBAL_UNIT_ASSIGNED_CONTEXT ( ( #25985, #24513, #13985 ) ) REPRESENTATION_CONTEXT ( 'NONE', 'WORKASPACE' ) );
#17621=CARTESIAN_POINT ( 'NONE',  ( -77.70103186979810062, -21.35019956121274731, -5.501793373024266742 ) ) ;
#17623=CARTESIAN_POINT ( 'NONE',  ( -213.1075012329537230, -9.698598906462304825, -66.26714140138675191 ) ) ;
#17624=CARTESIAN_POINT ( 'NONE',  ( -86.96347745069643054, 15.38646221621821297, -41.18208027870583265 ) ) ;
#17625=CARTESIAN_POINT ( 'NONE',  ( 151.7948205124836534, -23.49921654115981084, -33.06932595376387951 ) ) ;
#17626=CARTESIAN_POINT ( 'NONE',  ( -86.96347745069644475, -15.38646221621807442, 15.38646221621768184 ) ) ;
#17629=CARTESIAN_POINT ( 'NONE',  ( -192.9588430854690273, -40.00000000000011369, 14.46834944099955855 ) ) ;
#17631=CARTESIAN_POINT ( 'NONE',  ( 184.8905102610680444, 14.79361573936375507, 14.79361573936398067 ) ) ;
#17632=AXIS2_PLACEMENT_3D ( 'NONE', #23988, #7747, #13876 ) ;
#17633=CARTESIAN_POINT ( 'NONE',  ( 130.8568914410475088, -34.05028731879786363, 40.00000000000002132 ) ) ;
#17635=CARTESIAN_POINT ( 'NONE',  ( -280.0000000000000000, -14.14213562373098831, -14.14213562373098654 ) ) ;
#17637=CARTESIAN_POINT ( 'NONE',  ( 22.98934664983071841, 17.85845455616048483, 43.11412319250736402 ) ) ;
#17638=CARTESIAN_POINT ( 'NONE',  ( 192.4448373802100889, -20.00000000003938538, 0.000000000000000000 ) ) ;
#17640=CARTESIAN_POINT ( 'NONE',  ( -188.4701769959648061, -47.05181236278195911, 13.83721050407064190 ) ) ;
#17644=CARTESIAN_POINT ( 'NONE',  ( 67.78092418467272751, -12.11998378903902385, 29.26022923861282266 ) ) ;
#17645=CARTESIAN_POINT ( 'NONE',  ( 13.28449813601589824, 14.15462405554525382, -49.16593779332317382 ) ) ;
#17647=AXIS2_PLACEMENT_3D ( 'NONE', #481, #16567, #19098 ) ;
#17649=CARTESIAN_POINT ( 'NONE',  ( 0.2972598230769956662, 39.99999999999983658, 54.33493731733950938 ) ) ;
#17650=CARTESIAN_POINT ( 'NONE',  ( -100.7734535825088358, 6.065416334915073333E-14, -22.67402823373191723 ) ) ;
#17652=CARTESIAN_POINT ( 'NONE',  ( -208.1127848780264742, -55.00245453010926866, 40.00000000000002132 ) ) ;
#17653=CARTESIAN_POINT ( 'NONE',  ( 67.79414719525901489, -14.15005687183196237, -28.72755866871360553 ) ) ;
#17655=CARTESIAN_POINT ( 'NONE',  ( -100.7734535825088500, 22.67402823373189946, 40.00000000000002132 ) ) ;
#17657=CARTESIAN_POINT ( 'NONE',  ( -238.4067589809705794, -40.96449427990185654, -40.00000000000002132 ) ) ;
#17658=CARTESIAN_POINT ( 'NONE',  ( 57.59792236341147031, -2.435789363418150000, 40.00000000000002132 ) ) ;
#17659=CARTESIAN_POINT ( 'NONE',  ( 146.6084372240433709, 40.00000000000010658, -5.374981219216549810 ) ) ;
#17660=CARTESIAN_POINT ( 'NONE',  ( -199.9999999999999432, 14.17215463606929227, 49.28189405767592746 ) ) ;
#17661=CARTESIAN_POINT ( 'NONE',  ( -162.0762913951020892, -1.198031840385767266, -1.198031840385758384 ) ) ;
#17663=CARTESIAN_POINT ( 'NONE',  ( -87.13361725327072804, 21.49321519333427233, -1.448021113139547951E-30 ) ) ;
#17664=CARTESIAN_POINT ( 'NONE',  ( 200.0000000000000000, 20.00000000000013856, 40.00000000000002132 ) ) ;
#17665=EDGE_CURVE ( 'NONE', #6802, #11453, #24177, .T. ) ;
#17666=CARTESIAN_POINT ( 'NONE',  ( -188.5332420855723683, 47.07509783863601172, -13.84065984176399233 ) ) ;
#17668=VERTEX_POINT ( 'NONE', #10745 ) ;
#17672=CARTESIAN_POINT ( 'NONE',  ( -87.13361725327072804, 8.813415818526478339E-15, 21.49321519333429009 ) ) ;
#17674=CARTESIAN_POINT ( 'NONE',  ( -198.0356074513804572, 15.37879056873066830, -40.00000000000002132 ) ) ;
#17675=CARTESIAN_POINT ( 'NONE',  ( -100.0968563617724527, -20.72609133247079427, 8.149320301504525688 ) ) ;
#17678=CARTESIAN_POINT ( 'NONE',  ( -188.5332420855686166, 13.84065984174896435, 47.07509783864872333 ) ) ;
#17680=CARTESIAN_POINT ( 'NONE',  ( -259.2033419157646676, 49.83842185052027673, -6.730120644403441155 ) ) ;
#17681=CARTESIAN_POINT ( 'NONE',  ( -199.9999999999999432, 39.01096890182095223, -39.01096890182004273 ) ) ;
#17682=CARTESIAN_POINT ( 'NONE',  ( 4.995406935893290878, -5.232665749138292703E-14, 15.24977328854832592 ) ) ;
#17683=CARTESIAN_POINT ( 'NONE',  ( 4.990270234119178028, -14.15117691407206379, 49.14367003637716635 ) ) ;
#17684=CARTESIAN_POINT ( 'NONE',  ( -83.21262154144253032, 13.72187187061549274, -33.12752917118393015 ) ) ;
#17687=CARTESIAN_POINT ( 'NONE',  ( 170.2234770963711128, -39.99999999999982947, -15.44714144992858529 ) ) ;
#17688=CARTESIAN_POINT ( 'NONE',  ( -105.2053629887588500, -15.67233752939762503, 14.72427054407682157 ) ) ;
#17689=CARTESIAN_POINT ( 'NONE',  ( 151.7948205124835681, -4.785054706298153882, -51.78348778862540058 ) ) ;
#17690=CARTESIAN_POINT ( 'NONE',  ( -208.1127848780265026, -9.061048840815752106E-14, 15.00245453012669472 ) ) ;
#17691=CARTESIAN_POINT ( 'NONE',  ( 57.59792236341148453, -54.84617931850877426, -1.722363176415331099 ) ) ;
#17692=CARTESIAN_POINT ( 'NONE',  ( -99.29480781227083241, 8.165122821357551075, 20.80016781325174335 ) ) ;
#17693=CARTESIAN_POINT ( 'NONE',  ( 98.29820294267528880, -14.14213562373450017, -14.14213562373441668 ) ) ;
#17694=CARTESIAN_POINT ( 'NONE',  ( 0.2972598230769883387, 40.00000000000017053, -14.33493731733891607 ) ) ;
#17695=CARTESIAN_POINT ( 'NONE',  ( -280.0000000000000568, -40.00000000000014211, 19.99999999999987210 ) ) ;
#17696=CARTESIAN_POINT ( 'NONE',  ( -105.3755690713226585, -15.38646221621796251, 41.18208027870593924 ) ) ;
#17697=( BOUNDED_CURVE ( )  B_SPLINE_CURVE ( 3, ( #20328, #2105, #22596, #12603 ),
 .UNSPECIFIED., .F., .F. ) 
 B_SPLINE_CURVE_WITH_KNOTS ( ( 4, 4 ),
 ( 0.01388163287021765106, 0.02359082919310009213 ),
 .UNSPECIFIED. ) 
 CURVE ( )  GEOMETRIC_REPRESENTATION_ITEM ( )  RATIONAL_B_SPLINE_CURVE ( ( 1.000000000000000000, 0.8672072324488967476, 0.7608653435686154598, 0.6809743333591562475 ) ) 
 REPRESENTATION_ITEM ( '' )  );
#17698=CARTESIAN_POINT ( 'NONE',  ( -162.0762913951020607, -57.76657433537922515, -1.198031840455874963 ) ) ;
#17699=CARTESIAN_POINT ( 'NONE',  ( -166.3490736461184838, -12.23457872956201697, -39.29841219602351288 ) ) ;
#17700=CARTESIAN_POINT ( 'NONE',  ( 130.8568914410475372, 24.07718906447243867, -24.07718906447216156 ) ) ;
#17702=CARTESIAN_POINT ( 'NONE',  ( 136.1360204305621551, 31.79587985999232558, 24.77266263493161702 ) ) ;
#17703=DIRECTION ( 'NONE',  ( 1.000000000000000000, 1.836970198721030181E-16, 0.000000000000000000 ) ) ;
#17706=CARTESIAN_POINT ( 'NONE',  ( -192.9588430854690273, 10.23066800229588758, -66.79921049721882298 ) ) ;
#17707=CARTESIAN_POINT ( 'NONE',  ( -99.21568817060988010, 22.67402823373189591, -0.000000000000000000 ) ) ;
#17709=DIRECTION ( 'NONE',  ( 0.3301743754003874098, 0.000000000000000000, -0.9439199552022214945 ) ) ;
#17711=CARTESIAN_POINT ( 'NONE',  ( -24.51100708734949052, 15.48921386281993051, 37.39427017793874342 ) ) ;
#17714=ORIENTED_EDGE ( 'NONE', *, *, #11104, .F. ) ;
#17715=CARTESIAN_POINT ( 'NONE',  ( -280.0000000000000568, -20.00000000000006750, -40.00000000000002132 ) ) ;
#17716=CARTESIAN_POINT ( 'NONE',  ( -194.4222169613648532, -44.35789444895097233, -24.44978956117715541 ) ) ;
#17717=CARTESIAN_POINT ( 'NONE',  ( 184.8905102610680444, -3.509827109981123710E-14, 19.07866798485558490 ) ) ;
#17720=DIRECTION ( 'NONE',  ( 0.3301743753925353575, 0.9439199552049681863, 0.000000000000000000 ) ) ;
#17721=CARTESIAN_POINT ( 'NONE',  ( 14.38125909742182529, -40.00000000000021316, 55.17850393974251944 ) ) ;
#17723=CARTESIAN_POINT ( 'NONE',  ( 14.38125909742181108, -5.035366881890652543E-14, 15.17850393972633682 ) ) ;
#17725=CARTESIAN_POINT ( 'NONE',  ( 130.8568914410475372, -24.07718906447255947, 24.07718906447199458 ) ) ;
#17726=CARTESIAN_POINT ( 'NONE',  ( -56.48582580120558561, 6.472252184284607246, -50.09629031063960269 ) ) ;
#17727=CARTESIAN_POINT ( 'NONE',  ( 98.29820294267314296, 18.47759065023127079, 7.653668647304074923 ) ) ;
#17729=CARTESIAN_POINT ( 'NONE',  ( 14.38125909742181108, 1.616281842095393922E-13, -15.17850393972633682 ) ) ;
#17730=CARTESIAN_POINT ( 'NONE',  ( -30.26275506840324425, -1.694272468446265334, 40.00000000000002132 ) ) ;
#17731=CARTESIAN_POINT ( 'NONE',  ( 19.06497207195980792, -14.19242893257839988, -40.00000000000002132 ) ) ;
#17732=CARTESIAN_POINT ( 'NONE',  ( 136.1360204305621266, 53.05693388239316022, 3.511608612530967566 ) ) ;
#17733=CARTESIAN_POINT ( 'NONE',  ( -192.9588430854690273, -54.46834944101725284, -40.00000000000002132 ) ) ;
#17735=CARTESIAN_POINT ( 'NONE',  ( 0.2972598230769957217, 1.502051041545559470E-13, -14.33493731733933352 ) ) ;
#17736=CARTESIAN_POINT ( 'NONE',  ( 57.59792236341147031, 54.84617931850881689, -1.722363176414946073 ) ) ;
#17737=CARTESIAN_POINT ( 'NONE',  ( 199.9999999999999432, 19.99999999999996092, 2.449293598294708485E-15 ) ) ;
#17738=ORIENTED_EDGE ( 'NONE', *, *, #7370, .F. ) ;
#17739=CARTESIAN_POINT ( 'NONE',  ( 90.68848816910541188, -21.47805809224183449, 8.337973097871099526 ) ) ;
#17740=CARTESIAN_POINT ( 'NONE',  ( 130.8888609958234497, 12.21841679119692792, 29.49786752803550627 ) ) ;
#17742=( BOUNDED_SURFACE ( )  B_SPLINE_SURFACE ( 3, 3, ( 
 ( #21467, #21224, #19341, #18961, #999, #23348, #23472, #13348, #24962, #10981, #1131, #19091, #9235, #871, #742, #14960, #8846, #15218, #7228, #8979, #22954, #15086, #16955, #2739, #25093, #17087, #2997, #11101, #25349, #25219 ),
 ( #23095, #3121, #11225, #1252, #6972, #7106, #4866, #19465, #5243, #6840, #3245, #4998, #9356, #19218, #9102, #6708, #17343, #14822, #17211, #5125, #4732, #25479, #12842, #20958, #13229, #12239, #9617, #10114, #14366, #16091 ),
 ( #20363, #13475, #22230, #5497, #7351, #24492, #18214, #2267, #4276, #14101, #15591, #15464, #24221, #25726, #3368, #8240, #23716, #17721, #5370, #2137, #12365, #23591, #21597, #6253, #20494, #26353, #24358, #13597, #3503, #5994 ),
 ( #11469, #16358, #4006, #1383, #19595, #10247, #8111, #16228, #22497, #11601, #25608, #1510, #18357, #17465, #9484, #7478, #12105, #17588, #4146, #21727, #19724, #25862, #7973, #20230, #2009, #6122, #14230, #22370, #136, #12903 ),
 ( #8375, #10375, #18486, #2530, #24887, #12633, #8509, #14887, #23027, #13037, #18757, #18889, #16626, #4926, #803, #10509, #25154, #4536, #21155, #10647, #20760, #6905, #4802, #23152, #22627, #20623, #267, #21019, #17018, #2802 ),
 ( #8777, #24757, #15022, #16497, #19024, #14496, #10913, #6377, #16890, #4402, #22886, #25022, #14621, #22758, #24622, #539, #14756, #8644, #406, #668, #16753, #8908, #12496, #6642, #4665, #12767, #20894, #2398, #6510, #2671 ),
 ( #18623, #10776, #6775, #9042, #19655, #19406, #17147, #25410, #15152, #9418, #17650, #1441, #5432, #7035, #11038, #933, #2929, #19148, #21407, #17399, #5183, #1058, #7409, #15523, #5555, #11286, #11403, #9164, #23777, #9542 ) ),
 .UNSPECIFIED., .T., .F., .F. ) 
 B_SPLINE_SURFACE_WITH_KNOTS ( ( 4, 3, 4 ),
 ( 4, 2, 2, 2, 2, 2, 2, 2, 2, 2, 2, 2, 2, 2, 4 ),
 ( 0.000000000000000000, 0.5000000000000000000, 1.000000000000000000 ),
 ( 0.000000000000000000, 0.1357259735107005372, 0.1651108541090157700, 0.1944957347073310028, 0.3598804999793158710, 0.3867117631979620773, 0.4135430264166082281, 0.5789277916885930964, 0.6062785021374117456, 0.6336292125862302838, 0.8508620842112317728, 0.8814014469398914198, 0.9119408096685510667, 0.9559704048342755334, 1.000000000000000000 ),
 .UNSPECIFIED. ) 
 GEOMETRIC_REPRESENTATION_ITEM ( )  RATIONAL_B_SPLINE_SURFACE ( (
 ( 1.000000000000000000, 1.000000000000000000, 1.000000000000000000, 1.000000000000000000, 1.000000000000000000, 1.000000000000000000, 1.000000000000000000, 1.000000000000000000, 1.000000000000000000, 1.000000000000000000, 1.000000000000000000, 1.000000000000000000, 1.000000000000000000, 1.000000000000000000, 1.000000000000000000, 1.000000000000000000, 1.000000000000000000, 1.000000000000000000, 1.000000000000000000, 1.000000000000000000, 1.000000000000000000, 1.000000000000000000, 1.000000000000000000, 1.000000000000000000, 1.000000000000000000, 1.000000000000000000, 1.000000000000000000, 1.000000000000000000, 1.000000000000000000, 1.000000000000000000),
 ( 0.3333333333333333703, 0.3333333333333333703, 0.3333333333333333703, 0.3333333333333333703, 0.3333333333333333703, 0.3333333333333333703, 0.3333333333333333703, 0.3333333333333333703, 0.3333333333333333703, 0.3333333333333333703, 0.3333333333333333703, 0.3333333333333333703, 0.3333333333333333703, 0.3333333333333333703, 0.3333333333333333703, 0.3333333333333333703, 0.3333333333333333703, 0.3333333333333333703, 0.3333333333333333703, 0.3333333333333333703, 0.3333333333333333703, 0.3333333333333333703, 0.3333333333333333703, 0.3333333333333333703, 0.3333333333333333703, 0.3333333333333333703, 0.3333333333333333703, 0.3333333333333333703, 0.3333333333333333703, 0.3333333333333333703),
 ( 0.3333333333333333703, 0.3333333333333333703, 0.3333333333333333703, 0.3333333333333333703, 0.3333333333333333703, 0.3333333333333333703, 0.3333333333333333703, 0.3333333333333333703, 0.3333333333333333703, 0.3333333333333333703, 0.3333333333333333703, 0.3333333333333333703, 0.3333333333333333703, 0.3333333333333333703, 0.3333333333333333703, 0.3333333333333333703, 0.3333333333333333703, 0.3333333333333333703, 0.3333333333333333703, 0.3333333333333333703, 0.3333333333333333703, 0.3333333333333333703, 0.3333333333333333703, 0.3333333333333333703, 0.3333333333333333703, 0.3333333333333333703, 0.3333333333333333703, 0.3333333333333333703, 0.3333333333333333703, 0.3333333333333333703),
 ( 1.000000000000000000, 1.000000000000000000, 1.000000000000000000, 1.000000000000000000, 1.000000000000000000, 1.000000000000000000, 1.000000000000000000, 1.000000000000000000, 1.000000000000000000, 1.000000000000000000, 1.000000000000000000, 1.000000000000000000, 1.000000000000000000, 1.000000000000000000, 1.000000000000000000, 1.000000000000000000, 1.000000000000000000, 1.000000000000000000, 1.000000000000000000, 1.000000000000000000, 1.000000000000000000, 1.000000000000000000, 1.000000000000000000, 1.000000000000000000, 1.000000000000000000, 1.000000000000000000, 1.000000000000000000, 1.000000000000000000, 1.000000000000000000, 1.000000000000000000),
 ( 0.3333333333333333703, 0.3333333333333333703, 0.3333333333333333703, 0.3333333333333333703, 0.3333333333333333703, 0.3333333333333333703, 0.3333333333333333703, 0.3333333333333333703, 0.3333333333333333703, 0.3333333333333333703, 0.3333333333333333703, 0.3333333333333333703, 0.3333333333333333703, 0.3333333333333333703, 0.3333333333333333703, 0.3333333333333333703, 0.3333333333333333703, 0.3333333333333333703, 0.3333333333333333703, 0.3333333333333333703, 0.3333333333333333703, 0.3333333333333333703, 0.3333333333333333703, 0.3333333333333333703, 0.3333333333333333703, 0.3333333333333333703, 0.3333333333333333703, 0.3333333333333333703, 0.3333333333333333703, 0.3333333333333333703),
 ( 0.3333333333333333703, 0.3333333333333333703, 0.3333333333333333703, 0.3333333333333333703, 0.3333333333333333703, 0.3333333333333333703, 0.3333333333333333703, 0.3333333333333333703, 0.3333333333333333703, 0.3333333333333333703, 0.3333333333333333703, 0.3333333333333333703, 0.3333333333333333703, 0.3333333333333333703, 0.3333333333333333703, 0.3333333333333333703, 0.3333333333333333703, 0.3333333333333333703, 0.3333333333333333703, 0.3333333333333333703, 0.3333333333333333703, 0.3333333333333333703, 0.3333333333333333703, 0.3333333333333333703, 0.3333333333333333703, 0.3333333333333333703, 0.3333333333333333703, 0.3333333333333333703, 0.3333333333333333703, 0.3333333333333333703),
 ( 1.000000000000000000, 1.000000000000000000, 1.000000000000000000, 1.000000000000000000, 1.000000000000000000, 1.000000000000000000, 1.000000000000000000, 1.000000000000000000, 1.000000000000000000, 1.000000000000000000, 1.000000000000000000, 1.000000000000000000, 1.000000000000000000, 1.000000000000000000, 1.000000000000000000, 1.000000000000000000, 1.000000000000000000, 1.000000000000000000, 1.000000000000000000, 1.000000000000000000, 1.000000000000000000, 1.000000000000000000, 1.000000000000000000, 1.000000000000000000, 1.000000000000000000, 1.000000000000000000, 1.000000000000000000, 1.000000000000000000, 1.000000000000000000, 1.000000000000000000) ) ) 
 REPRESENTATION_ITEM ( '' )  SURFACE ( )  );
#17743=CARTESIAN_POINT ( 'NONE',  ( -86.96347745069644475, 12.89780903124410472, -43.67073346367977393 ) ) ;
#17744=CARTESIAN_POINT ( 'NONE',  ( 91.82158438592158234, -6.516925787240506436E-14, 22.79471317813470321 ) ) ;
#17745=CARTESIAN_POINT ( 'NONE',  ( -100.7734535825088500, 12.25131212657428748, 44.31723036834913643 ) ) ;
#17746=EDGE_CURVE ( 'NONE', #19647, #16477, #23568, .T. ) ;
#17747=CARTESIAN_POINT ( 'NONE',  ( -105.3755690713226585, -21.75974354311652448, -40.00000000000002132 ) ) ;
#17748=CARTESIAN_POINT ( 'NONE',  ( 169.9999999999999716, -22.62041470344880523, -9.369682556672316309 ) ) ;
#17750=ADVANCED_FACE ( 'NONE', ( #7382 ), #12319, .T. ) ;
#17751=ADVANCED_FACE ( 'NONE', ( #5501 ), #20488, .T. ) ;
#17752=CARTESIAN_POINT ( 'NONE',  ( -86.90968602935149079, -7.324300800229181618, -20.05592747609932758 ) ) ;
#17753=CARTESIAN_POINT ( 'NONE',  ( 165.3321726438082351, -26.53500608755489054, 0.000000000000000000 ) ) ;
#17754=CARTESIAN_POINT ( 'NONE',  ( 200.0000000000000000, 14.14213562373142352, -42.42640687119268961 ) ) ;
#17755=CARTESIAN_POINT ( 'NONE',  ( -105.4741150117381778, 19.77569912954994891, -7.943527260753209696 ) ) ;
#17756=CARTESIAN_POINT ( 'NONE',  ( -105.3755690713226727, -2.472783935621397949E-13, 21.75974354311649961 ) ) ;
#17757=CARTESIAN_POINT ( 'NONE',  ( -56.48582580120558561, 6.472252184284607246, -50.09629031063960269 ) ) ;
#17758=CARTESIAN_POINT ( 'NONE',  ( -100.7734535825088358, -12.25131212657475643, -12.25131212657495539 ) ) ;
#17759=CARTESIAN_POINT ( 'NONE',  ( -198.0356074513804572, 10.87444709761036066, -67.44298959253325165 ) ) ;
#17760=CARTESIAN_POINT ( 'NONE',  ( 184.8905102610680444, -14.79361573936330565, -41.77492675556016621 ) ) ;
#17761=CARTESIAN_POINT ( 'NONE',  ( -198.0356074513804572, -10.87444709759729911, 10.87444709759714812 ) ) ;
#17762=CARTESIAN_POINT ( 'NONE',  ( -86.86493150571116928, 19.77569912839177846, -7.943527260495974573 ) ) ;
#17764=CARTESIAN_POINT ( 'NONE',  ( 57.59792236341149163, -40.00000000000014211, 37.56421063658172699 ) ) ;
#17765=CARTESIAN_POINT ( 'NONE',  ( 184.8905102610680444, 14.79361573936366092, 41.77492675556006674 ) ) ;
#17767=CARTESIAN_POINT ( 'NONE',  ( -198.0356074513804572, 15.37879056873066830, 40.00000000000002132 ) ) ;
#17769=CARTESIAN_POINT ( 'NONE',  ( 14.38125909742180220, 39.01709431150916885, -17.55144818341463164 ) ) ;
#17771=CARTESIAN_POINT ( 'NONE',  ( -16.41532015025260804, -12.95569205545558766, -42.70629200445775098 ) ) ;
#17772=CARTESIAN_POINT ( 'NONE',  ( -105.3755690713226585, -21.75974354311652448, 40.00000000000002132 ) ) ;
#17774=CARTESIAN_POINT ( 'NONE',  ( -4.039451493210497901, 23.44932283416708074, -43.00522595893983890 ) ) ;
#17776=CARTESIAN_POINT ( 'NONE',  ( -3.336279363872675319, -17.94861674415315278, 43.33179396957154950 ) ) ;
#17777=CARTESIAN_POINT ( 'NONE',  ( 20.16956056504004380, 23.97604322321460657, -43.71646652951380219 ) ) ;
#17780=B_SPLINE_CURVE_WITH_KNOTS ( 'NONE', 3,
 ( #26259, #11586, #17707, #3753, #16113, #11858 ),
 .UNSPECIFIED., .F., .F.,
 ( 4, 2, 4 ),
 ( 0.3689590070116581799, 0.3867117631979620773, 0.4044645193949217843 ),
 .UNSPECIFIED. ) ;
#17782=CARTESIAN_POINT ( 'NONE',  ( -238.4067589809705794, -4.716212492215116094E-14, 0.9644942799825824142 ) ) ;
#17784=CARTESIAN_POINT ( 'NONE',  ( -30.26275506840325136, 57.76657404653985139, -1.198031551615314161 ) ) ;
#17785=CARTESIAN_POINT ( 'NONE',  ( -135.8532207217289738, 9.153146818113548022, 40.00000000000002132 ) ) ;
#17786=CARTESIAN_POINT ( 'NONE',  ( 83.06440094993928369, -10.91839312090031378, -23.65491511364134070 ) ) ;
#17788=CARTESIAN_POINT ( 'NONE',  ( 151.7948205124836250, 33.23291073765556547, 0.000000000000000000 ) ) ;
#17789=CARTESIAN_POINT ( 'NONE',  ( 136.1360204305621266, 35.03383547441298163, -40.00000000000002132 ) ) ;
#17790=CARTESIAN_POINT ( 'NONE',  ( 146.6084372240433993, -34.62501878078303008, 0.000000000000000000 ) ) ;
#17791=CARTESIAN_POINT ( 'NONE',  ( -100.7734535825088358, 1.654174317907124744E-13, -17.32597176626811120 ) ) ;
#17793=CARTESIAN_POINT ( 'NONE',  ( -56.48582580120559982, 34.75652343174628101, -21.81201906317743067 ) ) ;
#17798=CARTESIAN_POINT ( 'NONE',  ( -196.0240758340695777, 48.96019759410240368, -14.12332442061102356 ) ) ;
#17802=CARTESIAN_POINT ( 'NONE',  ( -30.26275506840324070, -29.48230279907780016, -27.08623969584605362 ) ) ;
#17803=CARTESIAN_POINT ( 'NONE',  ( 23.30336656375561688, -42.87878279885800481, -23.35569295765272457 ) ) ;
#17805=CARTESIAN_POINT ( 'NONE',  ( -86.96347745069644475, -21.75974354311652093, -40.00000000000002132 ) ) ;
#17806=CARTESIAN_POINT ( 'NONE',  ( -89.91646883261441303, -20.29783361052119872, 8.407637968115118099 ) ) ;
#17810=CARTESIAN_POINT ( 'NONE',  ( -105.3755690713226727, 12.89780903124400879, 12.89780903124407452 ) ) ;
#17811=CARTESIAN_POINT ( 'NONE',  ( -105.4741150117390021, -7.943527260764932763, -19.77569912954469800 ) ) ;
#17812=CARTESIAN_POINT ( 'NONE',  ( 151.7948205124836250, 1.439163438361279259E-13, -33.23291073765553705 ) ) ;
#17813=CARTESIAN_POINT ( 'NONE',  ( 4.995406935893288214, 15.24977328854832770, 40.00000000000002132 ) ) ;
#17815=FACE_OUTER_BOUND ( 'NONE', #23138, .T. ) ;
#17816=CARTESIAN_POINT ( 'NONE',  ( -213.1075012329537230, -8.703598725189323045E-14, 13.71589010951911902 ) ) ;
#17817=CARTESIAN_POINT ( 'NONE',  ( -102.2610585947572872, -15.74993999358175678, 15.74993999358135710 ) ) ;
#17818=CARTESIAN_POINT ( 'NONE',  ( 146.6084372240433709, -39.99999999999993605, -5.374981219217395356 ) ) ;
#17820=CARTESIAN_POINT ( 'NONE',  ( -135.8532207217289738, -50.09629031063965243, -6.472252184284438492 ) ) ;
#17821=CARTESIAN_POINT ( 'NONE',  ( 91.82158438592158234, 17.20528682183301683, 0.000000000000000000 ) ) ;
#17822=CARTESIAN_POINT ( 'NONE',  ( -30.26275506840324070, -29.48230279907780016, -27.08623969584605362 ) ) ;
#17826=CARTESIAN_POINT ( 'NONE',  ( 146.6084372240433993, 24.48358557860307272, 24.48358557860347418 ) ) ;
#17827=CARTESIAN_POINT ( 'NONE',  ( 130.8568914410475372, 1.429239637432775288E-13, -34.05028731879788495 ) ) ;
#17828=CARTESIAN_POINT ( 'NONE',  ( 57.59792236341147031, -1.722363176415123043, 54.84617931850879557 ) ) ;
#17829=CARTESIAN_POINT ( 'NONE',  ( 151.7948205124836250, 23.49921654116328540, 23.49921654116366554 ) ) ;
#17830=CARTESIAN_POINT ( 'NONE',  ( -188.3120606736147806, -23.45204117844517810, -43.00889065703323411 ) ) ;
#17831=CARTESIAN_POINT ( 'NONE',  ( 0.2972598230769976091, -10.13633138497479180, 10.13633138497468522 ) ) ;
#17832=ORIENTED_EDGE ( 'NONE', *, *, #19523, .F. ) ;
#17833=CARTESIAN_POINT ( 'NONE',  ( -135.8532207217289738, 21.81201906317798134, -21.81201906317747685 ) ) ;
#17835=CARTESIAN_POINT ( 'NONE',  ( -56.48582580120559982, 9.153146818113574668, -40.00000000000002132 ) ) ;
#17837=CARTESIAN_POINT ( 'NONE',  ( 57.59792236341147031, -30.00663442387662627, -26.56190807104723461 ) ) ;
#17838=CARTESIAN_POINT ( 'NONE',  ( -87.13361725324189422, 0.6800178180866376376, 21.49321519332665176 ) ) ;
#17840=CARTESIAN_POINT ( 'NONE',  ( 184.8905102610680444, -1.851754852062639767E-13, 20.92133201514444352 ) ) ;
#17842=CARTESIAN_POINT ( 'NONE',  ( -4.112199523541912427, 23.43514144949416078, 42.98379141459026442 ) ) ;
#17844=VERTEX_POINT ( 'NONE', #9421 ) ;
#17845=CARTESIAN_POINT ( 'NONE',  ( 151.7948205124836534, 6.767089262349062828, -40.00000000000002132 ) ) ;
#17846=CARTESIAN_POINT ( 'NONE',  ( 163.1118516004056573, 19.27778845538780317, -19.27778845538757224 ) ) ;
#17847=CARTESIAN_POINT ( 'NONE',  ( 170.2234770963711128, 40.00000000000000000, 15.44714144992830462 ) ) ;
#17848=CARTESIAN_POINT ( 'NONE',  ( 35.93675038278705358, 12.87543821110860520, -42.26938935684505338 ) ) ;
#17851=CARTESIAN_POINT ( 'NONE',  ( 98.29820294267312875, 7.653668647304333383, -18.47759065023115355 ) ) ;
#17852=CARTESIAN_POINT ( 'NONE',  ( 98.29820294267312875, 7.653668647304333383, -18.47759065023115355 ) ) ;
#17854=CARTESIAN_POINT ( 'NONE',  ( -129.2920181229026753, 10.46331487454523845, 25.26067667728931809 ) ) ;
#17855=CARTESIAN_POINT ( 'NONE',  ( 6.615221834201326701, -24.79576599683120008, -44.82734842560605415 ) ) ;
#17856=CARTESIAN_POINT ( 'NONE',  ( 0.2972598230770100991, -38.42060263243632079, -38.42060263243699580 ) ) ;
#17857=CARTESIAN_POINT ( 'NONE',  ( 107.5473083967383445, -16.96446921415050113, 16.96446921415010678 ) ) ;
#17858=CARTESIAN_POINT ( 'NONE',  ( 184.8905102610680444, -41.77492675555986779, -14.79361573936407304 ) ) ;
#17859=CARTESIAN_POINT ( 'NONE',  ( -238.4067589809705794, -3.369206980223063916E-14, -0.9644942799825824142 ) ) ;
#17862=CARTESIAN_POINT ( 'NONE',  ( 163.1118516004056573, -12.73709011382472234, -2.449293598294708485E-15 ) ) ;
#17863=CARTESIAN_POINT ( 'NONE',  ( 146.6084372240433709, 52.76785682606519146, 3.800685668858932775 ) ) ;
#17865=CARTESIAN_POINT ( 'NONE',  ( 19.06497207195982924, -54.19242893257843008, 40.00000000000002132 ) ) ;
#17867=CARTESIAN_POINT ( 'NONE',  ( -114.4712152604451347, 20.46962080079592994, 7.710842095506693639 ) ) ;
#17868=CARTESIAN_POINT ( 'NONE',  ( 170.2234770963711128, -17.36149277826995885, 39.20704971665388427 ) ) ;
#17869=CARTESIAN_POINT ( 'NONE',  ( 200.0000000000000000, -20.00000000000006750, -40.00000000000002132 ) ) ;
#17870=ORIENTED_EDGE ( 'NONE', *, *, #14818, .F. ) ;
#17872=CARTESIAN_POINT ( 'NONE',  ( -16.41654234047147654, -12.95560590355978725, 42.70586891282371056 ) ) ;
#17873=CARTESIAN_POINT ( 'NONE',  ( 184.8905102610680444, 13.49065550809817715, -43.07788698682574591 ) ) ;
#17874=CARTESIAN_POINT ( 'NONE',  ( 14.38125909742182529, -40.00000000000021316, 55.17850393974251944 ) ) ;
#17876=CARTESIAN_POINT ( 'NONE',  ( 19.06497207195979726, 38.31983398719604139, 18.24870850772803976 ) ) ;
#17879=CARTESIAN_POINT ( 'NONE',  ( 184.8905102610680444, 19.07866798485562398, -40.00000000000002132 ) ) ;
#17883=CARTESIAN_POINT ( 'NONE',  ( -162.0762913951021176, 57.76657433523994456, -1.198031840315424867 ) ) ;
#17884=CARTESIAN_POINT ( 'NONE',  ( -100.7734535825088500, 16.03295912088740494, -40.53558337403661938 ) ) ;
#17885=CARTESIAN_POINT ( 'NONE',  ( 192.4448373802100889, 14.14213562375893574, -14.14213562375874922 ) ) ;
#17886=CARTESIAN_POINT ( 'NONE',  ( -87.12812962367802072, 14.21201470107229881, -16.13326835689685623 ) ) ;
#17887=CARTESIAN_POINT ( 'NONE',  ( 130.8568914410475088, 24.07718906446937623, -32.49135343045455215 ) ) ;
#17888=CARTESIAN_POINT ( 'NONE',  ( 136.1360204305621551, 24.77266263493153176, -31.79587985999237887 ) ) ;
#17889=CARTESIAN_POINT ( 'NONE',  ( -28.75808802591302538, 12.03522322449776638, 38.33175228464047990 ) ) ;
#17890=CARTESIAN_POINT ( 'NONE',  ( 146.6084372240433709, -52.76785682606510619, -3.800685668859292043 ) ) ;
#17891=CARTESIAN_POINT ( 'NONE',  ( 192.4448373802100889, -20.00000000003938538, 0.000000000000000000 ) ) ;
#17892=CARTESIAN_POINT ( 'NONE',  ( 160.7895100360958622, 28.48799984206444336, 0.000000000000000000 ) ) ;
#17895=CARTESIAN_POINT ( 'NONE',  ( -86.96347745069643054, -39.99999999999995737, -21.75974354311664527 ) ) ;
#17896=CARTESIAN_POINT ( 'NONE',  ( -238.4067589809705794, 27.60227080167040370, 28.96627169325338613 ) ) ;
#17899=CARTESIAN_POINT ( 'NONE',  ( -91.56559293963834989, 17.32597176626808988, 40.00000000000002132 ) ) ;
#17900=ORIENTED_EDGE ( 'NONE', *, *, #6239, .T. ) ;
#17901=CARTESIAN_POINT ( 'NONE',  ( -162.0762913951020892, 57.76657433537918251, 1.198031840455469066 ) ) ;
#17903=( BOUNDED_SURFACE ( )  B_SPLINE_SURFACE ( 3, 2, ( 
 ( #16192, #6090, #9812 ),
 ( #6218, #13926, #21924 ),
 ( #7798, #15913, #20326 ),
 ( #26332, #24182, #2103 ),
 ( #18317, #3973, #22062 ),
 ( #100, #22462, #14330 ),
 ( #20460, #4242, #12332 ),
 ( #24046, #5823, #2234 ),
 ( #20063, #14065, #1839 ),
 ( #10342, #7938, #12070 ),
 ( #16056, #20188, #10077 ),
 ( #10746, #12461, #16463 ),
 ( #14591, #25123, #12600 ),
 ( #18451, #24992, #22857 ),
 ( #13005, #4497, #4633 ),
 ( #8471, #6342, #6743 ),
 ( #2902, #18720, #12735 ),
 ( #2770, #14725, #14856 ),
 ( #16590, #8877, #6874 ),
 ( #4896, #18857, #771 ),
 ( #505, #16860, #22991 ),
 ( #20856, #2637, #8342 ),
 ( #22720, #22594, #228 ),
 ( #8611, #20730, #4371 ),
 ( #2498, #10477, #21126 ),
 ( #10608, #16721, #24585 ),
 ( #14463, #4767, #637 ),
 ( #14989, #24853, #8742 ),
 ( #18591, #16987, #6605 ),
 ( #12871, #20988, #10879 ),
 ( #18994, #23123, #20588 ),
 ( #2363, #369, #24722 ),
 ( #6478, #21253, #11010 ),
 ( #13135, #19119, #7000 ) ),
 .UNSPECIFIED., .F., .F., .F. ) 
 B_SPLINE_SURFACE_WITH_KNOTS ( ( 4, 2, 2, 2, 2, 2, 2, 2, 2, 2, 2, 2, 2, 2, 2, 2, 4 ),
 ( 3, 3 ),
 ( 0.005135431517079875642, 0.02907016617529989064, 0.05300490083351990650, 0.07693963549173991889, 0.08292331915629491679, 0.08441924007243367667, 0.08446598760106301118, 0.08448936136537768538, 0.08451273512969234569, 0.08460623018695101472, 0.08479322030146836664, 0.08516720053050305661, 0.08591516098857242267, 0.08890700282084992856, 0.09189884465312743445, 0.09489068648540494033, 0.1008743701499599382 ),
 ( 0.000000000000000000, 1.000000000000000000 ),
 .UNSPECIFIED. ) 
 GEOMETRIC_REPRESENTATION_ITEM ( )  RATIONAL_B_SPLINE_SURFACE ( (
 ( 1.000000000000000000, 0.9997813423552078804, 1.000000000000000000),
 ( 1.000000000000000000, 0.9991063894442812066, 1.000000000000000000),
 ( 1.000000000000000000, 0.9968824679670513778, 1.000000000000000000),
 ( 1.000000000000000000, 0.9891556708430853107, 1.000000000000000000),
 ( 1.000000000000000000, 0.9836552227706821805, 1.000000000000000000),
 ( 1.000000000000000000, 0.9690804699595866323, 1.000000000000000000),
 ( 1.000000000000000000, 0.9600093828092017834, 1.000000000000000000),
 ( 1.000000000000000000, 0.9461484455228768020, 1.000000000000000000),
 ( 1.000000000000000000, 0.9432496483672407894, 1.000000000000000000),
 ( 1.000000000000000000, 0.9394619383806346313, 1.000000000000000000),
 ( 1.000000000000000000, 0.9386961831920884736, 1.000000000000000000),
 ( 1.000000000000000000, 0.9378979462694522207, 1.000000000000000000),
 ( 1.000000000000000000, 0.9378737491732492826, 1.000000000000000000),
 ( 1.000000000000000000, 0.9378374413774239748, 1.000000000000000000),
 ( 1.000000000000000000, 0.9378252326299131303, 1.000000000000000000),
 ( 1.000000000000000000, 0.9378013115143170042, 1.000000000000000000),
 ( 1.000000000000000000, 0.9377893564346097000, 1.000000000000000000),
 ( 1.000000000000000000, 0.9377296084626357553, 1.000000000000000000),
 ( 1.000000000000000000, 0.9376818978498919765, 1.000000000000000000),
 ( 1.000000000000000000, 0.9375390306864408441, 1.000000000000000000),
 ( 1.000000000000000000, 0.9374441388112029205, 1.000000000000000000),
 ( 1.000000000000000000, 0.9371605328928167555, 1.000000000000000000),
 ( 1.000000000000000000, 0.9369728885717006905, 1.000000000000000000),
 ( 1.000000000000000000, 0.9364143219789186068, 1.000000000000000000),
 ( 1.000000000000000000, 0.9360477663173443208, 1.000000000000000000),
 ( 1.000000000000000000, 0.9342452504721948658, 1.000000000000000000),
 ( 1.000000000000000000, 0.9329001521055332313, 1.000000000000000000),
 ( 1.000000000000000000, 0.9304320728630449677, 1.000000000000000000),
 ( 1.000000000000000000, 0.9293115496651194185, 1.000000000000000000),
 ( 1.000000000000000000, 0.9273349178229508549, 1.000000000000000000),
 ( 1.000000000000000000, 0.9264755994062412459, 1.000000000000000000),
 ( 1.000000000000000000, 0.9243018539388534460, 1.000000000000000000),
 ( 1.000000000000000000, 0.9233922906946859799, 1.000000000000000000),
 ( 1.000000000000000000, 0.9230540990195957862, 1.000000000000000000) ) ) 
 REPRESENTATION_ITEM ( '' )  SURFACE ( )  );
#17906=CARTESIAN_POINT ( 'NONE',  ( 0.2972598230769930572, 14.33493731733933352, 0.000000000000000000 ) ) ;
#17907=ADVANCED_FACE ( 'NONE', ( #9297 ), #1605, .T. ) ;
#17908=EDGE_CURVE ( 'NONE', #16948, #151, #21094, .T. ) ;
#17910=CARTESIAN_POINT ( 'NONE',  ( -188.3120147333550563, -43.00887716025417262, 23.45203116714296598 ) ) ;
#17912=CARTESIAN_POINT ( 'NONE',  ( 6.984886629842144146, -24.81009931999644635, 44.84679502273391449 ) ) ;
#17913=CARTESIAN_POINT ( 'NONE',  ( 22.01478053667198864, 23.63228119973664931, -43.25192662397402188 ) ) ;
#17916=CARTESIAN_POINT ( 'NONE',  ( 118.9130007099546305, -25.80693111732297496, 10.68958087202318374 ) ) ;
#17918=CARTESIAN_POINT ( 'NONE',  ( -162.0762913951020892, 29.48230308784799902, -29.48230308784730980 ) ) ;
#17919=CARTESIAN_POINT ( 'NONE',  ( 184.8905102610680444, -19.07866798485554938, 40.00000000000002132 ) ) ;
#17920=CARTESIAN_POINT ( 'NONE',  ( -114.4388184736417173, 8.352332320002227917, -20.16431396440712831 ) ) ;
#17923=CARTESIAN_POINT ( 'NONE',  ( -162.0762913951020892, -41.69427287672991866, -40.00000000000002132 ) ) ;
#17924=CARTESIAN_POINT ( 'NONE',  ( 163.1118516004056573, -27.26290988616869626, 40.00000000000002132 ) ) ;
#17925=CARTESIAN_POINT ( 'NONE',  ( -86.96347745069644475, 1.775309070576523494E-13, -18.24025645688352881 ) ) ;
#17926=CARTESIAN_POINT ( 'NONE',  ( 98.29820294267359770, -8.858778887854322548, 17.94316440882988317 ) ) ;
#17927=CARTESIAN_POINT ( 'NONE',  ( 14.38125909742180752, 17.55144818341503665, -39.01709431150898411 ) ) ;
#17929=CARTESIAN_POINT ( 'NONE',  ( 98.29820294267312875, 7.653668647304333383, -18.47759065023115355 ) ) ;
#17930=CARTESIAN_POINT ( 'NONE',  ( -105.3755690713226727, -15.38646221621786481, -15.38646221621789856 ) ) ;
#17935=CARTESIAN_POINT ( 'NONE',  ( -208.1127848780264742, -38.89260858015728672, -17.67593391476669851 ) ) ;
#17936=CARTESIAN_POINT ( 'NONE',  ( 23.35928221536256899, -42.86167611819477230, -23.34300348377128742 ) ) ;
#17937=EDGE_CURVE ( 'NONE', #2955, #5450, #776, .T. ) ;
#17939=CARTESIAN_POINT ( 'NONE',  ( 170.2234770963711128, 15.44714144992819627, -40.00000000000002132 ) ) ;
#17940=CARTESIAN_POINT ( 'NONE',  ( -102.4309680865952146, -20.17061239838023923, 8.733065090080391002 ) ) ;
#17941=EDGE_LOOP ( 'NONE', ( #23175, #15135, #20377, #2286 ) ) ;
#17943=CARTESIAN_POINT ( 'NONE',  ( -105.3175672232813724, 20.76674186929500365, -5.407869933822353481 ) ) ;
#17944=CARTESIAN_POINT ( 'NONE',  ( -162.0762913951020892, 57.76657433537918251, 1.198031840455469066 ) ) ;
#17945=CARTESIAN_POINT ( 'NONE',  ( -187.3037411062139483, -42.71163782367793260, -23.25513534570746899 ) ) ;
#17946=CARTESIAN_POINT ( 'NONE',  ( 184.8905102610680444, -40.00000000000005684, 19.07866798485543569 ) ) ;
#17947=CARTESIAN_POINT ( 'NONE',  ( -259.2033419157646676, 30.48217210827734647, 40.00000000000002132 ) ) ;
#17949=FACE_OUTER_BOUND ( 'NONE', #25947, .T. ) ;
#17950=CARTESIAN_POINT ( 'NONE',  ( -100.7734535825088500, -39.99999999999995737, -22.67402823373205578 ) ) ;
#17951=CARTESIAN_POINT ( 'NONE',  ( -238.4067589809705794, -40.00000000000005684, -0.9644942799830014124 ) ) ;
#17952=CARTESIAN_POINT ( 'NONE',  ( 169.9999999999999716, -9.369682556672181306, -22.62041470344887273 ) ) ;
#17953=CARTESIAN_POINT ( 'NONE',  ( -208.1127848780264742, -10.60833733268345469, 67.17687982760682530 ) ) ;
#17954=CARTESIAN_POINT ( 'NONE',  ( -280.0000000000000568, -20.00000000000006395, -40.00000000000002132 ) ) ;
#17955=CARTESIAN_POINT ( 'NONE',  ( -280.0000000000000000, -14.14213562373108779, 14.14213562373088529 ) ) ;
#17959=CARTESIAN_POINT ( 'NONE',  ( 136.1360204305621551, -39.99999999999987921, -35.03383547441310242 ) ) ;
#17960=CARTESIAN_POINT ( 'NONE',  ( 184.8905102610680444, 41.77492675556005253, -14.79361573936377461 ) ) ;
#17961=CARTESIAN_POINT ( 'NONE',  ( 130.8568914410475372, 24.07718906447210472, 24.07718906447249907 ) ) ;
#17962=CARTESIAN_POINT ( 'NONE',  ( -188.9524938556051552, -13.86227398172975533, -47.22059665005807716 ) ) ;
#17963=CARTESIAN_POINT ( 'NONE',  ( -162.0762913951021176, -29.48230308784755493, -27.08623940707632372 ) ) ;
#17965=CARTESIAN_POINT ( 'NONE',  ( -56.48582580120559271, -6.472252184284276844, 6.472252184284108978 ) ) ;
#17966=CARTESIAN_POINT ( 'NONE',  ( 151.7948205124835681, 51.78348778862537927, 4.785054706298732086 ) ) ;
#17967=CARTESIAN_POINT ( 'NONE',  ( 57.59792236341147031, 2.435789363418171760, 0.000000000000000000 ) ) ;
#17968=CARTESIAN_POINT ( 'NONE',  ( 98.29820294272414571, 7.653668647302724892, 18.47759065022804137 ) ) ;
#17969=CARTESIAN_POINT ( 'NONE',  ( -100.7734535825088500, -16.03295912088659492, -40.53558337403696044 ) ) ;
#17971=CARTESIAN_POINT ( 'NONE',  ( -200.0000000000000000, -60.00000000000009948, 7.347880794884132555E-15 ) ) ;
#17975=CARTESIAN_POINT ( 'NONE',  ( -7.233308327734865983, 17.51119053153846394, 42.27575367454018362 ) ) ;
#17978=CARTESIAN_POINT ( 'NONE',  ( 4.995406935893288214, 15.24977328854832770, 0.000000000000000000 ) ) ;
#17980=CARTESIAN_POINT ( 'NONE',  ( -110.0574646603687512, -6.254026121474651312, -19.22569902442541334 ) ) ;
#17981=CARTESIAN_POINT ( 'NONE',  ( 7.340276910564531576, 44.87059041559415817, -24.82763627182861299 ) ) ;
#17982=CARTESIAN_POINT ( 'NONE',  ( -91.56559293963834989, -2.543181659092656077E-13, 22.67402823373191723 ) ) ;
#17984=CARTESIAN_POINT ( 'NONE',  ( -82.26522454411171736, -19.58755215917935288, -5.034236609581555832 ) ) ;
#17987=ADVANCED_FACE ( 'NONE', ( #13011 ), #14026, .T. ) ;
#17988=CARTESIAN_POINT ( 'NONE',  ( -187.8979312699049729, 42.13932507928217319, 17.45467995708709452 ) ) ;
#17989=CARTESIAN_POINT ( 'NONE',  ( 9.006212071485066417, -14.17897189022234450, -49.32687279761056942 ) ) ;
#17990=CARTESIAN_POINT ( 'NONE',  ( -208.1127848780264742, -67.17687982760682530, -10.60833733268364298 ) ) ;
#17993=CARTESIAN_POINT ( 'NONE',  ( -56.48582580120558561, -21.81201906317785699, 21.81201906317761896 ) ) ;
#17994=CARTESIAN_POINT ( 'NONE',  ( 57.59792236341147031, -1.493297263419786540E-14, 2.435789363418160658 ) ) ;
#17995=CARTESIAN_POINT ( 'NONE',  ( -280.0000000000000000, -14.14213562373118549, 14.14213562373078936 ) ) ;
#17996=CARTESIAN_POINT ( 'NONE',  ( -198.0356074513804572, 17.40982414986501325, -39.15871834505897198 ) ) ;
#17998=CARTESIAN_POINT ( 'NONE',  ( 0.2972598230770129857, -54.33493731733938148, 40.00000000000002132 ) ) ;
#18000=CARTESIAN_POINT ( 'NONE',  ( 199.9999999999999432, -19.99999999999988987, -2.449293598294708485E-15 ) ) ;
#18001=CARTESIAN_POINT ( 'NONE',  ( -105.2243945160626026, 13.27818848189948575, 16.94163139060719203 ) ) ;
#18002=CARTESIAN_POINT ( 'NONE',  ( 57.59792236341146321, 40.00000000000000711, 2.435789363418579434 ) ) ;
#18003=CARTESIAN_POINT ( 'NONE',  ( 170.2234770963711128, 10.92277846919210660, -45.64576402573182889 ) ) ;
#18004=EDGE_CURVE ( 'NONE', #25674, #10228, #15909, .T. ) ;
#18005=CARTESIAN_POINT ( 'NONE',  ( -56.48582580120559982, -9.153146818113595984, -40.00000000000002132 ) ) ;
#18008=CARTESIAN_POINT ( 'NONE',  ( 60.14720761603590660, -31.22869220290919756, 15.75494750878411665 ) ) ;
#18009=CARTESIAN_POINT ( 'NONE',  ( 127.8236149080041173, 11.91256696755823086, 28.75948073575764141 ) ) ;
#18010=CARTESIAN_POINT ( 'NONE',  ( 130.8568914410475088, 32.49135343045483637, -24.07718906446901030 ) ) ;
#18011=CARTESIAN_POINT ( 'NONE',  ( 0.2972598230770103767, -40.00000000000021316, 54.33493731733921805 ) ) ;
#18012=CARTESIAN_POINT ( 'NONE',  ( 136.1360204305621266, -24.77266263493151044, 24.77266263493093135 ) ) ;
#18013=CARTESIAN_POINT ( 'NONE',  ( 146.6084372240433993, -3.357462877844280890E-13, 34.62501878078305850 ) ) ;
#18014=CARTESIAN_POINT ( 'NONE',  ( -135.8532207217289738, -9.153146818113595984, 0.000000000000000000 ) ) ;
#18018=CARTESIAN_POINT ( 'NONE',  ( 57.59792236341147031, 54.84617931850878136, 1.722363176415705910 ) ) ;
#18019=CARTESIAN_POINT ( 'NONE',  ( 14.38125909742182529, -39.01709431150879936, -39.01709431150948859 ) ) ;
#18020=CARTESIAN_POINT ( 'NONE',  ( -110.0368417077424965, 18.74474319002781897, -7.441767003009320369 ) ) ;
#18021=CARTESIAN_POINT ( 'NONE',  ( -82.26674357280032268, 17.37244534975081933, -10.27857254523484798 ) ) ;
#18022=CARTESIAN_POINT ( 'NONE',  ( -162.0762913951021176, -29.48230308784793152, 27.08623940707591515 ) ) ;
#18023=CARTESIAN_POINT ( 'NONE',  ( 136.1360204305621266, -3.511608612530630058, -3.511608612530719764 ) ) ;
#18025=CARTESIAN_POINT ( 'NONE',  ( -259.2033419157646676, -35.01439189186523748, -21.55415060305881170 ) ) ;
#18026=CARTESIAN_POINT ( 'NONE',  ( -114.4364955367327497, -8.064892380842218600, -20.29001642038850406 ) ) ;
#18029=CARTESIAN_POINT ( 'NONE',  ( -91.56559293963834989, -40.00000000000009948, 17.32597176626796553 ) ) ;
#18030=CARTESIAN_POINT ( 'NONE',  ( 151.7948205124835681, 51.78348778862537927, 4.785054706298732086 ) ) ;
#18032=CARTESIAN_POINT ( 'NONE',  ( 5.823571940252923795, 49.16771748719391155, -14.15488761396722239 ) ) ;
#18033=CARTESIAN_POINT ( 'NONE',  ( 192.4448373802101173, -20.00000000003938538, 40.00000000000002132 ) ) ;
#18035=CARTESIAN_POINT ( 'NONE',  ( 23.37394308801977871, -23.33966569535037294, -42.85717664514612579 ) ) ;
#18036=CARTESIAN_POINT ( 'NONE',  ( -10.17115291714076619, 40.74322563957075971, 16.87639663473746410 ) ) ;
#18039=ORIENTED_EDGE ( 'NONE', *, *, #7502, .T. ) ;
#18040=CARTESIAN_POINT ( 'NONE',  ( -188.4701769959780790, -43.05504096897843880, 23.48627020870801374 ) ) ;
#18042=CARTESIAN_POINT ( 'NONE',  ( 20.91285618074430275, -13.92631245144835539, 47.65039156503490148 ) ) ;
#18043=EDGE_CURVE ( 'NONE', #22478, #12165, #12445, .T. ) ;
#18045=CARTESIAN_POINT ( 'NONE',  ( 23.36927571439206375, 23.34061495561077137, -42.85861222363617884 ) ) ;
#18048=CARTESIAN_POINT ( 'NONE',  ( 158.3379117892986585, -26.51167085133963397, 10.98149362779608396 ) ) ;
#18049=CARTESIAN_POINT ( 'NONE',  ( -109.1264249741462748, 13.72187187126471386, -33.12752917268139896 ) ) ;
#18050=CARTESIAN_POINT ( 'NONE',  ( -100.7734535825088500, 40.53558337403654832, 16.03295912088756481 ) ) ;
#18051=CARTESIAN_POINT ( 'NONE',  ( 192.4448373802101173, -19.99999999996057554, 40.00000000000002132 ) ) ;
#18054=CARTESIAN_POINT ( 'NONE',  ( -188.9524938556052689, 13.86227398173258329, -47.22059665005700424 ) ) ;
#18055=CARTESIAN_POINT ( 'NONE',  ( 14.38125909742180220, 39.01709431150892016, 17.55144818341517166 ) ) ;
#18056=CARTESIAN_POINT ( 'NONE',  ( 98.29820294267527458, 2.689882573189819553E-13, -20.00000000000500222 ) ) ;
#18057=CARTESIAN_POINT ( 'NONE',  ( -208.1127848780264742, -15.00245453012673202, -40.00000000000002132 ) ) ;
#18058=CARTESIAN_POINT ( 'NONE',  ( -238.4067589809705794, 0.9644942799825385604, 40.00000000000002132 ) ) ;
#18059=CARTESIAN_POINT ( 'NONE',  ( -238.4067589809705794, -39.99999999999963762, -40.96449428006383187 ) ) ;
#18060=CARTESIAN_POINT ( 'NONE',  ( 130.8568914410475088, -24.07718906446910623, 32.49135343045471558 ) ) ;
#18061=CARTESIAN_POINT ( 'NONE',  ( 98.29820294267423719, -14.14213562374330024, 14.14213562372619926 ) ) ;
#18062=CARTESIAN_POINT ( 'NONE',  ( 98.38705101653206953, -18.51031735812086865, -7.667224493555860221 ) ) ;
#18063=ORIENTED_EDGE ( 'NONE', *, *, #21741, .T. ) ;
#18064=CARTESIAN_POINT ( 'NONE',  ( 91.82158438592158234, -12.16597498397761967, -12.16597498397768007 ) ) ;
#18065=CARTESIAN_POINT ( 'NONE',  ( 91.82158438592158234, 17.20528682183301683, 0.000000000000000000 ) ) ;
#18070=CARTESIAN_POINT ( 'NONE',  ( -30.26275506840322294, -57.76657404653985139, 1.198031551615709844 ) ) ;
#18071=CARTESIAN_POINT ( 'NONE',  ( 22.95085416411756540, -43.12496437194769783, -17.86294511971837551 ) ) ;
#18073=CARTESIAN_POINT ( 'NONE',  ( -135.8532207217289738, 30.84685318188643777, -40.00000000000002132 ) ) ;
#18075=ORIENTED_EDGE ( 'NONE', *, *, #3001, .T. ) ;
#18078=DIRECTION ( 'NONE',  ( -0.3301743753981520868, 0.9439199552030034246, 0.000000000000000000 ) ) ;
#18079=CARTESIAN_POINT ( 'NONE',  ( -30.26275506840325136, 29.48230279907798135, -27.08623969584585112 ) ) ;
#18080=CARTESIAN_POINT ( 'NONE',  ( -188.2871287166307184, -46.98614659774644053, -13.82723289751385387 ) ) ;
#18082=CARTESIAN_POINT ( 'NONE',  ( 4.995406935893305089, -40.00000000000021316, 55.24977328853194791 ) ) ;
#18083=CARTESIAN_POINT ( 'NONE',  ( 57.59792236341147031, -2.435789363418150000, 40.00000000000002132 ) ) ;
#18087=CARTESIAN_POINT ( 'NONE',  ( -198.0356074513804572, -9.007331120208026888E-14, 15.37879056873070560 ) ) ;
#18088=CARTESIAN_POINT ( 'NONE',  ( 200.0000000000000000, -40.00000000000019185, 19.99999999999968381 ) ) ;
#18089=CARTESIAN_POINT ( 'NONE',  ( -114.4364955367315559, -8.644468109196942862, 20.04994829328090589 ) ) ;
#18090=CARTESIAN_POINT ( 'NONE',  ( 146.6084372240433709, -32.08495691632041513, -24.48358557860343154 ) ) ;
#18092=CARTESIAN_POINT ( 'NONE',  ( -56.48582580120559271, 9.153146818113576444, -0.000000000000000000 ) ) ;
#18093=EDGE_CURVE ( 'NONE', #4362, #20612, #21966, .T. ) ;
#18094=CARTESIAN_POINT ( 'NONE',  ( 151.7948205124835681, -4.785054706298153882, -51.78348778862540058 ) ) ;
#18096=CARTESIAN_POINT ( 'NONE',  ( 0.4289713102705806080, -48.32239598606154374, 14.02712011273581894 ) ) ;
#18097=CARTESIAN_POINT ( 'NONE',  ( -192.9588430854690273, 40.00000000000014211, -14.46834944099927966 ) ) ;
#18098=CARTESIAN_POINT ( 'NONE',  ( 170.2234770963711128, 1.169953928977015745E-13, -24.55285855007187124 ) ) ;
#18099=CARTESIAN_POINT ( 'NONE',  ( 4.995406935893283773, 39.06748935135195211, -17.50105314357185193 ) ) ;
#18100=CARTESIAN_POINT ( 'NONE',  ( -30.26275506840324070, -1.198031551616016266, -1.198031551616031587 ) ) ;
#18101=CARTESIAN_POINT ( 'NONE',  ( -187.7699188115114737, -23.34606611632339579, -42.84915433765043957 ) ) ;
#18103=CARTESIAN_POINT ( 'NONE',  ( 163.1118516004056573, -19.27778845539181063, -37.29075403953176959 ) ) ;
#18105=CARTESIAN_POINT ( 'NONE',  ( 4.995406935893293543, -15.24977328854832592, 0.000000000000000000 ) ) ;
#18107=CARTESIAN_POINT ( 'NONE',  ( 163.1118516004056573, -47.56205970284945295, -9.006482792074823607 ) ) ;
#18111=CARTESIAN_POINT ( 'NONE',  ( 200.0000000000000000, -59.99999999999992895, 0.000000000000000000 ) ) ;
#18112=CARTESIAN_POINT ( 'NONE',  ( -8.720657192108735245, 22.53512351407145431, 41.62108041046444384 ) ) ;
#18115=ORIENTED_EDGE ( 'NONE', *, *, #6472, .F. ) ;
#18116=CARTESIAN_POINT ( 'NONE',  ( 57.59792236341147031, -2.435789363418150444, 0.000000000000000000 ) ) ;
#18118=CARTESIAN_POINT ( 'NONE',  ( -114.7826396786541778, -1.385196341758722305, -22.13135001983572536 ) ) ;
#18119=CARTESIAN_POINT ( 'NONE',  ( -280.0000000000000000, -14.14213562373098831, -14.14213562373098654 ) ) ;
#18120=CARTESIAN_POINT ( 'NONE',  ( -93.01854144617588815, -8.553566904151914230, -20.65013722626880366 ) ) ;
#18121=CARTESIAN_POINT ( 'NONE',  ( -208.1127848780264742, 40.00000000000014211, -15.00245453012627728 ) ) ;
#18126=CARTESIAN_POINT ( 'NONE',  ( -179.7979154981486545, 40.14328926550173549, 16.62789485202968365 ) ) ;
#18127=B_SPLINE_CURVE_WITH_KNOTS ( 'NONE', 3,
 ( #15729, #23854, #5632, #7235, #13739, #21865, #3252, #13237 ),
 .UNSPECIFIED., .F., .F.,
 ( 4, 2, 2, 4 ),
 ( 0.0002291728420353419319, 0.002290361214525118462, 0.004351549587014895588, 0.008473926331994447239 ),
 .UNSPECIFIED. ) ;
#18128=CARTESIAN_POINT ( 'NONE',  ( -3.439026802539704164, -17.93765581402000109, -43.30533194338906355 ) ) ;
#18129=CARTESIAN_POINT ( 'NONE',  ( 151.7948205124836534, -33.06932595376376582, 23.49921654115996006 ) ) ;
#18130=CIRCLE ( 'NONE', #24076, 14.99999999999999822 ) ;
#18131=CARTESIAN_POINT ( 'NONE',  ( -110.0961830519565012, 2.516413774691878658, -20.07657871247701209 ) ) ;
#18132=CARTESIAN_POINT ( 'NONE',  ( -162.0762913951020892, -57.76657433524000851, 1.198031840315820329 ) ) ;
#18133=CARTESIAN_POINT ( 'NONE',  ( 0.2972598230769957217, 1.502051041545559470E-13, -14.33493731733933352 ) ) ;
#18135=CARTESIAN_POINT ( 'NONE',  ( -238.4067589809705510, -40.96449427998265946, -2.449293598294708485E-15 ) ) ;
#18136=CARTESIAN_POINT ( 'NONE',  ( 146.6084372240433993, 24.48358557860341733, -24.48358557860313311 ) ) ;
#18138=CARTESIAN_POINT ( 'NONE',  ( -86.96347745069644475, -18.24025645688354302, -2.449293598294708485E-15 ) ) ;
#18139=CARTESIAN_POINT ( 'NONE',  ( -110.0799678180788135, 10.89276344593376500, 16.99803934748214118 ) ) ;
#18140=CARTESIAN_POINT ( 'NONE',  ( -208.1127848780264742, 40.00000000000014211, -15.00245453012627728 ) ) ;
#18141=CARTESIAN_POINT ( 'NONE',  ( 136.1360204305621266, -24.77266263493116583, -24.77266263493127951 ) ) ;
#18142=CARTESIAN_POINT ( 'NONE',  ( 91.82158438592158234, -17.20528682183298486, -40.00000000000002132 ) ) ;
#18143=ORIENTED_EDGE ( 'NONE', *, *, #9630, .T. ) ;
#18145=CARTESIAN_POINT ( 'NONE',  ( -192.9588430854689989, 14.46834944099965981, 0.000000000000000000 ) ) ;
#18146=CARTESIAN_POINT ( 'NONE',  ( -30.26275506840323359, -40.00000000000017053, 41.69427246844613677 ) ) ;
#18147=CARTESIAN_POINT ( 'NONE',  ( 19.06497207195980792, 10.03556273973447155, -10.03556273973422286 ) ) ;
#18149=B_SPLINE_CURVE_WITH_KNOTS ( 'NONE', 3,
 ( #13562, #3334, #23936, #7191, #9706, #17811 ),
 .UNSPECIFIED., .F., .F.,
 ( 4, 2, 4 ),
 ( 0.000000000000000000, 0.004090195167846852331, 0.008180390335693704662 ),
 .UNSPECIFIED. ) ;
#18150=CARTESIAN_POINT ( 'NONE',  ( -126.6834156230570443, -9.107266674891850045, -24.89646324314895409 ) ) ;
#18153=B_SPLINE_CURVE_WITH_KNOTS ( 'NONE', 3,
 ( #14671, #12953, #2855, #8559, #10963, #8827, #2444, #10556, #16541, #16674, #22937, #23200, #18808, #588 ),
 .UNSPECIFIED., .F., .F.,
 ( 4, 2, 2, 2, 2, 2, 4 ),
 ( 1.040834085586084257E-17, 0.002941681445496942097, 0.004412522168245415315, 0.005883362890993887664, 0.008825044336490834099, 0.01029588505923930211, 0.01176672578198776839 ),
 .UNSPECIFIED. ) ;
#18155=CARTESIAN_POINT ( 'NONE',  ( 192.4448373802101173, 42.42640687116487896, 14.14213562375934075 ) ) ;
#18156=CARTESIAN_POINT ( 'NONE',  ( -162.0762913951020607, -57.76657433537922515, -1.198031840455874963 ) ) ;
#18158=CARTESIAN_POINT ( 'NONE',  ( -105.5018569248037323, 19.60236078713514729, 8.316028620552629036 ) ) ;
#18159=CARTESIAN_POINT ( 'NONE',  ( -162.0762913951020892, -1.202636532414034422E-14, -1.694272876828323948 ) ) ;
#18160=CARTESIAN_POINT ( 'NONE',  ( 0.2972598230770027716, -38.42060263243681817, 18.14793986248684377 ) ) ;
#18161=CARTESIAN_POINT ( 'NONE',  ( -162.0762913951020892, 1.198031840385732849, -1.198031840385733515 ) ) ;
#18162=CARTESIAN_POINT ( 'NONE',  ( 151.7948205124836534, -23.49921654115981084, -33.06932595376387951 ) ) ;
#18163=CARTESIAN_POINT ( 'NONE',  ( -86.96347745069644475, 15.38646221621793586, -15.38646221621778842 ) ) ;
#18166=CARTESIAN_POINT ( 'NONE',  ( -91.56559293963836410, 39.99999999999994316, 17.32597176626825330 ) ) ;
#18168=CARTESIAN_POINT ( 'NONE',  ( 21.80824205441142638, 43.30754100652377758, -23.67346680102637890 ) ) ;
#18169=CARTESIAN_POINT ( 'NONE',  ( -162.0762913951020892, 41.69427287692678163, -40.00000000000002132 ) ) ;
#18170=ORIENTED_EDGE ( 'NONE', *, *, #24602, .F. ) ;
#18171=CARTESIAN_POINT ( 'NONE',  ( 136.1360204305621266, -24.77266263493116583, -24.77266263493127951 ) ) ;
#18172=CARTESIAN_POINT ( 'NONE',  ( -6.342283169553549982, -42.32555349774968789, 23.00001740814397877 ) ) ;
#18173=CARTESIAN_POINT ( 'NONE',  ( -198.0356074513804572, 15.37879056873066830, 40.00000000000002132 ) ) ;
#18174=VERTEX_POINT ( 'NONE', #13545 ) ;
#18175=CARTESIAN_POINT ( 'NONE',  ( -192.1963514251026481, -48.17613439256447094, 14.00508311691324259 ) ) ;
#18177=CARTESIAN_POINT ( 'NONE',  ( -3.696864809820544995, -13.84627154338493682, 47.11278487914830038 ) ) ;
#18179=CARTESIAN_POINT ( 'NONE',  ( 22.81400246987433178, 17.87890238636472517, -43.16348862150605470 ) ) ;
#18181=CARTESIAN_POINT ( 'NONE',  ( 155.1206158682455509, -27.79897307351034286, 11.51471166709224825 ) ) ;
#18182=DIRECTION ( 'NONE',  ( 0.7071067811865476838, 0.7071067811865474617, 0.000000000000000000 ) ) ;
#18183=CARTESIAN_POINT ( 'NONE',  ( 130.8568914410475372, 4.207082182992923691, -4.207082182992794017 ) ) ;
#18184=CARTESIAN_POINT ( 'NONE',  ( -56.48582580120559271, 9.153146818113576444, -0.000000000000000000 ) ) ;
#18185=CARTESIAN_POINT ( 'NONE',  ( -192.6563370915689575, 18.27409561807029093, -44.11756948121943367 ) ) ;
#18187=CARTESIAN_POINT ( 'NONE',  ( -198.0356074513804572, -55.37879056871328487, -40.00000000000002132 ) ) ;
#18188=CARTESIAN_POINT ( 'NONE',  ( 0.2972598230769930017, 54.33493731733936016, 40.00000000000002132 ) ) ;
#18189=CARTESIAN_POINT ( 'NONE',  ( 184.8905102610680444, 40.00000000000025580, -19.07866798485515503 ) ) ;
#18190=CARTESIAN_POINT ( 'NONE',  ( -91.56559293963834989, 40.53558337403677569, -16.03295912088699993 ) ) ;
#18194=CARTESIAN_POINT ( 'NONE',  ( -192.9588430854690273, -18.05360324515454096, 38.51493924976936967 ) ) ;
#18195=CARTESIAN_POINT ( 'NONE',  ( -102.4309680866550849, -8.733065090091864491, 20.17061239836789355 ) ) ;
#18196=ORIENTED_EDGE ( 'NONE', *, *, #20013, .T. ) ;
#18198=CARTESIAN_POINT ( 'NONE',  ( 192.4448373802101173, -14.14213562370283128, -42.42640687122081999 ) ) ;
#18199=CARTESIAN_POINT ( 'NONE',  ( 22.70429368897839595, -43.19357487035075849, -17.89136451867676314 ) ) ;
#18200=ORIENTED_EDGE ( 'NONE', *, *, #17112, .F. ) ;
#18201=CARTESIAN_POINT ( 'NONE',  ( -213.1075012329537230, 13.71589010951907994, 0.000000000000000000 ) ) ;
#18202=CARTESIAN_POINT ( 'NONE',  ( -99.31364972218746345, -20.48028939129060078, 8.933506367463246889 ) ) ;
#18207=CARTESIAN_POINT ( 'NONE',  ( 57.59792236341147031, 26.56190807104693619, -30.00663442387692115 ) ) ;
#18208=CARTESIAN_POINT ( 'NONE',  ( -151.4802930571904085, -33.96623840872754130, -11.09498731354133660 ) ) ;
#18209=CARTESIAN_POINT ( 'NONE',  ( 136.1360204305621551, -39.99999999999987921, -35.03383547441310242 ) ) ;
#18210=CARTESIAN_POINT ( 'NONE',  ( -280.0000000000000568, -20.00000000000006750, 40.00000000000002132 ) ) ;
#18213=CARTESIAN_POINT ( 'NONE',  ( 0.2972598230770030492, -40.00000000000007816, 14.33493731733919496 ) ) ;
#18214=CARTESIAN_POINT ( 'NONE',  ( -192.9588430854690273, -40.00000000000024158, 54.46834944101708231 ) ) ;
#18215=CARTESIAN_POINT ( 'NONE',  ( -30.26275506840324070, -40.00000000000001421, -1.694272468446678559 ) ) ;
#18216=CARTESIAN_POINT ( 'NONE',  ( -162.0762913951020892, -3.568845385355699554E-14, 1.694272876828323948 ) ) ;
#18217=CARTESIAN_POINT ( 'NONE',  ( 192.4448373802100889, 20.00000000003945644, 0.000000000000000000 ) ) ;
#18218=CARTESIAN_POINT ( 'NONE',  ( -238.4067589809705794, -28.96627169325343942, 28.96627169325309126 ) ) ;
#18219=CARTESIAN_POINT ( 'NONE',  ( -162.0762913951021176, -1.694272876828353702, -40.00000000000002132 ) ) ;
#18220=CARTESIAN_POINT ( 'NONE',  ( -100.7734535825088500, -40.53558337403669753, -16.03295912088728770 ) ) ;
#18222=CARTESIAN_POINT ( 'NONE',  ( 23.23834162556334348, -46.85950693572758041, 13.80856396598941593 ) ) ;
#18223=CARTESIAN_POINT ( 'NONE',  ( -162.0762913951020892, -1.202636532414034422E-14, -1.694272876828323948 ) ) ;
#18224=CARTESIAN_POINT ( 'NONE',  ( -105.3755690713226727, -8.549198663894545631E-14, 18.24025645688352881 ) ) ;
#18225=CARTESIAN_POINT ( 'NONE',  ( -91.56559293963834989, 40.53558337403677569, -16.03295912088699993 ) ) ;
#18227=CARTESIAN_POINT ( 'NONE',  ( -189.6939645179852789, -18.01965094556722136, -43.50328570201967437 ) ) ;
#18228=CARTESIAN_POINT ( 'NONE',  ( -208.1127848780264742, -38.89260858015728672, -17.67593391476669851 ) ) ;
#18231=CARTESIAN_POINT ( 'NONE',  ( 130.8568914410475372, -24.07718906447255947, 24.07718906447199458 ) ) ;
#18236=CARTESIAN_POINT ( 'NONE',  ( -162.0762913951021176, -27.08623940707584055, -29.48230308784799547 ) ) ;
#18237=SHAPE_REPRESENTATION_RELATIONSHIP ( 'NONE' , 'NONE' ,  #15720, #21994 ) ;
#18238=CARTESIAN_POINT ( 'NONE',  ( -77.61595200903278169, 3.459815247513496228, 21.80829238165218698 ) ) ;
#18242=CARTESIAN_POINT ( 'NONE',  ( -1.087763065929284290, 24.03018639663618927, 43.78960619332443116 ) ) ;
#18243=EDGE_CURVE ( 'NONE', #1858, #2889, #12113, .T. ) ;
#18251=CARTESIAN_POINT ( 'NONE',  ( -91.56559293963834989, -16.03295912088706388, -16.03295912088710651 ) ) ;
#18252=CARTESIAN_POINT ( 'NONE',  ( -97.73860346107333896, -8.987542150753291992, -20.56359266933904451 ) ) ;
#18253=CIRCLE ( 'NONE', #21652, 15.00000000000000178 ) ;
#18254=CARTESIAN_POINT ( 'NONE',  ( 14.38125909742180220, 40.00000000000017764, -15.17850393972591760 ) ) ;
#18256=CARTESIAN_POINT ( 'NONE',  ( -188.2995950289364089, 46.99046209955525200, -13.82811170417133617 ) ) ;
#18257=CARTESIAN_POINT ( 'NONE',  ( -105.4741150117389168, 7.943527260764259523, 19.77569912954497866 ) ) ;
#18259=CARTESIAN_POINT ( 'NONE',  ( -199.0572111222995488, 43.66164585888754601, 18.08524587028139052 ) ) ;
#18260=CARTESIAN_POINT ( 'NONE',  ( 11.38508063392463043, -14.17561098846331191, -49.30460303390994170 ) ) ;
#18261=CARTESIAN_POINT ( 'NONE',  ( -192.9588430854689705, -38.51493924976909966, -38.51493924976973915 ) ) ;
#18262=CARTESIAN_POINT ( 'NONE',  ( -96.93773665438781961, 20.58457565566406799, -9.001171854902132452 ) ) ;
#18263=CARTESIAN_POINT ( 'NONE',  ( 130.8568914410475088, -32.49135343045460900, -24.07718906446924478 ) ) ;
#18266=CARTESIAN_POINT ( 'NONE',  ( 184.8905102610680444, -19.07866798485555293, -2.449293598294708485E-15 ) ) ;
#18268=CARTESIAN_POINT ( 'NONE',  ( -238.4067589809705510, -40.96449427998265946, -2.449293598294708485E-15 ) ) ;
#18270=CARTESIAN_POINT ( 'NONE',  ( -238.4067589809705794, 40.00000000000040501, -40.96449427990138759 ) ) ;
#18271=CARTESIAN_POINT ( 'NONE',  ( -91.56559293963834989, -16.03295912088706388, -16.03295912088710651 ) ) ;
#18272=CARTESIAN_POINT ( 'NONE',  ( 146.6084372240433993, -34.62501878078303008, 0.000000000000000000 ) ) ;
#18275=ORIENTED_EDGE ( 'NONE', *, *, #17291, .T. ) ;
#18277=CARTESIAN_POINT ( 'NONE',  ( 91.82158438592158234, -17.20528682183298486, 40.00000000000002132 ) ) ;
#18278=CARTESIAN_POINT ( 'NONE',  ( -89.92902785008678279, -8.088236460649998349, -20.44110050034134929 ) ) ;
#18279=CARTESIAN_POINT ( 'NONE',  ( -192.9588430854689989, -2.280704836619014309E-13, 54.46834944099972375 ) ) ;
#18280=CARTESIAN_POINT ( 'NONE',  ( 163.1118516004056573, 37.29075403953132906, 19.27778845539275565 ) ) ;
#18281=CARTESIAN_POINT ( 'NONE',  ( -105.3755690713226727, -21.75974354311652093, 0.000000000000000000 ) ) ;
#18286=CARTESIAN_POINT ( 'NONE',  ( 151.7948205124836534, 33.06932595376333239, 23.49921654116065284 ) ) ;
#18287=CARTESIAN_POINT ( 'NONE',  ( -105.3755690713226585, -12.89780903124444578, 43.67073346367968156 ) ) ;
#18289=CARTESIAN_POINT ( 'NONE',  ( -87.11138134861613480, 17.02212146152260885, -13.16760794720424776 ) ) ;
#18290=CARTESIAN_POINT ( 'NONE',  ( -135.8532207217289738, -21.81201906317806305, 34.75652343174590442 ) ) ;
#18291=CARTESIAN_POINT ( 'NONE',  ( -86.95488169845621940, 9.644899311048764190, -19.11867441905801357 ) ) ;
#18292=CARTESIAN_POINT ( 'NONE',  ( -259.2033419157646676, -35.01439189186554302, 21.55415060305832498 ) ) ;
#18293=CARTESIAN_POINT ( 'NONE',  ( -213.1075012329537230, -37.98287015391232302, -18.58567234101164800 ) ) ;
#18296=CARTESIAN_POINT ( 'NONE',  ( 4.995406935893298872, -1.944352046434030652E-13, 55.24977328854835434 ) ) ;
#18298=CARTESIAN_POINT ( 'NONE',  ( 23.37583784646131235, 42.85659535397685005, -23.33923448557672131 ) ) ;
#18299=CARTESIAN_POINT ( 'NONE',  ( -100.7734535825088500, 17.32597176626809699, -40.00000000000002132 ) ) ;
#18301=CARTESIAN_POINT ( 'NONE',  ( -135.8532207217289738, -9.153146818113595984, 0.000000000000000000 ) ) ;
#18302=CARTESIAN_POINT ( 'NONE',  ( -4.915070467873723814, -42.74707758271747338, 23.27857837409242947 ) ) ;
#18304=CARTESIAN_POINT ( 'NONE',  ( -198.0356074513804572, 55.37879056873070027, 2.449293598294708485E-15 ) ) ;
#18306=CARTESIAN_POINT ( 'NONE',  ( -1.255560987024282094, 23.98612781107801695, -43.73013506549182949 ) ) ;
#18307=CIRCLE ( 'NONE', #24273, 14.99999999999999645 ) ;
#18312=CARTESIAN_POINT ( 'NONE',  ( -3.786831587087432727, -23.50387725152155838, 43.07879808621821383 ) ) ;
#18313=CARTESIAN_POINT ( 'NONE',  ( -3.443169733045677194, 17.93724492941721493, -43.30433998020576780 ) ) ;
#18315=CARTESIAN_POINT ( 'NONE',  ( 57.59792236341147031, -1.493297263419786540E-14, 2.435789363418160658 ) ) ;
#18316=CARTESIAN_POINT ( 'NONE',  ( 155.4809970915717372, -27.66446758342042500, 11.45899766888341986 ) ) ;
#18317=CARTESIAN_POINT ( 'NONE',  ( -151.4802930564399901, -16.17241674337392254, 31.86309827659608018 ) ) ;
#18318=CARTESIAN_POINT ( 'NONE',  ( 57.59792236341147031, 26.56190807104720975, -26.56190807104655249 ) ) ;
#18319=CARTESIAN_POINT ( 'NONE',  ( -105.2054292635175017, 14.23158570600623385, -16.16441072139837232 ) ) ;
#18320=AXIS2_PLACEMENT_3D ( 'NONE', #11032, #14614, #13029 ) ;
#18321=CARTESIAN_POINT ( 'NONE',  ( -188.6013942376037278, 13.84412886956844169, -47.09843442133356461 ) ) ;
#18322=CARTESIAN_POINT ( 'NONE',  ( -208.1127848780264742, 38.89260858015707356, 17.67593391476696141 ) ) ;
#18323=CARTESIAN_POINT ( 'NONE',  ( -208.1127848780264742, 67.17687982763172272, -10.60833733270698254 ) ) ;
#18324=EDGE_CURVE ( 'NONE', #1209, #25810, #530, .T. ) ;
#18325=CARTESIAN_POINT ( 'NONE',  ( -208.1127848780264742, -55.00245453010926866, 40.00000000000002132 ) ) ;
#18326=CARTESIAN_POINT ( 'NONE',  ( -213.1075012329537230, 53.71589010950162191, -40.00000000000002132 ) ) ;
#18327=CARTESIAN_POINT ( 'NONE',  ( -86.96347745069644475, -2.438961472018186339E-13, 21.75974354311649961 ) ) ;
#18328=CARTESIAN_POINT ( 'NONE',  ( 57.59792236341147031, -1.722363176415123043, 54.84617931850879557 ) ) ;
#18329=CARTESIAN_POINT ( 'NONE',  ( -105.4741150117379647, 19.77569912955136999, -7.943527260750081531 ) ) ;
#18330=CARTESIAN_POINT ( 'NONE',  ( 192.4448373802100889, -14.14213562370293431, -14.14213562370322030 ) ) ;
#18333=CARTESIAN_POINT ( 'NONE',  ( 130.8568914410475372, -24.07718906447222551, -24.07718906447233209 ) ) ;
#18334=B_SPLINE_CURVE_WITH_KNOTS ( 'NONE', 3,
 ( #21884, #25891, #7508, #12037, #24148, #17615 ),
 .UNSPECIFIED., .F., .F.,
 ( 4, 2, 4 ),
 ( -6.000000003830536561E-08, 0.03937727993095203882, 0.07875461986190411545 ),
 .UNSPECIFIED. ) ;
#18335=CARTESIAN_POINT ( 'NONE',  ( -99.31364972220134746, 8.933506367370242174, 20.48028939132513315 ) ) ;
#18338=CARTESIAN_POINT ( 'NONE',  ( -105.3755690713226585, -12.89780903124383471, -43.67073346367985920 ) ) ;
#18339=CARTESIAN_POINT ( 'NONE',  ( 22.01478053669594814, -43.25192662396801069, -23.63228119971946839 ) ) ;
#18342=CARTESIAN_POINT ( 'NONE',  ( 23.37394308801978582, -46.80823611210187352, -13.80096434448294396 ) ) ;
#18343=CARTESIAN_POINT ( 'NONE',  ( -105.3844866140388206, -9.640326247891781719, -19.12039797534664132 ) ) ;
#18344=EDGE_CURVE ( 'NONE', #20782, #16811, #24470, .T. ) ;
#18349=CARTESIAN_POINT ( 'NONE',  ( -56.48582580120559982, 21.81201906317778594, -34.75652343174606074 ) ) ;
#18350=CARTESIAN_POINT ( 'NONE',  ( -189.0115661350367873, -43.33404204260303061, -17.94954792649186004 ) ) ;
#18351=CARTESIAN_POINT ( 'NONE',  ( -213.1075012329537230, -40.00000000000011369, 13.71589010951897691 ) ) ;
#18352=CARTESIAN_POINT ( 'NONE',  ( -105.3755690713226727, -21.75974354311652093, 0.000000000000000000 ) ) ;
#18356=CARTESIAN_POINT ( 'NONE',  ( 151.7948205124836534, -39.99999999999987921, -33.23291073765567916 ) ) ;
#18357=CARTESIAN_POINT ( 'NONE',  ( -86.96347745069644475, -8.210974027862429531E-14, 18.24025645688352881 ) ) ;
#18358=CARTESIAN_POINT ( 'NONE',  ( -86.96347745069644475, 5.999880687339585546E-14, -21.75974354311649961 ) ) ;
#18359=CARTESIAN_POINT ( 'NONE',  ( -56.48582580120559982, 9.153146818113574668, -40.00000000000002132 ) ) ;
#18360=CARTESIAN_POINT ( 'NONE',  ( 192.4448373802101173, -42.42640687116490028, -14.14213562375904942 ) ) ;
#18361=CARTESIAN_POINT ( 'NONE',  ( 0.2972598230769983307, -14.33493731733933352, 0.000000000000000000 ) ) ;
#18362=CARTESIAN_POINT ( 'NONE',  ( 57.59792236341148453, -26.56190807104700369, 26.56190807104673723 ) ) ;
#18364=CARTESIAN_POINT ( 'NONE',  ( 20.59573805978979522, -47.74081960064684438, 13.93986955483953594 ) ) ;
#18365=CARTESIAN_POINT ( 'NONE',  ( -86.96347745069645896, 40.00000000000019895, -18.24025645688310249 ) ) ;
#18366=CARTESIAN_POINT ( 'NONE',  ( 136.1360204305621551, -40.00000000000001421, 4.966164525586921563 ) ) ;
#18367=CARTESIAN_POINT ( 'NONE',  ( 192.4448373802101173, 42.42640687116508502, -14.14213562375874567 ) ) ;
#18369=CARTESIAN_POINT ( 'NONE',  ( 57.59792236341147031, 1.722363176415040886, 1.722363176415060426 ) ) ;
#18370=CARTESIAN_POINT ( 'NONE',  ( -188.3611024622301215, -23.46270902204919651, -43.02327292323010255 ) ) ;
#18371=CARTESIAN_POINT ( 'NONE',  ( 163.1118516004056573, -37.29075403953139300, -19.27778845539249630 ) ) ;
#18373=CARTESIAN_POINT ( 'NONE',  ( 0.2972598230769990524, -18.14793986248671231, -38.42060263243687501 ) ) ;
#18375=CARTESIAN_POINT ( 'NONE',  ( -86.96347745069645896, 21.75974354311648895, -40.00000000000002132 ) ) ;
#18377=CARTESIAN_POINT ( 'NONE',  ( 130.8568914410475372, -24.07718906447255947, 24.07718906447199458 ) ) ;
#18382=CARTESIAN_POINT ( 'NONE',  ( -4.439300432588719758, 13.79990882516848849, 46.85201324744569717 ) ) ;
#18383=ORIENTED_EDGE ( 'NONE', *, *, #5649, .F. ) ;
#18388=B_SPLINE_CURVE_WITH_KNOTS ( 'NONE', 3,
 ( #5728, #9723, #21700, #3220, #1230, #1360, #3346, #9459, #17320, #25454, #7205, #15694, #1483, #9588, #7712, #11446 ),
 .UNSPECIFIED., .F., .F.,
 ( 4, 2, 2, 2, 2, 2, 2, 4 ),
 ( 0.0003146141176167394885, 0.002410294611447383068, 0.003458134858362704993, 0.004505975105278026485, 0.008697336092939303778, 0.01079301658676993375, 0.01288869708060056719, 0.01708005806826183581 ),
 .UNSPECIFIED. ) ;
#18389=EDGE_CURVE ( 'NONE', #6531, #15177, #7022, .T. ) ;
#18390=CARTESIAN_POINT ( 'NONE',  ( -2.937533998755706310, 43.32931883109341697, -23.68967259528445979 ) ) ;
#18391=CARTESIAN_POINT ( 'NONE',  ( -192.9588430854690273, 40.00000000000055422, -54.46834944101679810 ) ) ;
#18396=CARTESIAN_POINT ( 'NONE',  ( -188.3120147333545731, 23.45203116714302638, 43.00887716025393814 ) ) ;
#18397=CARTESIAN_POINT ( 'NONE',  ( -3.494657986427937679, -17.93150516116801185, -43.29048295385624101 ) ) ;
#18398=CARTESIAN_POINT ( 'NONE',  ( 57.59792236341148453, -54.84617931850879557, 1.722363176414566155 ) ) ;
#18399=CARTESIAN_POINT ( 'NONE',  ( -89.92902785008676858, 20.17328762787298402, -8.734793929541176283 ) ) ;
#18400=CARTESIAN_POINT ( 'NONE',  ( 200.0000000000000000, -42.42640687119269671, -14.14213562373124766 ) ) ;
#18401=CARTESIAN_POINT ( 'NONE',  ( -77.62168048241881024, 21.77704146685383790, 3.672512281558228509 ) ) ;
#18402=CARTESIAN_POINT ( 'NONE',  ( -259.2033419157646676, 6.730120644403426944, 6.730120644403592145 ) ) ;
#18403=CARTESIAN_POINT ( 'NONE',  ( 91.82158438592159655, -22.79471317813468900, 40.00000000000002132 ) ) ;
#18404=ADVANCED_FACE ( 'NONE', ( #15414 ), #11528, .T. ) ;
#18406=CARTESIAN_POINT ( 'NONE',  ( -198.0356074513804572, -55.37879056874826489, 40.00000000000002132 ) ) ;
#18407=CARTESIAN_POINT ( 'NONE',  ( -110.0927810291447599, 16.11098205474433342, 12.17528477497603667 ) ) ;
#18408=CARTESIAN_POINT ( 'NONE',  ( -135.8532207217289738, 40.00000000000031974, -30.84685318188603986 ) ) ;
#18409=CARTESIAN_POINT ( 'NONE',  ( -86.96347745069644475, 12.89780903124410472, -43.67073346367977393 ) ) ;
#18410=CARTESIAN_POINT ( 'NONE',  ( 19.06497207195980792, 14.19242893257840876, 0.000000000000000000 ) ) ;
#18414=CARTESIAN_POINT ( 'NONE',  ( 4.995406935893288214, 15.24977328854832770, 40.00000000000002132 ) ) ;
#18415=CARTESIAN_POINT ( 'NONE',  ( 156.5537079553357103, 11.28159757857181766, 27.23618587942438651 ) ) ;
#18416=CARTESIAN_POINT ( 'NONE',  ( -213.1075012329537230, 66.26714140138673770, -9.698598906462034819 ) ) ;
#18417=CARTESIAN_POINT ( 'NONE',  ( -110.1018001840315748, -20.19553435163851418, 0.6219992248507131283 ) ) ;
#18423=CARTESIAN_POINT ( 'NONE',  ( -86.96347745069644475, 41.18208027870576871, 15.38646221621837107 ) ) ;
#18424=CARTESIAN_POINT ( 'NONE',  ( 57.59792236341148453, -26.56190807104663421, -26.56190807104710672 ) ) ;
#18427=CARTESIAN_POINT ( 'NONE',  ( -30.26275506840325136, 40.00000000000003553, -1.694272468445841007 ) ) ;
#18428=CARTESIAN_POINT ( 'NONE',  ( -100.7734535825088500, -12.25131212657524316, 44.31723036834888774 ) ) ;
#18429=CARTESIAN_POINT ( 'NONE',  ( 146.6084372240433993, -24.48358557860353457, 24.48358557860296258 ) ) ;
#18430=CARTESIAN_POINT ( 'NONE',  ( -238.4067589809705794, -27.60227080167069147, 28.96627169325319429 ) ) ;
#18431=ADVANCED_FACE ( 'NONE', ( #8087 ), #5876, .T. ) ;
#18432=CARTESIAN_POINT ( 'NONE',  ( 151.7948205124836250, 23.49921654116361225, -23.49921654116333514 ) ) ;
#18436=CARTESIAN_POINT ( 'NONE',  ( -198.0356074513804572, 39.99999999999979394, 55.37879056874835726 ) ) ;
#18438=CARTESIAN_POINT ( 'NONE',  ( 20.69615274310878306, 47.71500688527101630, -13.93598092275249911 ) ) ;
#18439=CARTESIAN_POINT ( 'NONE',  ( -162.0762913951021176, 1.694272876828294194, -40.00000000000002132 ) ) ;
#18440=CARTESIAN_POINT ( 'NONE',  ( 91.82158438592158234, -12.16597498397761967, -12.16597498397768007 ) ) ;
#18441=CARTESIAN_POINT ( 'NONE',  ( -4.037857402784076122, -43.00569567200361121, 23.44963359339816122 ) ) ;
#18442=CARTESIAN_POINT ( 'NONE',  ( -86.96347745069644475, 18.24025645688350750, 40.00000000000002132 ) ) ;
#18444=CARTESIAN_POINT ( 'NONE',  ( -1.815588850254805431, 23.89016120430211387, -43.60036197523977108 ) ) ;
#18445=CARTESIAN_POINT ( 'NONE',  ( 136.1360204305621266, -24.77266263493116583, -24.77266263493127951 ) ) ;
#18446=CARTESIAN_POINT ( 'NONE',  ( -39.81953879987010936, -11.17638696923166286, 34.34246706546223038 ) ) ;
#18447=CARTESIAN_POINT ( 'NONE',  ( -3.966425590328896078, 13.83202835294368782, -47.01685867532415131 ) ) ;
#18449=CARTESIAN_POINT ( 'NONE',  ( -208.1127848780265026, 1.189126717069624012E-13, -15.00245453012669472 ) ) ;
#18451=CARTESIAN_POINT ( 'NONE',  ( -188.2871287166134096, -23.44689273421206721, 43.00155302796424905 ) ) ;
#18452=( BOUNDED_CURVE ( )  B_SPLINE_CURVE ( 3, ( #2113, #16335, #14207, #6230 ),
 .UNSPECIFIED., .F., .F. ) 
 B_SPLINE_CURVE_WITH_KNOTS ( ( 4, 4 ),
 ( 0.01576650722537254259, 0.02368120503278678748 ),
 .UNSPECIFIED. ) 
 CURVE ( )  GEOMETRIC_REPRESENTATION_ITEM ( )  RATIONAL_B_SPLINE_CURVE ( ( 0.7232313460858560417, 0.6666666666666658525, 0.6208516971803444973, 0.5857864376268920870 ) ) 
 REPRESENTATION_ITEM ( '' )  );
#18453=CARTESIAN_POINT ( 'NONE',  ( -208.1127848780264742, -17.67593391476605547, -38.89260858015755673 ) ) ;
#18454=CARTESIAN_POINT ( 'NONE',  ( 151.7948205124835681, 33.23291073765556547, 40.00000000000002132 ) ) ;
#18455=CARTESIAN_POINT ( 'NONE',  ( -188.3066136396993784, 13.82848859481245540, -46.99300418776407895 ) ) ;
#18456=CARTESIAN_POINT ( 'NONE',  ( -238.4067589809705794, 0.6820004457912851592, -0.6820004457913123597 ) ) ;
#18457=CARTESIAN_POINT ( 'NONE',  ( -198.0356074513804572, 67.44298959250878056, -10.87444709758402261 ) ) ;
#18458=CARTESIAN_POINT ( 'NONE',  ( -162.0762913951020607, -41.69427287682838568, -2.449293598294708485E-15 ) ) ;
#18459=CARTESIAN_POINT ( 'NONE',  ( 57.59792236341147031, 37.56421063658187620, 2.449293598294708485E-15 ) ) ;
#18460=CARTESIAN_POINT ( 'NONE',  ( -30.26275506840324070, 1.218738420030236455E-14, -1.694272468446259783 ) ) ;
#18461=CARTESIAN_POINT ( 'NONE',  ( 151.7948205124836250, 4.785054706301690608, 4.785054706301682614 ) ) ;
#18462=CARTESIAN_POINT ( 'NONE',  ( -97.73860346102681262, 20.56359266934609664, -8.987542150742756419 ) ) ;
#18464=CARTESIAN_POINT ( 'NONE',  ( -213.1075012329537230, -9.698598906462304825, -66.26714140138675191 ) ) ;
#18465=CARTESIAN_POINT ( 'NONE',  ( 57.59792236341147031, 30.00663442387683588, 26.56190807104703211 ) ) ;
#18467=CARTESIAN_POINT ( 'NONE',  ( -198.0356074513804572, 10.87444709759714989, 10.87444709759722450 ) ) ;
#18468=CARTESIAN_POINT ( 'NONE',  ( -97.73860346102743790, 8.987542150760905457, 20.56359266933915464 ) ) ;
#18469=CARTESIAN_POINT ( 'NONE',  ( 0.2972598230770048811, -10.13633138497510089, 66.70487387989852834 ) ) ;
#18470=CARTESIAN_POINT ( 'NONE',  ( -3.921555385250247827, -47.03297225793160408, -13.83441994316416590 ) ) ;
#18471=ORIENTED_EDGE ( 'NONE', *, *, #24791, .T. ) ;
#18478=CARTESIAN_POINT ( 'NONE',  ( -280.0000000000000000, -14.14213562373098831, -14.14213562373098654 ) ) ;
#18479=CARTESIAN_POINT ( 'NONE',  ( -166.7090905285257918, -37.06261835962623508, -15.35183918168495332 ) ) ;
#18480=CARTESIAN_POINT ( 'NONE',  ( 192.4448373802101173, -40.00000000000005684, 19.99999999996046185 ) ) ;
#18481=CARTESIAN_POINT ( 'NONE',  ( 14.38125909742180752, 55.17850393974265444, 40.00000000000002132 ) ) ;
#18484=CIRCLE ( 'NONE', #26158, 14.99999999999999822 ) ;
#18485=CARTESIAN_POINT ( 'NONE',  ( -198.0356074513804572, -40.00000000000025580, 55.37879056871310013 ) ) ;
#18486=CARTESIAN_POINT ( 'NONE',  ( -238.4067589809705794, 39.99999999999983658, 40.96449428006354765 ) ) ;
#18487=CARTESIAN_POINT ( 'NONE',  ( 57.59792236341146321, 40.00000000000004263, -2.435789363418021214 ) ) ;
#18488=CARTESIAN_POINT ( 'NONE',  ( 130.8568914410475372, 34.05028731879791337, 0.000000000000000000 ) ) ;
#18489=CARTESIAN_POINT ( 'NONE',  ( 4.995406935893307754, -55.24977328854835434, -2.449293598294708485E-15 ) ) ;
#18490=CARTESIAN_POINT ( 'NONE',  ( -259.2033419157646676, 6.730120644403214669, 49.83842185052034068 ) ) ;
#18491=CARTESIAN_POINT ( 'NONE',  ( 164.1122551457363841, -10.10009781492422576, -24.38379312608499205 ) ) ;
#18494=CARTESIAN_POINT ( 'NONE',  ( 130.8568914410475372, 8.880724697947696879E-14, -5.949712681206690945 ) ) ;
#18495=CARTESIAN_POINT ( 'NONE',  ( 170.2234770963711128, -2.511315425431857630E-14, 15.44714144992816074 ) ) ;
#18496=CARTESIAN_POINT ( 'NONE',  ( -280.0000000000000568, 14.14213562373097943, -42.42640687119285303 ) ) ;
#18499=CARTESIAN_POINT ( 'NONE',  ( 184.8905102610680444, -41.77492675555986779, -14.79361573936407304 ) ) ;
#18501=CARTESIAN_POINT ( 'NONE',  ( 170.2234770963711128, -45.64576402573167258, -10.92277846919254891 ) ) ;
#18503=CARTESIAN_POINT ( 'NONE',  ( -100.7734535825088500, -17.32597176626812185, -40.00000000000002132 ) ) ;
#18504=CARTESIAN_POINT ( 'NONE',  ( -114.4364955367335881, -20.04994829326802019, 8.644468109231409514 ) ) ;
#18505=CARTESIAN_POINT ( 'NONE',  ( -280.0000000000000000, -20.00000000000006750, 0.000000000000000000 ) ) ;
#18509=ORIENTED_EDGE ( 'NONE', *, *, #12049, .T. ) ;
#18512=FACE_OUTER_BOUND ( 'NONE', #4488, .T. ) ;
#18513=CARTESIAN_POINT ( 'NONE',  ( 22.90311673804424331, 13.82691048574062087, 46.98314248933976245 ) ) ;
#18514=ORIENTED_EDGE ( 'NONE', *, *, #7837, .F. ) ;
#18516=CARTESIAN_POINT ( 'NONE',  ( -135.8532207217289738, -6.472252184284190690, -6.472252184284188914 ) ) ;
#18518=CARTESIAN_POINT ( 'NONE',  ( -105.3174652557048603, -5.408042926937029371, -20.76738663211824942 ) ) ;
#18519=AXIS2_PLACEMENT_3D ( 'NONE', #2463, #69, #10179 ) ;
#18520=CARTESIAN_POINT ( 'NONE',  ( 23.37394308801976450, 46.80823611210215063, -13.80096434448263309 ) ) ;
#18522=CARTESIAN_POINT ( 'NONE',  ( 151.7948205124836534, 33.06932595376365924, -23.49921654116018743 ) ) ;
#18524=CARTESIAN_POINT ( 'NONE',  ( -100.0968563617722822, -8.893120081573353986, -20.41799937588055158 ) ) ;
#18525=CARTESIAN_POINT ( 'NONE',  ( 192.4448373802101173, 39.99999999999985079, 20.00000000003984013 ) ) ;
#18526=CARTESIAN_POINT ( 'NONE',  ( -105.3755690713226585, 39.99999999999977263, 21.75974354311691883 ) ) ;
#18531=CARTESIAN_POINT ( 'NONE',  ( -192.1963514250885225, 14.00508311691534047, 48.17613439255790553 ) ) ;
#18532=CARTESIAN_POINT ( 'NONE',  ( 146.6084372240433709, -3.800685668859084210, 52.76785682606516303 ) ) ;
#18533=CARTESIAN_POINT ( 'NONE',  ( -199.9999999999998863, 23.83166235904700514, 44.86667451853053734 ) ) ;
#18534=CARTESIAN_POINT ( 'NONE',  ( 14.38125909742180752, 17.55144818341448953, 39.01709431150923280 ) ) ;
#18536=CARTESIAN_POINT ( 'NONE',  ( 4.995406935893287326, 17.50105314357225694, -39.06748935135176026 ) ) ;
#18538=CARTESIAN_POINT ( 'NONE',  ( -30.26275506840324425, -1.694272468446265334, 40.00000000000002132 ) ) ;
#18540=CARTESIAN_POINT ( 'NONE',  ( 136.1360204305621266, 24.77266263493138965, -24.77266263493110188 ) ) ;
#18541=CARTESIAN_POINT ( 'NONE',  ( 19.06497207195980792, -14.19242893257839988, 40.00000000000002132 ) ) ;
#18542=CARTESIAN_POINT ( 'NONE',  ( -114.7719828131935600, 16.76092671198274076, 14.45533796058303899 ) ) ;
#18543=CARTESIAN_POINT ( 'NONE',  ( -100.7734535825088500, 39.99999999999976552, 22.67402823373233645 ) ) ;
#18544=CARTESIAN_POINT ( 'NONE',  ( 14.38125909742180752, 10.73282306404720465, 10.73282306404724018 ) ) ;
#18547=VERTEX_POINT ( 'NONE', #10331 ) ;
#18549=CARTESIAN_POINT ( 'NONE',  ( -30.26275506840324425, 1.694272468446254232, 40.00000000000002132 ) ) ;
#18551=CARTESIAN_POINT ( 'NONE',  ( 144.9504669809064978, 12.48392651407807108, 30.13886470195712164 ) ) ;
#18552=CARTESIAN_POINT ( 'NONE',  ( -192.9588430854689989, 38.51493924976983152, -38.51493924976893624 ) ) ;
#18556=CARTESIAN_POINT ( 'NONE',  ( 192.4448373802100889, -20.00000000003938538, 0.000000000000000000 ) ) ;
#18557=CARTESIAN_POINT ( 'NONE',  ( -87.10563802237732034, 2.725721811608155853, -21.31096006044499802 ) ) ;
#18560=CARTESIAN_POINT ( 'NONE',  ( -238.4067589809705794, 0.6820004458491113475, -57.25054294077229144 ) ) ;
#18561=CARTESIAN_POINT ( 'NONE',  ( -86.96347745069643054, -41.18208027870611687, 15.38646221621750954 ) ) ;
#18563=CARTESIAN_POINT ( 'NONE',  ( -135.8532207217289738, 39.99999999999990763, 9.153146818113990335 ) ) ;
#18564=CARTESIAN_POINT ( 'NONE',  ( 57.59792236341148453, -54.84617931850879557, 1.722363176414566155 ) ) ;
#18565=CARTESIAN_POINT ( 'NONE',  ( 4.995406935893293543, -15.24977328854832592, 0.000000000000000000 ) ) ;
#18566=CARTESIAN_POINT ( 'NONE',  ( -135.8532207217289738, -6.472252184284190690, -6.472252184284188914 ) ) ;
#18567=CARTESIAN_POINT ( 'NONE',  ( 200.0000000000000000, -14.14213562373062949, -42.42640687119301646 ) ) ;
#18568=DIRECTION ( 'NONE',  ( 0.000000000000000000, 1.000000000000000000, 0.000000000000000000 ) ) ;
#18570=CARTESIAN_POINT ( 'NONE',  ( -198.0356074513804572, -2.321818583541004323E-13, 55.37879056873073580 ) ) ;
#18572=CARTESIAN_POINT ( 'NONE',  ( 27.55177309528054863, 41.56868263114863282, -22.48880744266877940 ) ) ;
#18573=CARTESIAN_POINT ( 'NONE',  ( 19.06497207195980792, 54.19242893257844429, -40.00000000000002132 ) ) ;
#18574=CARTESIAN_POINT ( 'NONE',  ( 170.2234770963711128, 24.55285855007190321, 0.000000000000000000 ) ) ;
#18576=EDGE_CURVE ( 'NONE', #10807, #24743, #19687, .T. ) ;
#18577=CARTESIAN_POINT ( 'NONE',  ( -4.260882601032464301, -46.91379881627281634, 13.81249720866922281 ) ) ;
#18578=CARTESIAN_POINT ( 'NONE',  ( 57.59792236341147031, 37.56421063658187620, 40.00000000000002132 ) ) ;
#18579=ADVANCED_FACE ( 'NONE', ( #16042 ), #7037, .T. ) ;
#18581=DIRECTION ( 'NONE',  ( 0.000000000000000000, 1.000000000000000000, 0.000000000000000000 ) ) ;
#18583=CARTESIAN_POINT ( 'NONE',  ( -77.71213746886081708, 19.08763273111125258, 11.02205165069162973 ) ) ;
#18587=CARTESIAN_POINT ( 'NONE',  ( -4.151555265633122715, 13.82020782288901728, -46.95165237383025669 ) ) ;
#18589=CARTESIAN_POINT ( 'NONE',  ( -87.12809909135488340, -21.45715697399372957, 1.359879344826744774 ) ) ;
#18590=CARTESIAN_POINT ( 'NONE',  ( -86.95493927446865712, 6.698173996907309302, 20.33927854521555290 ) ) ;
#18591=CARTESIAN_POINT ( 'NONE',  ( -192.9370379451644055, -24.26711011076518787, 44.11033005022603959 ) ) ;
#18592=CARTESIAN_POINT ( 'NONE',  ( -162.0762913951021176, -27.08623940707584055, -29.48230308784799547 ) ) ;
#18593=CARTESIAN_POINT ( 'NONE',  ( -105.3220005116024112, 10.86457728909803144, -18.46446237098378518 ) ) ;
#18594=CARTESIAN_POINT ( 'NONE',  ( -188.8842637254077488, 17.93596642850458522, -43.30125340596324435 ) ) ;
#18595=CARTESIAN_POINT ( 'NONE',  ( 91.82158438592158234, 16.11829626348378142, 40.45024623143977749 ) ) ;
#18596=CARTESIAN_POINT ( 'NONE',  ( 192.4448373802101173, 14.14213562370261279, 42.42640687122091236 ) ) ;
#18597=CARTESIAN_POINT ( 'NONE',  ( -259.2033419157646676, -30.48217210827744239, -2.449293598294708485E-15 ) ) ;
#18598=CARTESIAN_POINT ( 'NONE',  ( 130.8568914410475372, 5.949712681206715814, 2.449293598294708485E-15 ) ) ;
#18599=CARTESIAN_POINT ( 'NONE',  ( -91.56559293963834989, -40.00000000000027711, 22.67402823373149801 ) ) ;
#18600=CARTESIAN_POINT ( 'NONE',  ( -30.26275506840323715, 29.48230279907789253, 29.48230279907799556 ) ) ;
#18601=CARTESIAN_POINT ( 'NONE',  ( -93.01854144614533482, 20.65013722618569147, -8.553566904202646981 ) ) ;
#18602=CARTESIAN_POINT ( 'NONE',  ( 91.82158438592159655, 12.16597498400091304, -44.40256751092321963 ) ) ;
#18603=CARTESIAN_POINT ( 'NONE',  ( 4.995406935893293543, -10.78321810389005364, 10.78321810388994173 ) ) ;
#18605=CARTESIAN_POINT ( 'NONE',  ( -135.8532207217289738, -34.75652343174615311, 21.81201906317767936 ) ) ;
#18606=CARTESIAN_POINT ( 'NONE',  ( -105.4741150117390021, 8.366608964593581277, 19.60045294982720776 ) ) ;
#18607=CARTESIAN_POINT ( 'NONE',  ( -259.2033419157646676, 6.730120644403214669, 49.83842185052034068 ) ) ;
#18608=CARTESIAN_POINT ( 'NONE',  ( 9.349823541315933184, -44.88994471603697178, -18.59402391556391620 ) ) ;
#18610=CARTESIAN_POINT ( 'NONE',  ( 0.2972598230769930572, 14.33493731733933352, 0.000000000000000000 ) ) ;
#18611=CARTESIAN_POINT ( 'NONE',  ( -87.11181986219450835, -13.17798114315252889, -17.01574595262779610 ) ) ;
#18614=FACE_OUTER_BOUND ( 'NONE', #19038, .T. ) ;
#18615=CARTESIAN_POINT ( 'NONE',  ( -190.7346372394673608, -43.65255821758116639, -23.92885340725679555 ) ) ;
#18616=B_SPLINE_CURVE_WITH_KNOTS ( 'NONE', 3,
 ( #11895, #1663, #23736, #22154, #19744, #9772, #1534, #18009, #10038, #9638, #17740, #7374, #5781, #13887, #20017, #1800, #26154, #16425, #18551, #22290, #14687, #22820, #14158, #6439, #14556, #24284, #20823, #6307, #18415, #22556, #24682, #22687, #8435, #26294 ),
 .UNSPECIFIED., .F., .F.,
 ( 4, 2, 2, 2, 2, 2, 2, 2, 2, 2, 2, 2, 2, 2, 2, 2, 4 ),
 ( -5.298243351207459470E-05, 0.01887868273877534031, 0.02834451532491906456, 0.03071097347145497133, 0.03307743161799088505, 0.03544388976452679529, 0.03781034791106270554, 0.04254326420413452603, 0.04727618049720634652, 0.04964263864374224983, 0.05200909679027816701, 0.05674201308334989730, 0.05910847122988576591, 0.06029170030315365858, 0.06147492937642155819, 0.06620784566949312888, 0.07567367825563638128 ),
 .UNSPECIFIED. ) ;
#18617=( BOUNDED_SURFACE ( )  B_SPLINE_SURFACE ( 3, 3, ( 
 ( #1714, #5694, #5569, #15925, #13799, #11673, #14208, #17661, #21934, #19665, #3845, #19797, #5834, #26071, #25802, #8085, #9552, #15662, #13675, #24195, #9953, #26213, #16205, #3709, #21797, #11811, #22209, #24337, #20203, #19931 ),
 ( #24058, #3984, #5967, #3570, #9824, #1584, #15792, #9687, #7949, #6101, #22342, #12082, #4119, #17793, #13937, #1983, #25938, #17927, #7809, #22073, #11949, #7680, #20074, #16067, #14078, #20337, #16602, #241, #2652, #12343 ),
 ( #24465, #25004, #10758, #18464, #10489, #8218, #14473, #6757, #18735, #6231, #2510, #20869, #8354, #10223, #2376, #4253, #16336, #518, #20741, #4511, #18602, #12613, #4382, #10624, #8485, #16475, #16734, #8623, #8757, #24866 ),
 ( #24599, #18869, #20472, #650, #6354, #14869, #12474, #22605, #16872, #6620, #23003, #14344, #22474, #20601, #381, #2246, #10353, #24735, #14738, #6491, #22869, #111, #14603, #22732, #12749, #12215, #4646, #2114, #18330, #11267 ),
 ( #9026, #25647, #17130, #9142, #25262, #21138, #3037, #2782, #2913, #21392, #1041, #19261, #5040, #11146, #17257, #1173, #11021, #19131, #913, #13018, #12884, #8889, #25394, #7012, #21000, #11386, #23390, #19386, #25135, #4781 ),
 ( #7145, #19007, #15133, #17000, #15505, #23264, #13146, #21265, #6887, #15261, #5164, #23135, #7393, #10894, #13270, #784, #3165, #4907, #9275, #17383, #15002, #21516, #25522, #7269, #15387, #23510, #5284, #13390, #1293, #3289 ),
 ( #19508, #9400, #17507, #12052, #9925, #21771, #24164, #25908, #3954, #13911, #14047, #3544, #23892, #11514, #7921, #10061, #21640, #1423, #20171, #26314, #15898, #3819, #11644, #9662, #21902, #19767, #20044, #17631, #1954, #1557 ) ),
 .UNSPECIFIED., .T., .F., .F. ) 
 B_SPLINE_SURFACE_WITH_KNOTS ( ( 4, 3, 4 ),
 ( 4, 2, 2, 2, 2, 2, 2, 2, 2, 2, 2, 2, 2, 2, 4 ),
 ( 0.000000000000000000, 0.5000000000000000000, 1.000000000000000000 ),
 ( 0.000000000000000000, 0.1357259735107005372, 0.1651108541090157700, 0.1944957347073310028, 0.3598804999793158710, 0.3867117631979620773, 0.4135430264166082281, 0.5789277916885930964, 0.6062785021374117456, 0.6336292125862302838, 0.8508620842112317728, 0.8814014469398914198, 0.9119408096685510667, 0.9559704048342755334, 1.000000000000000000 ),
 .UNSPECIFIED. ) 
 GEOMETRIC_REPRESENTATION_ITEM ( )  RATIONAL_B_SPLINE_SURFACE ( (
 ( 1.000000000000000000, 1.000000000000000000, 1.000000000000000000, 1.000000000000000000, 1.000000000000000000, 1.000000000000000000, 1.000000000000000000, 1.000000000000000000, 1.000000000000000000, 1.000000000000000000, 1.000000000000000000, 1.000000000000000000, 1.000000000000000000, 1.000000000000000000, 1.000000000000000000, 1.000000000000000000, 1.000000000000000000, 1.000000000000000000, 1.000000000000000000, 1.000000000000000000, 1.000000000000000000, 1.000000000000000000, 1.000000000000000000, 1.000000000000000000, 1.000000000000000000, 1.000000000000000000, 1.000000000000000000, 1.000000000000000000, 1.000000000000000000, 1.000000000000000000),
 ( 0.3333333333333333703, 0.3333333333333333703, 0.3333333333333333703, 0.3333333333333333703, 0.3333333333333333703, 0.3333333333333333703, 0.3333333333333333703, 0.3333333333333333703, 0.3333333333333333703, 0.3333333333333333703, 0.3333333333333333703, 0.3333333333333333703, 0.3333333333333333703, 0.3333333333333333703, 0.3333333333333333703, 0.3333333333333333703, 0.3333333333333333703, 0.3333333333333333703, 0.3333333333333333703, 0.3333333333333333703, 0.3333333333333333703, 0.3333333333333333703, 0.3333333333333333703, 0.3333333333333333703, 0.3333333333333333703, 0.3333333333333333703, 0.3333333333333333703, 0.3333333333333333703, 0.3333333333333333703, 0.3333333333333333703),
 ( 0.3333333333333333703, 0.3333333333333333703, 0.3333333333333333703, 0.3333333333333333703, 0.3333333333333333703, 0.3333333333333333703, 0.3333333333333333703, 0.3333333333333333703, 0.3333333333333333703, 0.3333333333333333703, 0.3333333333333333703, 0.3333333333333333703, 0.3333333333333333703, 0.3333333333333333703, 0.3333333333333333703, 0.3333333333333333703, 0.3333333333333333703, 0.3333333333333333703, 0.3333333333333333703, 0.3333333333333333703, 0.3333333333333333703, 0.3333333333333333703, 0.3333333333333333703, 0.3333333333333333703, 0.3333333333333333703, 0.3333333333333333703, 0.3333333333333333703, 0.3333333333333333703, 0.3333333333333333703, 0.3333333333333333703),
 ( 1.000000000000000000, 1.000000000000000000, 1.000000000000000000, 1.000000000000000000, 1.000000000000000000, 1.000000000000000000, 1.000000000000000000, 1.000000000000000000, 1.000000000000000000, 1.000000000000000000, 1.000000000000000000, 1.000000000000000000, 1.000000000000000000, 1.000000000000000000, 1.000000000000000000, 1.000000000000000000, 1.000000000000000000, 1.000000000000000000, 1.000000000000000000, 1.000000000000000000, 1.000000000000000000, 1.000000000000000000, 1.000000000000000000, 1.000000000000000000, 1.000000000000000000, 1.000000000000000000, 1.000000000000000000, 1.000000000000000000, 1.000000000000000000, 1.000000000000000000),
 ( 0.3333333333333333703, 0.3333333333333333703, 0.3333333333333333703, 0.3333333333333333703, 0.3333333333333333703, 0.3333333333333333703, 0.3333333333333333703, 0.3333333333333333703, 0.3333333333333333703, 0.3333333333333333703, 0.3333333333333333703, 0.3333333333333333703, 0.3333333333333333703, 0.3333333333333333703, 0.3333333333333333703, 0.3333333333333333703, 0.3333333333333333703, 0.3333333333333333703, 0.3333333333333333703, 0.3333333333333333703, 0.3333333333333333703, 0.3333333333333333703, 0.3333333333333333703, 0.3333333333333333703, 0.3333333333333333703, 0.3333333333333333703, 0.3333333333333333703, 0.3333333333333333703, 0.3333333333333333703, 0.3333333333333333703),
 ( 0.3333333333333333703, 0.3333333333333333703, 0.3333333333333333703, 0.3333333333333333703, 0.3333333333333333703, 0.3333333333333333703, 0.3333333333333333703, 0.3333333333333333703, 0.3333333333333333703, 0.3333333333333333703, 0.3333333333333333703, 0.3333333333333333703, 0.3333333333333333703, 0.3333333333333333703, 0.3333333333333333703, 0.3333333333333333703, 0.3333333333333333703, 0.3333333333333333703, 0.3333333333333333703, 0.3333333333333333703, 0.3333333333333333703, 0.3333333333333333703, 0.3333333333333333703, 0.3333333333333333703, 0.3333333333333333703, 0.3333333333333333703, 0.3333333333333333703, 0.3333333333333333703, 0.3333333333333333703, 0.3333333333333333703),
 ( 1.000000000000000000, 1.000000000000000000, 1.000000000000000000, 1.000000000000000000, 1.000000000000000000, 1.000000000000000000, 1.000000000000000000, 1.000000000000000000, 1.000000000000000000, 1.000000000000000000, 1.000000000000000000, 1.000000000000000000, 1.000000000000000000, 1.000000000000000000, 1.000000000000000000, 1.000000000000000000, 1.000000000000000000, 1.000000000000000000, 1.000000000000000000, 1.000000000000000000, 1.000000000000000000, 1.000000000000000000, 1.000000000000000000, 1.000000000000000000, 1.000000000000000000, 1.000000000000000000, 1.000000000000000000, 1.000000000000000000, 1.000000000000000000, 1.000000000000000000) ) ) 
 REPRESENTATION_ITEM ( '' )  SURFACE ( )  );
#18618=CARTESIAN_POINT ( 'NONE',  ( 14.38125909742181818, -1.924622159709266762E-13, 55.17850393972636880 ) ) ;
#18619=CARTESIAN_POINT ( 'NONE',  ( -198.0356074513804572, 55.37879056874818673, -40.00000000000002132 ) ) ;
#18622=CARTESIAN_POINT ( 'NONE',  ( 130.8568914410475088, -40.00000000000001421, 5.949712681206549725 ) ) ;
#18623=CARTESIAN_POINT ( 'NONE',  ( -280.0000000000000000, 1.839446121267387017E-14, -20.00000000000001421 ) ) ;
#18624=CARTESIAN_POINT ( 'NONE',  ( -200.0000000000000000, 1.308061781956697717E-29, 0.000000000000000000 ) ) ;
#18625=CARTESIAN_POINT ( 'NONE',  ( -280.0000000000000568, 19.99999999999996092, -40.00000000000002132 ) ) ;
#18626=CARTESIAN_POINT ( 'NONE',  ( -91.56559293963834989, -17.32597176626812185, -40.00000000000002132 ) ) ;
#18627=CARTESIAN_POINT ( 'NONE',  ( -162.0762913951021176, 27.08623940707598265, 29.48230308784781428 ) ) ;
#18628=CARTESIAN_POINT ( 'NONE',  ( 14.38125909742181108, 1.616281842095393922E-13, -15.17850393972633682 ) ) ;
#18629=CARTESIAN_POINT ( 'NONE',  ( -138.9613193423056146, -13.65853114841830696, 27.95779829447857523 ) ) ;
#18630=CARTESIAN_POINT ( 'NONE',  ( 151.7948205124836534, 40.00000000000012079, -6.767089262348609857 ) ) ;
#18631=CARTESIAN_POINT ( 'NONE',  ( 163.1118516004056573, -40.00000000000003553, 12.73709011382460687 ) ) ;
#18632=CARTESIAN_POINT ( 'NONE',  ( 170.2234770963711128, 10.92277846919210660, -45.64576402573182889 ) ) ;
#18634=CARTESIAN_POINT ( 'NONE',  ( -114.7537493279955214, -13.57142477595643371, 17.50316801954799928 ) ) ;
#18635=CARTESIAN_POINT ( 'NONE',  ( -192.9588430854689705, -38.51493924976963967, 38.51493924976919914 ) ) ;
#18637=CARTESIAN_POINT ( 'NONE',  ( -4.915070467873956517, 42.74707758271757285, -23.27857837409175801 ) ) ;
#18639=CARTESIAN_POINT ( 'NONE',  ( 19.06497207195982924, -54.19242893257843008, -40.00000000000002132 ) ) ;
#18640=CARTESIAN_POINT ( 'NONE',  ( -87.02160967420090287, -20.76757794971305060, -5.405368517529804073 ) ) ;
#18641=CARTESIAN_POINT ( 'NONE',  ( -208.1127848780265026, 15.00245453012665564, 0.000000000000000000 ) ) ;
#18642=ORIENTED_EDGE ( 'NONE', *, *, #1194, .F. ) ;
#18645=CARTESIAN_POINT ( 'NONE',  ( -97.73860346106548036, 8.185503821063067065, -20.89580782303987050 ) ) ;
#18646=CARTESIAN_POINT ( 'NONE',  ( 12.77879914714818632, 18.55776024549972547, 44.80239647188651020 ) ) ;
#18649=CARTESIAN_POINT ( 'NONE',  ( -192.9588430854690273, 10.23066800231970319, 66.79921049724369198 ) ) ;
#18652=CARTESIAN_POINT ( 'NONE',  ( -105.3755690713226727, -15.38646221621786481, -15.38646221621789856 ) ) ;
#18654=DIRECTION ( 'NONE',  ( 1.000000000000000000, 0.000000000000000000, 0.000000000000000000 ) ) ;
#18656=CARTESIAN_POINT ( 'NONE',  ( 136.1360204305621551, 40.00000000000009948, -4.966164525586641787 ) ) ;
#18657=CARTESIAN_POINT ( 'NONE',  ( -259.2033419157646676, 40.00000000000029843, -30.48217210827696988 ) ) ;
#18662=CARTESIAN_POINT ( 'NONE',  ( -188.9478457324750877, 17.94276812689866674, 43.31767415847477309 ) ) ;
#18663=CARTESIAN_POINT ( 'NONE',  ( -238.4067589809705794, -28.96627169325352469, 27.60227080167035041 ) ) ;
#18664=CARTESIAN_POINT ( 'NONE',  ( -86.86493150571116928, 8.366608963953661160, 19.60045294882771572 ) ) ;
#18665=CARTESIAN_POINT ( 'NONE',  ( 91.82158438592159655, -16.11829626346147393, 16.11829626346132116 ) ) ;
#18667=CARTESIAN_POINT ( 'NONE',  ( 151.7948205124836534, 23.49921654116056047, -33.06932595376338213 ) ) ;
#18669=CARTESIAN_POINT ( 'NONE',  ( 146.6084372240433993, 34.62501878078308692, 0.000000000000000000 ) ) ;
#18671=CARTESIAN_POINT ( 'NONE',  ( -198.0356074513804572, 67.44298959250878056, -10.87444709758402261 ) ) ;
#18672=CARTESIAN_POINT ( 'NONE',  ( 4.995406935893293543, -15.24977328854832592, 0.000000000000000000 ) ) ;
#18674=CARTESIAN_POINT ( 'NONE',  ( -198.0356074513804572, -39.99999999999948130, -55.37879056874863437 ) ) ;
#18676=EDGE_CURVE ( 'NONE', #25051, #3040, #23844, .T. ) ;
#18678=B_SPLINE_CURVE_WITH_KNOTS ( 'NONE', 3,
 ( #24898, #16901, #22637, #6264, #24767, #278 ),
 .UNSPECIFIED., .F., .F.,
 ( 4, 2, 4 ),
 ( 1.971482511941758420E-15, 0.03937685683732546071, 0.07875371367464895078 ),
 .UNSPECIFIED. ) ;
#18681=CARTESIAN_POINT ( 'NONE',  ( 19.06497207195980792, 14.19242893257840876, 0.000000000000000000 ) ) ;
#18684=CARTESIAN_POINT ( 'NONE',  ( 130.8568914410475372, 4.207082182992923691, -4.207082182992794017 ) ) ;
#18685=CARTESIAN_POINT ( 'NONE',  ( 90.68848423409737336, 21.28058941648435720, -8.814708753004696362 ) ) ;
#18691=CARTESIAN_POINT ( 'NONE',  ( 192.4448373802101173, -42.42640687122053578, -14.14213562370360577 ) ) ;
#18692=CARTESIAN_POINT ( 'NONE',  ( -105.3755690713226727, 15.38646221621771737, 15.38646221621800514 ) ) ;
#18693=CARTESIAN_POINT ( 'NONE',  ( -114.5171371270916296, 20.71058515352653018, 7.156716672343439001 ) ) ;
#18695=CARTESIAN_POINT ( 'NONE',  ( 14.38125909742180930, 40.00000000000060396, -55.17850393974224232 ) ) ;
#18696=CARTESIAN_POINT ( 'NONE',  ( -192.9588430854689989, -10.23066800230742501, -10.23066800230756712 ) ) ;
#18697=CARTESIAN_POINT ( 'NONE',  ( -100.7734535825088500, 22.67402823373189591, -0.000000000000000000 ) ) ;
#18698=CARTESIAN_POINT ( 'NONE',  ( 146.6084372240433993, -24.48358557860353457, 24.48358557860296258 ) ) ;
#18699=CARTESIAN_POINT ( 'NONE',  ( -135.8532207217289738, -21.81201906317758343, -34.75652343174620995 ) ) ;
#18703=CARTESIAN_POINT ( 'NONE',  ( -213.1075012329537230, -2.291445344039133686E-13, 53.71589010951915100 ) ) ;
#18705=CARTESIAN_POINT ( 'NONE',  ( 23.36462152323055363, 46.81175967489679834, -13.80148662728979581 ) ) ;
#18706=CARTESIAN_POINT ( 'NONE',  ( -91.56559293963834989, -22.67402823373193499, -40.00000000000002132 ) ) ;
#18707=CARTESIAN_POINT ( 'NONE',  ( 192.4448373802100889, -14.14213562375876698, -14.14213562375885047 ) ) ;
#18708=CARTESIAN_POINT ( 'NONE',  ( -213.1075012329537230, 13.71589010951907817, 40.00000000000002132 ) ) ;
#18709=CARTESIAN_POINT ( 'NONE',  ( -62.72988123315177944, -25.36777511011030484, 10.50767649784149427 ) ) ;
#18710=CARTESIAN_POINT ( 'NONE',  ( 184.8905102610680444, 19.07866798485561333, 40.00000000000002132 ) ) ;
#18712=CARTESIAN_POINT ( 'NONE',  ( -196.0240701931631691, -48.96019555158521541, -14.12332411430270440 ) ) ;
#18713=CARTESIAN_POINT ( 'NONE',  ( -3.488770945845345750, -17.93216134257419014, 43.29206711590394008 ) ) ;
#18714=AXIS2_PLACEMENT_3D ( 'NONE', #2959, #16659, #18792 ) ;
#18715=CARTESIAN_POINT ( 'NONE',  ( -4.081455915265743251, 17.86600351371890127, -43.13234798823334160 ) ) ;
#18717=CARTESIAN_POINT ( 'NONE',  ( 14.38125909742180752, 10.73282306404735387, -10.73282306404708919 ) ) ;
#18718=CARTESIAN_POINT ( 'NONE',  ( -77.56353172720405098, -22.09247646619704497, 1.385506815421064353 ) ) ;
#18719=CARTESIAN_POINT ( 'NONE',  ( -4.039451493210478361, -43.00522595893993838, -23.44932283416681429 ) ) ;
#18720=CARTESIAN_POINT ( 'NONE',  ( -188.9001659262686132, -17.93767091109507916, 43.30536839095043433 ) ) ;
#18721=CARTESIAN_POINT ( 'NONE',  ( -100.7734535825088500, 16.03295912088691821, 16.03295912088721309 ) ) ;
#18723=CARTESIAN_POINT ( 'NONE',  ( -135.8532207217289738, -34.75652343174584757, -21.81201906317816253 ) ) ;
#18724=FACE_OUTER_BOUND ( 'NONE', #19210, .T. ) ;
#18725=( BOUNDED_SURFACE ( )  B_SPLINE_SURFACE ( 3, 3, ( 
 ( #11138, #21385, #4771, #16992, #906, #508, #22860, #12876, #25386, #1034, #13139, #642, #4637, #9018, #17249, #19254, #17123, #7005, #20992, #12739, #18861, #10750, #16725, #15125, #20859, #6749, #7138, #2642, #21258, #16864 ),
 ( #24996, #24856, #15253, #14861, #23383, #23256, #23128, #5157, #22995, #6608, #13262, #13009, #14993, #21131, #2906, #7386, #15888, #21761, #9393, #23503, #1547, #13636, #9652, #1416, #3535, #3668, #23882, #19632, #23748, #21630 ),
 ( #1165, #9517, #11379, #17623, #3406, #15497, #11635, #23627, #5277, #5406, #19758, #24016, #13507, #17757, #1285, #11507, #5530, #25767, #13902, #25640, #15380, #17887, #9268, #11777, #25898, #1680, #7517, #15625, #7639, #5794 ),
 ( #19895, #15754, #5659, #13382, #11259, #21892, #22035, #13765, #9785, #26036, #19377, #7262, #7773, #17376, #25515, #21509, #19500, #3281, #17499, #12438, #14438, #4080, #2212, #205, #9916, #16166, #22303, #24155, #14170, #12181 ),
 ( #22439, #7912, #20302, #8049, #16030, #76, #8185, #10451, #4216, #20035, #14567, #1813, #12306, #12044, #20164, #2079, #24300, #20566, #24426, #18564, #5932, #343, #26306, #8447, #14305, #1946, #14038, #20433, #6192, #10321 ),
 ( #16302, #22173, #6068, #16566, #3947, #10186, #22567, #18022, #18290, #10053, #18428, #8314, #16437, #24563, #6318, #18160, #4346, #2337, #24696, #6451, #3808, #11913, #26171, #8853, #24969, #25358, #10722, #480, #3004, #20704 ),
 ( #12706, #12849, #16836, #20965, #9109, #17094, #18696, #5005, #10850, #18831, #8585, #22697, #6979, #7113, #8718, #22962, #14967, #4472, #16696, #6716, #11110, #13110, #25226, #4610, #24829, #23102, #21231, #15093, #4742, #21100 ) ),
 .UNSPECIFIED., .T., .F., .T. ) 
 B_SPLINE_SURFACE_WITH_KNOTS ( ( 4, 3, 4 ),
 ( 4, 2, 2, 2, 2, 2, 2, 2, 2, 2, 2, 2, 2, 2, 4 ),
 ( 0.000000000000000000, 0.5000000000000000000, 1.000000000000000000 ),
 ( 0.000000000000000000, 0.1357259735107005372, 0.1651108541090157700, 0.1944957347073310028, 0.3598804999793158710, 0.3867117631979620773, 0.4135430264166082281, 0.5789277916885930964, 0.6062785021374117456, 0.6336292125862302838, 0.8508620842112317728, 0.8814014469398914198, 0.9119408096685510667, 0.9559704048342755334, 1.000000000000000000 ),
 .UNSPECIFIED. ) 
 GEOMETRIC_REPRESENTATION_ITEM ( )  RATIONAL_B_SPLINE_SURFACE ( (
 ( 1.000000000000000000, 1.000000000000000000, 1.000000000000000000, 1.000000000000000000, 1.000000000000000000, 1.000000000000000000, 1.000000000000000000, 1.000000000000000000, 1.000000000000000000, 1.000000000000000000, 1.000000000000000000, 1.000000000000000000, 1.000000000000000000, 1.000000000000000000, 1.000000000000000000, 1.000000000000000000, 1.000000000000000000, 1.000000000000000000, 1.000000000000000000, 1.000000000000000000, 1.000000000000000000, 1.000000000000000000, 1.000000000000000000, 1.000000000000000000, 1.000000000000000000, 1.000000000000000000, 1.000000000000000000, 1.000000000000000000, 1.000000000000000000, 1.000000000000000000),
 ( 0.3333333333333333703, 0.3333333333333333703, 0.3333333333333333703, 0.3333333333333333703, 0.3333333333333333703, 0.3333333333333333703, 0.3333333333333333703, 0.3333333333333333703, 0.3333333333333333703, 0.3333333333333333703, 0.3333333333333333703, 0.3333333333333333703, 0.3333333333333333703, 0.3333333333333333703, 0.3333333333333333703, 0.3333333333333333703, 0.3333333333333333703, 0.3333333333333333703, 0.3333333333333333703, 0.3333333333333333703, 0.3333333333333333703, 0.3333333333333333703, 0.3333333333333333703, 0.3333333333333333703, 0.3333333333333333703, 0.3333333333333333703, 0.3333333333333333703, 0.3333333333333333703, 0.3333333333333333703, 0.3333333333333333703),
 ( 0.3333333333333333703, 0.3333333333333333703, 0.3333333333333333703, 0.3333333333333333703, 0.3333333333333333703, 0.3333333333333333703, 0.3333333333333333703, 0.3333333333333333703, 0.3333333333333333703, 0.3333333333333333703, 0.3333333333333333703, 0.3333333333333333703, 0.3333333333333333703, 0.3333333333333333703, 0.3333333333333333703, 0.3333333333333333703, 0.3333333333333333703, 0.3333333333333333703, 0.3333333333333333703, 0.3333333333333333703, 0.3333333333333333703, 0.3333333333333333703, 0.3333333333333333703, 0.3333333333333333703, 0.3333333333333333703, 0.3333333333333333703, 0.3333333333333333703, 0.3333333333333333703, 0.3333333333333333703, 0.3333333333333333703),
 ( 1.000000000000000000, 1.000000000000000000, 1.000000000000000000, 1.000000000000000000, 1.000000000000000000, 1.000000000000000000, 1.000000000000000000, 1.000000000000000000, 1.000000000000000000, 1.000000000000000000, 1.000000000000000000, 1.000000000000000000, 1.000000000000000000, 1.000000000000000000, 1.000000000000000000, 1.000000000000000000, 1.000000000000000000, 1.000000000000000000, 1.000000000000000000, 1.000000000000000000, 1.000000000000000000, 1.000000000000000000, 1.000000000000000000, 1.000000000000000000, 1.000000000000000000, 1.000000000000000000, 1.000000000000000000, 1.000000000000000000, 1.000000000000000000, 1.000000000000000000),
 ( 0.3333333333333333703, 0.3333333333333333703, 0.3333333333333333703, 0.3333333333333333703, 0.3333333333333333703, 0.3333333333333333703, 0.3333333333333333703, 0.3333333333333333703, 0.3333333333333333703, 0.3333333333333333703, 0.3333333333333333703, 0.3333333333333333703, 0.3333333333333333703, 0.3333333333333333703, 0.3333333333333333703, 0.3333333333333333703, 0.3333333333333333703, 0.3333333333333333703, 0.3333333333333333703, 0.3333333333333333703, 0.3333333333333333703, 0.3333333333333333703, 0.3333333333333333703, 0.3333333333333333703, 0.3333333333333333703, 0.3333333333333333703, 0.3333333333333333703, 0.3333333333333333703, 0.3333333333333333703, 0.3333333333333333703),
 ( 0.3333333333333333703, 0.3333333333333333703, 0.3333333333333333703, 0.3333333333333333703, 0.3333333333333333703, 0.3333333333333333703, 0.3333333333333333703, 0.3333333333333333703, 0.3333333333333333703, 0.3333333333333333703, 0.3333333333333333703, 0.3333333333333333703, 0.3333333333333333703, 0.3333333333333333703, 0.3333333333333333703, 0.3333333333333333703, 0.3333333333333333703, 0.3333333333333333703, 0.3333333333333333703, 0.3333333333333333703, 0.3333333333333333703, 0.3333333333333333703, 0.3333333333333333703, 0.3333333333333333703, 0.3333333333333333703, 0.3333333333333333703, 0.3333333333333333703, 0.3333333333333333703, 0.3333333333333333703, 0.3333333333333333703),
 ( 1.000000000000000000, 1.000000000000000000, 1.000000000000000000, 1.000000000000000000, 1.000000000000000000, 1.000000000000000000, 1.000000000000000000, 1.000000000000000000, 1.000000000000000000, 1.000000000000000000, 1.000000000000000000, 1.000000000000000000, 1.000000000000000000, 1.000000000000000000, 1.000000000000000000, 1.000000000000000000, 1.000000000000000000, 1.000000000000000000, 1.000000000000000000, 1.000000000000000000, 1.000000000000000000, 1.000000000000000000, 1.000000000000000000, 1.000000000000000000, 1.000000000000000000, 1.000000000000000000, 1.000000000000000000, 1.000000000000000000, 1.000000000000000000, 1.000000000000000000) ) ) 
 REPRESENTATION_ITEM ( '' )  SURFACE ( )  );
#18727=CARTESIAN_POINT ( 'NONE',  ( 0.2972598230769907257, 66.70487387989869887, -10.13633138497392494 ) ) ;
#18728=CARTESIAN_POINT ( 'NONE',  ( 57.59792236341147031, -1.722363176415055985, 1.722363176415024677 ) ) ;
#18729=CARTESIAN_POINT ( 'NONE',  ( -30.26275506840323004, -41.69427246844627888, -40.00000000000002132 ) ) ;
#18730=CARTESIAN_POINT ( 'NONE',  ( -91.56559293963834989, 17.32597176626808988, 40.00000000000002132 ) ) ;
#18732=CARTESIAN_POINT ( 'NONE',  ( -198.0356074513804572, -39.99999999999990052, -15.37879056873112482 ) ) ;
#18733=CARTESIAN_POINT ( 'NONE',  ( 146.6084372240433709, 3.800685668858776900, -52.76785682606518435 ) ) ;
#18735=CARTESIAN_POINT ( 'NONE',  ( -135.8532207217289738, 6.472252184284583265, -50.09629031063960980 ) ) ;
#18739=CARTESIAN_POINT ( 'NONE',  ( 184.8905102610680444, 13.49065550809807945, 13.49065550809809544 ) ) ;
#18742=CARTESIAN_POINT ( 'NONE',  ( 57.59792236341148453, 1.722363176414758668, 54.84617931850880268 ) ) ;
#18743=CARTESIAN_POINT ( 'NONE',  ( 8.602182264136155609, -44.88373884392252933, -18.59145335915702901 ) ) ;
#18744=ORIENTED_EDGE ( 'NONE', *, *, #22984, .F. ) ;
#18745=CARTESIAN_POINT ( 'NONE',  ( 17.76569288431005234, -48.46476365406682163, -14.04863394049459302 ) ) ;
#18746=CARTESIAN_POINT ( 'NONE',  ( -102.2610585947573298, -15.74993999358153829, -15.74993999358157204 ) ) ;
#18749=CARTESIAN_POINT ( 'NONE',  ( -114.6382724355125191, -21.35157561685035787, 5.497872032160216804 ) ) ;
#18750=CARTESIAN_POINT ( 'NONE',  ( 130.8568914410475088, 5.949712681206712261, 40.00000000000002132 ) ) ;
#18755=CARTESIAN_POINT ( 'NONE',  ( -86.96347745069643054, -41.18208027870611687, 15.38646221621750954 ) ) ;
#18756=CARTESIAN_POINT ( 'NONE',  ( -198.0356074513804572, 39.99999999999979394, 55.37879056874835726 ) ) ;
#18757=CARTESIAN_POINT ( 'NONE',  ( -100.7734535825088500, 39.99999999999994316, 17.32597176626825686 ) ) ;
#18758=CARTESIAN_POINT ( 'NONE',  ( -200.0000000000000853, -24.82633483071228753, -44.86878812508721381 ) ) ;
#18759=CARTESIAN_POINT ( 'NONE',  ( -56.48582580120559271, 9.153146818113576444, -0.000000000000000000 ) ) ;
#18761=CARTESIAN_POINT ( 'NONE',  ( -135.8532207217289738, -30.84685318188647685, -2.449293598294708485E-15 ) ) ;
#18762=CARTESIAN_POINT ( 'NONE',  ( 14.38125909742181996, -10.73282306403606157, 67.30136555895948902 ) ) ;
#18763=CARTESIAN_POINT ( 'NONE',  ( 147.2817042152898352, -12.35516179550122118, -29.82799917201325002 ) ) ;
#18764=CARTESIAN_POINT ( 'NONE',  ( -114.5514240058867586, 19.59008466206002197, -9.949107728601523704 ) ) ;
#18765=CARTESIAN_POINT ( 'NONE',  ( -238.4067589809705794, 3.877349844572403567E-13, -40.96449427998260973 ) ) ;
#18766=CARTESIAN_POINT ( 'NONE',  ( -100.7734535825088358, -8.145438380286941744E-14, 17.32597176626811120 ) ) ;
#18768=CARTESIAN_POINT ( 'NONE',  ( -105.4741150117398263, -19.77569912953930498, 7.943527260776862775 ) ) ;
#18769=CARTESIAN_POINT ( 'NONE',  ( -114.7252611291636128, -17.87002000140759250, 12.98773421617053714 ) ) ;
#18770=CARTESIAN_POINT ( 'NONE',  ( -105.3755690713226585, -41.18208027870589660, -15.38646221621809040 ) ) ;
#18773=CARTESIAN_POINT ( 'NONE',  ( -193.0908841288064650, 24.29092413197486522, -44.14257353178361143 ) ) ;
#18775=CARTESIAN_POINT ( 'NONE',  ( 130.8568914410475088, -5.949712681206664300, -40.00000000000002132 ) ) ;
#18782=CARTESIAN_POINT ( 'NONE',  ( 98.29820294267490510, 4.808046699556526995E-12, 20.00000000000513722 ) ) ;
#18783=CARTESIAN_POINT ( 'NONE',  ( 21.25019396252800519, 18.04326867293863756, 43.56030393974966586 ) ) ;
#18784=B_SPLINE_CURVE_WITH_KNOTS ( 'NONE', 3,
 ( #23690, #2967, #21697, #3473, #19691, #19192, #1479, #975, #9080, #17186, #15194, #5097, #13202, #21324 ),
 .UNSPECIFIED., .F., .F.,
 ( 4, 2, 2, 2, 2, 2, 4 ),
 ( 8.673617379884035472E-18, 0.002941681445496974190, 0.004412522168245463020, 0.005883362890993952717, 0.008825044336490939917, 0.01029588505923942701, 0.01176672578198791584 ),
 .UNSPECIFIED. ) ;
#18785=ORIENTED_EDGE ( 'NONE', *, *, #23766, .F. ) ;
#18786=VERTEX_POINT ( 'NONE', #13096 ) ;
#18787=( BOUNDED_SURFACE ( )  B_SPLINE_SURFACE ( 3, 3, ( 
 ( #24331, #23783, #6095, #15787, #23914, #5689, #13794, #21929, #4640, #16728, #22863, #24999, #22468, #105, #20862, #12606, #16596, #22600, #2504, #18728, #10482, #10615, #14597, #24592, #14864, #374, #20735, #2370, #6752, #14336 ),
 ( #8212, #4247, #12337, #2777, #16468, #22998, #6485, #20465, #12742, #6613, #8478, #2646, #512, #18864, #6348, #16330, #10753, #14467, #20995, #4376, #12466, #20594, #24729, #2239, #24859, #10347, #4505, #14731, #18596, #22726 ),
 ( #8617, #645, #8751, #16867, #18323, #18457, #4775, #12879, #235, #24459, #8347, #6223, #25389, #1288, #3284, #25643, #5035, #11382, #19503, #7008, #9396, #7265, #11017, #8884, #7141, #1168, #17503, #13510, #17253, #15256 ),
 ( #21134, #23386, #19127, #14996, #909, #19257, #11142, #21633, #3160, #19381, #10889, #19001, #17126, #23630, #7389, #5160, #5280, #23131, #1037, #15384, #15500, #778, #5409, #25518, #16995, #13266, #25130, #21388, #11262, #21512 ),
 ( #6880, #4903, #9137, #2909, #9271, #13013, #23506, #3033, #13385, #17379, #9022, #25257, #15129, #13142, #23259, #21261, #13905, #19898, #11780, #11916, #1551, #24302, #20166, #3538, #18162, #23885, #20038, #17760, #15757, #8051 ),
 ( #24157, #18025, #1683, #5934, #3811, #3949, #9655, #19636, #14040, #25901, #6070, #7642, #5662, #13768, #9788, #25770, #1816, #7520, #15891, #9919, #21895, #3672, #14172, #17890, #7776, #26039, #19761, #22175, #1948, #16168 ),
 ( #13639, #12046, #11638, #10055, #24019, #26308, #3409, #11510, #5798, #1419, #9520, #22039, #17626, #26174, #7914, #15628, #16032, #23751, #5533, #21765, #2339, #10453, #10188, #18698, #14569, #20836, #22699, #14307, #6718, #6584 ) ),
 .UNSPECIFIED., .T., .F., .F. ) 
 B_SPLINE_SURFACE_WITH_KNOTS ( ( 4, 3, 4 ),
 ( 4, 2, 2, 2, 2, 2, 2, 2, 2, 2, 2, 2, 2, 2, 4 ),
 ( 0.000000000000000000, 0.5000000000000000000, 1.000000000000000000 ),
 ( 0.000000000000000000, 0.1357259735107005372, 0.1651108541090157700, 0.1944957347073310028, 0.3598804999793158710, 0.3867117631979620773, 0.4135430264166082281, 0.5789277916885930964, 0.6062785021374117456, 0.6336292125862302838, 0.8508620842112317728, 0.8814014469398914198, 0.9119408096685510667, 0.9559704048342755334, 1.000000000000000000 ),
 .UNSPECIFIED. ) 
 GEOMETRIC_REPRESENTATION_ITEM ( )  RATIONAL_B_SPLINE_SURFACE ( (
 ( 1.000000000000000000, 1.000000000000000000, 1.000000000000000000, 1.000000000000000000, 1.000000000000000000, 1.000000000000000000, 1.000000000000000000, 1.000000000000000000, 1.000000000000000000, 1.000000000000000000, 1.000000000000000000, 1.000000000000000000, 1.000000000000000000, 1.000000000000000000, 1.000000000000000000, 1.000000000000000000, 1.000000000000000000, 1.000000000000000000, 1.000000000000000000, 1.000000000000000000, 1.000000000000000000, 1.000000000000000000, 1.000000000000000000, 1.000000000000000000, 1.000000000000000000, 1.000000000000000000, 1.000000000000000000, 1.000000000000000000, 1.000000000000000000, 1.000000000000000000),
 ( 0.3333333333333333703, 0.3333333333333333703, 0.3333333333333333703, 0.3333333333333333703, 0.3333333333333333703, 0.3333333333333333703, 0.3333333333333333703, 0.3333333333333333703, 0.3333333333333333703, 0.3333333333333333703, 0.3333333333333333703, 0.3333333333333333703, 0.3333333333333333703, 0.3333333333333333703, 0.3333333333333333703, 0.3333333333333333703, 0.3333333333333333703, 0.3333333333333333703, 0.3333333333333333703, 0.3333333333333333703, 0.3333333333333333703, 0.3333333333333333703, 0.3333333333333333703, 0.3333333333333333703, 0.3333333333333333703, 0.3333333333333333703, 0.3333333333333333703, 0.3333333333333333703, 0.3333333333333333703, 0.3333333333333333703),
 ( 0.3333333333333333703, 0.3333333333333333703, 0.3333333333333333703, 0.3333333333333333703, 0.3333333333333333703, 0.3333333333333333703, 0.3333333333333333703, 0.3333333333333333703, 0.3333333333333333703, 0.3333333333333333703, 0.3333333333333333703, 0.3333333333333333703, 0.3333333333333333703, 0.3333333333333333703, 0.3333333333333333703, 0.3333333333333333703, 0.3333333333333333703, 0.3333333333333333703, 0.3333333333333333703, 0.3333333333333333703, 0.3333333333333333703, 0.3333333333333333703, 0.3333333333333333703, 0.3333333333333333703, 0.3333333333333333703, 0.3333333333333333703, 0.3333333333333333703, 0.3333333333333333703, 0.3333333333333333703, 0.3333333333333333703),
 ( 1.000000000000000000, 1.000000000000000000, 1.000000000000000000, 1.000000000000000000, 1.000000000000000000, 1.000000000000000000, 1.000000000000000000, 1.000000000000000000, 1.000000000000000000, 1.000000000000000000, 1.000000000000000000, 1.000000000000000000, 1.000000000000000000, 1.000000000000000000, 1.000000000000000000, 1.000000000000000000, 1.000000000000000000, 1.000000000000000000, 1.000000000000000000, 1.000000000000000000, 1.000000000000000000, 1.000000000000000000, 1.000000000000000000, 1.000000000000000000, 1.000000000000000000, 1.000000000000000000, 1.000000000000000000, 1.000000000000000000, 1.000000000000000000, 1.000000000000000000),
 ( 0.3333333333333333703, 0.3333333333333333703, 0.3333333333333333703, 0.3333333333333333703, 0.3333333333333333703, 0.3333333333333333703, 0.3333333333333333703, 0.3333333333333333703, 0.3333333333333333703, 0.3333333333333333703, 0.3333333333333333703, 0.3333333333333333703, 0.3333333333333333703, 0.3333333333333333703, 0.3333333333333333703, 0.3333333333333333703, 0.3333333333333333703, 0.3333333333333333703, 0.3333333333333333703, 0.3333333333333333703, 0.3333333333333333703, 0.3333333333333333703, 0.3333333333333333703, 0.3333333333333333703, 0.3333333333333333703, 0.3333333333333333703, 0.3333333333333333703, 0.3333333333333333703, 0.3333333333333333703, 0.3333333333333333703),
 ( 0.3333333333333333703, 0.3333333333333333703, 0.3333333333333333703, 0.3333333333333333703, 0.3333333333333333703, 0.3333333333333333703, 0.3333333333333333703, 0.3333333333333333703, 0.3333333333333333703, 0.3333333333333333703, 0.3333333333333333703, 0.3333333333333333703, 0.3333333333333333703, 0.3333333333333333703, 0.3333333333333333703, 0.3333333333333333703, 0.3333333333333333703, 0.3333333333333333703, 0.3333333333333333703, 0.3333333333333333703, 0.3333333333333333703, 0.3333333333333333703, 0.3333333333333333703, 0.3333333333333333703, 0.3333333333333333703, 0.3333333333333333703, 0.3333333333333333703, 0.3333333333333333703, 0.3333333333333333703, 0.3333333333333333703),
 ( 1.000000000000000000, 1.000000000000000000, 1.000000000000000000, 1.000000000000000000, 1.000000000000000000, 1.000000000000000000, 1.000000000000000000, 1.000000000000000000, 1.000000000000000000, 1.000000000000000000, 1.000000000000000000, 1.000000000000000000, 1.000000000000000000, 1.000000000000000000, 1.000000000000000000, 1.000000000000000000, 1.000000000000000000, 1.000000000000000000, 1.000000000000000000, 1.000000000000000000, 1.000000000000000000, 1.000000000000000000, 1.000000000000000000, 1.000000000000000000, 1.000000000000000000, 1.000000000000000000, 1.000000000000000000, 1.000000000000000000, 1.000000000000000000, 1.000000000000000000) ) ) 
 REPRESENTATION_ITEM ( '' )  SURFACE ( )  );
#18788=CARTESIAN_POINT ( 'NONE',  ( 91.82158438592158234, -40.45024623143958564, 16.11829626348418998 ) ) ;
#18791=CARTESIAN_POINT ( 'NONE',  ( 4.995406935893297096, 10.78321810387837232, 67.35176059880234334 ) ) ;
#18792=DIRECTION ( 'NONE',  ( -0.2259624731742164438, 0.000000000000000000, -0.9741360072992845121 ) ) ;
#18793=CARTESIAN_POINT ( 'NONE',  ( 192.4448373802101173, 40.00000000000012790, -20.00000000003928236 ) ) ;
#18796=CARTESIAN_POINT ( 'NONE',  ( 163.1118516004056573, 40.00000000000017764, -12.73709011382432976 ) ) ;
#18797=CARTESIAN_POINT ( 'NONE',  ( -208.1127848780264742, 40.00000000000055422, -55.00245453014380814 ) ) ;
#18799=AXIS2_PLACEMENT_3D ( 'NONE', #16441, #22443, #18568 ) ;
#18802=CARTESIAN_POINT ( 'NONE',  ( -188.6889827002260631, 13.84869468768024703, 47.12918603174951926 ) ) ;
#18803=CARTESIAN_POINT ( 'NONE',  ( -280.0000000000000000, 14.14213562373078581, 14.14213562373108424 ) ) ;
#18804=CARTESIAN_POINT ( 'NONE',  ( -192.1166648175283456, -48.16216898722870354, 14.00295691731075109 ) ) ;
#18805=CARTESIAN_POINT ( 'NONE',  ( -280.0000000000000568, 42.42640687119274645, 14.14213562373118194 ) ) ;
#18807=CARTESIAN_POINT ( 'NONE',  ( -135.8532207217289738, -21.81201906317757633, -21.81201906317793515 ) ) ;
#18808=CARTESIAN_POINT ( 'NONE',  ( -200.0000000000000284, 48.92947633520098805, -14.52307781036565437 ) ) ;
#18809=CARTESIAN_POINT ( 'NONE',  ( 170.2234770963711128, 24.55285855007190321, 0.000000000000000000 ) ) ;
#18810=CARTESIAN_POINT ( 'NONE',  ( 192.4448373802100889, -14.14213562375896061, 14.14213562375865330 ) ) ;
#18811=CARTESIAN_POINT ( 'NONE',  ( -135.8532207217289738, 9.153146818113548022, 40.00000000000002132 ) ) ;
#18813=ORIENTED_EDGE ( 'NONE', *, *, #7511, .T. ) ;
#18814=CARTESIAN_POINT ( 'NONE',  ( -259.2033419157646676, -40.00000000000017053, 9.517827891722212996 ) ) ;
#18816=CARTESIAN_POINT ( 'NONE',  ( 147.2817042152898352, -12.35516179550165283, 29.82799917201307238 ) ) ;
#18817=EDGE_LOOP ( 'NONE', ( #9410, #3720, #5880, #3853 ) ) ;
#18818=ORIENTED_EDGE ( 'NONE', *, *, #25191, .T. ) ;
#18819=CARTESIAN_POINT ( 'NONE',  ( -259.2033419157646676, 30.48217210827734647, 2.449293598294708485E-15 ) ) ;
#18821=CARTESIAN_POINT ( 'NONE',  ( -105.3846709045546106, -20.33574920587810908, 6.705972854941914640 ) ) ;
#18824=CARTESIAN_POINT ( 'NONE',  ( -199.9999999999999432, 14.17215463606722636, -49.28189405767596298 ) ) ;
#18826=CARTESIAN_POINT ( 'NONE',  ( -105.3174603216990590, 5.405945607584760282, -20.76742684539521022 ) ) ;
#18827=CARTESIAN_POINT ( 'NONE',  ( -280.0000000000000000, -14.14213562373118549, 14.14213562373078936 ) ) ;
#18828=CARTESIAN_POINT ( 'NONE',  ( -135.8532207217289738, 6.472252184284096543, 6.472252184284234211 ) ) ;
#18829=CARTESIAN_POINT ( 'NONE',  ( -94.58238812364415082, 20.73544118676234405, 8.588900961346663365 ) ) ;
#18830=CARTESIAN_POINT ( 'NONE',  ( 4.995406935893283773, 40.00000000000017764, -15.24977328854790848 ) ) ;
#18831=CARTESIAN_POINT ( 'NONE',  ( -105.3755690713226727, 15.38646221621771737, 15.38646221621800514 ) ) ;
#18833=CARTESIAN_POINT ( 'NONE',  ( 23.23834162557122696, 13.80856396595914504, 46.85950693575291837 ) ) ;
#18834=CARTESIAN_POINT ( 'NONE',  ( 91.82158438592158234, -12.16597498397761967, -12.16597498397768007 ) ) ;
#18835=EDGE_CURVE ( 'NONE', #13885, #9833, #1442, .T. ) ;
#18836=CARTESIAN_POINT ( 'NONE',  ( -30.26275506840322294, -57.76657404653985139, 1.198031551615709844 ) ) ;
#18838=EDGE_CURVE ( 'NONE', #817, #12121, #11774, .T. ) ;
#18840=CARTESIAN_POINT ( 'NONE',  ( 57.59792236341146321, 40.00000000000004263, -2.435789363418021214 ) ) ;
#18841=CARTESIAN_POINT ( 'NONE',  ( 60.14720761588542075, 31.22869220292431081, -15.75494750901078689 ) ) ;
#18843=CARTESIAN_POINT ( 'NONE',  ( 199.9999999999999432, -14.14213562373096345, -14.14213562373104871 ) ) ;
#18844=CARTESIAN_POINT ( 'NONE',  ( 4.995406935893288214, 15.24977328854832770, 40.00000000000002132 ) ) ;
#18846=CARTESIAN_POINT ( 'NONE',  ( 12.96694272564372952, -44.79869582453225263, 24.77464205076265102 ) ) ;
#18847=CARTESIAN_POINT ( 'NONE',  ( -208.1127848780265026, 55.00245453012668406, 2.449293598294708485E-15 ) ) ;
#18850=CARTESIAN_POINT ( 'NONE',  ( -208.1127848780265026, 10.60833733269537049, 10.60833733269544510 ) ) ;
#18851=CARTESIAN_POINT ( 'NONE',  ( -8.255580677152480007, -13.52904896325719442, 45.52720393890135853 ) ) ;
#18852=CARTESIAN_POINT ( 'NONE',  ( 2.332272417553664212, 14.08759251168236126, -48.72342300851929053 ) ) ;
#18854=CARTESIAN_POINT ( 'NONE',  ( 199.9999999999999432, -14.14213562373115884, 14.14213562373085153 ) ) ;
#18855=CARTESIAN_POINT ( 'NONE',  ( -87.08748155317185535, -21.19318107433443643, 3.397954955125616294 ) ) ;
#18857=CARTESIAN_POINT ( 'NONE',  ( -189.0115661350366167, -17.94954792649329178, 43.33404204260367720 ) ) ;
#18858=CARTESIAN_POINT ( 'NONE',  ( 146.6084372240433993, 24.48358557860307272, 24.48358557860347418 ) ) ;
#18859=CARTESIAN_POINT ( 'NONE',  ( -30.26275506840323359, -1.198031551616339341, 57.76657404653985139 ) ) ;
#18860=CARTESIAN_POINT ( 'NONE',  ( 0.2972598230770011618, 10.13633138497555919, -66.70487387989845729 ) ) ;
#18861=CARTESIAN_POINT ( 'NONE',  ( 91.82158438592158234, 12.16597498397756993, 12.16597498397776356 ) ) ;
#18862=CARTESIAN_POINT ( 'NONE',  ( -197.4153392275520673, 14.14666332909923874, -49.11379398044257982 ) ) ;
#18863=CARTESIAN_POINT ( 'NONE',  ( -162.0762913951020892, 29.48230308784799902, -29.48230308784730980 ) ) ;
#18864=CARTESIAN_POINT ( 'NONE',  ( -56.48582580120559982, 21.81201906317729922, 34.75652343174635917 ) ) ;
#18865=CARTESIAN_POINT ( 'NONE',  ( 130.8568914410475088, -5.949712681206671405, 40.00000000000002132 ) ) ;
#18866=CARTESIAN_POINT ( 'NONE',  ( 163.1118516004056573, 12.73709011382478806, -40.00000000000002132 ) ) ;
#18867=CARTESIAN_POINT ( 'NONE',  ( -105.3755690713226585, 12.89780903124410472, -43.67073346367977393 ) ) ;
#18868=CARTESIAN_POINT ( 'NONE',  ( -103.9663809734196747, 20.15238534367561130, -8.026122150878887140 ) ) ;
#18869=CARTESIAN_POINT ( 'NONE',  ( -259.2033419157646676, -21.55415060305824326, -21.55415060305857367 ) ) ;
#18871=CARTESIAN_POINT ( 'NONE',  ( -188.3065677117184578, 43.00727648871550457, -23.45084385698009655 ) ) ;
#18872=ORIENTED_EDGE ( 'NONE', *, *, #9553, .F. ) ;
#18873=CARTESIAN_POINT ( 'NONE',  ( 57.59792236341147031, 26.56190807104684382, 26.56190807104692553 ) ) ;
#18875=CARTESIAN_POINT ( 'NONE',  ( -100.7734535825088358, -12.25131212657493052, 12.25131212657478130 ) ) ;
#18876=CARTESIAN_POINT ( 'NONE',  ( -4.076660308449255865, -46.97758120990484798, -13.82548859978903266 ) ) ;
#18877=ORIENTED_EDGE ( 'NONE', *, *, #7793, .F. ) ;
#18878=CARTESIAN_POINT ( 'NONE',  ( 7.307793755307403494, -49.33439594495633429, -14.18010697691869026 ) ) ;
#18879=CARTESIAN_POINT ( 'NONE',  ( -200.0000000000000284, -42.45148791631893204, 35.57044988732123159 ) ) ;
#18882=CARTESIAN_POINT ( 'NONE',  ( -114.4364955367328491, -20.29001642038857156, 8.064892380842218600 ) ) ;
#18883=EDGE_CURVE ( 'NONE', #12962, #9216, #14325, .T. ) ;
#18884=CARTESIAN_POINT ( 'NONE',  ( 57.59792236341147031, 37.56421063658187620, 2.449293598294708485E-15 ) ) ;
#18887=CARTESIAN_POINT ( 'NONE',  ( -213.1075012329537230, -37.98287015391257881, 18.58567234101111509 ) ) ;
#18888=CARTESIAN_POINT ( 'NONE',  ( -105.3755690713226727, -8.549198663894545631E-14, 18.24025645688352881 ) ) ;
#18889=CARTESIAN_POINT ( 'NONE',  ( -91.56559293963836410, 39.99999999999994316, 17.32597176626825330 ) ) ;
#18890=CARTESIAN_POINT ( 'NONE',  ( -3.486753633152357867, 47.18604396268668921, -13.85715877881427538 ) ) ;
#18891=CARTESIAN_POINT ( 'NONE',  ( 151.7948205124836534, -6.767089262349000656, -40.00000000000002132 ) ) ;
#18892=CARTESIAN_POINT ( 'NONE',  ( 23.40652632868016170, -23.33303889678506948, -42.84715492600943776 ) ) ;
#18893=CARTESIAN_POINT ( 'NONE',  ( 146.6084372240433993, 24.48358557860341733, -24.48358557860313311 ) ) ;
#18894=CARTESIAN_POINT ( 'NONE',  ( 151.7948205124836250, -6.767089262349004208, -2.449293598294708485E-15 ) ) ;
#18895=CARTESIAN_POINT ( 'NONE',  ( -192.9588430854689705, -38.51493924976963967, 38.51493924976919914 ) ) ;
#18896=CARTESIAN_POINT ( 'NONE',  ( 154.0339099654740949, -11.67508747798869528, -28.18615453125294223 ) ) ;
#18898=CARTESIAN_POINT ( 'NONE',  ( -213.1075012329537230, 40.00000000000055422, -53.71589010953623244 ) ) ;
#18899=CARTESIAN_POINT ( 'NONE',  ( 0.2972598230769956662, 39.99999999999983658, 54.33493731733950938 ) ) ;
#18901=CARTESIAN_POINT ( 'NONE',  ( -114.4364955367327497, -8.064892380842218600, -20.29001642038850406 ) ) ;
#18902=CARTESIAN_POINT ( 'NONE',  ( -114.7827960788991248, -16.12461489702645423, 15.17504536827576977 ) ) ;
#18903=CARTESIAN_POINT ( 'NONE',  ( 57.59792236341147031, -26.56190807104670171, -30.00663442387710234 ) ) ;
#18906=CARTESIAN_POINT ( 'NONE',  ( -24.88648382766318790, 39.69105101984397521, -12.31763033301884391 ) ) ;
#18907=CARTESIAN_POINT ( 'NONE',  ( 155.1206158682453804, 27.79897307351031088, -11.51471166709240634 ) ) ;
#18908=CARTESIAN_POINT ( 'NONE',  ( 57.59792236341148453, -37.56421063658185489, -40.00000000000002132 ) ) ;
#18909=CARTESIAN_POINT ( 'NONE',  ( -86.86493150571118349, -7.943527260495776510, -19.77569912839190280 ) ) ;
#18911=ORIENTED_EDGE ( 'NONE', *, *, #24699, .T. ) ;
#18914=FACE_OUTER_BOUND ( 'NONE', #14716, .T. ) ;
#18916=ADVANCED_FACE ( 'NONE', ( #21461 ), #9599, .T. ) ;
#18918=CARTESIAN_POINT ( 'NONE',  ( 163.1118516004056573, -19.27778845538761132, -19.27778845538770724 ) ) ;
#18920=CARTESIAN_POINT ( 'NONE',  ( -114.4364955367334318, -8.064892380823156515, 20.29001642039686004 ) ) ;
#18922=CARTESIAN_POINT ( 'NONE',  ( -100.7734535825088500, -44.31723036834903695, 12.25131212657476709 ) ) ;
#18923=CARTESIAN_POINT ( 'NONE',  ( -198.0356074513804572, 10.87444709759714989, 10.87444709759722450 ) ) ;
#18924=CARTESIAN_POINT ( 'NONE',  ( 14.38125909742180220, 39.99999999999997158, 15.17850393972647716 ) ) ;
#18927=EDGE_CURVE ( 'NONE', #12165, #12795, #2896, .T. ) ;
#18928=CARTESIAN_POINT ( 'NONE',  ( -105.4741150117382062, 7.943527260750565588, -19.77569912955109288 ) ) ;
#18929=CARTESIAN_POINT ( 'NONE',  ( 4.995406935893298872, 5.820775922023080204E-13, -55.24977328854835434 ) ) ;
#18930=CARTESIAN_POINT ( 'NONE',  ( -162.0762913951021176, 40.00000000000001421, -1.694272876827905394 ) ) ;
#18931=CARTESIAN_POINT ( 'NONE',  ( -87.10188448154612217, 17.05386097136903700, 13.04993700312317628 ) ) ;
#18934=CARTESIAN_POINT ( 'NONE',  ( -188.8531444083250790, 17.93248118558191706, 43.29283928523306457 ) ) ;
#18935=CARTESIAN_POINT ( 'NONE',  ( 130.8568914410475088, -4.207082182990058428, 52.36146031193416661 ) ) ;
#18936=CARTESIAN_POINT ( 'NONE',  ( -88.39148973765269091, 8.577159256668403842, 19.92926839984458098 ) ) ;
#18937=CARTESIAN_POINT ( 'NONE',  ( -280.0000000000000568, 14.14213562373067745, 42.42640687119295251 ) ) ;
#18938=CARTESIAN_POINT ( 'NONE',  ( -77.55632011645045054, -15.16702236933177517, 16.13210123264064322 ) ) ;
#18939=CIRCLE ( 'NONE', #5742, 14.99999999999999822 ) ;
#18941=CARTESIAN_POINT ( 'NONE',  ( 91.82158438592159655, 12.16597498400091304, -44.40256751092321963 ) ) ;
#18943=CARTESIAN_POINT ( 'NONE',  ( -238.4067589809705794, -0.9644942799826262680, 0.000000000000000000 ) ) ;
#18944=CARTESIAN_POINT ( 'NONE',  ( -135.8532207217289738, 21.81201906317729566, 34.75652343174635917 ) ) ;
#18945=CARTESIAN_POINT ( 'NONE',  ( -259.2033419157646676, 9.517827891722582478, 40.00000000000002132 ) ) ;
#18946=( BOUNDED_SURFACE ( )  B_SPLINE_SURFACE ( 3, 3, ( 
 ( #19297, #21553, #23797, #19425, #17171, #13307, #25304, #3454, #21426, #1080, #7559, #15671, #17302, #9189, #15178, #23303, #5081, #25561, #25434, #7181, #23426, #3198, #5203, #1211, #23549, #3327, #13808, #15933, #6107, #26221 ),
 ( #5702, #3718, #10229, #5842, #17935, #4128, #24475, #14215, #1860, #18338, #12222, #7689, #22350, #9695, #17802, #4258, #13946, #11820, #21942, #120, #7957, #15802, #20344, #22081, #24066, #26351, #16075, #22215, #18198, #3854 ),
 ( #8225, #2121, #9964, #8092, #24343, #23927, #11957, #19938, #16343, #6237, #24203, #1723, #14351, #26082, #18070, #9831, #22479, #12348, #25948, #7817, #1594, #20082, #20212, #16212, #5976, #14084, #3991, #1990, #12090, #10096 ),
 ( #10763, #8894, #12754, #20607, #14874, #6762, #14479, #24872, #655, #8762, #18875, #2250, #4651, #24606, #23141, #17005, #16480, #20477, #6627, #10631, #6360, #20878, #23014, #2516, #2658, #16877, #25009, #19012, #22738, #790 ),
 ( #4787, #18607, #22612, #12891, #16608, #21005, #2787, #25142, #10900, #6893, #523, #4388, #4521, #15008, #14744, #18469, #4912, #10359, #386, #18742, #250, #8359, #12480, #2382, #8495, #10494, #24741, #6496, #14607, #12619 ),
 ( #20747, #8628, #16739, #22874, #13024, #7018, #21144, #2918, #11026, #17135, #920, #9031, #19136, #25268, #15139, #23269, #15973, #7852, #10490, #18465, #6355, #2377, #26113, #20742, #17966, #3891, #15832, #16735, #22870, #14474 ),
 ( #23962, #8488, #16603, #242, #5737, #2511, #9864, #11991, #25981, #22733, #24867, #9732, #13842, #519, #14739, #4383, #18603, #24099, #5874, #9996, #12475, #21976, #8624, #20602, #382, #13981, #3748, #11854, #22114, #24736 ) ),
 .UNSPECIFIED., .T., .F., .T. ) 
 B_SPLINE_SURFACE_WITH_KNOTS ( ( 4, 3, 4 ),
 ( 4, 2, 2, 2, 2, 2, 2, 2, 2, 2, 2, 2, 2, 2, 4 ),
 ( 0.000000000000000000, 0.5000000000000000000, 1.000000000000000000 ),
 ( 0.000000000000000000, 0.1357259735107005372, 0.1651108541090157700, 0.1944957347073310028, 0.3598804999793158710, 0.3867117631979620773, 0.4135430264166082281, 0.5789277916885930964, 0.6062785021374117456, 0.6336292125862302838, 0.8508620842112317728, 0.8814014469398914198, 0.9119408096685510667, 0.9559704048342755334, 1.000000000000000000 ),
 .UNSPECIFIED. ) 
 GEOMETRIC_REPRESENTATION_ITEM ( )  RATIONAL_B_SPLINE_SURFACE ( (
 ( 1.000000000000000000, 1.000000000000000000, 1.000000000000000000, 1.000000000000000000, 1.000000000000000000, 1.000000000000000000, 1.000000000000000000, 1.000000000000000000, 1.000000000000000000, 1.000000000000000000, 1.000000000000000000, 1.000000000000000000, 1.000000000000000000, 1.000000000000000000, 1.000000000000000000, 1.000000000000000000, 1.000000000000000000, 1.000000000000000000, 1.000000000000000000, 1.000000000000000000, 1.000000000000000000, 1.000000000000000000, 1.000000000000000000, 1.000000000000000000, 1.000000000000000000, 1.000000000000000000, 1.000000000000000000, 1.000000000000000000, 1.000000000000000000, 1.000000000000000000),
 ( 0.3333333333333333703, 0.3333333333333333703, 0.3333333333333333703, 0.3333333333333333703, 0.3333333333333333703, 0.3333333333333333703, 0.3333333333333333703, 0.3333333333333333703, 0.3333333333333333703, 0.3333333333333333703, 0.3333333333333333703, 0.3333333333333333703, 0.3333333333333333703, 0.3333333333333333703, 0.3333333333333333703, 0.3333333333333333703, 0.3333333333333333703, 0.3333333333333333703, 0.3333333333333333703, 0.3333333333333333703, 0.3333333333333333703, 0.3333333333333333703, 0.3333333333333333703, 0.3333333333333333703, 0.3333333333333333703, 0.3333333333333333703, 0.3333333333333333703, 0.3333333333333333703, 0.3333333333333333703, 0.3333333333333333703),
 ( 0.3333333333333333703, 0.3333333333333333703, 0.3333333333333333703, 0.3333333333333333703, 0.3333333333333333703, 0.3333333333333333703, 0.3333333333333333703, 0.3333333333333333703, 0.3333333333333333703, 0.3333333333333333703, 0.3333333333333333703, 0.3333333333333333703, 0.3333333333333333703, 0.3333333333333333703, 0.3333333333333333703, 0.3333333333333333703, 0.3333333333333333703, 0.3333333333333333703, 0.3333333333333333703, 0.3333333333333333703, 0.3333333333333333703, 0.3333333333333333703, 0.3333333333333333703, 0.3333333333333333703, 0.3333333333333333703, 0.3333333333333333703, 0.3333333333333333703, 0.3333333333333333703, 0.3333333333333333703, 0.3333333333333333703),
 ( 1.000000000000000000, 1.000000000000000000, 1.000000000000000000, 1.000000000000000000, 1.000000000000000000, 1.000000000000000000, 1.000000000000000000, 1.000000000000000000, 1.000000000000000000, 1.000000000000000000, 1.000000000000000000, 1.000000000000000000, 1.000000000000000000, 1.000000000000000000, 1.000000000000000000, 1.000000000000000000, 1.000000000000000000, 1.000000000000000000, 1.000000000000000000, 1.000000000000000000, 1.000000000000000000, 1.000000000000000000, 1.000000000000000000, 1.000000000000000000, 1.000000000000000000, 1.000000000000000000, 1.000000000000000000, 1.000000000000000000, 1.000000000000000000, 1.000000000000000000),
 ( 0.3333333333333333703, 0.3333333333333333703, 0.3333333333333333703, 0.3333333333333333703, 0.3333333333333333703, 0.3333333333333333703, 0.3333333333333333703, 0.3333333333333333703, 0.3333333333333333703, 0.3333333333333333703, 0.3333333333333333703, 0.3333333333333333703, 0.3333333333333333703, 0.3333333333333333703, 0.3333333333333333703, 0.3333333333333333703, 0.3333333333333333703, 0.3333333333333333703, 0.3333333333333333703, 0.3333333333333333703, 0.3333333333333333703, 0.3333333333333333703, 0.3333333333333333703, 0.3333333333333333703, 0.3333333333333333703, 0.3333333333333333703, 0.3333333333333333703, 0.3333333333333333703, 0.3333333333333333703, 0.3333333333333333703),
 ( 0.3333333333333333703, 0.3333333333333333703, 0.3333333333333333703, 0.3333333333333333703, 0.3333333333333333703, 0.3333333333333333703, 0.3333333333333333703, 0.3333333333333333703, 0.3333333333333333703, 0.3333333333333333703, 0.3333333333333333703, 0.3333333333333333703, 0.3333333333333333703, 0.3333333333333333703, 0.3333333333333333703, 0.3333333333333333703, 0.3333333333333333703, 0.3333333333333333703, 0.3333333333333333703, 0.3333333333333333703, 0.3333333333333333703, 0.3333333333333333703, 0.3333333333333333703, 0.3333333333333333703, 0.3333333333333333703, 0.3333333333333333703, 0.3333333333333333703, 0.3333333333333333703, 0.3333333333333333703, 0.3333333333333333703),
 ( 1.000000000000000000, 1.000000000000000000, 1.000000000000000000, 1.000000000000000000, 1.000000000000000000, 1.000000000000000000, 1.000000000000000000, 1.000000000000000000, 1.000000000000000000, 1.000000000000000000, 1.000000000000000000, 1.000000000000000000, 1.000000000000000000, 1.000000000000000000, 1.000000000000000000, 1.000000000000000000, 1.000000000000000000, 1.000000000000000000, 1.000000000000000000, 1.000000000000000000, 1.000000000000000000, 1.000000000000000000, 1.000000000000000000, 1.000000000000000000, 1.000000000000000000, 1.000000000000000000, 1.000000000000000000, 1.000000000000000000, 1.000000000000000000, 1.000000000000000000) ) ) 
 REPRESENTATION_ITEM ( '' )  SURFACE ( )  );
#18948=EDGE_LOOP ( 'NONE', ( #8673, #19547, #14684, #13544, #13580, #23796 ) ) ;
#18949=CARTESIAN_POINT ( 'NONE',  ( -105.3755690713226727, 1.741486606973311632E-13, -18.24025645688352881 ) ) ;
#18951=CARTESIAN_POINT ( 'NONE',  ( 121.8740240556052612, -11.10671848392298777, 26.81399039734603207 ) ) ;
#18952=ORIENTED_EDGE ( 'NONE', *, *, #7511, .F. ) ;
#18955=CARTESIAN_POINT ( 'NONE',  ( 14.38125909742180752, 55.17850393974265444, 40.00000000000002132 ) ) ;
#18957=CARTESIAN_POINT ( 'NONE',  ( -102.4309680866992238, -20.17061239832209196, -8.733065090195987423 ) ) ;
#18959=CARTESIAN_POINT ( 'NONE',  ( -110.0563856373316440, -19.19543633473033850, -6.246938629539779519 ) ) ;
#18961=CARTESIAN_POINT ( 'NONE',  ( -213.1075012329537230, -8.703598725189323045E-14, 13.71589010951911902 ) ) ;
#18963=CONICAL_SURFACE ( 'NONE', #1133, 30.00000000000003908, 0.7853981633974531640 ) ;
#18964=CARTESIAN_POINT ( 'NONE',  ( 170.0000000000000284, -3.062538285713274799, 24.95097643316997704 ) ) ;
#18965=CARTESIAN_POINT ( 'NONE',  ( -208.1127848780265026, 10.60833733269551615, -10.60833733269529766 ) ) ;
#18968=CARTESIAN_POINT ( 'NONE',  ( -56.48582580120559982, 40.00000000000034106, -30.84685318188602210 ) ) ;
#18969=CARTESIAN_POINT ( 'NONE',  ( -103.9474983245001312, -8.027156558344865189, 20.15710290851540520 ) ) ;
#18970=CARTESIAN_POINT ( 'NONE',  ( -208.1127848780265026, -15.00245453012673202, 0.000000000000000000 ) ) ;
#18971=CARTESIAN_POINT ( 'NONE',  ( 200.0000000000000000, -42.42640687119269671, -14.14213562373124766 ) ) ;
#18972=CARTESIAN_POINT ( 'NONE',  ( -162.0762913951020892, -1.694272876828353702, 0.000000000000000000 ) ) ;
#18974=CARTESIAN_POINT ( 'NONE',  ( -238.4067589809705794, 39.99999999999997158, 0.9644942799827220803 ) ) ;
#18977=CARTESIAN_POINT ( 'NONE',  ( 0.2972598230770011618, 10.13633138497462305, 66.70487387989858519 ) ) ;
#18978=CARTESIAN_POINT ( 'NONE',  ( 200.0000000000000000, -20.00000000000006750, 40.00000000000002132 ) ) ;
#18980=CARTESIAN_POINT ( 'NONE',  ( 9.006212071528537422, -44.90541342374581291, 24.85331907608552271 ) ) ;
#18981=CARTESIAN_POINT ( 'NONE',  ( 200.0000000000000000, 19.99999999999996447, -40.00000000000002132 ) ) ;
#18982=CONICAL_SURFACE ( 'NONE', #25777, 30.00000000000003908, 0.7853981633974531640 ) ;
#18985=CARTESIAN_POINT ( 'NONE',  ( -100.7734535825088500, -44.31723036834903695, 12.25131212657476709 ) ) ;
#18986=CARTESIAN_POINT ( 'NONE',  ( -70.30307074921901744, -10.20829450076744394, 22.52851052539943666 ) ) ;
#18988=CARTESIAN_POINT ( 'NONE',  ( -47.45115950041520136, 10.57586762663035707, -31.57405104335990487 ) ) ;
#18991=CARTESIAN_POINT ( 'NONE',  ( -162.0762913951020892, 1.198031840385732849, -1.198031840385733515 ) ) ;
#18992=CARTESIAN_POINT ( 'NONE',  ( -87.13361725324693907, -21.49321519332800889, 0.6800178180920880555 ) ) ;
#18993=CARTESIAN_POINT ( 'NONE',  ( 136.1360204305621266, -35.03383547441293899, 0.000000000000000000 ) ) ;
#18994=CARTESIAN_POINT ( 'NONE',  ( -195.1685814578020484, -24.52825302093954107, 44.46431112710764211 ) ) ;
#18996=CARTESIAN_POINT ( 'NONE',  ( -192.9588430854689989, -10.23066800230756890, 10.23066800230742501 ) ) ;
#18997=CARTESIAN_POINT ( 'NONE',  ( -198.0356074513804572, 10.87444709759730088, -10.87444709759707173 ) ) ;
#18999=CARTESIAN_POINT ( 'NONE',  ( -259.2033419157646676, 6.730120644403426944, 6.730120644403592145 ) ) ;
#19000=CARTESIAN_POINT ( 'NONE',  ( -91.56559293963834989, 12.25131212657497848, -12.25131212657469426 ) ) ;
#19001=CARTESIAN_POINT ( 'NONE',  ( -91.56559293963834989, 12.25131212657497848, -12.25131212657469426 ) ) ;
#19002=CARTESIAN_POINT ( 'NONE',  ( -100.7734535825088500, 22.67402823373189591, -0.000000000000000000 ) ) ;
#19003=CARTESIAN_POINT ( 'NONE',  ( 91.82158438592158234, -17.20528682183298486, -40.00000000000002132 ) ) ;
#19004=CARTESIAN_POINT ( 'NONE',  ( -280.0000000000000568, 14.14213562373097943, -42.42640687119285303 ) ) ;
#19007=CARTESIAN_POINT ( 'NONE',  ( -259.2033419157646676, -21.55415060305872998, 35.01439189186525880 ) ) ;
#19008=DIRECTION ( 'NONE',  ( 1.000000000000000000, 0.000000000000000000, 0.000000000000000000 ) ) ;
#19010=CARTESIAN_POINT ( 'NONE',  ( 91.82158438592158234, -12.16597498400057198, 44.40256751092329779 ) ) ;
#19011=FACE_OUTER_BOUND ( 'NONE', #12656, .T. ) ;
#19012=CARTESIAN_POINT ( 'NONE',  ( 184.8905102610680444, -13.49065550809810965, 13.49065550809799596 ) ) ;
#19013=CARTESIAN_POINT ( 'NONE',  ( 13.28449813601913654, -44.77439867187360534, -24.75673736220152676 ) ) ;
#19014=VERTEX_POINT ( 'NONE', #11791 ) ;
#19015=CARTESIAN_POINT ( 'NONE',  ( -184.9729924864174677, -45.83719276899095263, 13.59277144555537298 ) ) ;
#19016=CARTESIAN_POINT ( 'NONE',  ( -110.1017833366007892, -13.38816311907946144, -15.17212531755836125 ) ) ;
#19018=CARTESIAN_POINT ( 'NONE',  ( -200.0000000000000000, 60.00000000000011369, 0.000000000000000000 ) ) ;
#19019=CARTESIAN_POINT ( 'NONE',  ( -91.56559293963834989, 17.32597176626809699, -40.00000000000002132 ) ) ;
#19022=CARTESIAN_POINT ( 'NONE',  ( 163.1118516004056573, -9.006482792074626431, 47.56205970284951690 ) ) ;
#19023=CARTESIAN_POINT ( 'NONE',  ( -91.56559293963834989, -40.00000000000009948, 17.32597176626796553 ) ) ;
#19024=CARTESIAN_POINT ( 'NONE',  ( -208.1127848780264742, 39.99999999999992895, 15.00245453012683683 ) ) ;
#19026=CARTESIAN_POINT ( 'NONE',  ( 57.59792236341148453, -37.56421063658185489, -2.449293598294708485E-15 ) ) ;
#19027=CARTESIAN_POINT ( 'NONE',  ( 22.89778847645061788, -17.86913359794365874, -43.13990468001261291 ) ) ;
#19029=CARTESIAN_POINT ( 'NONE',  ( -162.0762913951020892, -41.69427287672991866, -40.00000000000002132 ) ) ;
#19030=CARTESIAN_POINT ( 'NONE',  ( -86.96347745069645896, 43.67073346367970288, 12.89780903124427702 ) ) ;
#19031=CARTESIAN_POINT ( 'NONE',  ( 153.3020327024398455, -11.77299484472929159, -28.42252382389425946 ) ) ;
#19032=CARTESIAN_POINT ( 'NONE',  ( -114.7755410848721880, 16.60116338994188467, -14.64251757340711357 ) ) ;
#19033=CARTESIAN_POINT ( 'NONE',  ( -208.1127848780264742, -39.99999999999948841, -55.00245453010965235 ) ) ;
#19034=CARTESIAN_POINT ( 'NONE',  ( 192.4448373802101173, 14.14213562370320076, -42.42640687122072762 ) ) ;
#19036=CARTESIAN_POINT ( 'NONE',  ( -103.9474983244996196, -8.577167319634884990, -19.92928099173804668 ) ) ;
#19037=CARTESIAN_POINT ( 'NONE',  ( -259.2033419157646676, 35.01439189186528722, 21.55415060305857011 ) ) ;
#19038=EDGE_LOOP ( 'NONE', ( #26220, #12191, #17002, #9350, #13918, #4126, #12928 ) ) ;
#19039=CARTESIAN_POINT ( 'NONE',  ( -77.72892396114323788, -5.803299710953224277, -21.20265378149535351 ) ) ;
#19040=CARTESIAN_POINT ( 'NONE',  ( -77.90255099906771363, 20.04994828523961203, -8.644468104261394004 ) ) ;
#19041=CARTESIAN_POINT ( 'NONE',  ( 118.9130007099546305, 25.80693111732296074, -10.68958087202326723 ) ) ;
#19042=CARTESIAN_POINT ( 'NONE',  ( 200.0000000000000000, 20.00000000000013856, -40.00000000000002132 ) ) ;
#19044=CARTESIAN_POINT ( 'NONE',  ( -194.4222775681010376, 48.65439176090173135, -14.07715774766184502 ) ) ;
#19049=ORIENTED_EDGE ( 'NONE', *, *, #14014, .F. ) ;
#19050=CARTESIAN_POINT ( 'NONE',  ( 184.8905102610680444, -43.07788698682576722, 13.49065550809799063 ) ) ;
#19053=CARTESIAN_POINT ( 'NONE',  ( -105.3755690713226585, -43.67073346367983788, 12.89780903124397149 ) ) ;
#19055=CARTESIAN_POINT ( 'NONE',  ( 19.06497207195980792, 39.99999999999983658, 54.19242893257857929 ) ) ;
#19057=CARTESIAN_POINT ( 'NONE',  ( -199.9999999999999147, -14.17215463606694925, 49.28189405767609088 ) ) ;
#19058=CARTESIAN_POINT ( 'NONE',  ( 91.82158438592159655, -39.99999999999976552, -22.79471317813512599 ) ) ;
#19059=CARTESIAN_POINT ( 'NONE',  ( 184.8905102610680444, 39.99999999999983658, 20.92133201514485563 ) ) ;
#19061=CARTESIAN_POINT ( 'NONE',  ( -86.95492405012092263, 9.645501174397823618, 19.11844758104726694 ) ) ;
#19063=CARTESIAN_POINT ( 'NONE',  ( -91.56559293963836410, 16.03295912088714203, -16.03295912088699282 ) ) ;
#19064=CARTESIAN_POINT ( 'NONE',  ( 192.4448373802101173, -42.42640687116510634, 14.14213562375845257 ) ) ;
#19066=CARTESIAN_POINT ( 'NONE',  ( -189.2428547182112197, -47.31876910929170776, 13.87687415872445662 ) ) ;
#19067=CARTESIAN_POINT ( 'NONE',  ( 151.7948205124836534, 23.49921654116009506, 33.06932595376371609 ) ) ;
#19068=FACE_OUTER_BOUND ( 'NONE', #8630, .T. ) ;
#19069=CARTESIAN_POINT ( 'NONE',  ( 91.82158438592156813, 40.45024623143973486, -16.11829626348390931 ) ) ;
#19070=LINE ( 'NONE', #25072, #22747 ) ;
#19071=CARTESIAN_POINT ( 'NONE',  ( 192.4448373802100889, 20.00000000003945644, 0.000000000000000000 ) ) ;
#19073=CARTESIAN_POINT ( 'NONE',  ( -86.96347745069644475, 41.18208027870576871, 15.38646221621837107 ) ) ;
#19075=CARTESIAN_POINT ( 'NONE',  ( 130.8568914410475088, 34.05028731879790627, 40.00000000000002132 ) ) ;
#19077=VERTEX_POINT ( 'NONE', #24170 ) ;
#19078=CARTESIAN_POINT ( 'NONE',  ( -213.1075012329537230, -39.99999999999948841, -53.71589010950208376 ) ) ;
#19082=CARTESIAN_POINT ( 'NONE',  ( 144.1620285550791039, -12.51613133675892975, 30.21661402164544441 ) ) ;
#19083=ORIENTED_EDGE ( 'NONE', *, *, #1189, .T. ) ;
#19086=CARTESIAN_POINT ( 'NONE',  ( -86.96347745069644475, 18.24025645688351105, 2.449293598294708485E-15 ) ) ;
#19088=AXIS2_PLACEMENT_3D ( 'NONE', #9361, #1518, #1648 ) ;
#19090=CARTESIAN_POINT ( 'NONE',  ( 169.9999999999674571, -17.64300463372919836, -17.64300463252165585 ) ) ;
#19091=CARTESIAN_POINT ( 'NONE',  ( -91.56559293963834989, 6.234561990864368500E-14, -22.67402823373191723 ) ) ;
#19094=CARTESIAN_POINT ( 'NONE',  ( -86.96347745069644475, -43.67073346367964604, -12.89780903124457545 ) ) ;
#19095=CARTESIAN_POINT ( 'NONE',  ( 14.38125909742181285, -10.73282306404712472, -10.73282306404731301 ) ) ;
#19096=CARTESIAN_POINT ( 'NONE',  ( -91.56559293963834989, 1.671088883502053755E-13, -17.32597176626811120 ) ) ;
#19098=DIRECTION ( 'NONE',  ( 0.000000000000000000, -0.3995982397413241904, 0.9166903767334068087 ) ) ;
#19099=CARTESIAN_POINT ( 'NONE',  ( -105.3755690713226585, 15.38646221621762678, 41.18208027870604582 ) ) ;
#19100=CARTESIAN_POINT ( 'NONE',  ( -238.4067589809705794, -0.9644942799826262680, 0.000000000000000000 ) ) ;
#19102=CARTESIAN_POINT ( 'NONE',  ( 19.06497207195979726, 39.99999999999997158, 14.19242893257854554 ) ) ;
#19104=CARTESIAN_POINT ( 'NONE',  ( -213.1075012329537230, -18.58567234101155208, 37.98287015391234434 ) ) ;
#19105=CARTESIAN_POINT ( 'NONE',  ( 170.2234770963711128, -24.55285855007183926, 0.000000000000000000 ) ) ;
#19107=CARTESIAN_POINT ( 'NONE',  ( 17.65190073994094533, -44.23515346912825663, 24.35922420890246087 ) ) ;
#19108=CARTESIAN_POINT ( 'NONE',  ( -86.96347745069644475, 18.24025645688350750, -40.00000000000002132 ) ) ;
#19111=CARTESIAN_POINT ( 'NONE',  ( 163.1118516004056573, -47.56205970284957374, 9.006482792074162802 ) ) ;
#19112=CARTESIAN_POINT ( 'NONE',  ( -91.56559293963834989, -39.99999999999995737, -22.67402823373205933 ) ) ;
#19113=CARTESIAN_POINT ( 'NONE',  ( -82.29166192294638904, 18.99061817120102802, -6.834568285704429869 ) ) ;
#19114=CARTESIAN_POINT ( 'NONE',  ( -24.53392603775095537, 19.42583462371737113, -36.88304647106937750 ) ) ;
#19116=CARTESIAN_POINT ( 'NONE',  ( -91.56559293963834989, 12.25131212657428748, 44.31723036834913643 ) ) ;
#19117=CARTESIAN_POINT ( 'NONE',  ( -82.23726319238257076, -20.19517362728035437, 0.6309363043619388156 ) ) ;
#19118=CARTESIAN_POINT ( 'NONE',  ( -77.90255099906863734, -20.04994828524331396, -8.644468104250957907 ) ) ;
#19119=CARTESIAN_POINT ( 'NONE',  ( -200.5022929845067381, -18.58571294254484840, 44.86988025226722243 ) ) ;
#19120=CARTESIAN_POINT ( 'NONE',  ( 91.82158438592158234, 12.16597498397756993, 12.16597498397776356 ) ) ;
#19121=AXIS2_PLACEMENT_3D ( 'NONE', #20639, #17036, #12922 ) ;
#19122=CARTESIAN_POINT ( 'NONE',  ( -259.2033419157646676, 6.730120644403521979, -6.730120644403498886 ) ) ;
#19123=DIRECTION ( 'NONE',  ( 0.000000000000000000, -0.9307566067079452443, 0.3656393565653338062 ) ) ;
#19125=CARTESIAN_POINT ( 'NONE',  ( -135.8532207217289738, 34.75652343174625258, -21.81201906317744132 ) ) ;
#19126=CARTESIAN_POINT ( 'NONE',  ( -238.4067589809705794, 57.25054294065799354, -0.6820004457334954973 ) ) ;
#19127=CARTESIAN_POINT ( 'NONE',  ( -238.4067589809705794, 28.96627169325354956, -28.96627169325289231 ) ) ;
#19128=CARTESIAN_POINT ( 'NONE',  ( -91.56559293963834989, 17.32597176626809699, -40.00000000000002132 ) ) ;
#19129=CARTESIAN_POINT ( 'NONE',  ( 192.4448373802101173, 42.42640687116508502, -14.14213562375874567 ) ) ;
#19131=CARTESIAN_POINT ( 'NONE',  ( 14.38125909742183062, -67.30136555895943218, -10.73282306403629605 ) ) ;
#19132=CARTESIAN_POINT ( 'NONE',  ( -188.3120147333544310, 43.00887716025408025, -23.45203116714288427 ) ) ;
#19133=ORIENTED_EDGE ( 'NONE', *, *, #25271, .F. ) ;
#19134=CARTESIAN_POINT ( 'NONE',  ( -198.0356074513804572, 10.87444709758468875, 67.44298959250869530 ) ) ;
#19136=CARTESIAN_POINT ( 'NONE',  ( -86.96347745069645896, 43.67073346367970288, 12.89780903124427702 ) ) ;
#19137=CARTESIAN_POINT ( 'NONE',  ( 98.29820294267362613, -18.95183585406276094, -6.423630604794682064 ) ) ;
#19139=CARTESIAN_POINT ( 'NONE',  ( -188.2870673237729306, -43.00153493964099738, 23.44688076656430198 ) ) ;
#19142=CARTESIAN_POINT ( 'NONE',  ( 45.01779936581511521, -18.90344565813661859, 36.09695843556287542 ) ) ;
#19143=CARTESIAN_POINT ( 'NONE',  ( -56.48582580120559982, -9.153146818113595984, -40.00000000000002132 ) ) ;
#19144=CARTESIAN_POINT ( 'NONE',  ( 67.78092418456155599, 12.11998378897419570, -29.26022923856843860 ) ) ;
#19146=CARTESIAN_POINT ( 'NONE',  ( 130.8568914410475088, -32.49135343045495006, 24.07718906446878648 ) ) ;
#19147=CARTESIAN_POINT ( 'NONE',  ( 14.38125909742181818, -1.924622159709266762E-13, 55.17850393972636880 ) ) ;
#19148=CARTESIAN_POINT ( 'NONE',  ( 14.38125909742181108, -5.035366881890652543E-14, 15.17850393972633682 ) ) ;
#19149=CARTESIAN_POINT ( 'NONE',  ( 192.4448373802100889, 1.051811698935164031E-13, -20.00000000003942091 ) ) ;
#19150=CARTESIAN_POINT ( 'NONE',  ( 151.7948205124835681, 33.23291073765556547, -40.00000000000002132 ) ) ;
#19151=CARTESIAN_POINT ( 'NONE',  ( 23.49666234703796519, -13.79192166426271626, -46.76389514419435756 ) ) ;
#19153=CARTESIAN_POINT ( 'NONE',  ( -105.3755690713226869, 21.75974354311648540, -0.000000000000000000 ) ) ;
#19155=CARTESIAN_POINT ( 'NONE',  ( -91.56559293963836410, 44.31723036834890905, 12.25131212657507795 ) ) ;
#19156=CARTESIAN_POINT ( 'NONE',  ( 0.2972598230769883387, 40.00000000000017053, -14.33493731733891607 ) ) ;
#19158=CARTESIAN_POINT ( 'NONE',  ( 0.2972598230770030492, -39.99999999999987210, -14.33493731733975451 ) ) ;
#19160=CARTESIAN_POINT ( 'NONE',  ( 147.2811880046590147, -29.82808195031421405, -12.35519608339632214 ) ) ;
#19162=CARTESIAN_POINT ( 'NONE',  ( 19.06497207195980792, 18.24870850772737185, 38.31983398719634692 ) ) ;
#19164=ORIENTED_EDGE ( 'NONE', *, *, #15559, .F. ) ;
#19165=CARTESIAN_POINT ( 'NONE',  ( -77.90255099906767100, 8.064892378658102601, -20.29001641120677846 ) ) ;
#19166=CARTESIAN_POINT ( 'NONE',  ( -198.0012279374158481, 24.77357825033897498, -44.79720170867052786 ) ) ;
#19168=CARTESIAN_POINT ( 'NONE',  ( -105.3755690713226585, 21.75974354311648185, 40.00000000000002132 ) ) ;
#19169=EDGE_CURVE ( 'NONE', #14253, #11184, #17085, .T. ) ;
#19171=CARTESIAN_POINT ( 'NONE',  ( -192.1963514251034724, 48.17613439255902108, -14.00508311691898733 ) ) ;
#19173=ORIENTED_EDGE ( 'NONE', *, *, #26237, .T. ) ;
#19174=ORIENTED_EDGE ( 'NONE', *, *, #3298, .F. ) ;
#19175=CARTESIAN_POINT ( 'NONE',  ( 73.43468551893278118, -9.843145830824733267, 28.18272074650135295 ) ) ;
#19176=CARTESIAN_POINT ( 'NONE',  ( -200.0000000000000000, 1.308061781956697717E-29, 0.000000000000000000 ) ) ;
#19177=CARTESIAN_POINT ( 'NONE',  ( 98.29820294267527458, 2.689882573189819553E-13, -20.00000000000500222 ) ) ;
#19178=ORIENTED_EDGE ( 'NONE', *, *, #12164, .F. ) ;
#19181=CARTESIAN_POINT ( 'NONE',  ( -114.6821015619662489, -4.467609313239589319, 21.58745106896960664 ) ) ;
#19182=CARTESIAN_POINT ( 'NONE',  ( 151.7948205124836250, -23.49921654116339553, -23.49921654116350211 ) ) ;
#19185=CARTESIAN_POINT ( 'NONE',  ( 130.8568914410475088, 40.00000000000002842, 5.949712681206834830 ) ) ;
#19187=DIRECTION ( 'NONE',  ( 1.000000000000000000, 1.836970198721030181E-16, 0.000000000000000000 ) ) ;
#19188=CARTESIAN_POINT ( 'NONE',  ( 151.7948205124836534, -39.99999999999992184, -6.767089262349454515 ) ) ;
#19189=CARTESIAN_POINT ( 'NONE',  ( -100.7734535825088358, 1.654174317907124744E-13, -17.32597176626811120 ) ) ;
#19190=CARTESIAN_POINT ( 'NONE',  ( -77.62095083827057351, 17.94746523758837142, 12.85593168005540043 ) ) ;
#19192=CARTESIAN_POINT ( 'NONE',  ( -200.0000000000000000, 18.14835560308000950, -46.41341197396098295 ) ) ;
#19193=CARTESIAN_POINT ( 'NONE',  ( 184.8905102610680444, 14.79361573936396113, -14.79361573936377461 ) ) ;
#19194=CARTESIAN_POINT ( 'NONE',  ( -86.86493150571115507, 7.943527260496353826, 19.77569912839162569 ) ) ;
#19196=FACE_OUTER_BOUND ( 'NONE', #14553, .T. ) ;
#19197=CARTESIAN_POINT ( 'NONE',  ( -77.78761611096672368, -9.949180589415803411, 19.59005896970126770 ) ) ;
#19199=CARTESIAN_POINT ( 'NONE',  ( 14.38125909742183062, -67.30136555895943218, -10.73282306403629605 ) ) ;
#19202=ORIENTED_EDGE ( 'NONE', *, *, #9711, .F. ) ;
#19203=CARTESIAN_POINT ( 'NONE',  ( 130.8568914410475372, -24.07718906447255947, 24.07718906447199458 ) ) ;
#19207=CARTESIAN_POINT ( 'NONE',  ( -100.7734535825088500, -40.00000000000027711, 22.67402823373149801 ) ) ;
#19209=VERTEX_POINT ( 'NONE', #8053 ) ;
#19210=EDGE_LOOP ( 'NONE', ( #12224, #25216, #20508, #26020 ) ) ;
#19212=CARTESIAN_POINT ( 'NONE',  ( -259.2033419157646676, 30.48217210827735713, -40.00000000000002132 ) ) ;
#19214=( NAMED_UNIT ( * ) SI_UNIT ( $, .STERADIAN. ) SOLID_ANGLE_UNIT ( ) );
#19217=CARTESIAN_POINT ( 'NONE',  ( 136.1360204305621266, -24.77266263493116583, -24.77266263493127951 ) ) ;
#19218=CARTESIAN_POINT ( 'NONE',  ( -56.48582580120558561, -40.00000000000000000, -9.153146818113723882 ) ) ;
#19222=CARTESIAN_POINT ( 'NONE',  ( -30.26275506840324070, 1.198031551616030033, -1.198031551616006496 ) ) ;
#19223=CARTESIAN_POINT ( 'NONE',  ( 200.0000000000000000, -14.14213562373122457, 42.42640687119282461 ) ) ;
#19224=CARTESIAN_POINT ( 'NONE',  ( -397.9898987322331436, -3.637015436189069562E-14, 0.000000000000000000 ) ) ;
#19225=CARTESIAN_POINT ( 'NONE',  ( -100.7734535825088358, 1.654174317907124744E-13, -17.32597176626811120 ) ) ;
#19226=CARTESIAN_POINT ( 'NONE',  ( -93.02511667906880177, -8.169918093965820916, 20.82219708225673571 ) ) ;
#19227=CARTESIAN_POINT ( 'NONE',  ( 14.38125909742182884, -55.17850393974264733, -40.00000000000002132 ) ) ;
#19228=CARTESIAN_POINT ( 'NONE',  ( 4.995406935893301537, -10.78321810390187530, 67.35176059882529387 ) ) ;
#19229=CARTESIAN_POINT ( 'NONE',  ( 163.1118516004056573, 27.26290988616875310, 0.000000000000000000 ) ) ;
#19231=CARTESIAN_POINT ( 'NONE',  ( -56.48582580120560692, 40.00000000000004263, -9.153146818113443217 ) ) ;
#19232=CARTESIAN_POINT ( 'NONE',  ( 130.8568914410475088, -34.05028731879786363, -40.00000000000002132 ) ) ;
#19233=CARTESIAN_POINT ( 'NONE',  ( -198.0356074513804572, -17.40982414986482141, 39.15871834505909987 ) ) ;
#19234=CARTESIAN_POINT ( 'NONE',  ( 0.2972598230769930017, 14.33493731733933352, 40.00000000000002132 ) ) ;
#19236=CARTESIAN_POINT ( 'NONE',  ( 2.303792037518819669, -44.43800799079054542, 18.40682559463526502 ) ) ;
#19237=CARTESIAN_POINT ( 'NONE',  ( 136.1360204305621551, -35.03383547441293899, -40.00000000000002132 ) ) ;
#19239=ADVANCED_FACE ( 'NONE', ( #12980 ), #4187, .T. ) ;
#19240=CARTESIAN_POINT ( 'NONE',  ( 163.1118516004056573, 9.006482792069629539, 9.006482792069634868 ) ) ;
#19241=CARTESIAN_POINT ( 'NONE',  ( 151.7948205124836250, 1.439163438361279259E-13, -33.23291073765553705 ) ) ;
#19243=CARTESIAN_POINT ( 'NONE',  ( -70.28815428469411586, 9.450978466794646593, -22.81668038993611347 ) ) ;
#19245=EDGE_CURVE ( 'NONE', #16255, #3931, #5038, .T. ) ;
#19246=CARTESIAN_POINT ( 'NONE',  ( 184.8905102610680444, 13.49065550809757497, 43.07788698682593065 ) ) ;
#19248=CARTESIAN_POINT ( 'NONE',  ( -82.26533530497842150, 5.042645448768844574, -19.58509566191921181 ) ) ;
#19249=CARTESIAN_POINT ( 'NONE',  ( 199.9999999999999432, -14.14213562373115884, 14.14213562373085153 ) ) ;
#19252=CARTESIAN_POINT ( 'NONE',  ( -280.0000000000000568, 42.42640687119274645, 14.14213562373118194 ) ) ;
#19254=CARTESIAN_POINT ( 'NONE',  ( 0.2972598230769976091, -10.13633138497465147, -10.13633138497482733 ) ) ;
#19255=CARTESIAN_POINT ( 'NONE',  ( -197.6433718613433825, 18.53520099273998412, -44.74793361789878787 ) ) ;
#19256=CARTESIAN_POINT ( 'NONE',  ( 136.1360204305621266, 3.511608612530757068, -3.511608612530642937 ) ) ;
#19257=CARTESIAN_POINT ( 'NONE',  ( -198.0356074513804572, 39.15871834505956173, -39.15871834505865223 ) ) ;
#19258=CARTESIAN_POINT ( 'NONE',  ( -259.2033419157646676, -9.517827891722680178, 0.000000000000000000 ) ) ;
#19259=CARTESIAN_POINT ( 'NONE',  ( 146.6084372240433709, 32.08495691632064961, -24.48358557860320417 ) ) ;
#19261=CARTESIAN_POINT ( 'NONE',  ( -91.56559293963834989, -40.53558337403692491, 16.03295912088671571 ) ) ;
#19263=CARTESIAN_POINT ( 'NONE',  ( 130.8568914410475372, 4.207082182992862407, 4.207082182992856190 ) ) ;
#19264=CARTESIAN_POINT ( 'NONE',  ( -105.4741150117382773, -19.77569912955116749, -7.943527260750395946 ) ) ;
#19265=CARTESIAN_POINT ( 'NONE',  ( 22.72189371635424138, 23.48424859981869517, 43.05215026464263417 ) ) ;
#19266=CARTESIAN_POINT ( 'NONE',  ( -47.30403195807869565, -30.40121262112982237, -12.59259458005243282 ) ) ;
#19268=CARTESIAN_POINT ( 'NONE',  ( -129.2920181225733813, -25.26067667731744848, 10.46331487444209074 ) ) ;
#19270=CARTESIAN_POINT ( 'NONE',  ( 22.72611120194076761, -17.88893075486376105, 43.18769924474467814 ) ) ;
#19271=CARTESIAN_POINT ( 'NONE',  ( 98.29820294270297154, 18.47759065022021474, -7.653668647299666894 ) ) ;
#19273=CARTESIAN_POINT ( 'NONE',  ( -86.96347745069645896, -12.89780903124443689, 43.67073346367968156 ) ) ;
#19274=CARTESIAN_POINT ( 'NONE',  ( -135.8532207217289738, 7.002209520526292428E-15, -9.153146818113572891 ) ) ;
#19275=CARTESIAN_POINT ( 'NONE',  ( -82.28158553065811986, -6.254237062281328363, 19.22561360847505085 ) ) ;
#19277=CARTESIAN_POINT ( 'NONE',  ( -56.48582580120558561, -30.84685318188645553, -40.00000000000002132 ) ) ;
#19278=CARTESIAN_POINT ( 'NONE',  ( 23.64688638900278050, -23.28414885118052524, -42.77321027809716725 ) ) ;
#19280=CARTESIAN_POINT ( 'NONE',  ( 151.7948205124835681, 33.23291073765556547, 40.00000000000002132 ) ) ;
#19281=CARTESIAN_POINT ( 'NONE',  ( 0.2972598230769976091, -10.13633138497479180, 10.13633138497468522 ) ) ;
#19282=CARTESIAN_POINT ( 'NONE',  ( -213.1075012329537230, 40.00000000000055422, -53.71589010953623244 ) ) ;
#19284=CARTESIAN_POINT ( 'NONE',  ( 170.2234770963711128, 1.955190573858485757E-13, -15.44714144992816074 ) ) ;
#19285=CARTESIAN_POINT ( 'NONE',  ( 130.8879939280389237, -29.49769239790404640, -12.21834424992166923 ) ) ;
#19287=CARTESIAN_POINT ( 'NONE',  ( -91.56559293963834989, 16.03295912088683650, 40.53558337403684675 ) ) ;
#19288=VERTEX_POINT ( 'NONE', #19705 ) ;
#19289=CARTESIAN_POINT ( 'NONE',  ( 199.9999999999999432, 14.14213562373093680, 14.14213562373114641 ) ) ;
#19290=CARTESIAN_POINT ( 'NONE',  ( 11.38508063392656666, 49.30460303390188415, -14.17561098847166967 ) ) ;
#19291=CARTESIAN_POINT ( 'NONE',  ( 146.6084372240433709, 34.62501878078307982, 40.00000000000002132 ) ) ;
#19297=CARTESIAN_POINT ( 'NONE',  ( -280.0000000000000000, 14.14213562373098299, -14.14213562373088706 ) ) ;
#19298=CARTESIAN_POINT ( 'NONE',  ( 98.29820294267321401, -18.47759065023119973, -7.653668647304142425 ) ) ;
#19299=VERTEX_POINT ( 'NONE', #17329 ) ;
#19300=ORIENTED_EDGE ( 'NONE', *, *, #6706, .T. ) ;
#19303=CARTESIAN_POINT ( 'NONE',  ( -56.48582580120559982, -34.75652343174615311, 21.81201906317766870 ) ) ;
#19304=CARTESIAN_POINT ( 'NONE',  ( -199.9999999999998010, 24.82633483071100500, -44.86878812508844305 ) ) ;
#19305=CARTESIAN_POINT ( 'NONE',  ( -198.0356074513804572, 39.99999999999992895, 15.37879056873084771 ) ) ;
#19306=CARTESIAN_POINT ( 'NONE',  ( -199.9999999999999432, -45.24754806068997937, 21.40989205436307685 ) ) ;
#19309=CARTESIAN_POINT ( 'NONE',  ( 184.8905102610680444, 2.362515690532070066E-13, -19.07866798485558490 ) ) ;
#19310=CARTESIAN_POINT ( 'NONE',  ( -56.48582580120558561, 3.151766524733697544E-13, -30.84685318188644132 ) ) ;
#19311=CARTESIAN_POINT ( 'NONE',  ( -77.56416967749056823, 16.64106674400274954, 14.59748372935088412 ) ) ;
#19312=CARTESIAN_POINT ( 'NONE',  ( 163.1118516004056573, -9.006482792073960297, -47.56205970284963769 ) ) ;
#19314=CARTESIAN_POINT ( 'NONE',  ( -195.1686598215018762, 24.52826087131413502, 44.46432177480297554 ) ) ;
#19315=CARTESIAN_POINT ( 'NONE',  ( 144.9504669809063557, 30.13886470195693335, 12.48392651407845122 ) ) ;
#19318=CARTESIAN_POINT ( 'NONE',  ( -162.0762913951020892, -1.198031840385783919, 1.198031840385741731 ) ) ;
#19319=CARTESIAN_POINT ( 'NONE',  ( -82.24857225180262787, -11.87278284862285105, 16.34324723836312998 ) ) ;
#19320=CARTESIAN_POINT ( 'NONE',  ( -162.0762913951021176, 1.198031840315997298, 57.76657433523996588 ) ) ;
#19321=CARTESIAN_POINT ( 'NONE',  ( 19.06497207195982568, -38.31983398719592770, -38.31983398719660272 ) ) ;
#19322=CARTESIAN_POINT ( 'NONE',  ( -187.3037411061693263, -13.75782484033365449, -46.64555264106012800 ) ) ;
#19323=CARTESIAN_POINT ( 'NONE',  ( 5.009866156928151071, 24.71463403307581430, 44.71726210619342368 ) ) ;
#19324=EDGE_LOOP ( 'NONE', ( #116, #14947, #2354, #20882 ) ) ;
#19325=CARTESIAN_POINT ( 'NONE',  ( 192.4448373802100889, 14.14213562370330379, -14.14213562370292365 ) ) ;
#19328=ORIENTED_EDGE ( 'NONE', *, *, #9622, .F. ) ;
#19329=CARTESIAN_POINT ( 'NONE',  ( -30.26275506840324070, 1.218738420030236455E-14, -1.694272468446259783 ) ) ;
#19333=VERTEX_POINT ( 'NONE', #986 ) ;
#19334=CARTESIAN_POINT ( 'NONE',  ( 57.59792236341147031, 37.56421063658187620, 40.00000000000002132 ) ) ;
#19335=CARTESIAN_POINT ( 'NONE',  ( 192.4448373802100889, 14.14213562375893574, -14.14213562375874922 ) ) ;
#19336=CARTESIAN_POINT ( 'NONE',  ( 14.38125909742180220, 39.99999999999997158, 15.17850393972647716 ) ) ;
#19340=CARTESIAN_POINT ( 'NONE',  ( -77.90255099906859471, -8.644468104251766150, 20.04994828524300843 ) ) ;
#19341=CARTESIAN_POINT ( 'NONE',  ( -238.4067589809705794, -4.716212492215116094E-14, 0.9644942799825824142 ) ) ;
#19343=MECHANICAL_DESIGN_GEOMETRIC_PRESENTATION_REPRESENTATION('',(#11689),#15105);
#19345=CARTESIAN_POINT ( 'NONE',  ( -86.95455990305946159, 9.640326247162176898, 19.12039797428042220 ) ) ;
#19346=CARTESIAN_POINT ( 'NONE',  ( 163.1118516004056573, -19.27778845538787422, 19.27778845538743724 ) ) ;
#19347=CARTESIAN_POINT ( 'NONE',  ( 184.8905102610680444, 14.79361573936375507, 14.79361573936398067 ) ) ;
#19349=CARTESIAN_POINT ( 'NONE',  ( 192.4448373802101173, -39.99999999999977973, -19.99999999996102673 ) ) ;
#19351=CARTESIAN_POINT ( 'NONE',  ( -30.26275506840324425, -1.694272468446265334, -40.00000000000002132 ) ) ;
#19352=CARTESIAN_POINT ( 'NONE',  ( -259.2033419157646676, 6.730120644403521979, -6.730120644403498886 ) ) ;
#19353=CARTESIAN_POINT ( 'NONE',  ( -30.26275506840324425, -1.694272468446265334, -40.00000000000002132 ) ) ;
#19355=CARTESIAN_POINT ( 'NONE',  ( 146.6084372240433993, 1.478241399363601114E-13, -34.62501878078305850 ) ) ;
#19356=CARTESIAN_POINT ( 'NONE',  ( -56.48582580120559271, -9.153146818113595984, 0.000000000000000000 ) ) ;
#19357=CARTESIAN_POINT ( 'NONE',  ( -56.48582580120559982, 50.09629031063966664, -6.472252184284094767 ) ) ;
#19358=CARTESIAN_POINT ( 'NONE',  ( -198.0356074513804572, 55.37879056873070027, 2.449293598294708485E-15 ) ) ;
#19360=CARTESIAN_POINT ( 'NONE',  ( 22.90311673804475845, -46.98314248934332227, 13.82691048573679815 ) ) ;
#19362=CARTESIAN_POINT ( 'NONE',  ( -4.039451493210497901, 23.44932283416708074, -43.00522595893983890 ) ) ;
#19363=CARTESIAN_POINT ( 'NONE',  ( 170.2234770963711128, -17.36149277826995885, 39.20704971665388427 ) ) ;
#19364=CARTESIAN_POINT ( 'NONE',  ( -135.8532207217289738, 7.002209520526292428E-15, -9.153146818113572891 ) ) ;
#19365=CARTESIAN_POINT ( 'NONE',  ( -82.23936494317537438, 20.15025730830772233, 1.484621625134467937 ) ) ;
#19369=CARTESIAN_POINT ( 'NONE',  ( 18.89824444022307048, -14.00990882958388184, -48.20791849611967450 ) ) ;
#19372=CARTESIAN_POINT ( 'NONE',  ( -82.29192131167501145, -6.849507299441772723, -18.98456886706201274 ) ) ;
#19373=CARTESIAN_POINT ( 'NONE',  ( 170.2234770963711128, 10.92277846919147066, 45.64576402573197811 ) ) ;
#19374=CARTESIAN_POINT ( 'NONE',  ( 163.1118516004056573, 19.27778845539265618, -37.29075403953135037 ) ) ;
#19375=CARTESIAN_POINT ( 'NONE',  ( 0.2972598230769923355, 18.14793986248697166, 38.42060263243675422 ) ) ;
#19376=DIRECTION ( 'NONE',  ( -0.01051738777840964360, -0.3656191333258750342, -0.9307051272558644062 ) ) ;
#19377=CARTESIAN_POINT ( 'NONE',  ( -100.7734535825088358, -12.25131212657475643, -12.25131212657495539 ) ) ;
#19379=CARTESIAN_POINT ( 'NONE',  ( 19.06497207195980792, 18.24870850772790831, -38.31983398719609824 ) ) ;
#19380=CARTESIAN_POINT ( 'NONE',  ( 200.0000000000000000, -42.42640687119272513, -14.14213562373140753 ) ) ;
#19381=CARTESIAN_POINT ( 'NONE',  ( -105.3755690713226727, 12.89780903124418998, -12.89780903124389155 ) ) ;
#19382=CARTESIAN_POINT ( 'NONE',  ( -280.0000000000000000, -20.00000000000006750, 0.000000000000000000 ) ) ;
#19383=CARTESIAN_POINT ( 'NONE',  ( 170.2234770963711128, -17.36149277826985937, -17.36149277826995174 ) ) ;
#19386=CARTESIAN_POINT ( 'NONE',  ( 184.8905102610680444, -41.77492675556007384, 14.79361573936348684 ) ) ;
#19388=CARTESIAN_POINT ( 'NONE',  ( -121.8281105898230692, 22.46071553299150381, -10.16551987237939336 ) ) ;
#19389=ORIENTED_EDGE ( 'NONE', *, *, #11896, .F. ) ;
#19391=CARTESIAN_POINT ( 'NONE',  ( -56.48582580120559982, 50.09629031063966664, -6.472252184284094767 ) ) ;
#19392=CARTESIAN_POINT ( 'NONE',  ( -28.75808802591298630, 38.33175228464058648, -12.03522322449772552 ) ) ;
#19393=CARTESIAN_POINT ( 'NONE',  ( 11.28112952480474895, 18.58737866930062665, 44.87390167243342631 ) ) ;
#19394=CARTESIAN_POINT ( 'NONE',  ( -24.53392603777601977, -39.81639166317236800, -12.34411287782893041 ) ) ;
#19398=CARTESIAN_POINT ( 'NONE',  ( -151.4802849348335769, -33.96623543976281212, 11.09498666344389761 ) ) ;
#19401=CARTESIAN_POINT ( 'NONE',  ( 23.10188454848158557, -13.81611343686630100, 46.91040837924295204 ) ) ;
#19404=FACE_OUTER_BOUND ( 'NONE', #23454, .T. ) ;
#19405=CARTESIAN_POINT ( 'NONE',  ( 4.995406935893290878, -5.232665749138292703E-14, 15.24977328854832592 ) ) ;
#19406=CARTESIAN_POINT ( 'NONE',  ( -198.0356074513804572, -9.007331120208026888E-14, 15.37879056873070560 ) ) ;
#19407=CARTESIAN_POINT ( 'NONE',  ( 23.37394308801976450, 46.80823611210215063, -13.80096434448263309 ) ) ;
#19408=CARTESIAN_POINT ( 'NONE',  ( 163.1118516004056573, -12.73709011382471878, -40.00000000000002132 ) ) ;
#19409=CARTESIAN_POINT ( 'NONE',  ( -184.9730489280930215, 22.80026000644289752, -42.02334742179726135 ) ) ;
#19410=CARTESIAN_POINT ( 'NONE',  ( -280.0000000000000000, -20.00000000000006750, 0.000000000000000000 ) ) ;
#19411=CARTESIAN_POINT ( 'NONE',  ( -56.48582580120558561, -30.84685318188645908, 40.00000000000002132 ) ) ;
#19412=CARTESIAN_POINT ( 'NONE',  ( 130.8568914410475372, 24.07718906447243867, -24.07718906447216156 ) ) ;
#19413=CARTESIAN_POINT ( 'NONE',  ( 130.8568914410475088, 40.00000000000011369, -5.949712681206269949 ) ) ;
#19414=CARTESIAN_POINT ( 'NONE',  ( 146.6084372240433709, -40.00000000000036238, 34.62501878078263218 ) ) ;
#19417=CARTESIAN_POINT ( 'NONE',  ( 14.38125909742181285, -10.73282306404712472, -10.73282306404731301 ) ) ;
#19418=CARTESIAN_POINT ( 'NONE',  ( 9.028290303185290355, 44.88859993222921929, -18.59346688788140867 ) ) ;
#19419=CARTESIAN_POINT ( 'NONE',  ( 184.8905102610680444, -19.07866798485554938, 40.00000000000002132 ) ) ;
#19421=CARTESIAN_POINT ( 'NONE',  ( -193.3669111531376075, 44.23532963564892384, -18.32287347112458065 ) ) ;
#19424=VERTEX_POINT ( 'NONE', #4984 ) ;
#19425=CARTESIAN_POINT ( 'NONE',  ( -213.1075012329537230, -9.698598906450557777, 9.698598906450415669 ) ) ;
#19426=CARTESIAN_POINT ( 'NONE',  ( 83.11963132847050417, -23.63628489299456348, -10.90660717668977497 ) ) ;
#19431=CARTESIAN_POINT ( 'NONE',  ( 0.2972598230769959993, 38.42060263243659080, 38.42060263243672580 ) ) ;
#19433=CARTESIAN_POINT ( 'NONE',  ( -105.3755690713226727, 5.661656051307470077E-14, -21.75974354311649961 ) ) ;
#19435=CARTESIAN_POINT ( 'NONE',  ( 200.0000000000000000, -39.99999999999977973, -20.00000000000034817 ) ) ;
#19436=CARTESIAN_POINT ( 'NONE',  ( -56.48582580120559982, 40.00000000000034106, -30.84685318188602210 ) ) ;
#19437=CARTESIAN_POINT ( 'NONE',  ( -114.7248266913187678, -17.87714126012797422, 12.97729011816987565 ) ) ;
#19438=CARTESIAN_POINT ( 'NONE',  ( -135.8532207217289738, -21.81201906317758343, -34.75652343174620995 ) ) ;
#19440=CARTESIAN_POINT ( 'NONE',  ( -194.7885354600661572, 18.40784581029643263, 44.44047100928790428 ) ) ;
#19441=CARTESIAN_POINT ( 'NONE',  ( 130.1167162091013836, 29.33455044752954777, 12.15076864148460878 ) ) ;
#19442=CARTESIAN_POINT ( 'NONE',  ( -3.903133374382439236, -47.03983734342246947, 13.83543723413883342 ) ) ;
#19443=CARTESIAN_POINT ( 'NONE',  ( 136.1360204305621266, 24.77266263493138965, -24.77266263493110188 ) ) ;
#19444=CARTESIAN_POINT ( 'NONE',  ( -82.24297220891752147, -15.98176361808475576, 12.40742895866242890 ) ) ;
#19445=CARTESIAN_POINT ( 'NONE',  ( 146.6084372240433709, -52.76785682606516303, 3.800685668858563737 ) ) ;
#19446=CARTESIAN_POINT ( 'NONE',  ( -280.0000000000000568, -42.42640687119305198, 14.14213562373058686 ) ) ;
#19448=CARTESIAN_POINT ( 'NONE',  ( 98.29820294267490510, 4.808046699556526995E-12, 20.00000000000513722 ) ) ;
#19450=CARTESIAN_POINT ( 'NONE',  ( -259.2033419157646676, 21.55415060305860209, -21.55415060305812602 ) ) ;
#19452=CARTESIAN_POINT ( 'NONE',  ( -28.75791583366072501, 12.03523584680509551, -38.33181286256363052 ) ) ;
#19454=CARTESIAN_POINT ( 'NONE',  ( 19.06497207195981147, 1.521599808664285085E-13, -14.19242893257840521 ) ) ;
#19455=CARTESIAN_POINT ( 'NONE',  ( -4.039451493210490796, -23.44932283416679297, 43.00522595894000943 ) ) ;
#19456=CARTESIAN_POINT ( 'NONE',  ( -28.75808802781981655, 18.59445401971606060, 35.61482992978285722 ) ) ;
#19458=ORIENTED_EDGE ( 'NONE', *, *, #15475, .F. ) ;
#19459=CARTESIAN_POINT ( 'NONE',  ( 151.7948205124836250, 23.49921654116361225, -23.49921654116333514 ) ) ;
#19461=CARTESIAN_POINT ( 'NONE',  ( -100.7734535825088500, 39.99999999999994316, 17.32597176626825686 ) ) ;
#19462=CARTESIAN_POINT ( 'NONE',  ( -96.94449363886086246, -20.74048850971937696, -8.590991631070833634 ) ) ;
#19464=( BOUNDED_SURFACE ( )  B_SPLINE_SURFACE ( 3, 2, ( 
 ( #12282, #2183, #16003 ),
 ( #4050, #3919, #10552 ),
 ( #8157, #12151, #12018 ),
 ( #20274, #18131, #20671 ),
 ( #2052, #26138, #10292 ),
 ( #16135, #16270, #10159 ) ),
 .UNSPECIFIED., .F., .F., .F. ) 
 B_SPLINE_SURFACE_WITH_KNOTS ( ( 4, 2, 4 ),
 ( 3, 3 ),
 ( 0.04143195986180998186, 0.04845790097405862362, 0.05548384208630727232 ),
 ( 0.000000000000000000, 1.000000000000000000 ),
 .UNSPECIFIED. ) 
 GEOMETRIC_REPRESENTATION_ITEM ( )  RATIONAL_B_SPLINE_SURFACE ( (
 ( 1.000000000000000000, 0.9541700777564564584, 1.000000000000000000),
 ( 1.000000000000000000, 0.9520117016566322921, 1.000000000000000000),
 ( 1.000000000000000000, 0.9503157806802187135, 1.000000000000000000),
 ( 1.000000000000000000, 0.9480088156000070487, 1.000000000000000000),
 ( 1.000000000000000000, 0.9474362554095308031, 1.000000000000000000),
 ( 1.000000000000000000, 0.9474350312570029020, 1.000000000000000000) ) ) 
 REPRESENTATION_ITEM ( '' )  SURFACE ( )  );
#19465=CARTESIAN_POINT ( 'NONE',  ( -162.0762913951021176, -40.00000000000005684, 1.694272876828184504 ) ) ;
#19469=CARTESIAN_POINT ( 'NONE',  ( 136.1360204305621551, 24.77266263493153176, -31.79587985999237887 ) ) ;
#19471=CARTESIAN_POINT ( 'NONE',  ( -86.96347745069643054, -39.99999999999985079, -18.24025645688394448 ) ) ;
#19472=CARTESIAN_POINT ( 'NONE',  ( 23.37394308801978582, -46.80823611210187352, -13.80096434448294396 ) ) ;
#19473=CARTESIAN_POINT ( 'NONE',  ( -198.0356074513804572, -15.37879056873074290, 40.00000000000002132 ) ) ;
#19474=CARTESIAN_POINT ( 'NONE',  ( -100.7734535825088500, -17.32597176626812185, -40.00000000000002132 ) ) ;
#19476=CARTESIAN_POINT ( 'NONE',  ( -198.0356074513804572, -10.87444709759729911, 10.87444709759714812 ) ) ;
#19477=CARTESIAN_POINT ( 'NONE',  ( -105.3755690713226585, 21.75974354311648185, -40.00000000000002132 ) ) ;
#19478=CARTESIAN_POINT ( 'NONE',  ( -3.762763306026898569, -43.08566851766588712, -23.50897034858821399 ) ) ;
#19480=B_SPLINE_CURVE_WITH_KNOTS ( 'NONE', 3,
 ( #20635, #16639, #24899, #14769, #12916, #18634, #24633, #18902, #12647, #6391, #18769, #20772, #24768, #2411 ),
 .UNSPECIFIED., .F., .F.,
 ( 4, 2, 2, 2, 2, 2, 4 ),
 ( 0.0003146819161523679766, 0.002410867973011127964, 0.004507054029869887735, 0.008699426143587403806, 0.01079561220044616271, 0.01289179825730491814, 0.01708417037102243421 ),
 .UNSPECIFIED. ) ;
#19481=CARTESIAN_POINT ( 'NONE',  ( -213.1075012329537230, 1.045191102001431893E-13, -13.71589010951911902 ) ) ;
#19482=CARTESIAN_POINT ( 'NONE',  ( 130.8568914410475088, -24.07718906446910623, 32.49135343045471558 ) ) ;
#19483=CARTESIAN_POINT ( 'NONE',  ( -56.48582580120559271, 30.84685318188643066, 2.449293598294708485E-15 ) ) ;
#19487=CARTESIAN_POINT ( 'NONE',  ( 60.14720761599947707, -33.22245024482351994, 10.94158980378562163 ) ) ;
#19488=DIRECTION ( 'NONE',  ( -0.01051738777841029586, 0.3995761382614174129, 0.9166396752739929266 ) ) ;
#19489=CARTESIAN_POINT ( 'NONE',  ( -30.26275506840324070, 1.198031551615912571, 57.76657404653985139 ) ) ;
#19490=CARTESIAN_POINT ( 'NONE',  ( 163.1118516004056573, 1.251511021549353291E-13, -27.26290988616872824 ) ) ;
#19491=CARTESIAN_POINT ( 'NONE',  ( -82.30853939107804251, 18.59635467392883612, 7.798227509426476800 ) ) ;
#19492=CARTESIAN_POINT ( 'NONE',  ( -16.87994666116171061, 20.93785811897321025, -39.19724034061671603 ) ) ;
#19495=CARTESIAN_POINT ( 'NONE',  ( -82.25988539629348395, -4.395343885513712578, -19.70400758346194436 ) ) ;
#19496=CARTESIAN_POINT ( 'NONE',  ( -198.0356074513804572, 39.15871834505887250, 17.40982414986519089 ) ) ;
#19497=CARTESIAN_POINT ( 'NONE',  ( -259.2033419157646676, 6.730120644403918995, -49.83842185052024831 ) ) ;
#19498=CARTESIAN_POINT ( 'NONE',  ( -110.0995178903039715, 20.14662320684453789, -1.423929044649810516 ) ) ;
#19499=CARTESIAN_POINT ( 'NONE',  ( 184.8905102610680444, -14.79361573936399665, 14.79361573936367158 ) ) ;
#19500=CARTESIAN_POINT ( 'NONE',  ( 4.995406935893305977, -39.06748935135157552, -39.06748935135225764 ) ) ;
#19501=CARTESIAN_POINT ( 'NONE',  ( -105.3755690713226727, -12.89780903124395550, -12.89780903124416511 ) ) ;
#19502=CARTESIAN_POINT ( 'NONE',  ( 192.4448373802101173, -14.14213562375826605, -42.42640687116518450 ) ) ;
#19503=CARTESIAN_POINT ( 'NONE',  ( 19.06497207195980792, 66.60410523465830579, -10.03556273973354251 ) ) ;
#19508=CARTESIAN_POINT ( 'NONE',  ( -280.0000000000000000, 14.14213562373078581, 14.14213562373108424 ) ) ;
#19509=CARTESIAN_POINT ( 'NONE',  ( -198.0356074513804572, 55.37879056871320671, 40.00000000000002132 ) ) ;
#19511=CARTESIAN_POINT ( 'NONE',  ( -91.56559293963834989, 12.25131212657490209, -44.31723036834897300 ) ) ;
#19512=CARTESIAN_POINT ( 'NONE',  ( -82.28158354860731549, -18.01692715714676041, -9.172261728117373281 ) ) ;
#19513=CARTESIAN_POINT ( 'NONE',  ( 23.42154907652751561, 13.79745687233752349, 46.79103593565447738 ) ) ;
#19516=FACE_OUTER_BOUND ( 'NONE', #25396, .T. ) ;
#19518=CARTESIAN_POINT ( 'NONE',  ( 37.37129771730447203, -12.75330473319407254, 41.71823991403014276 ) ) ;
#19523=EDGE_CURVE ( 'NONE', #14253, #17137, #21709, .T. ) ;
#19525=CARTESIAN_POINT ( 'NONE',  ( -213.1075012329537230, 39.99999999999992895, 13.71589010951925935 ) ) ;
#19526=CARTESIAN_POINT ( 'NONE',  ( -82.30220482034330587, -7.441767004318910139, 18.74474319042423076 ) ) ;
#19527=CARTESIAN_POINT ( 'NONE',  ( 21.99343714674524364, 47.30053030063396591, -13.87412077874980554 ) ) ;
#19528=CARTESIAN_POINT ( 'NONE',  ( 151.7948205124836250, -6.767089262349004208, -2.449293598294708485E-15 ) ) ;
#19529=CARTESIAN_POINT ( 'NONE',  ( -166.7090905287452358, 15.35183918158013405, -37.06261835976449248 ) ) ;
#19532=CARTESIAN_POINT ( 'NONE',  ( 170.2234770963711128, 24.55285855007190676, 40.00000000000002132 ) ) ;
#19533=CARTESIAN_POINT ( 'NONE',  ( 151.7948205124836250, 23.49921654116361225, -23.49921654116333514 ) ) ;
#19534=CARTESIAN_POINT ( 'NONE',  ( -56.48582580120559982, -9.153146818113595984, 40.00000000000002132 ) ) ;
#19535=CARTESIAN_POINT ( 'NONE',  ( -135.8532207217289738, 39.99999999999990763, 9.153146818113990335 ) ) ;
#19536=CARTESIAN_POINT ( 'NONE',  ( 163.1118516004056573, -40.00000000000027711, 27.26290988616830546 ) ) ;
#19537=CARTESIAN_POINT ( 'NONE',  ( 140.2228883168555456, -30.42137490627649044, -12.60094607221633289 ) ) ;
#19540=CARTESIAN_POINT ( 'NONE',  ( -3.417371742523410028, 43.31092608455699633, -17.93997298316182665 ) ) ;
#19541=CARTESIAN_POINT ( 'NONE',  ( 136.1360204305621266, -4.966164525587039691, -2.449293598294708485E-15 ) ) ;
#19542=AXIS2_PLACEMENT_3D ( 'NONE', #19842, #5231, #7339 ) ;
#19544=CARTESIAN_POINT ( 'NONE',  ( -200.5022718138935431, 44.86987976039424098, -18.58571273880625441 ) ) ;
#19546=EDGE_LOOP ( 'NONE', ( #23700, #23340, #14156, #1149, #9277, #21043 ) ) ;
#19547=ORIENTED_EDGE ( 'NONE', *, *, #9481, .T. ) ;
#19549=CARTESIAN_POINT ( 'NONE',  ( 151.0853911467766295, 12.04115959308003525, -29.06993079631216048 ) ) ;
#19550=CARTESIAN_POINT ( 'NONE',  ( -192.1131137119204766, 43.98782916596428549, -24.17676406461154315 ) ) ;
#19554=CARTESIAN_POINT ( 'NONE',  ( -30.26275506840323715, 29.48230279907789253, 29.48230279907799556 ) ) ;
#19556=CARTESIAN_POINT ( 'NONE',  ( 91.82158438592158234, 7.693928927950222250E-14, -17.20528682183300262 ) ) ;
#19557=CARTESIAN_POINT ( 'NONE',  ( -199.9999999999999716, -49.28189405767602693, 14.17215463606940595 ) ) ;
#19560=CIRCLE ( 'NONE', #18714, 14.99999999999999645 ) ;
#19561=CARTESIAN_POINT ( 'NONE',  ( 4.995406935893297984, -39.99999999999986500, -15.24977328854874870 ) ) ;
#19562=CARTESIAN_POINT ( 'NONE',  ( 170.2234770963711128, 1.955190573858485757E-13, -15.44714144992816074 ) ) ;
#19563=CARTESIAN_POINT ( 'NONE',  ( -114.7755410848754281, -16.60116338991689489, 14.64251757343854976 ) ) ;
#19564=CARTESIAN_POINT ( 'NONE',  ( -56.48582580120559982, -21.81201906317755501, -34.75652343174621706 ) ) ;
#19565=CARTESIAN_POINT ( 'NONE',  ( 184.8905102610680444, 1.070102760522089011E-13, -20.92133201514444352 ) ) ;
#19567=CARTESIAN_POINT ( 'NONE',  ( -30.26275506840324070, -1.198031551616032919, 1.198031551616014712 ) ) ;
#19568=CARTESIAN_POINT ( 'NONE',  ( 147.2817042152898068, 29.82799917201313633, 12.35516179550145210 ) ) ;
#19570=CARTESIAN_POINT ( 'NONE',  ( 146.6084372240433709, 52.76785682606519146, 3.800685668858932775 ) ) ;
#19571=CARTESIAN_POINT ( 'NONE',  ( -213.1075012329537230, -40.00000000000011369, 13.71589010951897691 ) ) ;
#19572=CARTESIAN_POINT ( 'NONE',  ( 14.38125909742181463, 10.73282306405862485, 67.30136555898259587 ) ) ;
#19573=( BOUNDED_SURFACE ( )  B_SPLINE_SURFACE ( 3, 2, ( 
 ( #13078, #25576, #23563 ),
 ( #8817, #6814, #13320 ),
 ( #5216, #10818, #16928 ),
 ( #2846, #23190, #7322 ),
 ( #19190, #21440, #25062 ),
 ( #25320, #5338, #18931 ),
 ( #21322, #6942, #23066 ),
 ( #19311, #15436, #21193 ),
 ( #25194, #5095, #8952 ),
 ( #17184, #4838, #13447 ) ),
 .UNSPECIFIED., .F., .F., .F. ) 
 B_SPLINE_SURFACE_WITH_KNOTS ( ( 4, 2, 2, 2, 4 ),
 ( 3, 3 ),
 ( 0.04080948307332495084, 0.04814637154418376086, 0.04998059366189846336, 0.05181481577961316587, 0.05548326001504257088 ),
 ( 0.000000000000000000, 1.000000000000000000 ),
 .UNSPECIFIED. ) 
 GEOMETRIC_REPRESENTATION_ITEM ( )  RATIONAL_B_SPLINE_SURFACE ( (
 ( 1.000000000000000000, 0.9547549646669141188, 1.000000000000000000),
 ( 1.000000000000000000, 0.9524144703618939722, 1.000000000000000000),
 ( 1.000000000000000000, 0.9505737003611494096, 1.000000000000000000),
 ( 1.000000000000000000, 0.9490046242078488126, 1.000000000000000000),
 ( 1.000000000000000000, 0.9487292854021939226, 1.000000000000000000),
 ( 1.000000000000000000, 0.9482585386214895662, 1.000000000000000000),
 ( 1.000000000000000000, 0.9480625482234854573, 1.000000000000000000),
 ( 1.000000000000000000, 0.9475921161413758398, 1.000000000000000000),
 ( 1.000000000000000000, 0.9474351228594215524, 1.000000000000000000),
 ( 1.000000000000000000, 0.9474350314971546894, 1.000000000000000000) ) ) 
 REPRESENTATION_ITEM ( '' )  SURFACE ( )  );
#19574=CARTESIAN_POINT ( 'NONE',  ( -198.0356074513804572, -39.15871834505931304, 17.40982414986437377 ) ) ;
#19576=CARTESIAN_POINT ( 'NONE',  ( 22.27781863254865158, 23.58928354748257661, 43.19367102556063287 ) ) ;
#19578=CARTESIAN_POINT ( 'NONE',  ( -30.26275506840323715, 29.48230279907829754, -29.48230279907758344 ) ) ;
#19584=CARTESIAN_POINT ( 'NONE',  ( -3.762763306026896792, -23.50897034858817491, 43.08566851766595107 ) ) ;
#19585=CARTESIAN_POINT ( 'NONE',  ( -62.79433447035942351, 9.335111860984262933, 25.93934121792603875 ) ) ;
#19591=CARTESIAN_POINT ( 'NONE',  ( -238.4067589809705794, -28.96627169325313389, -27.60227080167074831 ) ) ;
#19592=CARTESIAN_POINT ( 'NONE',  ( -198.0356074513804572, 39.99999999999992895, 15.37879056873084771 ) ) ;
#19593=CARTESIAN_POINT ( 'NONE',  ( 48.46159167847756066, 11.89574563387566464, -37.63079830025095163 ) ) ;
#19595=CARTESIAN_POINT ( 'NONE',  ( -208.1127848780265026, -2.327190355601776466E-13, 55.00245453012672670 ) ) ;
#19598=CARTESIAN_POINT ( 'NONE',  ( 91.82158438592156813, 39.99999999999995737, 22.79471317813484887 ) ) ;
#19601=CARTESIAN_POINT ( 'NONE',  ( -5.304449574936379364, -17.72890873421744473, -42.80137191221640336 ) ) ;
#19602=CARTESIAN_POINT ( 'NONE',  ( -280.0000000000000568, 42.42640687119294540, -14.14213562373059041 ) ) ;
#19603=CARTESIAN_POINT ( 'NONE',  ( -105.2334157265396044, -21.31091308246848115, 2.725992507772964757 ) ) ;
#19604=CARTESIAN_POINT ( 'NONE',  ( 130.8568914410475088, -39.99999999999992895, -5.949712681207114606 ) ) ;
#19606=CARTESIAN_POINT ( 'NONE',  ( 57.59792236341147031, 2.435789363418170872, 40.00000000000002132 ) ) ;
#19607=CARTESIAN_POINT ( 'NONE',  ( -280.0000000000000568, -20.00000000000006395, -40.00000000000002132 ) ) ;
#19608=CARTESIAN_POINT ( 'NONE',  ( -86.96347745069645896, 43.67073346367970288, 12.89780903124427702 ) ) ;
#19609=CARTESIAN_POINT ( 'NONE',  ( 57.59792236341147031, 2.435789363418170872, -40.00000000000002132 ) ) ;
#19610=CARTESIAN_POINT ( 'NONE',  ( -3.901164313503183934, -43.04571088859058392, -23.47934491069905505 ) ) ;
#19611=DIRECTION ( 'NONE',  ( -0.3301743753983408247, 0.000000000000000000, -0.9439199552029374773 ) ) ;
#19612=CARTESIAN_POINT ( 'NONE',  ( -86.96347745069644475, -2.438961472018186339E-13, 21.75974354311649961 ) ) ;
#19613=CARTESIAN_POINT ( 'NONE',  ( 170.2234770963711128, 10.92277846919201068, 10.92277846919202133 ) ) ;
#19614=CARTESIAN_POINT ( 'NONE',  ( 130.8568914410475088, 5.949712681206719367, -40.00000000000002132 ) ) ;
#19615=ORIENTED_EDGE ( 'NONE', *, *, #16052, .T. ) ;
#19616=CARTESIAN_POINT ( 'NONE',  ( 59.93546481438061591, -31.86477106141256499, 13.19882033579247960 ) ) ;
#19619=( BOUNDED_SURFACE ( )  B_SPLINE_SURFACE ( 3, 2, ( 
 ( #11876, #22408, #22273 ),
 ( #4184, #10288, #19859 ),
 ( #1645, #17854, #26005 ),
 ( #5761, #13869, #19996 ),
 ( #1782, #9886, #26135 ),
 ( #7878, #5897, #22135 ),
 ( #22801, #16798, #6421 ),
 ( #4578, #173, #20938 ),
 ( #14407, #24935, #22537 ),
 ( #6684, #22669, #4441 ),
 ( #12535, #12675, #20669 ),
 ( #2716, #8689, #10550 ),
 ( #2304, #18934, #312 ),
 ( #14799, #16536, #24664 ),
 ( #6817, #8414, #4841 ),
 ( #14539, #8279, #25066 ),
 ( #22931, #12408, #18396 ),
 ( #20805, #582, #2438 ),
 ( #8820, #18662, #448 ),
 ( #10821, #12947, #16405 ),
 ( #14933, #21063, #10690 ),
 ( #2576, #10413, #2849 ),
 ( #18802, #8552, #16668 ),
 ( #24533, #24799, #4711 ),
 ( #6551, #14661, #12815 ),
 ( #716, #16931, #23070 ),
 ( #6289, #4318, #20533 ),
 ( #18531, #13323, #7452 ),
 ( #17318, #13203, #9332 ),
 ( #17064, #19440, #15196 ),
 ( #21698, #9081, #19314 ),
 ( #23691, #8955, #15063 ),
 ( #13572, #3218, #17441 ),
 ( #23322, #9207, #25323 ) ),
 .UNSPECIFIED., .F., .F., .F. ) 
 B_SPLINE_SURFACE_WITH_KNOTS ( ( 4, 2, 2, 2, 2, 2, 2, 2, 2, 2, 2, 2, 2, 2, 2, 2, 4 ),
 ( 3, 3 ),
 ( 0.005135432767688113270, 0.02907015807668449081, 0.05300488338568087182, 0.07693960869467725283, 0.08292329002192634635, 0.08441921035373861626, 0.08446595786410775186, 0.08448933161929231273, 0.08451270537447688747, 0.08460620039521515867, 0.08479319043669168721, 0.08516717051964475815, 0.08591513068555090005, 0.08890697134917543987, 0.09189881201279997969, 0.09489065267642453338, 0.1008743340036736269 ),
 ( 0.000000000000000000, 1.000000000000000000 ),
 .UNSPECIFIED. ) 
 GEOMETRIC_REPRESENTATION_ITEM ( )  RATIONAL_B_SPLINE_SURFACE ( (
 ( 1.000000000000000000, 0.9997813423552078804, 1.000000000000000000),
 ( 1.000000000000000000, 0.9991063898506408192, 1.000000000000000000),
 ( 1.000000000000000000, 0.9968824705949637099, 1.000000000000000000),
 ( 1.000000000000000000, 0.9891556793369806755, 1.000000000000000000),
 ( 1.000000000000000000, 0.9836552277522174759, 1.000000000000000000),
 ( 1.000000000000000000, 0.9690805015303916026, 1.000000000000000000),
 ( 1.000000000000000000, 0.9600094330334334458, 1.000000000000000000),
 ( 1.000000000000000000, 0.9461485276689314272, 1.000000000000000000),
 ( 1.000000000000000000, 0.9432497373318702305, 1.000000000000000000),
 ( 1.000000000000000000, 0.9394620364517939359, 1.000000000000000000),
 ( 1.000000000000000000, 0.9386962831138077057, 1.000000000000000000),
 ( 1.000000000000000000, 0.9378980481303066385, 1.000000000000000000),
 ( 1.000000000000000000, 0.9378738510928930072, 1.000000000000000000),
 ( 1.000000000000000000, 0.9378375433852924603, 1.000000000000000000),
 ( 1.000000000000000000, 0.9378253334781214701, 1.000000000000000000),
 ( 1.000000000000000000, 0.9378014123365938648, 1.000000000000000000),
 ( 1.000000000000000000, 0.9377894572438921772, 1.000000000000000000),
 ( 1.000000000000000000, 0.9377297092068129780, 1.000000000000000000),
 ( 1.000000000000000000, 0.9376819985415359993, 1.000000000000000000),
 ( 1.000000000000000000, 0.9375391312191762028, 1.000000000000000000),
 ( 1.000000000000000000, 0.9374442392361908016, 1.000000000000000000),
 ( 1.000000000000000000, 0.9371606329892256948, 1.000000000000000000),
 ( 1.000000000000000000, 0.9369729884417120624, 1.000000000000000000),
 ( 1.000000000000000000, 0.9364144211479323854, 1.000000000000000000),
 ( 1.000000000000000000, 0.9360478649890134895, 1.000000000000000000),
 ( 1.000000000000000000, 0.9342453465010656100, 1.000000000000000000),
 ( 1.000000000000000000, 0.9329002455189610021, 1.000000000000000000),
 ( 1.000000000000000000, 0.9304321598239908564, 1.000000000000000000),
 ( 1.000000000000000000, 0.9293115443287026656, 1.000000000000000000),
 ( 1.000000000000000000, 0.9273348408776519447, 1.000000000000000000),
 ( 1.000000000000000000, 0.9264755133098839801, 1.000000000000000000),
 ( 1.000000000000000000, 0.9243017816397209874, 1.000000000000000000),
 ( 1.000000000000000000, 0.9233922826851888033, 1.000000000000000000),
 ( 1.000000000000000000, 0.9230541040371973427, 1.000000000000000000) ) ) 
 REPRESENTATION_ITEM ( '' )  SURFACE ( )  );
#19620=CARTESIAN_POINT ( 'NONE',  ( -198.0356074513804572, 39.15871834505901461, 39.15871834505919935 ) ) ;
#19621=CARTESIAN_POINT ( 'NONE',  ( -100.7734535825088500, -39.99999999999995737, -22.67402823373205578 ) ) ;
#19622=CARTESIAN_POINT ( 'NONE',  ( 130.8568914410475372, -24.07718906447255947, 24.07718906447199458 ) ) ;
#19623=CARTESIAN_POINT ( 'NONE',  ( 4.995406935893289102, 55.24977328856464709, -40.00000000000002132 ) ) ;
#19626=CARTESIAN_POINT ( 'NONE',  ( -86.95438060917183520, 6.705903726404473630, -20.33578048843545361 ) ) ;
#19627=CARTESIAN_POINT ( 'NONE',  ( 130.8568914410475372, -24.07718906447255947, 24.07718906447199458 ) ) ;
#19628=CARTESIAN_POINT ( 'NONE',  ( -135.8532207217289738, 6.472252184284583265, -50.09629031063960980 ) ) ;
#19630=CARTESIAN_POINT ( 'NONE',  ( -110.1018896729135577, 20.19745059498566064, -0.1210535641494778075 ) ) ;
#19631=CARTESIAN_POINT ( 'NONE',  ( 170.2234770963711128, -17.36149277827010096, 17.36149277826970660 ) ) ;
#19632=CARTESIAN_POINT ( 'NONE',  ( 184.8905102610680444, 43.07788698682591644, -13.49065550809769221 ) ) ;
#19634=CARTESIAN_POINT ( 'NONE',  ( -208.1127848780264742, -10.60833733270725787, -67.17687982763172272 ) ) ;
#19635=CARTESIAN_POINT ( 'NONE',  ( -56.48582580120559982, -6.472252184283581400, -50.09629031063973059 ) ) ;
#19636=CARTESIAN_POINT ( 'NONE',  ( -162.0762913951021176, -27.08623940707584055, -29.48230308784799547 ) ) ;
#19637=CARTESIAN_POINT ( 'NONE',  ( 19.06497207195980792, 14.19242893257840876, 0.000000000000000000 ) ) ;
#19639=CARTESIAN_POINT ( 'NONE',  ( -198.0356074513804572, -40.00000000000025580, 55.37879056871310013 ) ) ;
#19641=CARTESIAN_POINT ( 'NONE',  ( -208.1127848780265026, 55.00245453012668406, 2.449293598294708485E-15 ) ) ;
#19642=VERTEX_POINT ( 'NONE', #13982 ) ;
#19643=CARTESIAN_POINT ( 'NONE',  ( -192.9588430854690273, 66.79921049721887982, 10.23066800229522677 ) ) ;
#19644=CARTESIAN_POINT ( 'NONE',  ( -26.85274238233094479, 36.33581074325618232, 15.05078560967874424 ) ) ;
#19645=CARTESIAN_POINT ( 'NONE',  ( 44.82887508595239723, 12.17256213114513130, 38.96139886165431676 ) ) ;
#19646=CARTESIAN_POINT ( 'NONE',  ( -87.10560006382461040, -21.31071338413648064, 2.727320883041552957 ) ) ;
#19647=VERTEX_POINT ( 'NONE', #6013 ) ;
#19648=CARTESIAN_POINT ( 'NONE',  ( -188.3392535381819926, -43.01687576774265409, 23.45796413246070244 ) ) ;
#19650=CARTESIAN_POINT ( 'NONE',  ( 23.72853009152353820, -23.26754081577996658, 42.74808902029987223 ) ) ;
#19651=CARTESIAN_POINT ( 'NONE',  ( 85.88462004898991609, 22.72792989851439316, -10.32535764751219176 ) ) ;
#19653=CARTESIAN_POINT ( 'NONE',  ( -87.12771530791273733, 21.45464684660704791, 1.404361561684027704 ) ) ;
#19654=CARTESIAN_POINT ( 'NONE',  ( -259.2033419157646676, -1.438356298054549103E-14, -9.517827891722632216 ) ) ;
#19655=CARTESIAN_POINT ( 'NONE',  ( -208.1127848780265026, -9.061048840815752106E-14, 15.00245453012669472 ) ) ;
#19657=CARTESIAN_POINT ( 'NONE',  ( 57.59792236341147031, 2.435789363418170872, 40.00000000000002132 ) ) ;
#19658=CARTESIAN_POINT ( 'NONE',  ( -166.3490736462251220, 19.13702016909153514, -36.43932733833390358 ) ) ;
#19660=CARTESIAN_POINT ( 'NONE',  ( -135.8532207217289454, -30.84685318188649106, 40.00000000000002132 ) ) ;
#19661=CARTESIAN_POINT ( 'NONE',  ( 170.2234770963711128, 24.55285855007190321, 0.000000000000000000 ) ) ;
#19662=CARTESIAN_POINT ( 'NONE',  ( -91.56559293963834989, -22.67402823373193499, 40.00000000000002132 ) ) ;
#19663=CARTESIAN_POINT ( 'NONE',  ( -56.48582580120560692, 39.99999999999991473, 9.153146818114004546 ) ) ;
#19664=CARTESIAN_POINT ( 'NONE',  ( -162.0762913951020892, -1.202636532414034422E-14, -1.694272876828323948 ) ) ;
#19665=CARTESIAN_POINT ( 'NONE',  ( -105.3755690713226727, 15.38646221621771737, 15.38646221621800514 ) ) ;
#19666=ORIENTED_EDGE ( 'NONE', *, *, #3474, .F. ) ;
#19668=CARTESIAN_POINT ( 'NONE',  ( 3.774039766332595747, 44.61221010187614411, -18.47898247163319851 ) ) ;
#19669=CARTESIAN_POINT ( 'NONE',  ( -30.26275506840324070, 1.198031551616013601, 1.198031551616023371 ) ) ;
#19670=CARTESIAN_POINT ( 'NONE',  ( -97.73860346100528318, -8.185503821043738526, 20.89580782305262829 ) ) ;
#19671=ORIENTED_EDGE ( 'NONE', *, *, #348, .F. ) ;
#19673=CARTESIAN_POINT ( 'NONE',  ( -94.58366989427237570, 9.000605044545558542, -20.58370269626824367 ) ) ;
#19674=CARTESIAN_POINT ( 'NONE',  ( 156.1979191798867532, 11.34289806466608219, -27.38417834433175102 ) ) ;
#19676=CARTESIAN_POINT ( 'NONE',  ( -105.4741150117398831, -19.77569912955107156, 7.943527260749587704 ) ) ;
#19677=EDGE_LOOP ( 'NONE', ( #26079, #9404, #5968, #14155, #699, #16074 ) ) ;
#19679=CARTESIAN_POINT ( 'NONE',  ( 169.9999999999999716, 21.59613885783086928, 12.70659020859114818 ) ) ;
#19680=CARTESIAN_POINT ( 'NONE',  ( 0.2972598230769907257, 66.70487387989857098, 10.13633138497486641 ) ) ;
#19681=CARTESIAN_POINT ( 'NONE',  ( -109.1264249741457775, -13.72187187121248719, 33.12752917270314867 ) ) ;
#19682=CARTESIAN_POINT ( 'NONE',  ( 199.9999999999999432, 1.065690307512836407E-13, -20.00000000000010303 ) ) ;
#19683=CARTESIAN_POINT ( 'NONE',  ( -199.9999999999999716, -44.96258949770061264, 22.85346793133696153 ) ) ;
#19686=CARTESIAN_POINT ( 'NONE',  ( 14.38125909742181108, 1.616281842095393922E-13, -15.17850393972633682 ) ) ;
#19687=B_SPLINE_CURVE_WITH_KNOTS ( 'NONE', 3,
 ( #18035, #8197, #22450, #4358, #2350, #24030, #12056, #215, #20176, #8459, #22316, #5808, #12192, #26187, #14316, #10463 ),
 .UNSPECIFIED., .F., .F.,
 ( 4, 2, 2, 2, 2, 2, 2, 4 ),
 ( -5.998499567488215554E-08, 0.003520343011582076007, 0.007040746008159827485, 0.01408155200131532524, 0.01760195499789306978, 0.02112235799447082299, 0.02464276099104856926, 0.02816316398762631901 ),
 .UNSPECIFIED. ) ;
#19688=CARTESIAN_POINT ( 'NONE',  ( -198.0356074513804572, -39.99999999999990052, -15.37879056873112482 ) ) ;
#19689=CARTESIAN_POINT ( 'NONE',  ( -110.0791661673102766, -10.82529631553216554, 17.04053483149554182 ) ) ;
#19690=CARTESIAN_POINT ( 'NONE',  ( -135.8532207217289738, 6.472252184284186249, -6.472252184284142729 ) ) ;
#19691=CARTESIAN_POINT ( 'NONE',  ( -200.0000000000000568, 17.27712336974197882, -46.88040655664261891 ) ) ;
#19692=CARTESIAN_POINT ( 'NONE',  ( 151.7948205124836534, -33.06932595376343897, -23.49921654116042902 ) ) ;
#19693=CARTESIAN_POINT ( 'NONE',  ( -103.9474983245025044, 8.027156558344222148, 20.15710290851511033 ) ) ;
#19696=CARTESIAN_POINT ( 'NONE',  ( -135.8532207217289738, 6.472252184284186249, -6.472252184284142729 ) ) ;
#19697=CARTESIAN_POINT ( 'NONE',  ( -30.26275506840324070, -1.147469862568086380E-14, 1.694272468446259783 ) ) ;
#19698=CARTESIAN_POINT ( 'NONE',  ( -198.0356074513804572, 10.87444709758468875, 67.44298959250869530 ) ) ;
#19699=CARTESIAN_POINT ( 'NONE',  ( 151.7948205124836250, -4.785054706301600902, -4.785054706301715477 ) ) ;
#19700=CARTESIAN_POINT ( 'NONE',  ( -173.7925586249088212, -20.60916590992073338, -38.69493321930081464 ) ) ;
#19701=CARTESIAN_POINT ( 'NONE',  ( 12.01676469546555204, 24.84032989753427501, 44.88780742856546624 ) ) ;
#19702=ORIENTED_EDGE ( 'NONE', *, *, #7195, .F. ) ;
#19703=CARTESIAN_POINT ( 'NONE',  ( -100.7734535825088358, 12.25131212657497848, -12.25131212657469604 ) ) ;
#19704=B_SPLINE_CURVE_WITH_KNOTS ( 'NONE', 3,
 ( #22341, #10622, #8484, #24464, #16601, #14343, #6490, #12473 ),
 .UNSPECIFIED., .F., .F.,
 ( 4, 2, 2, 4 ),
 ( -5.298247996846965421E-05, 0.001923793760055677064, 0.003900570000079824073, 0.007854122480128121128 ),
 .UNSPECIFIED. ) ;
#19705=CARTESIAN_POINT ( 'NONE',  ( 169.9999999999999716, -9.369682556672181306, -22.62041470344887273 ) ) ;
#19708=CARTESIAN_POINT ( 'NONE',  ( -82.23726319250467043, 0.6309363043577198571, 20.19517362731287946 ) ) ;
#19710=CARTESIAN_POINT ( 'NONE',  ( 136.1360204305621266, -3.419521671106983309E-13, 35.03383547441296741 ) ) ;
#19712=ADVANCED_FACE ( 'NONE', ( #11992 ), #7881, .T. ) ;
#19715=ORIENTED_EDGE ( 'NONE', *, *, #1929, .F. ) ;
#19716=CARTESIAN_POINT ( 'NONE',  ( 184.8905102610680444, 19.07866798485562398, -40.00000000000002132 ) ) ;
#19717=CARTESIAN_POINT ( 'NONE',  ( -197.4153392275576664, -44.73189834454027647, -24.72549520222428754 ) ) ;
#19718=CARTESIAN_POINT ( 'NONE',  ( -259.2033419157646676, 40.00000000000000711, -9.517827891722491884 ) ) ;
#19723=CARTESIAN_POINT ( 'NONE',  ( 73.43467957758505804, 12.96803903966637961, -26.88835007753401385 ) ) ;
#19724=CARTESIAN_POINT ( 'NONE',  ( 91.82158438592158234, -6.516925787240506436E-14, 22.79471317813470321 ) ) ;
#19726=( BOUNDED_CURVE ( )  B_SPLINE_CURVE ( 3, ( #3655, #5392, #20151, #16016, #5517, #11761, #15871 ),
 .UNSPECIFIED., .F., .F. ) 
 B_SPLINE_CURVE_WITH_KNOTS ( ( 4, 3, 4 ),
 ( 0.007504621739143852409, 0.02318610956072935173, 0.03886759738231801431 ),
 .UNSPECIFIED. ) 
 CURVE ( )  GEOMETRIC_REPRESENTATION_ITEM ( )  RATIONAL_B_SPLINE_CURVE ( ( 0.5852718452494395374, 0.6660804010233950523, 0.8043231192735819102, 1.000000000000000000, 0.8043231192735423862, 0.6660804010233392081, 0.5852718452493905765 ) ) 
 REPRESENTATION_ITEM ( '' )  );
#19727=CARTESIAN_POINT ( 'NONE',  ( 184.8905102610680444, 40.00000000000013500, -20.92133201514430141 ) ) ;
#19729=CARTESIAN_POINT ( 'NONE',  ( -5.866564133087009303, -23.09290806364241533, -42.46617576965061858 ) ) ;
#19730=CARTESIAN_POINT ( 'NONE',  ( 4.995406935893287326, 17.50105314357225694, -39.06748935135176026 ) ) ;
#19731=CARTESIAN_POINT ( 'NONE',  ( -77.70130000790287284, -21.34877220993438485, 5.505113979786321110 ) ) ;
#19732=CARTESIAN_POINT ( 'NONE',  ( -30.26275506840324070, 1.218738420030236455E-14, -1.694272468446259783 ) ) ;
#19734=CARTESIAN_POINT ( 'NONE',  ( 19.06497207195981503, -14.19242893257840166, 0.000000000000000000 ) ) ;
#19735=CARTESIAN_POINT ( 'NONE',  ( 14.38125909742181285, -15.17850393972633505, -40.00000000000002132 ) ) ;
#19736=CARTESIAN_POINT ( 'NONE',  ( 184.8905102610680444, 14.79361573936366092, 41.77492675556006674 ) ) ;
#19737=CARTESIAN_POINT ( 'NONE',  ( -208.1127848780264742, -55.00245453014425578, -40.00000000000002132 ) ) ;
#19738=CARTESIAN_POINT ( 'NONE',  ( -110.0524710260411325, 18.17485046464500442, 8.855238217227519470 ) ) ;
#19739=CARTESIAN_POINT ( 'NONE',  ( -114.7756370326901134, 22.09321776683328764, -1.238720794240111500 ) ) ;
#19740=CARTESIAN_POINT ( 'NONE',  ( -198.0356074513804572, 39.15871834505901461, 39.15871834505919935 ) ) ;
#19741=CARTESIAN_POINT ( 'NONE',  ( 130.8568914410475088, 5.949712681206712261, 40.00000000000002132 ) ) ;
#19743=CARTESIAN_POINT ( 'NONE',  ( 23.64688638900328144, -46.70960658758826867, 13.78084749393243769 ) ) ;
#19744=CARTESIAN_POINT ( 'NONE',  ( 121.8740240556054317, 11.10671848392250638, 26.81399039734629497 ) ) ;
#19745=CARTESIAN_POINT ( 'NONE',  ( -56.48582580120559982, 21.81201906317778594, -34.75652343174606074 ) ) ;
#19746=CARTESIAN_POINT ( 'NONE',  ( -86.96347745069643054, -40.00000000000009948, 18.24025645688337960 ) ) ;
#19747=CARTESIAN_POINT ( 'NONE',  ( 200.0000000000000000, 14.14213562373041455, 42.42640687119311593 ) ) ;
#19748=B_SPLINE_CURVE_WITH_KNOTS ( 'NONE', 3,
 ( #11027, #13025, #19137, #23898, #7531, #26051, #1563, #13653 ),
 .UNSPECIFIED., .F., .F.,
 ( 4, 2, 2, 4 ),
 ( -5.298247996938804799E-05, 0.001923793760048753132, 0.003900570000066894312, 0.007854122480103177539 ),
 .UNSPECIFIED. ) ;
#19749=CARTESIAN_POINT ( 'NONE',  ( 91.82158438592158234, -17.20528682183298486, -40.00000000000002132 ) ) ;
#19752=CARTESIAN_POINT ( 'NONE',  ( -82.24857225180258524, 3.161095685030960833, -19.95174621266928128 ) ) ;
#19753=CARTESIAN_POINT ( 'NONE',  ( 130.8568914410475088, 4.207082182989012153, 52.36146031193425188 ) ) ;
#19754=CARTESIAN_POINT ( 'NONE',  ( -105.3755690713226727, -12.89780903124395550, -12.89780903124416511 ) ) ;
#19756=CARTESIAN_POINT ( 'NONE',  ( -114.5543403404773528, 20.90252105098865698, -6.785539716556657552 ) ) ;
#19757=CARTESIAN_POINT ( 'NONE',  ( -30.26275506840324070, 1.218738420030236455E-14, -1.694272468446259783 ) ) ;
#19758=CARTESIAN_POINT ( 'NONE',  ( -100.7734535825088500, 16.03295912088740494, -40.53558337403661938 ) ) ;
#19759=CARTESIAN_POINT ( 'NONE',  ( -213.1075012329536946, -37.98287015391210275, -37.98287015391272092 ) ) ;
#19760=CARTESIAN_POINT ( 'NONE',  ( -198.0356074513804572, -17.40982414986427429, -39.15871834505933435 ) ) ;
#19761=CARTESIAN_POINT ( 'NONE',  ( 170.2234770963711128, -45.64576402573167258, -10.92277846919254891 ) ) ;
#19762=CARTESIAN_POINT ( 'NONE',  ( 146.6084372240433993, 34.62501878078308692, 0.000000000000000000 ) ) ;
#19764=CARTESIAN_POINT ( 'NONE',  ( 14.38125909742182529, -40.00000000000021316, 55.17850393974251944 ) ) ;
#19765=CARTESIAN_POINT ( 'NONE',  ( 14.38125909742181996, -10.73282306403606157, 67.30136555895948902 ) ) ;
#19767=CARTESIAN_POINT ( 'NONE',  ( 163.1118516004056573, 19.27778845538753316, 19.27778845538783870 ) ) ;
#19769=CARTESIAN_POINT ( 'NONE',  ( 91.82158438592158234, 22.79471317813471742, 40.00000000000002132 ) ) ;
#19771=CARTESIAN_POINT ( 'NONE',  ( -259.2033419157646676, -6.730120644403570829, -6.730120644403545960 ) ) ;
#19772=CARTESIAN_POINT ( 'NONE',  ( 84.01322141327635507, 23.61859044091702131, 9.783140484763423572 ) ) ;
#19773=CARTESIAN_POINT ( 'NONE',  ( 23.49666234703665424, 23.31470603676248032, 42.81942870555097613 ) ) ;
#19774=CARTESIAN_POINT ( 'NONE',  ( -86.96347745069644475, -21.75974354311652093, 40.00000000000002132 ) ) ;
#19776=ORIENTED_EDGE ( 'NONE', *, *, #12467, .T. ) ;
#19777=CARTESIAN_POINT ( 'NONE',  ( -188.3065677117183441, -43.00727648871537667, 23.45084385698005391 ) ) ;
#19781=CARTESIAN_POINT ( 'NONE',  ( 11.71430589699291502, -24.82930166510167069, 44.87285427231071111 ) ) ;
#19782=CARTESIAN_POINT ( 'NONE',  ( 22.89002945277437817, 17.87003923493782764, -43.14209108112063973 ) ) ;
#19785=CARTESIAN_POINT ( 'NONE',  ( -86.86493150571114086, -19.60045294882784717, -8.366608963953355627 ) ) ;
#19786=CARTESIAN_POINT ( 'NONE',  ( 130.8568914410475088, 40.00000000000015632, -34.05028731879774284 ) ) ;
#19789=CARTESIAN_POINT ( 'NONE',  ( -213.1075012329537230, -53.71589010950170717, 40.00000000000002132 ) ) ;
#19790=CARTESIAN_POINT ( 'NONE',  ( -129.2303573020045633, 11.67678754050021617, -24.84170325986431038 ) ) ;
#19793=CARTESIAN_POINT ( 'NONE',  ( -56.48582580120559271, 9.153146818113576444, -0.000000000000000000 ) ) ;
#19794=CARTESIAN_POINT ( 'NONE',  ( 4.995406935893288214, 15.24977328854832770, 40.00000000000002132 ) ) ;
#19795=CARTESIAN_POINT ( 'NONE',  ( 130.8568914410475088, -39.99999999999992895, -5.949712681207114606 ) ) ;
#19796=CARTESIAN_POINT ( 'NONE',  ( -86.96347745069644475, -2.438961472018186339E-13, 21.75974354311649961 ) ) ;
#19797=CARTESIAN_POINT ( 'NONE',  ( -91.56559293963836410, 16.03295912088692177, 16.03295912088721664 ) ) ;
#19798=ADVANCED_FACE ( 'NONE', ( #24573 ), #15049, .T. ) ;
#19801=CARTESIAN_POINT ( 'NONE',  ( 14.38125909742181285, -15.17850393972633505, 0.000000000000000000 ) ) ;
#19803=CARTESIAN_POINT ( 'NONE',  ( -94.58414068594231594, -8.590713000773435581, 20.73981583680210150 ) ) ;
#19808=CARTESIAN_POINT ( 'NONE',  ( -86.86493150571111244, 8.366608963953098055, -19.60045294882791467 ) ) ;
#19809=CARTESIAN_POINT ( 'NONE',  ( 23.32574057153203029, -46.82643129194535447, -13.80366151303456235 ) ) ;
#19811=CARTESIAN_POINT ( 'NONE',  ( 136.1360204305621551, 4.966164525587093870, -40.00000000000002132 ) ) ;
#19812=VERTEX_POINT ( 'NONE', #23083 ) ;
#19815=CARTESIAN_POINT ( 'NONE',  ( 163.1118516004056573, -19.27778845539233998, 37.29075403953149959 ) ) ;
#19819=CARTESIAN_POINT ( 'NONE',  ( 130.8568914410475372, 1.429239637432775288E-13, -34.05028731879788495 ) ) ;
#19821=CARTESIAN_POINT ( 'NONE',  ( -99.21568817060988010, -2.557234656049328691E-13, 22.67402823373191723 ) ) ;
#19823=CARTESIAN_POINT ( 'NONE',  ( -105.2054292635175585, -15.19799821370250825, 15.19799821370211923 ) ) ;
#19824=CARTESIAN_POINT ( 'NONE',  ( -162.0762913951021176, -40.00000000000003553, -1.694272876828743168 ) ) ;
#19825=CARTESIAN_POINT ( 'NONE',  ( -105.2958943009710708, -11.44501736922669366, 18.12177707673897586 ) ) ;
#19826=CARTESIAN_POINT ( 'NONE',  ( -105.3755690713226585, -12.89780903124383471, -43.67073346367985920 ) ) ;
#19827=CARTESIAN_POINT ( 'NONE',  ( 163.1118516004056573, 27.26290988616876021, -40.00000000000002132 ) ) ;
#19828=CARTESIAN_POINT ( 'NONE',  ( -213.1075012329536946, -37.98287015391263566, 37.98287015391218802 ) ) ;
#19829=DIRECTION ( 'NONE',  ( 0.000000000000000000, 0.3995982397413447851, -0.9166903767333977049 ) ) ;
#19831=CARTESIAN_POINT ( 'NONE',  ( 199.9999999999999432, -1.727494763561684666E-13, 20.00000000000010303 ) ) ;
#19832=CARTESIAN_POINT ( 'NONE',  ( 14.38125909742181108, -5.035366881890652543E-14, 15.17850393972633682 ) ) ;
#19833=CARTESIAN_POINT ( 'NONE',  ( 57.59792236341147031, -30.00663442387700641, 26.56190807104681895 ) ) ;
#19834=CARTESIAN_POINT ( 'NONE',  ( 146.6084372240433993, 24.48358557860307272, 24.48358557860347418 ) ) ;
#19835=CARTESIAN_POINT ( 'NONE',  ( -194.4222169614567974, -24.44978956119031466, -44.35789444896748535 ) ) ;
#19836=CARTESIAN_POINT ( 'NONE',  ( -56.48582580120559982, -21.81201906317755501, -34.75652343174621706 ) ) ;
#19838=CARTESIAN_POINT ( 'NONE',  ( -56.48582580120559271, 21.81201906317798489, -21.81201906317746619 ) ) ;
#19839=FACE_OUTER_BOUND ( 'NONE', #5201, .T. ) ;
#19840=CARTESIAN_POINT ( 'NONE',  ( 0.2972598230769983307, -14.33493731733933352, 0.000000000000000000 ) ) ;
#19842=CARTESIAN_POINT ( 'NONE',  ( -200.0000000000000000, 6.162975822039154730E-30, 0.000000000000000000 ) ) ;
#19843=CARTESIAN_POINT ( 'NONE',  ( -56.48582580120559982, -34.75652343174584047, -21.81201906317815187 ) ) ;
#19844=FACE_OUTER_BOUND ( 'NONE', #14977, .T. ) ;
#19846=CARTESIAN_POINT ( 'NONE',  ( -280.0000000000000000, -2.609240458947769655E-13, 20.00000000000001421 ) ) ;
#19848=CARTESIAN_POINT ( 'NONE',  ( -3.615356597031627039, 17.91804473398352471, 43.25798660799035389 ) ) ;
#19851=CARTESIAN_POINT ( 'NONE',  ( -198.0356074513804572, 55.37879056874818673, -40.00000000000002132 ) ) ;
#19852=CARTESIAN_POINT ( 'NONE',  ( 146.6084372240433993, 24.48358557860341733, -24.48358557860313311 ) ) ;
#19853=CARTESIAN_POINT ( 'NONE',  ( 14.38125909742180930, 39.99999999999982947, 55.17850393971022527 ) ) ;
#19854=CARTESIAN_POINT ( 'NONE',  ( -89.91498783735231370, -20.17141720490575452, -8.733585467941317404 ) ) ;
#19857=CARTESIAN_POINT ( 'NONE',  ( 4.995406935893290878, 1.606505379428369110E-13, -15.24977328854832592 ) ) ;
#19859=CARTESIAN_POINT ( 'NONE',  ( -121.8281105897340382, 10.16551987017660252, 22.46071553381061037 ) ) ;
#19860=CARTESIAN_POINT ( 'NONE',  ( -4.201409602818432454, -13.81669219312479058, -46.93439176590607786 ) ) ;
#19862=CARTESIAN_POINT ( 'NONE',  ( -105.3755690713226585, 15.38646221621820764, -41.18208027870583265 ) ) ;
#19863=CARTESIAN_POINT ( 'NONE',  ( -77.55640685876514340, -22.13135000837104371, 0.6996548653676145646 ) ) ;
#19864=CARTESIAN_POINT ( 'NONE',  ( 192.4448373802101173, -42.42640687116490028, -14.14213562375904942 ) ) ;
#19865=CARTESIAN_POINT ( 'NONE',  ( 184.8905102610680444, -40.00000000000021316, 20.92133201514402430 ) ) ;
#19867=CARTESIAN_POINT ( 'NONE',  ( 146.6084372240433993, 34.62501878078308692, 0.000000000000000000 ) ) ;
#19869=CARTESIAN_POINT ( 'NONE',  ( -208.1127848780264742, -15.00245453012673202, 40.00000000000002132 ) ) ;
#19871=EDGE_CURVE ( 'NONE', #162, #19333, #6358, .T. ) ;
#19872=CARTESIAN_POINT ( 'NONE',  ( -135.8532207217289738, 34.75652343174594705, 21.81201906317792449 ) ) ;
#19873=CARTESIAN_POINT ( 'NONE',  ( -91.56559293963834989, -17.32597176626812896, -2.449293598294708485E-15 ) ) ;
#19874=CARTESIAN_POINT ( 'NONE',  ( 21.98945382326337139, -43.25809532770868060, -23.63684424402663709 ) ) ;
#19875=CARTESIAN_POINT ( 'NONE',  ( -114.4098922876147384, 20.15198150140922451, 8.347224046571190215 ) ) ;
#19876=CARTESIAN_POINT ( 'NONE',  ( -259.2033419157646676, 49.83842185052027673, -6.730120644403441155 ) ) ;
#19877=CARTESIAN_POINT ( 'NONE',  ( -198.0356074513804572, 55.37879056874818673, -40.00000000000002132 ) ) ;
#19878=ORIENTED_EDGE ( 'NONE', *, *, #19169, .T. ) ;
#19879=CARTESIAN_POINT ( 'NONE',  ( -77.92915424793434909, 20.15198149301296482, 8.347224043097730473 ) ) ;
#19881=B_SPLINE_CURVE_WITH_KNOTS ( 'NONE', 3,
 ( #7735, #11736, #15989, #21724, #1380, #3499 ),
 .UNSPECIFIED., .F., .F.,
 ( 4, 2, 4 ),
 ( 0.0003134494097674369825, 0.004478637758889606260, 0.008643826108011775158 ),
 .UNSPECIFIED. ) ;
#19882=CARTESIAN_POINT ( 'NONE',  ( -56.48582580120559982, 50.09629031063966664, -6.472252184284094767 ) ) ;
#19883=CARTESIAN_POINT ( 'NONE',  ( 192.4448373802101173, -39.99999999999991473, -20.00000000003956302 ) ) ;
#19884=CARTESIAN_POINT ( 'NONE',  ( -100.7734535825088358, -16.03295912088728770, 16.03295912088687913 ) ) ;
#19886=CARTESIAN_POINT ( 'NONE',  ( 170.2234770963711128, 15.44714144992819627, -40.00000000000002132 ) ) ;
#19891=CARTESIAN_POINT ( 'NONE',  ( -280.0000000000000568, 42.42640687119265408, 14.14213562373147504 ) ) ;
#19892=CARTESIAN_POINT ( 'NONE',  ( 14.38125909742180752, 17.55144818341503665, -39.01709431150898411 ) ) ;
#19894=CARTESIAN_POINT ( 'NONE',  ( -280.0000000000000000, -2.609240458947769655E-13, 20.00000000000001421 ) ) ;
#19895=CARTESIAN_POINT ( 'NONE',  ( -280.0000000000000000, -14.14213562373088706, -14.14213562373108424 ) ) ;
#19896=CARTESIAN_POINT ( 'NONE',  ( 0.2972598230769923355, 18.14793986248751168, -38.42060263243650553 ) ) ;
#19897=CARTESIAN_POINT ( 'NONE',  ( -56.48582580120559271, -6.472252184284276844, 6.472252184284108978 ) ) ;
#19898=CARTESIAN_POINT ( 'NONE',  ( 14.38125909742181463, 10.73282306403652875, -67.30136555895941797 ) ) ;
#19900=CARTESIAN_POINT ( 'NONE',  ( -4.039451493210490796, 46.99046209229823745, -13.82811171175438147 ) ) ;
#19904=CARTESIAN_POINT ( 'NONE',  ( 199.9999999999999432, 1.065690307512836407E-13, -20.00000000000010303 ) ) ;
#19905=CARTESIAN_POINT ( 'NONE',  ( 130.8568914410475088, 24.07718906446891793, 32.49135343045489321 ) ) ;
#19907=CARTESIAN_POINT ( 'NONE',  ( 163.1118516004056573, -27.26290988616869626, 40.00000000000002132 ) ) ;
#19909=CARTESIAN_POINT ( 'NONE',  ( 14.38125909742180397, 67.30136555895953165, 10.73282306403583242 ) ) ;
#19911=CARTESIAN_POINT ( 'NONE',  ( 27.55177309533993579, 13.49150912997473029, 45.29548561695333575 ) ) ;
#19912=CARTESIAN_POINT ( 'NONE',  ( -91.56559293963834989, -22.67402823373193499, 40.00000000000002132 ) ) ;
#19913=EDGE_LOOP ( 'NONE', ( #19389, #22910, #24778, #15209 ) ) ;
#19914=CARTESIAN_POINT ( 'NONE',  ( -188.4265004370476504, -43.04236487214783580, 23.47686928852971278 ) ) ;
#19916=CARTESIAN_POINT ( 'NONE',  ( -4.022465846214261731, -13.82902411340761617, 46.99661175925233891 ) ) ;
#19918=CARTESIAN_POINT ( 'NONE',  ( 23.72853009152652248, 23.26754081577798061, -42.74808902029882773 ) ) ;
#19921=CARTESIAN_POINT ( 'NONE',  ( 192.4448373802100889, 1.051811698935164031E-13, -20.00000000003942091 ) ) ;
#19922=CARTESIAN_POINT ( 'NONE',  ( -100.7734535825088500, -16.03295912088659492, -40.53558337403696044 ) ) ;
#19923=CARTESIAN_POINT ( 'NONE',  ( -198.0356074513804572, -55.37879056874826489, 40.00000000000002132 ) ) ;
#19924=CARTESIAN_POINT ( 'NONE',  ( -173.7925586250955803, 20.60916590995285702, -38.69493321937137154 ) ) ;
#19926=CARTESIAN_POINT ( 'NONE',  ( -56.48582580120559271, 9.153146818113576444, -0.000000000000000000 ) ) ;
#19927=CARTESIAN_POINT ( 'NONE',  ( 200.0000000000000000, 20.00000000000013856, -40.00000000000002132 ) ) ;
#19928=CARTESIAN_POINT ( 'NONE',  ( -135.8532207217289738, -9.153146818113595984, 0.000000000000000000 ) ) ;
#19929=CARTESIAN_POINT ( 'NONE',  ( 170.2234770963711128, -39.99999999999982947, -15.44714144992858529 ) ) ;
#19930=CARTESIAN_POINT ( 'NONE',  ( 57.59792236341147031, -1.493297263419786540E-14, 2.435789363418160658 ) ) ;
#19931=CARTESIAN_POINT ( 'NONE',  ( 199.9999999999999432, 14.14213562373093680, 14.14213562373114641 ) ) ;
#19933=CARTESIAN_POINT ( 'NONE',  ( -65.65550967573776120, 24.04430752631801482, -11.16467289560278786 ) ) ;
#19934=CARTESIAN_POINT ( 'NONE',  ( 199.9999999999999432, 20.00000000000013856, 0.000000000000000000 ) ) ;
#19935=CARTESIAN_POINT ( 'NONE',  ( -99.31364972222458221, -8.164808577129251788, 20.79869444140758361 ) ) ;
#19938=CARTESIAN_POINT ( 'NONE',  ( -162.0762913951020892, -57.76657433524000851, 1.198031840315820329 ) ) ;
#19939=CARTESIAN_POINT ( 'NONE',  ( 25.88393124179782134, -42.08451360835658761, -22.82896322160914693 ) ) ;
#19940=VERTEX_POINT ( 'NONE', #18111 ) ;
#19941=CARTESIAN_POINT ( 'NONE',  ( -86.96347745069644475, 18.24025645688350750, -40.00000000000002132 ) ) ;
#19942=CARTESIAN_POINT ( 'NONE',  ( -96.94449363885364335, -20.74048850981448666, 8.590991630952846236 ) ) ;
#19944=EDGE_LOOP ( 'NONE', ( #1083, #17900, #3485, #20285, #16604, #3608, #5975, #15214, #13551, #6016 ) ) ;
#19947=CARTESIAN_POINT ( 'NONE',  ( -192.9588430854689989, 38.51493924976929861, 38.51493924976947625 ) ) ;
#19948=CARTESIAN_POINT ( 'NONE',  ( -188.6890294954709759, -47.12920239600229166, -13.84869711777369616 ) ) ;
#19949=CARTESIAN_POINT ( 'NONE',  ( 14.38125909742182529, -40.00000000000021316, 55.17850393974251944 ) ) ;
#19950=CARTESIAN_POINT ( 'NONE',  ( -162.0762913951021176, 41.69427287672986182, 40.00000000000002132 ) ) ;
#19952=DIRECTION ( 'NONE',  ( 1.000000000000000000, 0.000000000000000000, 0.000000000000000000 ) ) ;
#19954=CARTESIAN_POINT ( 'NONE',  ( -259.2033419157646676, -40.00000000000003553, -9.517827891722768996 ) ) ;
#19956=CARTESIAN_POINT ( 'NONE',  ( 184.8905102610680444, -39.99999999999978684, -19.07866798485600768 ) ) ;
#19957=CARTESIAN_POINT ( 'NONE',  ( -199.9999999999999147, -49.28189405767606956, -14.17215463606684267 ) ) ;
#19958=CARTESIAN_POINT ( 'NONE',  ( -238.4067589809705794, -0.6820004458488042598, 57.25054294077229855 ) ) ;
#19959=CARTESIAN_POINT ( 'NONE',  ( 184.8905102610680444, 20.92133201514447549, 0.000000000000000000 ) ) ;
#19961=CARTESIAN_POINT ( 'NONE',  ( 19.06497207195982924, -66.60410523465823474, 10.03556273973400081 ) ) ;
#19966=CARTESIAN_POINT ( 'NONE',  ( -30.26275506840324070, 1.218738420030236455E-14, -1.694272468446259783 ) ) ;
#19967=CARTESIAN_POINT ( 'NONE',  ( 4.995406935893297984, -40.00000000000007816, 15.24977328854818914 ) ) ;
#19968=CARTESIAN_POINT ( 'NONE',  ( -213.1075012329537230, 37.98287015391236565, -18.58567234101138510 ) ) ;
#19969=CARTESIAN_POINT ( 'NONE',  ( -114.6128314109029134, 10.93000550580449470, 19.07544683981866029 ) ) ;
#19970=CARTESIAN_POINT ( 'NONE',  ( -188.8384220655410957, -17.93083973458429270, -43.28887647197308297 ) ) ;
#19971=CARTESIAN_POINT ( 'NONE',  ( 146.6084372240433993, 24.48358557860341733, -24.48358557860313311 ) ) ;
#19972=ORIENTED_EDGE ( 'NONE', *, *, #16296, .T. ) ;
#19973=CARTESIAN_POINT ( 'NONE',  ( -213.1075012329537230, -18.58567234101102272, -37.98287015391260013 ) ) ;
#19974=CARTESIAN_POINT ( 'NONE',  ( -114.7827960788993380, 0.6714470530296268169, 22.13220202243102719 ) ) ;
#19975=CARTESIAN_POINT ( 'NONE',  ( -91.56559293963836410, 22.67402823373189946, -0.000000000000000000 ) ) ;
#19977=CARTESIAN_POINT ( 'NONE',  ( 151.7948205124836250, 4.785054706301759886, -4.785054706301612448 ) ) ;
#19978=CARTESIAN_POINT ( 'NONE',  ( -82.24289765308560618, 2.209159509541283040, 20.07413437147899771 ) ) ;
#19979=ORIENTED_EDGE ( 'NONE', *, *, #10379, .T. ) ;
#19981=CARTESIAN_POINT ( 'NONE',  ( -105.2054292635175585, -15.19799821370250825, 15.19799821370211923 ) ) ;
#19982=CARTESIAN_POINT ( 'NONE',  ( -3.977426076245963671, 17.87762021094844656, 43.16039317622611549 ) ) ;
#19983=ORIENTED_EDGE ( 'NONE', *, *, #14445, .T. ) ;
#19984=EDGE_LOOP ( 'NONE', ( #14213, #7695, #10468, #2253, #18642 ) ) ;
#19985=CARTESIAN_POINT ( 'NONE',  ( 0.2972598230769938343, 10.13633138497472252, 10.13633138497475628 ) ) ;
#19988=CARTESIAN_POINT ( 'NONE',  ( -96.94475454971986039, -20.58449551006464162, -9.001119816733867296 ) ) ;
#19991=CARTESIAN_POINT ( 'NONE',  ( 130.8568914410475372, -3.326198072800416995E-13, 34.05028731879788495 ) ) ;
#19993=CARTESIAN_POINT ( 'NONE',  ( -77.55640685891414421, -22.13135000830937926, -1.385220247072852517 ) ) ;
#19996=CARTESIAN_POINT ( 'NONE',  ( -144.0562564040095879, 14.68019406005356586, 29.54282788278102956 ) ) ;
#19997=CARTESIAN_POINT ( 'NONE',  ( 1.925538622596224103, -24.44644315488275055, -44.35335385591496049 ) ) ;
#19998=CARTESIAN_POINT ( 'NONE',  ( -91.56559293963834989, -40.53558337403692491, 16.03295912088671571 ) ) ;
#19999=CARTESIAN_POINT ( 'NONE',  ( -87.13361725327074225, -16.16366093424068495, 14.23233549117614416 ) ) ;
#20000=CARTESIAN_POINT ( 'NONE',  ( 146.6084372240433709, -3.800685668858344801, -52.76785682606520567 ) ) ;
#20001=CARTESIAN_POINT ( 'NONE',  ( -30.26275506840324070, -40.00000000000001421, -1.694272468446678559 ) ) ;
#20002=CARTESIAN_POINT ( 'NONE',  ( -259.2033419157646676, -6.730120644403663199, 6.730120644403451813 ) ) ;
#20003=CARTESIAN_POINT ( 'NONE',  ( -280.0000000000000568, 42.42640687119294540, -14.14213562373059041 ) ) ;
#20004=CARTESIAN_POINT ( 'NONE',  ( -91.56559293963834989, -17.32597176626812896, 40.00000000000002132 ) ) ;
#20005=CARTESIAN_POINT ( 'NONE',  ( -238.4067589809705794, 0.6820004457912851592, -0.6820004457913123597 ) ) ;
#20006=AXIS2_PLACEMENT_3D ( 'NONE', #13707, #25972, #7328 ) ;
#20007=CARTESIAN_POINT ( 'NONE',  ( 130.8568914410475372, -5.949712681206667853, -2.449293598294708485E-15 ) ) ;
#20008=CARTESIAN_POINT ( 'NONE',  ( -114.6863919488549470, 12.18775077807936569, 18.37411471036764965 ) ) ;
#20009=CARTESIAN_POINT ( 'NONE',  ( 184.8905102610680444, 39.99999999999983658, 20.92133201514485563 ) ) ;
#20010=CARTESIAN_POINT ( 'NONE',  ( -198.0356074513804572, 10.87444709759714989, 10.87444709759722450 ) ) ;
#20011=CARTESIAN_POINT ( 'NONE',  ( -86.96347745069644475, -21.75974354311652093, -40.00000000000002132 ) ) ;
#20013=EDGE_CURVE ( 'NONE', #22947, #1902, #26144, .T. ) ;
#20014=( BOUNDED_SURFACE ( )  B_SPLINE_SURFACE ( 3, 3, ( 
 ( #21852, #5621, #7223, #23975, #15714, #1637, #23586, #5751, #21346, #13727, #23711, #11222, #5491, #1124, #13591, #11464, #9478, #3624, #3116, #3240, #11734, #21722, #5238, #19852, #19459, #17846, #17584, #25996, #19335, #9229 ),
 ( #3497, #15339, #19591, #11596, #23467, #13343, #1247, #9351, #17461, #5365, #13470, #21591, #1378, #15857, #24537, #5765, #12152, #13874, #13737, #24400, #21863, #3639, #1917, #20000, #20275, #12283, #16004, #10022, #23986, #24130 ),
 ( #6040, #22277, #24266, #3777, #7745, #2053, #10293, #18132, #8158, #26009, #6166, #9890, #16271, #8020, #22413, #10160, #11746, #26281, #5902, #4189, #26139, #18263, #14010, #45, #14276, #20410, #2184, #17858, #19864, #18400 ),
 ( #177, #4051, #14145, #8283, #16409, #1649, #22139, #9758, #22007, #3920, #12019, #11880, #1786, #17993, #7883, #20139, #16136, #452, #14802, #20672, #18665, #10960, #8555, #849, #22934, #20941, #6293, #8824, #10693, #14666 ),
 ( #18937, #21066, #4445, #10553, #6554, #4714, #12818, #2852, #16671, #6424, #10824, #12678, #14542, #585, #20808, #22804, #24802, #4581, #23073, #8692, #24940, #22672, #2719, #12411, #19067, #2579, #16538, #16801, #8958, #719 ),
 ( #18805, #6688, #16934, #22541, #12538, #25069, #2441, #17067, #6820, #14937, #4844, #14411, #2308, #12950, #4321, #20537, #10416, #18534, #316, #8417, #24668, #13326, #2973, #19570, #13454, #7206, #1361, #25582, #25704, #5102 ),
 ( #11447, #13574, #9460, #21201, #11576, #5345, #5474, #19318, #19696, #25201, #21573, #3221, #15066, #11327, #4977, #17444, #15321, #21447, #17567, #1484, #25326, #3347, #19443, #9084, #7455, #7085, #15570, #1231, #23694, #21701 ) ),
 .UNSPECIFIED., .T., .F., .T. ) 
 B_SPLINE_SURFACE_WITH_KNOTS ( ( 4, 3, 4 ),
 ( 4, 2, 2, 2, 2, 2, 2, 2, 2, 2, 2, 2, 2, 2, 4 ),
 ( 0.000000000000000000, 0.5000000000000000000, 1.000000000000000000 ),
 ( 0.000000000000000000, 0.1357259735107005372, 0.1651108541090157700, 0.1944957347073310028, 0.3598804999793158710, 0.3867117631979620773, 0.4135430264166082281, 0.5789277916885930964, 0.6062785021374117456, 0.6336292125862302838, 0.8508620842112317728, 0.8814014469398914198, 0.9119408096685510667, 0.9559704048342755334, 1.000000000000000000 ),
 .UNSPECIFIED. ) 
 GEOMETRIC_REPRESENTATION_ITEM ( )  RATIONAL_B_SPLINE_SURFACE ( (
 ( 1.000000000000000000, 1.000000000000000000, 1.000000000000000000, 1.000000000000000000, 1.000000000000000000, 1.000000000000000000, 1.000000000000000000, 1.000000000000000000, 1.000000000000000000, 1.000000000000000000, 1.000000000000000000, 1.000000000000000000, 1.000000000000000000, 1.000000000000000000, 1.000000000000000000, 1.000000000000000000, 1.000000000000000000, 1.000000000000000000, 1.000000000000000000, 1.000000000000000000, 1.000000000000000000, 1.000000000000000000, 1.000000000000000000, 1.000000000000000000, 1.000000000000000000, 1.000000000000000000, 1.000000000000000000, 1.000000000000000000, 1.000000000000000000, 1.000000000000000000),
 ( 0.3333333333333333703, 0.3333333333333333703, 0.3333333333333333703, 0.3333333333333333703, 0.3333333333333333703, 0.3333333333333333703, 0.3333333333333333703, 0.3333333333333333703, 0.3333333333333333703, 0.3333333333333333703, 0.3333333333333333703, 0.3333333333333333703, 0.3333333333333333703, 0.3333333333333333703, 0.3333333333333333703, 0.3333333333333333703, 0.3333333333333333703, 0.3333333333333333703, 0.3333333333333333703, 0.3333333333333333703, 0.3333333333333333703, 0.3333333333333333703, 0.3333333333333333703, 0.3333333333333333703, 0.3333333333333333703, 0.3333333333333333703, 0.3333333333333333703, 0.3333333333333333703, 0.3333333333333333703, 0.3333333333333333703),
 ( 0.3333333333333333703, 0.3333333333333333703, 0.3333333333333333703, 0.3333333333333333703, 0.3333333333333333703, 0.3333333333333333703, 0.3333333333333333703, 0.3333333333333333703, 0.3333333333333333703, 0.3333333333333333703, 0.3333333333333333703, 0.3333333333333333703, 0.3333333333333333703, 0.3333333333333333703, 0.3333333333333333703, 0.3333333333333333703, 0.3333333333333333703, 0.3333333333333333703, 0.3333333333333333703, 0.3333333333333333703, 0.3333333333333333703, 0.3333333333333333703, 0.3333333333333333703, 0.3333333333333333703, 0.3333333333333333703, 0.3333333333333333703, 0.3333333333333333703, 0.3333333333333333703, 0.3333333333333333703, 0.3333333333333333703),
 ( 1.000000000000000000, 1.000000000000000000, 1.000000000000000000, 1.000000000000000000, 1.000000000000000000, 1.000000000000000000, 1.000000000000000000, 1.000000000000000000, 1.000000000000000000, 1.000000000000000000, 1.000000000000000000, 1.000000000000000000, 1.000000000000000000, 1.000000000000000000, 1.000000000000000000, 1.000000000000000000, 1.000000000000000000, 1.000000000000000000, 1.000000000000000000, 1.000000000000000000, 1.000000000000000000, 1.000000000000000000, 1.000000000000000000, 1.000000000000000000, 1.000000000000000000, 1.000000000000000000, 1.000000000000000000, 1.000000000000000000, 1.000000000000000000, 1.000000000000000000),
 ( 0.3333333333333333703, 0.3333333333333333703, 0.3333333333333333703, 0.3333333333333333703, 0.3333333333333333703, 0.3333333333333333703, 0.3333333333333333703, 0.3333333333333333703, 0.3333333333333333703, 0.3333333333333333703, 0.3333333333333333703, 0.3333333333333333703, 0.3333333333333333703, 0.3333333333333333703, 0.3333333333333333703, 0.3333333333333333703, 0.3333333333333333703, 0.3333333333333333703, 0.3333333333333333703, 0.3333333333333333703, 0.3333333333333333703, 0.3333333333333333703, 0.3333333333333333703, 0.3333333333333333703, 0.3333333333333333703, 0.3333333333333333703, 0.3333333333333333703, 0.3333333333333333703, 0.3333333333333333703, 0.3333333333333333703),
 ( 0.3333333333333333703, 0.3333333333333333703, 0.3333333333333333703, 0.3333333333333333703, 0.3333333333333333703, 0.3333333333333333703, 0.3333333333333333703, 0.3333333333333333703, 0.3333333333333333703, 0.3333333333333333703, 0.3333333333333333703, 0.3333333333333333703, 0.3333333333333333703, 0.3333333333333333703, 0.3333333333333333703, 0.3333333333333333703, 0.3333333333333333703, 0.3333333333333333703, 0.3333333333333333703, 0.3333333333333333703, 0.3333333333333333703, 0.3333333333333333703, 0.3333333333333333703, 0.3333333333333333703, 0.3333333333333333703, 0.3333333333333333703, 0.3333333333333333703, 0.3333333333333333703, 0.3333333333333333703, 0.3333333333333333703),
 ( 1.000000000000000000, 1.000000000000000000, 1.000000000000000000, 1.000000000000000000, 1.000000000000000000, 1.000000000000000000, 1.000000000000000000, 1.000000000000000000, 1.000000000000000000, 1.000000000000000000, 1.000000000000000000, 1.000000000000000000, 1.000000000000000000, 1.000000000000000000, 1.000000000000000000, 1.000000000000000000, 1.000000000000000000, 1.000000000000000000, 1.000000000000000000, 1.000000000000000000, 1.000000000000000000, 1.000000000000000000, 1.000000000000000000, 1.000000000000000000, 1.000000000000000000, 1.000000000000000000, 1.000000000000000000, 1.000000000000000000, 1.000000000000000000, 1.000000000000000000) ) ) 
 REPRESENTATION_ITEM ( '' )  SURFACE ( )  );
#20015=CARTESIAN_POINT ( 'NONE',  ( 37.15749683988774876, -41.79699086507135775, 12.76981037570783606 ) ) ;
#20017=CARTESIAN_POINT ( 'NONE',  ( 137.0939645874031214, 12.56330697291228837, 30.33050608226204048 ) ) ;
#20018=B_SPLINE_CURVE_WITH_KNOTS ( 'NONE', 3,
 ( #20590, #14199, #4108, #6345, #24725, #10479 ),
 .UNSPECIFIED., .F., .F.,
 ( 4, 2, 4 ),
 ( 0.3689590070116581244, 0.3867117631979620773, 0.4044645193949217843 ),
 .UNSPECIFIED. ) ;
#20019=EDGE_CURVE ( 'NONE', #24743, #12221, #2007, .T. ) ;
#20020=CARTESIAN_POINT ( 'NONE',  ( 57.59792236341147031, 54.84617931850881689, -1.722363176414946073 ) ) ;
#20021=CARTESIAN_POINT ( 'NONE',  ( -238.4067589809705794, -1.892706720741712928E-13, 40.96449427998260973 ) ) ;
#20023=CARTESIAN_POINT ( 'NONE',  ( -192.9588430854690273, 38.51493924976913519, 18.05360324515490333 ) ) ;
#20027=CARTESIAN_POINT ( 'NONE',  ( -280.0000000000000000, -20.00000000000006750, 0.000000000000000000 ) ) ;
#20028=CARTESIAN_POINT ( 'NONE',  ( 170.0000000000000000, 24.95097643317003744, 0.000000000000000000 ) ) ;
#20031=CARTESIAN_POINT ( 'NONE',  ( -208.1127848780265026, 38.89260858015777700, -38.89260858015687461 ) ) ;
#20032=CARTESIAN_POINT ( 'NONE',  ( -208.1127848780264742, -38.89260858015753541, 17.67593391476614784 ) ) ;
#20033=CARTESIAN_POINT ( 'NONE',  ( -198.0012279766650636, -14.15883993157157583, 49.19397028317943210 ) ) ;
#20034=CARTESIAN_POINT ( 'NONE',  ( -82.25678930352327711, 16.86921253968387191, -11.09265870502121309 ) ) ;
#20035=CARTESIAN_POINT ( 'NONE',  ( -105.3755690713226585, -41.18208027870611687, 15.38646221621750954 ) ) ;
#20036=CARTESIAN_POINT ( 'NONE',  ( 91.82158438592159655, -16.11829626346125011, -16.11829626346154853 ) ) ;
#20038=CARTESIAN_POINT ( 'NONE',  ( 170.2234770963711128, -17.36149277826940462, -39.20704971665412586 ) ) ;
#20042=CARTESIAN_POINT ( 'NONE',  ( -135.8532207217289738, -40.00000000000014921, 30.84685318188631697 ) ) ;
#20043=CARTESIAN_POINT ( 'NONE',  ( -208.1127848780265026, -10.60833733269551971, 10.60833733269537049 ) ) ;
#20044=CARTESIAN_POINT ( 'NONE',  ( 170.2234770963711128, 17.36149277826980253, 17.36149277827007253 ) ) ;
#20046=CARTESIAN_POINT ( 'NONE',  ( -135.8532207217289738, -9.153146818113595984, 40.00000000000002132 ) ) ;
#20047=ORIENTED_EDGE ( 'NONE', *, *, #11565, .F. ) ;
#20049=EDGE_CURVE ( 'NONE', #13332, #14842, #20096, .T. ) ;
#20050=CARTESIAN_POINT ( 'NONE',  ( 80.42747805147106988, 24.86641259896651945, 10.30000534605719942 ) ) ;
#20051=CARTESIAN_POINT ( 'NONE',  ( 90.68848816912746713, 8.337973097143857260, 21.47805809253356557 ) ) ;
#20052=CARTESIAN_POINT ( 'NONE',  ( 199.9999999999999432, -20.00000000000006750, 0.000000000000000000 ) ) ;
#20054=CARTESIAN_POINT ( 'NONE',  ( -199.0731274800660628, -44.83667511839421849, 18.57195892574306484 ) ) ;
#20056=CARTESIAN_POINT ( 'NONE',  ( 22.37977766477492381, -23.55755712319357542, 43.15105302556570166 ) ) ;
#20059=CARTESIAN_POINT ( 'NONE',  ( 13.08024833509950824, 18.54957993046981812, -44.78264744455110957 ) ) ;
#20061=AXIS2_PLACEMENT_3D ( 'NONE', #5836, #1716, #14476 ) ;
#20062=CARTESIAN_POINT ( 'NONE',  ( 156.5537079553356250, -27.23618587942440783, 11.28159757857190826 ) ) ;
#20063=CARTESIAN_POINT ( 'NONE',  ( -184.9730489280364338, -22.80026000646345352, 42.02334742177978200 ) ) ;
#20064=CARTESIAN_POINT ( 'NONE',  ( 19.06497207195980792, 66.60410523465830579, -10.03556273973354251 ) ) ;
#20065=CARTESIAN_POINT ( 'NONE',  ( -91.56559293963834989, -17.32597176626812896, 40.00000000000002132 ) ) ;
#20066=CARTESIAN_POINT ( 'NONE',  ( -188.3066136396869297, 23.45085387054259485, -43.00728998844432027 ) ) ;
#20067=CARTESIAN_POINT ( 'NONE',  ( -56.48582580120559982, 21.81201906317729922, 34.75652343174635917 ) ) ;
#20068=CARTESIAN_POINT ( 'NONE',  ( 19.06497207195981503, -14.19242893257840166, 0.000000000000000000 ) ) ;
#20069=CARTESIAN_POINT ( 'NONE',  ( -198.0356074513804572, -15.37879056873074290, -40.00000000000002132 ) ) ;
#20070=CARTESIAN_POINT ( 'NONE',  ( -280.0000000000000568, 19.99999999999995737, 40.00000000000002132 ) ) ;
#20071=CARTESIAN_POINT ( 'NONE',  ( 136.1360204305621266, 7.947488714877270288E-14, -4.966164525587064560 ) ) ;
#20072=CARTESIAN_POINT ( 'NONE',  ( 170.2234770963711128, 10.92277846919201068, 10.92277846919202133 ) ) ;
#20073=CARTESIAN_POINT ( 'NONE',  ( 151.7948205124836250, -3.202120068677277203E-13, 33.23291073765553705 ) ) ;
#20074=CARTESIAN_POINT ( 'NONE',  ( 136.1360204305621266, 53.05693388239320285, -3.511608612530223716 ) ) ;
#20076=CARTESIAN_POINT ( 'NONE',  ( -135.8532207217289738, -6.472252184284190690, -6.472252184284188914 ) ) ;
#20078=CARTESIAN_POINT ( 'NONE',  ( -93.01741312764214342, -8.169811846330309990, 20.82169463875505500 ) ) ;
#20079=PRODUCT_CONTEXT ( 'NONE', #21093, 'mechanical' ) ;
#20080=ORIENTED_EDGE ( 'NONE', *, *, #4556, .F. ) ;
#20082=CARTESIAN_POINT ( 'NONE',  ( 130.8568914410475088, -32.49135343045460900, -24.07718906446924478 ) ) ;
#20083=CARTESIAN_POINT ( 'NONE',  ( 23.36927571439214901, -46.80992244775434585, -13.80130822340160002 ) ) ;
#20084=ORIENTED_EDGE ( 'NONE', *, *, #5807, .T. ) ;
#20085=CARTESIAN_POINT ( 'NONE',  ( -280.0000000000000568, -20.00000000000006750, -40.00000000000002132 ) ) ;
#20090=CARTESIAN_POINT ( 'NONE',  ( 151.7948205124836534, 4.785054706298574878, -51.78348778862537927 ) ) ;
#20091=CARTESIAN_POINT ( 'NONE',  ( -188.3509229510420937, -43.15764231844811150, -17.87648076834712185 ) ) ;
#20092=CARTESIAN_POINT ( 'NONE',  ( -238.4067589809705794, -1.892706720741712928E-13, 40.96449427998260973 ) ) ;
#20093=CARTESIAN_POINT ( 'NONE',  ( 57.59792236341147031, -2.435789363418150444, 0.000000000000000000 ) ) ;
#20096=B_SPLINE_CURVE_WITH_KNOTS ( 'NONE', 3,
 ( #1632, #11861, #1763, #7998, #9871, #7862 ),
 .UNSPECIFIED., .F., .F.,
 ( 4, 2, 4 ),
 ( -6.000000000418191541E-08, 0.04016968421219337809, 0.08033942842438676624 ),
 .UNSPECIFIED. ) ;
#20097=CARTESIAN_POINT ( 'NONE',  ( -162.0762913951021176, -40.00000000000019895, 41.69427287672974813 ) ) ;
#20098=CARTESIAN_POINT ( 'NONE',  ( 19.06497207195981858, -39.99999999999987210, -14.19242893257882621 ) ) ;
#20099=CARTESIAN_POINT ( 'NONE',  ( -105.2109270643165218, -16.13380223201193076, 14.21138704488140192 ) ) ;
#20100=CARTESIAN_POINT ( 'NONE',  ( 192.4448373802100889, -14.14213562370313682, 14.14213562370301958 ) ) ;
#20101=CARTESIAN_POINT ( 'NONE',  ( -162.0762913951020892, -1.694272876828353702, 0.000000000000000000 ) ) ;
#20102=CARTESIAN_POINT ( 'NONE',  ( -238.4067589809705794, -57.25054294065807881, 0.6820004457338858517 ) ) ;
#20105=CARTESIAN_POINT ( 'NONE',  ( 170.2234770963711128, -2.259079968736224833E-13, 24.55285855007187124 ) ) ;
#20106=CARTESIAN_POINT ( 'NONE',  ( -198.0356074513804572, -9.007331120208026888E-14, 15.37879056873070560 ) ) ;
#20107=CARTESIAN_POINT ( 'NONE',  ( -30.26275506840325136, 29.48230279907798135, -27.08623969584585112 ) ) ;
#20109=CARTESIAN_POINT ( 'NONE',  ( -189.2667921706123479, -17.97629039507333104, -43.39860407294602851 ) ) ;
#20112=CARTESIAN_POINT ( 'NONE',  ( 192.4448373802101173, -14.14213562375826605, -42.42640687116518450 ) ) ;
#20113=CARTESIAN_POINT ( 'NONE',  ( -105.4741150117390021, -8.366608964578313490, 19.60045294983322961 ) ) ;
#20114=CARTESIAN_POINT ( 'NONE',  ( -114.5523123854244005, 6.807555700458402193, 20.89198064830843649 ) ) ;
#20115=CARTESIAN_POINT ( 'NONE',  ( -83.21262154144247347, -33.12752917118416462, -13.72187187061500069 ) ) ;
#20116=CARTESIAN_POINT ( 'NONE',  ( 184.8905102610680444, 13.49065550809826952, -13.49065550809790359 ) ) ;
#20117=CARTESIAN_POINT ( 'NONE',  ( -198.9233928135560916, -24.80620717269025732, -44.84148042516699917 ) ) ;
#20118=CARTESIAN_POINT ( 'NONE',  ( -87.10437264496880516, 2.718829733098547585, 21.30276644673244490 ) ) ;
#20121=CARTESIAN_POINT ( 'NONE',  ( -105.4741150117382915, -19.60045294982753461, 8.366608964593266862 ) ) ;
#20122=CARTESIAN_POINT ( 'NONE',  ( -3.993758944537799671, 23.45926997169888040, 43.01863922058791445 ) ) ;
#20123=ORIENTED_EDGE ( 'NONE', *, *, #25999, .T. ) ;
#20125=CARTESIAN_POINT ( 'NONE',  ( 163.1118516004056573, -27.26290988616869626, 0.000000000000000000 ) ) ;
#20128=ADVANCED_FACE ( 'NONE', ( #18512 ), #10804, .T. ) ;
#20129=CARTESIAN_POINT ( 'NONE',  ( -103.9663809733204118, -8.574562931466585880, -19.92521373417671526 ) ) ;
#20130=CARTESIAN_POINT ( 'NONE',  ( -213.1075012329537230, 1.045191102001431893E-13, -13.71589010951911902 ) ) ;
#20135=CARTESIAN_POINT ( 'NONE',  ( -188.3485952524935669, 42.24825774596409644, 17.49980134501263507 ) ) ;
#20136=CARTESIAN_POINT ( 'NONE',  ( -4.558244102846323642, -23.34817229225983581, -42.85231560262757711 ) ) ;
#20137=CARTESIAN_POINT ( 'NONE',  ( 146.6084372240433709, 24.48358557860356655, -32.08495691632035118 ) ) ;
#20138=CARTESIAN_POINT ( 'NONE',  ( -200.0000000000000284, 17.28402242884629914, 46.84854965773176616 ) ) ;
#20139=CARTESIAN_POINT ( 'NONE',  ( 0.2972598230770100991, -38.42060263243686791, 38.42060263243645579 ) ) ;
#20140=CARTESIAN_POINT ( 'NONE',  ( 4.995406935893297984, -39.99999999999986500, -15.24977328854874870 ) ) ;
#20141=FACE_OUTER_BOUND ( 'NONE', #6801, .T. ) ;
#20142=CARTESIAN_POINT ( 'NONE',  ( 14.38125909742182884, -55.17850393971007605, 40.00000000000002132 ) ) ;
#20143=CARTESIAN_POINT ( 'NONE',  ( 170.2234770963711128, 17.36149277827004411, -17.36149277826983095 ) ) ;
#20144=CARTESIAN_POINT ( 'NONE',  ( -259.2033419157646676, -30.48217210827744950, 40.00000000000002132 ) ) ;
#20145=CARTESIAN_POINT ( 'NONE',  ( -110.0692149585521946, 10.04884809978941185, 17.50500459063693626 ) ) ;
#20146=CARTESIAN_POINT ( 'NONE',  ( -86.96347745069645896, 40.00000000000019895, -18.24025645688310249 ) ) ;
#20147=CARTESIAN_POINT ( 'NONE',  ( 200.0000000000000000, 14.14213562373100608, -42.42640687119291698 ) ) ;
#20148=CARTESIAN_POINT ( 'NONE',  ( -238.4067589809705794, 0.9644942799825386714, 0.000000000000000000 ) ) ;
#20149=ORIENTED_EDGE ( 'NONE', *, *, #25230, .F. ) ;
#20150=CARTESIAN_POINT ( 'NONE',  ( -105.3755690713226585, -21.75974354311652448, 40.00000000000002132 ) ) ;
#20151=CARTESIAN_POINT ( 'NONE',  ( -199.9999999999999716, -35.57044988732110369, -42.45148791631905283 ) ) ;
#20152=CARTESIAN_POINT ( 'NONE',  ( -100.7734535825088500, -40.00000000000009948, 17.32597176626796909 ) ) ;
#20153=CARTESIAN_POINT ( 'NONE',  ( 4.995406935893283773, 39.06748935135171052, 17.50105314357239195 ) ) ;
#20154=CARTESIAN_POINT ( 'NONE',  ( 19.06497207195980792, 14.19242893257840876, 0.000000000000000000 ) ) ;
#20155=CARTESIAN_POINT ( 'NONE',  ( -189.2428623074474103, -43.27185639470908285, -23.64699222226066766 ) ) ;
#20160=CARTESIAN_POINT ( 'NONE',  ( -91.56559293963834989, 12.25131212657497848, -12.25131212657469426 ) ) ;
#20161=CARTESIAN_POINT ( 'NONE',  ( -213.1075012329537230, -37.98287015391257881, 18.58567234101111509 ) ) ;
#20162=CARTESIAN_POINT ( 'NONE',  ( -105.2080558454215407, 21.47607500789820278, 1.614329345468047183 ) ) ;
#20163=CARTESIAN_POINT ( 'NONE',  ( -198.0356074513804572, 1.247057299367198800E-13, -15.37879056873070560 ) ) ;
#20164=CARTESIAN_POINT ( 'NONE',  ( -30.26275506840322294, -57.76657404653985139, -1.198031551616531853 ) ) ;
#20165=CARTESIAN_POINT ( 'NONE',  ( -87.13361725327075646, 14.71749760136616558, -15.67849882405064932 ) ) ;
#20166=CARTESIAN_POINT ( 'NONE',  ( 136.1360204305621551, -24.77266263493081766, -31.79587985999290112 ) ) ;
#20167=CARTESIAN_POINT ( 'NONE',  ( -100.7734535825088500, 16.03295912088713848, -16.03295912088698927 ) ) ;
#20170=CARTESIAN_POINT ( 'NONE',  ( -30.26275506840323359, -40.00000000000017053, 41.69427246844613677 ) ) ;
#20171=CARTESIAN_POINT ( 'NONE',  ( 19.06497207195981147, -10.03556273973425483, -10.03556273973443247 ) ) ;
#20173=CARTESIAN_POINT ( 'NONE',  ( 23.64688638900461015, 42.77321027809668408, -23.28414885118040445 ) ) ;
#20174=CARTESIAN_POINT ( 'NONE',  ( 0.2972598230769930572, 54.33493731733936016, 2.449293598294708485E-15 ) ) ;
#20176=CARTESIAN_POINT ( 'NONE',  ( 7.340276910564544011, -24.82763627182848154, -44.87059041559408001 ) ) ;
#20177=CARTESIAN_POINT ( 'NONE',  ( 20.31814284189117004, 42.80521382620615611, 17.73050010709527768 ) ) ;
#20179=CARTESIAN_POINT ( 'NONE',  ( 184.8905102610680444, -20.92133201514440799, 0.000000000000000000 ) ) ;
#20180=ORIENTED_EDGE ( 'NONE', *, *, #536, .T. ) ;
#20181=CARTESIAN_POINT ( 'NONE',  ( -189.1288337602814238, -47.28029723722803368, 13.87115233298298733 ) ) ;
#20183=CARTESIAN_POINT ( 'NONE',  ( 9.345847406360801912, -24.85453859511385488, 44.90706793518310036 ) ) ;
#20185=CARTESIAN_POINT ( 'NONE',  ( 21.80484139881497185, 17.98806631651988397, -43.42703366220747085 ) ) ;
#20187=CARTESIAN_POINT ( 'NONE',  ( 164.1122551457365546, -24.38379312608502403, 10.10009781492401082 ) ) ;
#20188=CARTESIAN_POINT ( 'NONE',  ( -188.3509229510694638, -17.87648076834458521, 43.15764231845329846 ) ) ;
#20189=ADVANCED_FACE ( 'NONE', ( #18914 ), #24215, .T. ) ;
#20190=CARTESIAN_POINT ( 'NONE',  ( -100.7734535825088358, 12.25131212657497848, -12.25131212657469604 ) ) ;
#20191=CARTESIAN_POINT ( 'NONE',  ( -213.1075012329537230, -13.71589010951915810, 0.000000000000000000 ) ) ;
#20194=CARTESIAN_POINT ( 'NONE',  ( -188.4702232936889459, 13.83721295434279774, -47.05182887786761370 ) ) ;
#20195=CARTESIAN_POINT ( 'NONE',  ( 130.8568914410475372, -24.07718906447255947, 24.07718906447199458 ) ) ;
#20196=CARTESIAN_POINT ( 'NONE',  ( -114.4364955367327070, 8.644468109209567430, -20.04994829327642947 ) ) ;
#20197=B_SPLINE_CURVE_WITH_KNOTS ( 'NONE', 3,
 ( #22033, #25896, #16028, #26034, #20033, #9515 ),
 .UNSPECIFIED., .F., .F.,
 ( 4, 2, 4 ),
 ( -5.998616628085171876E-08, 0.005995031700373180950, 0.01199012338691264265 ),
 .UNSPECIFIED. ) ;
#20198=CARTESIAN_POINT ( 'NONE',  ( 0.2972598230769983307, -14.33493731733933352, -40.00000000000002132 ) ) ;
#20199=CARTESIAN_POINT ( 'NONE',  ( 199.9999999999999432, 19.99999999999996092, 2.449293598294708485E-15 ) ) ;
#20200=CARTESIAN_POINT ( 'NONE',  ( -91.56559293963834989, 1.671088883502053755E-13, -17.32597176626811120 ) ) ;
#20201=CARTESIAN_POINT ( 'NONE',  ( -259.2033419157646676, 49.83842185052027673, -6.730120644403441155 ) ) ;
#20202=CARTESIAN_POINT ( 'NONE',  ( 98.29820294267166503, -13.21553301705472627, 15.06873823041648031 ) ) ;
#20203=CARTESIAN_POINT ( 'NONE',  ( 192.4448373802100889, 14.14213562375873678, 14.14213562375894817 ) ) ;
#20204=EDGE_CURVE ( 'NONE', #10094, #23960, #16917, .T. ) ;
#20205=EDGE_CURVE ( 'NONE', #4362, #23332, #22322, .T. ) ;
#20206=ORIENTED_EDGE ( 'NONE', *, *, #12873, .T. ) ;
#20207=CARTESIAN_POINT ( 'NONE',  ( 151.7948205124836250, -23.49921654116339553, -23.49921654116350211 ) ) ;
#20208=CARTESIAN_POINT ( 'NONE',  ( -96.94449363882321791, -8.590991630976864357, 20.74048850979724534 ) ) ;
#20211=ORIENTED_EDGE ( 'NONE', *, *, #14818, .T. ) ;
#20212=CARTESIAN_POINT ( 'NONE',  ( 136.1360204305621551, -31.79587985999244282, -24.77266263493140386 ) ) ;
#20213=CARTESIAN_POINT ( 'NONE',  ( 37.37129771729572525, -38.51719860174896581, -20.48130208320684531 ) ) ;
#20215=CARTESIAN_POINT ( 'NONE',  ( 192.4448373802101173, -20.00000000003938538, -40.00000000000002132 ) ) ;
#20216=CARTESIAN_POINT ( 'NONE',  ( -103.9650464694730374, -20.03380587394293144, 8.298274102034335797 ) ) ;
#20217=EDGE_LOOP ( 'NONE', ( #23336, #26227, #12723, #9311 ) ) ;
#20219=AXIS2_PLACEMENT_3D ( 'NONE', #9749, #11869, #23471 ) ;
#20221=CARTESIAN_POINT ( 'NONE',  ( -105.3841539895568786, 20.33898584361668682, -6.698820788730287745 ) ) ;
#20222=CARTESIAN_POINT ( 'NONE',  ( -56.48582580120559271, -6.472252184284187138, -6.472252184284199572 ) ) ;
#20223=CARTESIAN_POINT ( 'NONE',  ( -188.2652746676488960, -42.99511404081843580, -23.44263257803740785 ) ) ;
#20224=CARTESIAN_POINT ( 'NONE',  ( -86.96347745069643054, -39.99999999999995737, -21.75974354311664527 ) ) ;
#20225=CARTESIAN_POINT ( 'NONE',  ( -91.56559293963834989, -22.67402823373193499, 0.000000000000000000 ) ) ;
#20229=CARTESIAN_POINT ( 'NONE',  ( 57.59792236341147031, 1.908507979671054758E-14, -2.435789363418160658 ) ) ;
#20230=CARTESIAN_POINT ( 'NONE',  ( 146.6084372240433993, 5.715592784339989804E-15, 5.374981219216972583 ) ) ;
#20231=CARTESIAN_POINT ( 'NONE',  ( -105.3755690713226727, -2.472783935621397949E-13, 21.75974354311649961 ) ) ;
#20232=CARTESIAN_POINT ( 'NONE',  ( 163.1118516004056573, 40.00000000000014921, -27.26290988616858968 ) ) ;
#20233=CARTESIAN_POINT ( 'NONE',  ( -208.1127848780265026, -15.00245453012673202, 0.000000000000000000 ) ) ;
#20234=CARTESIAN_POINT ( 'NONE',  ( 199.9999999999999432, -14.14213562373093680, 14.14213562373082311 ) ) ;
#20235=CARTESIAN_POINT ( 'NONE',  ( -280.0000000000000000, 19.99999999999996092, -0.000000000000000000 ) ) ;
#20236=CARTESIAN_POINT ( 'NONE',  ( -259.2033419157646676, -21.55415060305824326, -35.01439189186556433 ) ) ;
#20237=CARTESIAN_POINT ( 'NONE',  ( -97.72675010090208048, -8.987772175319811652, 20.56394680065903202 ) ) ;
#20238=CARTESIAN_POINT ( 'NONE',  ( 23.09931156284630305, -46.91113948292957758, 13.81622350327238458 ) ) ;
#20239=CARTESIAN_POINT ( 'NONE',  ( -30.26275506840325136, 40.00000000000003553, -1.694272468445841007 ) ) ;
#20240=CARTESIAN_POINT ( 'NONE',  ( -56.48582580120558561, -1.205267837095813407E-13, 30.84685318188644132 ) ) ;
#20241=CARTESIAN_POINT ( 'NONE',  ( 163.1118516004056573, 9.006482792069629539, 9.006482792069634868 ) ) ;
#20242=AXIS2_PLACEMENT_3D ( 'NONE', #14251, #10000, #23966 ) ;
#20243=CARTESIAN_POINT ( 'NONE',  ( -114.6329851429147482, 11.24672612388742543, 18.91064981619980756 ) ) ;
#20244=CARTESIAN_POINT ( 'NONE',  ( -189.0115661350361336, -17.94954792649098607, -43.33404204260301640 ) ) ;
#20245=CARTESIAN_POINT ( 'NONE',  ( -56.48582580120559271, 6.472252184284211118, -6.472252184284153387 ) ) ;
#20247=CARTESIAN_POINT ( 'NONE',  ( 4.995406935893289102, 10.78321810389013002, -10.78321810388986712 ) ) ;
#20249=CARTESIAN_POINT ( 'NONE',  ( -213.1075012329537230, -13.71589010951915810, -40.00000000000002132 ) ) ;
#20250=CARTESIAN_POINT ( 'NONE',  ( 151.7948205124836534, -23.49921654115981084, -33.06932595376387951 ) ) ;
#20251=CARTESIAN_POINT ( 'NONE',  ( -77.78745312868143458, 6.815361097864228945, 20.88824371463043761 ) ) ;
#20254=CARTESIAN_POINT ( 'NONE',  ( -16.41594856591132157, -21.03672847018052394, -39.35878123509505855 ) ) ;
#20255=CARTESIAN_POINT ( 'NONE',  ( -4.037857402786209526, 23.44963359339744002, 43.00569567200292198 ) ) ;
#20256=AXIS2_PLACEMENT_3D ( 'NONE', #9323, #25443, #5091 ) ;
#20257=ORIENTED_EDGE ( 'NONE', *, *, #11744, .T. ) ;
#20258=CIRCLE ( 'NONE', #23639, 15.00000000000000000 ) ;
#20260=CARTESIAN_POINT ( 'NONE',  ( 192.4448373802101173, -20.00000000003938538, -40.00000000000002132 ) ) ;
#20263=CARTESIAN_POINT ( 'NONE',  ( 98.29820294270297154, 18.47759065022021474, -7.653668647299666894 ) ) ;
#20264=CARTESIAN_POINT ( 'NONE',  ( -105.4732637872235443, -8.153770687239559223, -19.68494377761379610 ) ) ;
#20265=CARTESIAN_POINT ( 'NONE',  ( -30.26275506840325136, 40.00000000000003553, -1.694272468445841007 ) ) ;
#20267=CARTESIAN_POINT ( 'NONE',  ( -77.90255099906771363, -20.29001641120656174, -8.064892378658559124 ) ) ;
#20268=CARTESIAN_POINT ( 'NONE',  ( -114.7826396787322665, -15.64922767586156915, -15.64922767586183383 ) ) ;
#20270=FACE_OUTER_BOUND ( 'NONE', #13216, .T. ) ;
#20271=CARTESIAN_POINT ( 'NONE',  ( 8.209392600928307360, -24.84362085272598364, -44.89226883836247595 ) ) ;
#20272=CARTESIAN_POINT ( 'NONE',  ( 146.6084372240433993, -3.800685668858596156, -3.800685668858692967 ) ) ;
#20274=CARTESIAN_POINT ( 'NONE',  ( -114.7544849858170721, 2.764938904914928219, -21.97700360082519566 ) ) ;
#20275=CARTESIAN_POINT ( 'NONE',  ( 151.7948205124835681, -4.785054706298153882, -51.78348778862540058 ) ) ;
#20276=CARTESIAN_POINT ( 'NONE',  ( -192.9588430854690273, -39.99999999999991473, -14.46834944100011633 ) ) ;
#20278=CARTESIAN_POINT ( 'NONE',  ( -259.2033419157646676, 9.517827891722582478, 40.00000000000002132 ) ) ;
#20280=CARTESIAN_POINT ( 'NONE',  ( 4.995406935893307754, -55.24977328853207581, -40.00000000000002132 ) ) ;
#20281=CARTESIAN_POINT ( 'NONE',  ( -110.0568454066791730, 9.184575013437996205, 17.97667584252678807 ) ) ;
#20282=CARTESIAN_POINT ( 'NONE',  ( -208.1127848780265026, 5.403397259664334602E-13, -55.00245453012672670 ) ) ;
#20283=CARTESIAN_POINT ( 'NONE',  ( -91.56559293963834989, 12.25131212657490209, -44.31723036834897300 ) ) ;
#20284=CARTESIAN_POINT ( 'NONE',  ( -213.1075012329537230, 13.71589010951907994, 0.000000000000000000 ) ) ;
#20285=ORIENTED_EDGE ( 'NONE', *, *, #8162, .T. ) ;
#20286=ORIENTED_EDGE ( 'NONE', *, *, #22352, .F. ) ;
#20287=CARTESIAN_POINT ( 'NONE',  ( 192.4448373802101173, -20.00000000003938538, 40.00000000000002132 ) ) ;
#20288=CARTESIAN_POINT ( 'NONE',  ( -102.4068193528146651, -8.088405365068982888, -20.44188272012847918 ) ) ;
#20289=CARTESIAN_POINT ( 'NONE',  ( 151.7948205124836534, -40.00000000000001421, 6.767089262348889633 ) ) ;
#20290=CARTESIAN_POINT ( 'NONE',  ( -192.9588430854690273, 66.79921049724377724, -10.23066800231904239 ) ) ;
#20291=CARTESIAN_POINT ( 'NONE',  ( 192.4448373802100889, -20.00000000003938538, 0.000000000000000000 ) ) ;
#20292=EDGE_CURVE ( 'NONE', #21913, #9180, #11939, .T. ) ;
#20294=CARTESIAN_POINT ( 'NONE',  ( -188.2995950289365226, 23.44932284465886241, 43.00522595870971543 ) ) ;
#20298=CARTESIAN_POINT ( 'NONE',  ( -280.0000000000000568, -14.14213562373049449, -42.42640687119305198 ) ) ;
#20299=CARTESIAN_POINT ( 'NONE',  ( -105.3755690713226585, -41.18208027870611687, 15.38646221621750954 ) ) ;
#20300=CARTESIAN_POINT ( 'NONE',  ( -114.7464620073225348, 21.93325705637180079, 3.051371648169525663 ) ) ;
#20301=CARTESIAN_POINT ( 'NONE',  ( 0.2972598230769957217, 1.502051041545559470E-13, -14.33493731733933352 ) ) ;
#20302=CARTESIAN_POINT ( 'NONE',  ( -238.4067589809705794, -57.25054294077233408, -0.6820004458489551391 ) ) ;
#20303=CARTESIAN_POINT ( 'NONE',  ( 130.8568914410475372, -24.07718906447255947, 24.07718906447199458 ) ) ;
#20304=CARTESIAN_POINT ( 'NONE',  ( 184.8905102610680444, -14.79361573936379415, -14.79361573936387941 ) ) ;
#20305=CARTESIAN_POINT ( 'NONE',  ( -56.48582580120559982, -21.81201906317755501, -34.75652343174621706 ) ) ;
#20307=EDGE_CURVE ( 'NONE', #12520, #3292, #11494, .T. ) ;
#20309=CARTESIAN_POINT ( 'NONE',  ( 163.1118516004056573, -1.695744499706194789E-14, 12.73709011382475254 ) ) ;
#20311=CARTESIAN_POINT ( 'NONE',  ( 23.49666234703892442, 46.76389514419409466, -13.79192166426290633 ) ) ;
#20312=CARTESIAN_POINT ( 'NONE',  ( -86.96347745069644475, 18.24025645688350750, -40.00000000000002132 ) ) ;
#20315=B_SPLINE_CURVE_WITH_KNOTS ( 'NONE', 3,
 ( #15138, #10899, #25398, #19392, #25267, #1046 ),
 .UNSPECIFIED., .F., .F.,
 ( 4, 2, 4 ),
 ( 3.836816584462350783E-15, 0.03937634048171193696, 0.07875268096342002977 ),
 .UNSPECIFIED. ) ;
#20316=CARTESIAN_POINT ( 'NONE',  ( -8.197988474474012577, -42.01088836872121135, 17.40147972967339385 ) ) ;
#20317=CARTESIAN_POINT ( 'NONE',  ( -238.4067589809705794, 0.9644942799825385604, 40.00000000000002132 ) ) ;
#20321=CARTESIAN_POINT ( 'NONE',  ( 22.01478053667031176, -23.63228119973013008, 43.25192662397473953 ) ) ;
#20322=CARTESIAN_POINT ( 'NONE',  ( 19.66474694218035424, 18.18658454059308482, -43.90629905111418196 ) ) ;
#20324=CARTESIAN_POINT ( 'NONE',  ( -90.07798792367799479, -15.74993999324200011, 15.74993999324160399 ) ) ;
#20326=CARTESIAN_POINT ( 'NONE',  ( -129.2303573020127772, -9.309001178986628489, 25.82247248359045599 ) ) ;
#20327=CARTESIAN_POINT ( 'NONE',  ( -56.48582580120559982, 50.09629031063956717, 6.472252184284792875 ) ) ;
#20328=CARTESIAN_POINT ( 'NONE',  ( 170.0000000000000000, 24.95097643317003744, 0.000000000000000000 ) ) ;
#20329=CARTESIAN_POINT ( 'NONE',  ( -189.1816166312696623, 17.96744819725043385, -43.37725711903431858 ) ) ;
#20330=CARTESIAN_POINT ( 'NONE',  ( -213.1075012329537230, 37.98287015391211696, 18.58567234101190735 ) ) ;
#20331=CARTESIAN_POINT ( 'NONE',  ( 136.1360204305621266, 35.03383547441298873, 0.000000000000000000 ) ) ;
#20332=CARTESIAN_POINT ( 'NONE',  ( 130.8568914410475372, -5.949712681206667853, -2.449293598294708485E-15 ) ) ;
#20333=CARTESIAN_POINT ( 'NONE',  ( -280.0000000000000568, 19.99999999999996447, -40.00000000000002132 ) ) ;
#20334=CARTESIAN_POINT ( 'NONE',  ( -208.1127848780264742, -39.99999999999948841, -55.00245453010965235 ) ) ;
#20335=CARTESIAN_POINT ( 'NONE',  ( -280.0000000000000000, 14.14213562373088351, 14.14213562373098654 ) ) ;
#20336=CARTESIAN_POINT ( 'NONE',  ( -99.31364972220157483, 20.48028939131803128, -8.933506367388797997 ) ) ;
#20337=CARTESIAN_POINT ( 'NONE',  ( 163.1118516004056573, 47.56205970284970164, -9.006482792073828847 ) ) ;
#20339=CARTESIAN_POINT ( 'NONE',  ( -56.48582580120559982, -34.75652343174615311, 21.81201906317766870 ) ) ;
#20340=CARTESIAN_POINT ( 'NONE',  ( -100.0957100001695608, 8.517115559328161112, 20.56213589534488406 ) ) ;
#20342=ORIENTED_EDGE ( 'NONE', *, *, #17291, .F. ) ;
#20343=ORIENTED_EDGE ( 'NONE', *, *, #12467, .F. ) ;
#20344=CARTESIAN_POINT ( 'NONE',  ( 136.1360204305621266, -3.511608612530379592, -53.05693388239318153 ) ) ;
#20345=CARTESIAN_POINT ( 'NONE',  ( 67.90397382963038808, -30.27708616532465413, -10.29861769453878040 ) ) ;
#20346=ORIENTED_EDGE ( 'NONE', *, *, #5308, .T. ) ;
#20347=CARTESIAN_POINT ( 'NONE',  ( -192.9588430854689989, 14.46834944099965981, 0.000000000000000000 ) ) ;
#20348=CARTESIAN_POINT ( 'NONE',  ( -99.21568817060988010, -16.03295912088706743, -16.03295912088710296 ) ) ;
#20351=ORIENTED_EDGE ( 'NONE', *, *, #4311, .F. ) ;
#20354=CARTESIAN_POINT ( 'NONE',  ( 4.995406935893283773, 39.06748935135195211, -17.50105314357185193 ) ) ;
#20356=CARTESIAN_POINT ( 'NONE',  ( -188.3611024622295815, -47.01268868735291306, -13.83140737835780953 ) ) ;
#20357=CARTESIAN_POINT ( 'NONE',  ( 19.06497207195982924, -40.00000000000021316, 54.19242893257830218 ) ) ;
#20358=CARTESIAN_POINT ( 'NONE',  ( -30.26275506840324425, 1.694272468446254232, 40.00000000000002132 ) ) ;
#20362=CARTESIAN_POINT ( 'NONE',  ( 199.9999999999999432, 1.065690307512836407E-13, -20.00000000000010303 ) ) ;
#20363=CARTESIAN_POINT ( 'NONE',  ( -280.0000000000000568, -40.00000000000014211, 19.99999999999987210 ) ) ;
#20364=CARTESIAN_POINT ( 'NONE',  ( -105.3755690713226727, 5.661656051307470077E-14, -21.75974354311649961 ) ) ;
#20365=CARTESIAN_POINT ( 'NONE',  ( -91.56559293963836410, 22.67402823373189946, -0.000000000000000000 ) ) ;
#20366=CARTESIAN_POINT ( 'NONE',  ( -192.9588430854690273, -10.23066800229550388, 66.79921049721887982 ) ) ;
#20367=CARTESIAN_POINT ( 'NONE',  ( 200.0000000000000000, 20.00000000000013856, -40.00000000000002132 ) ) ;
#20368=CARTESIAN_POINT ( 'NONE',  ( -280.0000000000000568, 14.14213562373067745, 42.42640687119295251 ) ) ;
#20371=CARTESIAN_POINT ( 'NONE',  ( -238.4067589809705794, -3.369206980223063916E-14, -0.9644942799825824142 ) ) ;
#20372=CARTESIAN_POINT ( 'NONE',  ( -56.48582580120557850, -40.00000000000014211, 30.84685318188629921 ) ) ;
#20373=CARTESIAN_POINT ( 'NONE',  ( 91.82158438592158234, 44.40256751092336884, -12.16597498400043342 ) ) ;
#20374=CARTESIAN_POINT ( 'NONE',  ( 170.2234770963711128, 17.36149277826980253, 17.36149277827007253 ) ) ;
#20375=CARTESIAN_POINT ( 'NONE',  ( -189.0540493709920611, -17.95404051684892011, -43.34488811517432794 ) ) ;
#20376=CARTESIAN_POINT ( 'NONE',  ( 57.59792236341148453, -54.84617931850877426, -1.722363176415331099 ) ) ;
#20377=ORIENTED_EDGE ( 'NONE', *, *, #18676, .T. ) ;
#20379=CARTESIAN_POINT ( 'NONE',  ( 184.8905102610680444, -14.79361573936330565, -41.77492675556016621 ) ) ;
#20380=CARTESIAN_POINT ( 'NONE',  ( -85.37145963729155085, 19.33814434286730588, 8.010121657944045737 ) ) ;
#20381=CARTESIAN_POINT ( 'NONE',  ( -135.8532207217289738, 9.153146818113548022, -40.00000000000002132 ) ) ;
#20383=CARTESIAN_POINT ( 'NONE',  ( 0.2972598230769938343, 10.13633138497486286, -10.13633138497461594 ) ) ;
#20384=B_SPLINE_CURVE_WITH_KNOTS ( 'NONE', 3,
 ( #26244, #7979, #1745, #24228, #4013, #20237, #1615, #2018, #6128, #22376, #8651, #16502 ),
 .UNSPECIFIED., .F., .F.,
 ( 4, 2, 2, 2, 2, 4 ),
 ( 1.597743418105305181E-15, 0.004698945756008282397, 0.007048418634011624322, 0.009397891512014965379, 0.01409683726802164923, 0.01879578302402833134 ),
 .UNSPECIFIED. ) ;
#20388=B_SPLINE_CURVE_WITH_KNOTS ( 'NONE', 3,
 ( #6952, #13088, #23699, #11581, #1236, #3104 ),
 .UNSPECIFIED., .F., .F.,
 ( 4, 2, 4 ),
 ( 0.0003134736701598289828, 0.004478999675054296317, 0.008644525679948764085 ),
 .UNSPECIFIED. ) ;
#20390=CARTESIAN_POINT ( 'NONE',  ( -2.557884977177247610, 13.90734923101136111, 47.52441970261063631 ) ) ;
#20396=CARTESIAN_POINT ( 'NONE',  ( -114.6380899717675987, -5.502349596714755542, -21.35059266670068467 ) ) ;
#20401=CARTESIAN_POINT ( 'NONE',  ( -238.4067589809705794, 3.877349844572403567E-13, -40.96449427998260973 ) ) ;
#20403=CARTESIAN_POINT ( 'NONE',  ( 169.9999999999999432, 6.285860131565304876, -24.25569233607180308 ) ) ;
#20404=CARTESIAN_POINT ( 'NONE',  ( 23.37394308801977871, -42.85717664514601921, 23.33966569535066071 ) ) ;
#20407=CARTESIAN_POINT ( 'NONE',  ( -4.260882601031172889, -23.40615483283773557, -42.93997571557876114 ) ) ;
#20408=CARTESIAN_POINT ( 'NONE',  ( -56.48582580120558561, -50.09629031063971638, 6.472252184283745713 ) ) ;
#20409=CARTESIAN_POINT ( 'NONE',  ( -199.9999999999999432, 14.17215463606929227, 49.28189405767592746 ) ) ;
#20410=CARTESIAN_POINT ( 'NONE',  ( 163.1118516004056573, -37.29075403953139300, -19.27778845539249630 ) ) ;
#20411=CARTESIAN_POINT ( 'NONE',  ( 98.29820294270304259, -18.47759065022024672, 7.653668647299475047 ) ) ;
#20413=CARTESIAN_POINT ( 'NONE',  ( 163.1118516004056573, -12.73709011382472589, 40.00000000000002132 ) ) ;
#20414=CARTESIAN_POINT ( 'NONE',  ( 170.0000000000428315, 17.64300463311351308, -17.64300463311329992 ) ) ;
#20415=CARTESIAN_POINT ( 'NONE',  ( -198.0356074513804288, -55.37879056873077133, -2.449293598294708485E-15 ) ) ;
#20416=CARTESIAN_POINT ( 'NONE',  ( -96.93773665438794751, 20.92028269119439443, -8.190703376740675168 ) ) ;
#20417=CARTESIAN_POINT ( 'NONE',  ( -135.8532207217289738, 39.99999999999990763, 9.153146818113990335 ) ) ;
#20418=CARTESIAN_POINT ( 'NONE',  ( 57.59792236341147031, 26.56190807104693619, -30.00663442387692115 ) ) ;
#20419=CARTESIAN_POINT ( 'NONE',  ( 4.995406935893288214, 15.24977328854832770, -40.00000000000002132 ) ) ;
#20422=CARTESIAN_POINT ( 'NONE',  ( 151.7948205124836250, -33.23291073765550863, 0.000000000000000000 ) ) ;
#20423=CARTESIAN_POINT ( 'NONE',  ( -100.7734535825088358, 12.25131212657497848, -12.25131212657469604 ) ) ;
#20424=CARTESIAN_POINT ( 'NONE',  ( 136.1360204305621266, -35.03383547441293899, 0.000000000000000000 ) ) ;
#20426=CARTESIAN_POINT ( 'NONE',  ( -188.2995950289364373, 13.82811170417284075, -46.99046209955416487 ) ) ;
#20429=CARTESIAN_POINT ( 'NONE',  ( -208.1127848780264742, 67.17687982763172272, -10.60833733270698254 ) ) ;
#20430=CARTESIAN_POINT ( 'NONE',  ( 184.8905102610680444, -13.49065550809791603, -13.49065550809818781 ) ) ;
#20432=CARTESIAN_POINT ( 'NONE',  ( 0.2972598230769956662, 40.00000000000058975, -54.33493731733894094 ) ) ;
#20433=CARTESIAN_POINT ( 'NONE',  ( 184.8905102610680444, -41.77492675556007384, 14.79361573936348684 ) ) ;
#20436=CARTESIAN_POINT ( 'NONE',  ( -175.9235640290363563, -21.03681942415335726, -39.35891869721508840 ) ) ;
#20437=CARTESIAN_POINT ( 'NONE',  ( -135.8532207217289738, -50.09629031063965243, -6.472252184284438492 ) ) ;
#20440=CARTESIAN_POINT ( 'NONE',  ( 200.0000000000000000, -40.00000000000005684, 19.99999999999978328 ) ) ;
#20441=( BOUNDED_SURFACE ( )  B_SPLINE_SURFACE ( 3, 3, ( 
 ( #19410, #26064, #21928, #3841, #21931, #11808, #15531, #7945, #19928, #9821, #5566, #23659, #11538, #25799, #7806, #22205, #26209, #24189, #3566, #11412, #17532, #5439, #7416, #17790, #13540, #9425, #1846, #21666, #3440, #9949 ),
 ( #16063, #9549, #18058, #25670, #11945, #3705, #5963, #24055, #11670, #14074, #13934, #19662, #5831, #19534, #13672, #1449, #19794, #1711, #1319, #17658, #21794, #1581, #15922, #15659, #7547, #17924, #25935, #5691, #26068, #23785 ),
 ( #20070, #22069, #9684, #7677, #15789, #23916, #13796, #24594, #10349, #22729, #6487, #18730, #12211, #12339, #14204, #18188, #14599, #16730, #1978, #8081, #514, #6616, #22602, #6350, #14469, #4507, #4378, #12469, #16200, #8619 ),
 ( #20596, #24861, #2372, #4113, #24731, #16598, #24333, #20467, #10084, #12608, #6097, #2242, #16470, #14338, #20737, #14733, #26339, #3980, #10484, #18459, #22338, #18598, #376, #237, #8480, #2506, #10617, #12077, #6226, #20199 ),
 ( #20333, #2110, #10219, #18326, #107, #8214, #22470, #16332, #24461, #4249, #8349, #19128, #17127, #11143, #15130, #2779, #6882, #7009, #910, #23132, #23260, #11018, #14866, #9023, #25390, #18866, #10891, #4904, #780, #12881 ),
 ( #7266, #2648, #8753, #647, #2910, #25001, #20864, #13267, #16869, #23387, #6754, #4642, #1038, #25258, #12744, #5161, #5036, #3161, #23000, #11263, #19003, #1169, #13143, #20997, #4777, #21262, #8886, #17380, #25132, #3034 ),
 ( #19382, #19258, #9138, #17254, #7142, #16997, #14997, #15258, #21389, #13014, #9272, #25519, #21135, #22865, #10755, #11383, #21635, #15629, #19637, #5410, #9397, #5799, #21896, #1817, #11781, #11639, #9657, #7777, #17891, #13511 ) ),
 .UNSPECIFIED., .T., .F., .F. ) 
 B_SPLINE_SURFACE_WITH_KNOTS ( ( 4, 3, 4 ),
 ( 4, 2, 2, 2, 2, 2, 2, 2, 2, 2, 2, 2, 2, 2, 4 ),
 ( 0.000000000000000000, 0.5000000000000000000, 1.000000000000000000 ),
 ( 0.000000000000000000, 0.1357259735107005372, 0.1651108541090157700, 0.1944957347073310028, 0.3598804999793158710, 0.3867117631979620773, 0.4135430264166082281, 0.5789277916885930964, 0.6062785021374117456, 0.6336292125862302838, 0.8508620842112317728, 0.8814014469398914198, 0.9119408096685510667, 0.9559704048342755334, 1.000000000000000000 ),
 .UNSPECIFIED. ) 
 GEOMETRIC_REPRESENTATION_ITEM ( )  RATIONAL_B_SPLINE_SURFACE ( (
 ( 1.000000000000000000, 1.000000000000000000, 1.000000000000000000, 1.000000000000000000, 1.000000000000000000, 1.000000000000000000, 1.000000000000000000, 1.000000000000000000, 1.000000000000000000, 1.000000000000000000, 1.000000000000000000, 1.000000000000000000, 1.000000000000000000, 1.000000000000000000, 1.000000000000000000, 1.000000000000000000, 1.000000000000000000, 1.000000000000000000, 1.000000000000000000, 1.000000000000000000, 1.000000000000000000, 1.000000000000000000, 1.000000000000000000, 1.000000000000000000, 1.000000000000000000, 1.000000000000000000, 1.000000000000000000, 1.000000000000000000, 1.000000000000000000, 1.000000000000000000),
 ( 0.3333333333333333703, 0.3333333333333333703, 0.3333333333333333703, 0.3333333333333333703, 0.3333333333333333703, 0.3333333333333333703, 0.3333333333333333703, 0.3333333333333333703, 0.3333333333333333703, 0.3333333333333333703, 0.3333333333333333703, 0.3333333333333333703, 0.3333333333333333703, 0.3333333333333333703, 0.3333333333333333703, 0.3333333333333333703, 0.3333333333333333703, 0.3333333333333333703, 0.3333333333333333703, 0.3333333333333333703, 0.3333333333333333703, 0.3333333333333333703, 0.3333333333333333703, 0.3333333333333333703, 0.3333333333333333703, 0.3333333333333333703, 0.3333333333333333703, 0.3333333333333333703, 0.3333333333333333703, 0.3333333333333333703),
 ( 0.3333333333333333703, 0.3333333333333333703, 0.3333333333333333703, 0.3333333333333333703, 0.3333333333333333703, 0.3333333333333333703, 0.3333333333333333703, 0.3333333333333333703, 0.3333333333333333703, 0.3333333333333333703, 0.3333333333333333703, 0.3333333333333333703, 0.3333333333333333703, 0.3333333333333333703, 0.3333333333333333703, 0.3333333333333333703, 0.3333333333333333703, 0.3333333333333333703, 0.3333333333333333703, 0.3333333333333333703, 0.3333333333333333703, 0.3333333333333333703, 0.3333333333333333703, 0.3333333333333333703, 0.3333333333333333703, 0.3333333333333333703, 0.3333333333333333703, 0.3333333333333333703, 0.3333333333333333703, 0.3333333333333333703),
 ( 1.000000000000000000, 1.000000000000000000, 1.000000000000000000, 1.000000000000000000, 1.000000000000000000, 1.000000000000000000, 1.000000000000000000, 1.000000000000000000, 1.000000000000000000, 1.000000000000000000, 1.000000000000000000, 1.000000000000000000, 1.000000000000000000, 1.000000000000000000, 1.000000000000000000, 1.000000000000000000, 1.000000000000000000, 1.000000000000000000, 1.000000000000000000, 1.000000000000000000, 1.000000000000000000, 1.000000000000000000, 1.000000000000000000, 1.000000000000000000, 1.000000000000000000, 1.000000000000000000, 1.000000000000000000, 1.000000000000000000, 1.000000000000000000, 1.000000000000000000),
 ( 0.3333333333333333703, 0.3333333333333333703, 0.3333333333333333703, 0.3333333333333333703, 0.3333333333333333703, 0.3333333333333333703, 0.3333333333333333703, 0.3333333333333333703, 0.3333333333333333703, 0.3333333333333333703, 0.3333333333333333703, 0.3333333333333333703, 0.3333333333333333703, 0.3333333333333333703, 0.3333333333333333703, 0.3333333333333333703, 0.3333333333333333703, 0.3333333333333333703, 0.3333333333333333703, 0.3333333333333333703, 0.3333333333333333703, 0.3333333333333333703, 0.3333333333333333703, 0.3333333333333333703, 0.3333333333333333703, 0.3333333333333333703, 0.3333333333333333703, 0.3333333333333333703, 0.3333333333333333703, 0.3333333333333333703),
 ( 0.3333333333333333703, 0.3333333333333333703, 0.3333333333333333703, 0.3333333333333333703, 0.3333333333333333703, 0.3333333333333333703, 0.3333333333333333703, 0.3333333333333333703, 0.3333333333333333703, 0.3333333333333333703, 0.3333333333333333703, 0.3333333333333333703, 0.3333333333333333703, 0.3333333333333333703, 0.3333333333333333703, 0.3333333333333333703, 0.3333333333333333703, 0.3333333333333333703, 0.3333333333333333703, 0.3333333333333333703, 0.3333333333333333703, 0.3333333333333333703, 0.3333333333333333703, 0.3333333333333333703, 0.3333333333333333703, 0.3333333333333333703, 0.3333333333333333703, 0.3333333333333333703, 0.3333333333333333703, 0.3333333333333333703),
 ( 1.000000000000000000, 1.000000000000000000, 1.000000000000000000, 1.000000000000000000, 1.000000000000000000, 1.000000000000000000, 1.000000000000000000, 1.000000000000000000, 1.000000000000000000, 1.000000000000000000, 1.000000000000000000, 1.000000000000000000, 1.000000000000000000, 1.000000000000000000, 1.000000000000000000, 1.000000000000000000, 1.000000000000000000, 1.000000000000000000, 1.000000000000000000, 1.000000000000000000, 1.000000000000000000, 1.000000000000000000, 1.000000000000000000, 1.000000000000000000, 1.000000000000000000, 1.000000000000000000, 1.000000000000000000, 1.000000000000000000, 1.000000000000000000, 1.000000000000000000) ) ) 
 REPRESENTATION_ITEM ( '' )  SURFACE ( )  );
#20443=CARTESIAN_POINT ( 'NONE',  ( 16.10036699862805420, 48.79524671500497845, -14.09853761975148068 ) ) ;
#20444=CARTESIAN_POINT ( 'NONE',  ( -198.0356074513804572, 15.37879056873066830, -40.00000000000002132 ) ) ;
#20445=CARTESIAN_POINT ( 'NONE',  ( 57.59792236341147031, -1.722363176415032004, -1.722363176415048880 ) ) ;
#20446=CARTESIAN_POINT ( 'NONE',  ( -4.112199523540587265, -46.96527782736856693, 13.82298295336165950 ) ) ;
#20448=CARTESIAN_POINT ( 'NONE',  ( -86.96347745069644475, 18.24025645688351105, 2.449293598294708485E-15 ) ) ;
#20449=VERTEX_POINT ( 'NONE', #17672 ) ;
#20453=CARTESIAN_POINT ( 'NONE',  ( 57.59792236341147031, -30.00663442387700641, 26.56190807104681895 ) ) ;
#20454=CARTESIAN_POINT ( 'NONE',  ( -4.810655158399423925, -17.78437748360810744, 42.93528531928082970 ) ) ;
#20456=CARTESIAN_POINT ( 'NONE',  ( -3.488770945845315552, 17.93216134257417238, -43.29206711590411061 ) ) ;
#20460=CARTESIAN_POINT ( 'NONE',  ( -173.7925586247448564, -20.60916590994201059, 38.69493321926378826 ) ) ;
#20461=CARTESIAN_POINT ( 'NONE',  ( 200.0000000000000000, -42.42640687119272513, -14.14213562373140753 ) ) ;
#20462=CARTESIAN_POINT ( 'NONE',  ( -87.11144460433696679, -2.726859767319054662, 21.34775726304732402 ) ) ;
#20463=CARTESIAN_POINT ( 'NONE',  ( -192.1964066538403983, 14.00508515770237850, -48.17614796926574172 ) ) ;
#20464=CARTESIAN_POINT ( 'NONE',  ( -135.8532207217289738, 21.81201906317729566, 34.75652343174635917 ) ) ;
#20465=CARTESIAN_POINT ( 'NONE',  ( -162.0762913951021176, 29.48230308784730980, 27.08623940707652622 ) ) ;
#20466=CARTESIAN_POINT ( 'NONE',  ( 199.9999999999999432, -19.99999999999988987, -2.449293598294708485E-15 ) ) ;
#20467=CARTESIAN_POINT ( 'NONE',  ( -162.0762913951020892, 41.69427287682832173, 2.449293598294708485E-15 ) ) ;
#20468=CARTESIAN_POINT ( 'NONE',  ( -259.2033419157646676, -40.00000000000017053, 9.517827891722212996 ) ) ;
#20469=CARTESIAN_POINT ( 'NONE',  ( 4.995406935893297096, 10.78321810387837232, 67.35176059880234334 ) ) ;
#20470=CARTESIAN_POINT ( 'NONE',  ( -102.4309680866695658, 20.43798635339614123, -8.087567261645812522 ) ) ;
#20472=CARTESIAN_POINT ( 'NONE',  ( -238.4067589809705794, -28.96627169325303797, -28.96627169325349627 ) ) ;
#20474=CARTESIAN_POINT ( 'NONE',  ( 192.4448373802100889, -14.14213562375876698, -14.14213562375885047 ) ) ;
#20475=CARTESIAN_POINT ( 'NONE',  ( -103.9663809734228010, 8.574562933000146714, 19.92521373354193059 ) ) ;
#20477=CARTESIAN_POINT ( 'NONE',  ( 14.38125909742182529, -39.01709431150933938, 39.01709431150894147 ) ) ;
#20478=CARTESIAN_POINT ( 'NONE',  ( -3.696864809820963771, -47.11278487914724877, -13.84627154338573440 ) ) ;
#20480=CARTESIAN_POINT ( 'NONE',  ( 21.15358250000286944, -47.58740525741999505, -13.91686544622497479 ) ) ;
#20486=CARTESIAN_POINT ( 'NONE',  ( 170.2234770963711128, 10.92277846919210660, -45.64576402573182889 ) ) ;
#20487=CARTESIAN_POINT ( 'NONE',  ( -188.2957210513760913, -43.00408675155287597, -23.44847782072231368 ) ) ;
#20488=( BOUNDED_SURFACE ( )  B_SPLINE_SURFACE ( 3, 2, ( 
 ( #21731, #15467, #23223 ),
 ( #11352, #21356, #11106 ),
 ( #5128, #9105, #13602 ),
 ( #15351, #17215, #25732 ),
 ( #25354, #1255, #3125 ),
 ( #1135, #7109, #7354 ),
 ( #9359, #5375, #15220 ),
 ( #13479, #11228, #25482 ),
 ( #21601, #3374, #11606 ),
 ( #5247, #11473, #13351 ),
 ( #19729, #19601, #1387 ),
 ( #9488, #17592, #7483 ),
 ( #1516, #9621, #1914 ),
 ( #20136, #21860, #12016 ),
 ( #23850, #14273, #8017 ),
 ( #20407, #3917, #5762 ),
 ( #14006, #15853, #19860 ),
 ( #13870, #7879, #3636 ),
 ( #10019, #18397, #22136 ),
 ( #14142, #11877, #7610 ),
 ( #26006, #18128, #26278 ),
 ( #22409, #22003, #22274 ),
 ( #13734, #4185, #16132 ),
 ( #1646, #24262, #6036 ),
 ( #12280, #15725, #3773 ),
 ( #19997, #5628, #24127 ),
 ( #4048, #9754, #12149 ),
 ( #1783, #11741, #5898 ),
 ( #17855, #7742, #9887 ),
 ( #20271, #2050, #26136 ),
 ( #10157, #23983, #17989 ),
 ( #16000, #2181, #18260 ),
 ( #41, #8154, #16268 ),
 ( #10289, #24397, #6163 ),
 ( #22538, #2805, #13289 ),
 ( #13165, #21158, #8912 ),
 ( #11289, #21410, #25413 ),
 ( #15280, #9167, #4668 ),
 ( #12770, #25284, #20897 ),
 ( #7040, #4805, #12907 ),
 ( #21022, #15156, #25025 ),
 ( #13040, #6908, #6290 ),
 ( #4929, #10780, #2675 ),
 ( #9045, #23283, #23410 ),
 ( #8280, #10916, #3059 ),
 ( #174, #14890, #11162 ),
 ( #16406, #17021, #24534 ),
 ( #18892, #17150, #17281 ),
 ( #14408, #25157, #671 ),
 ( #8780, #23030, #2932 ),
 ( #936, #19027, #19151 ),
 ( #5059, #21285, #3183 ),
 ( #19278, #6778, #16893 ),
 ( #806, #5187, #15025 ),
 ( #23155, #11041, #1061 ),
 ( #7164, #5302, #3311 ),
 ( #21927, #26063, #23911 ),
 ( #1192, #5687, #25931 ),
 ( #17653, #17402, #15406 ),
 ( #17786, #23531, #5560 ),
 ( #23655, #5435, #13929 ),
 ( #9545, #7543, #25795 ) ),
 .UNSPECIFIED., .F., .F., .F. ) 
 B_SPLINE_SURFACE_WITH_KNOTS ( ( 4, 2, 2, 2, 2, 2, 2, 2, 2, 2, 2, 2, 2, 2, 2, 2, 2, 2, 2, 2, 2, 2, 2, 2, 2, 2, 2, 2, 2, 2, 4 ),
 ( 3, 3 ),
 ( 0.005118828937694972631, 0.02956064127319301543, 0.05400245360869105476, 0.07844426594418910104, 0.08149949248612635422, 0.08302710575709498775, 0.08379091239257929757, 0.08417281571032145249, 0.08436376736919252994, 0.08445924319862807561, 0.08450698111334584151, 0.08455471902806360740, 0.09066517211193811376, 0.09677562519581262013, 0.09983085173774988719, 0.1028860782796871404, 0.1089965313635616606, 0.1151069844474361670, 0.1181622109893734202, 0.1196898242603420537, 0.1204536308958263635, 0.1208355342135685184, 0.1208594031709274014, 0.1208832721282862843, 0.1209310100430040502, 0.1210264858724395959, 0.1212174375313106733, 0.1273278906151851797, 0.1517697029506832329, 0.1762115152861812861, 0.2006533276216793116 ),
 ( 0.000000000000000000, 1.000000000000000000 ),
 .UNSPECIFIED. ) 
 GEOMETRIC_REPRESENTATION_ITEM ( )  RATIONAL_B_SPLINE_SURFACE ( (
 ( 1.000000000000000000, 0.9997813423572989855, 1.000000000000000000),
 ( 1.000000000000000000, 0.9990919206318849000, 1.000000000000000000),
 ( 1.000000000000000000, 0.9967874177841468120, 1.000000000000000000),
 ( 1.000000000000000000, 0.9887544623280423162, 1.000000000000000000),
 ( 1.000000000000000000, 0.9830290792194826821, 1.000000000000000000),
 ( 1.000000000000000000, 0.9678345454226084943, 1.000000000000000000),
 ( 1.000000000000000000, 0.9583650305405041481, 1.000000000000000000),
 ( 1.000000000000000000, 0.9453335293271442064, 1.000000000000000000),
 ( 1.000000000000000000, 0.9438523872746331644, 1.000000000000000000),
 ( 1.000000000000000000, 0.9415799504611004345, 1.000000000000000000),
 ( 1.000000000000000000, 0.9408140170423924253, 1.000000000000000000),
 ( 1.000000000000000000, 0.9396523143999068184, 1.000000000000000000),
 ( 1.000000000000000000, 0.9392629463989446981, 1.000000000000000000),
 ( 1.000000000000000000, 0.9386756783046028563, 1.000000000000000000),
 ( 1.000000000000000000, 0.9384793862554876576, 1.000000000000000000),
 ( 1.000000000000000000, 0.9381841422086912852, 1.000000000000000000),
 ( 1.000000000000000000, 0.9380855931974644291, 1.000000000000000000),
 ( 1.000000000000000000, 0.9379375679425655532, 1.000000000000000000),
 ( 1.000000000000000000, 0.9378881925679135589, 1.000000000000000000),
 ( 1.000000000000000000, 0.9378140790407650806, 1.000000000000000000),
 ( 1.000000000000000000, 0.9377896949153100570, 1.000000000000000000),
 ( 1.000000000000000000, 0.9377409313168981742, 1.000000000000000000),
 ( 1.000000000000000000, 0.9377165729686738338, 1.000000000000000000),
 ( 1.000000000000000000, 0.9345773786263239513, 1.000000000000000000),
 ( 1.000000000000000000, 0.9318492984271956603, 1.000000000000000000),
 ( 1.000000000000000000, 0.9273872927432106339, 1.000000000000000000),
 ( 1.000000000000000000, 0.9256532593469934955, 1.000000000000000000),
 ( 1.000000000000000000, 0.9239357372751176856, 1.000000000000000000),
 ( 1.000000000000000000, 0.9235102113428155235, 1.000000000000000000),
 ( 1.000000000000000000, 0.9229728558028649221, 1.000000000000000000),
 ( 1.000000000000000000, 0.9228633126626060168, 1.000000000000000000),
 ( 1.000000000000000000, 0.9230139704737757578, 1.000000000000000000),
 ( 1.000000000000000000, 0.9237531682200380567, 1.000000000000000000),
 ( 1.000000000000000000, 0.9264156051934421265, 1.000000000000000000),
 ( 1.000000000000000000, 0.9283388455997357847, 1.000000000000000000),
 ( 1.000000000000000000, 0.9320050037532509046, 1.000000000000000000),
 ( 1.000000000000000000, 0.9333574575349512514, 1.000000000000000000),
 ( 1.000000000000000000, 0.9355411998008567043, 1.000000000000000000),
 ( 1.000000000000000000, 0.9362956009275962277, 1.000000000000000000),
 ( 1.000000000000000000, 0.9374637148016307098, 1.000000000000000000),
 ( 1.000000000000000000, 0.9378591705544923052, 1.000000000000000000),
 ( 1.000000000000000000, 0.9384610703419788980, 1.000000000000000000),
 ( 1.000000000000000000, 0.9386631562400657991, 1.000000000000000000),
 ( 1.000000000000000000, 0.9388793792114339398, 1.000000000000000000),
 ( 1.000000000000000000, 0.9388921037490453037, 1.000000000000000000),
 ( 1.000000000000000000, 0.9389175638858661133, 1.000000000000000000),
 ( 1.000000000000000000, 0.9389305010154688214, 1.000000000000000000),
 ( 1.000000000000000000, 0.9389691441648042591, 1.000000000000000000),
 ( 1.000000000000000000, 0.9389948969011616686, 1.000000000000000000),
 ( 1.000000000000000000, 0.9390721270299958734, 1.000000000000000000),
 ( 1.000000000000000000, 0.9391235763422339788, 1.000000000000000000),
 ( 1.000000000000000000, 0.9392778120326576996, 1.000000000000000000),
 ( 1.000000000000000000, 0.9393804861645823623, 1.000000000000000000),
 ( 1.000000000000000000, 0.9427638002345609669, 1.000000000000000000),
 ( 1.000000000000000000, 0.9458915987233159628, 1.000000000000000000),
 ( 1.000000000000000000, 0.9607963039206450784, 1.000000000000000000),
 ( 1.000000000000000000, 0.9703812854709533697, 1.000000000000000000),
 ( 1.000000000000000000, 0.9854660764533723638, 1.000000000000000000),
 ( 1.000000000000000000, 0.9909632567906727640, 1.000000000000000000),
 ( 1.000000000000000000, 0.9982308762622302822, 1.000000000000000000),
 ( 1.000000000000000000, 0.9999976772054812724, 1.000000000000000000),
 ( 1.000000000000000000, 1.000000000000000000, 1.000000000000000000) ) ) 
 REPRESENTATION_ITEM ( '' )  SURFACE ( )  );
#20489=CARTESIAN_POINT ( 'NONE',  ( 146.6084372240433709, -40.00000000000001421, 5.374981219216829587 ) ) ;
#20490=CARTESIAN_POINT ( 'NONE',  ( -192.9588430854690273, 54.46834944101718889, 40.00000000000002132 ) ) ;
#20493=CARTESIAN_POINT ( 'NONE',  ( -213.1075012329537230, -40.00000000000025580, 53.71589010953650956 ) ) ;
#20494=CARTESIAN_POINT ( 'NONE',  ( 151.7948205124836534, -40.00000000000001421, 6.767089262348889633 ) ) ;
#20495=CARTESIAN_POINT ( 'NONE',  ( -30.26275506840324070, -1.147469862568086380E-14, 1.694272468446259783 ) ) ;
#20496=CARTESIAN_POINT ( 'NONE',  ( -100.7734535825088500, 22.67402823373189591, -0.000000000000000000 ) ) ;
#20497=CARTESIAN_POINT ( 'NONE',  ( 91.82158438592159655, -16.11829626346147393, 16.11829626346132116 ) ) ;
#20498=CARTESIAN_POINT ( 'NONE',  ( 146.6084372240433709, -5.374981219216942385, -40.00000000000002132 ) ) ;
#20499=CARTESIAN_POINT ( 'NONE',  ( 151.7948205124836250, -4.785054706301671068, 4.785054706301645311 ) ) ;
#20500=CARTESIAN_POINT ( 'NONE',  ( 156.5537079553355966, -11.28159757857204326, -27.23618587942440783 ) ) ;
#20502=CARTESIAN_POINT ( 'NONE',  ( 57.59792236341147742, 4.064940816252731242E-13, -37.56421063658186199 ) ) ;
#20503=CARTESIAN_POINT ( 'NONE',  ( 136.1360204305621266, 5.219216885335291329E-15, 4.966164525587064560 ) ) ;
#20504=CARTESIAN_POINT ( 'NONE',  ( 4.995406935893290878, 39.06748935135185263, 39.06748935135198764 ) ) ;
#20507=CARTESIAN_POINT ( 'NONE',  ( -86.96347745069643054, -41.18208027870589660, -15.38646221621809040 ) ) ;
#20508=ORIENTED_EDGE ( 'NONE', *, *, #19169, .F. ) ;
#20509=CARTESIAN_POINT ( 'NONE',  ( 163.1118516004056573, -47.56205970284945295, -9.006482792074823607 ) ) ;
#20510=CARTESIAN_POINT ( 'NONE',  ( 132.4338126186517002, 29.78211700502426496, -12.33615677966331248 ) ) ;
#20511=CARTESIAN_POINT ( 'NONE',  ( -198.0356074513804288, -55.37879056873077133, -2.449293598294708485E-15 ) ) ;
#20512=CARTESIAN_POINT ( 'NONE',  ( 170.0000000000000000, -2.301191124287261779E-13, 24.95097643317000546 ) ) ;
#20517=CARTESIAN_POINT ( 'NONE',  ( 104.1600437297061745, 8.548029201969624680, -20.63676802892751994 ) ) ;
#20518=CARTESIAN_POINT ( 'NONE',  ( 23.35901252181126964, 13.80180065670255907, 46.81387818480148866 ) ) ;
#20523=CARTESIAN_POINT ( 'NONE',  ( -110.0961829990539655, -2.516385845105195251, -20.07657727077722853 ) ) ;
#20524=CARTESIAN_POINT ( 'NONE',  ( 19.06497207195980792, 10.03556273973433299, 10.03556273973436319 ) ) ;
#20525=CARTESIAN_POINT ( 'NONE',  ( 199.9999999999999432, 14.14213562373090838, 14.14213562373092437 ) ) ;
#20526=CARTESIAN_POINT ( 'NONE',  ( -200.0000000000000284, -17.27712336974170881, 46.88040655664276102 ) ) ;
#20527=CARTESIAN_POINT ( 'NONE',  ( -94.58360650938202241, -9.000712009885686982, -20.58386743642789440 ) ) ;
#20528=CARTESIAN_POINT ( 'NONE',  ( 91.82158438592156813, 40.00000000000027711, -22.79471317813428044 ) ) ;
#20529=CARTESIAN_POINT ( 'NONE',  ( 151.7948205124836250, -3.202120068677277203E-13, 33.23291073765553705 ) ) ;
#20533=CARTESIAN_POINT ( 'NONE',  ( -190.7345856381493263, 23.92884448222178406, 43.65254615102011115 ) ) ;
#20534=CARTESIAN_POINT ( 'NONE',  ( 146.6084372240433993, 24.48358557860307272, 24.48358557860347418 ) ) ;
#20535=ADVANCED_FACE ( 'NONE', ( #3083 ), #23218, .T. ) ;
#20537=CARTESIAN_POINT ( 'NONE',  ( 0.2972598230769923355, 18.14793986248697166, 38.42060263243675422 ) ) ;
#20539=CARTESIAN_POINT ( 'NONE',  ( 170.2234770963711128, 45.64576402573196390, -10.92277846919159856 ) ) ;
#20541=CARTESIAN_POINT ( 'NONE',  ( -259.2033419157646676, 9.517827891722584255, -0.000000000000000000 ) ) ;
#20542=EDGE_CURVE ( 'NONE', #18174, #13223, #14399, .T. ) ;
#20543=B_SPLINE_CURVE_WITH_KNOTS ( 'NONE', 3,
 ( #9757, #19863, #3250, #5630, #11354, #19731, #13736, #11475 ),
 .UNSPECIFIED., .F., .F.,
 ( 4, 2, 2, 4 ),
 ( 0.000000000000000000, 0.002089226651538985107, 0.004178453303077970214, 0.008356906606155938694 ),
 .UNSPECIFIED. ) ;
#20544=CARTESIAN_POINT ( 'NONE',  ( 116.7964245048381713, 19.78678521258536449, -19.78678521258513356 ) ) ;
#20545=CARTESIAN_POINT ( 'NONE',  ( -213.1075012329537230, -13.71589010951915810, 40.00000000000002132 ) ) ;
#20546=CARTESIAN_POINT ( 'NONE',  ( -114.7810454938858982, 16.28728334995616933, 14.99889064788714066 ) ) ;
#20547=CARTESIAN_POINT ( 'NONE',  ( 136.1360204305621551, 39.99999999999968026, 35.03383547441337953 ) ) ;
#20549=CARTESIAN_POINT ( 'NONE',  ( -100.7734535825088500, 12.25131212657490209, -44.31723036834897300 ) ) ;
#20551=CARTESIAN_POINT ( 'NONE',  ( 127.8236149080042026, -11.91256696755882771, 28.75948073575737141 ) ) ;
#20554=CARTESIAN_POINT ( 'NONE',  ( -198.0356074513804572, 15.37879056873067007, 0.000000000000000000 ) ) ;
#20556=CARTESIAN_POINT ( 'NONE',  ( -135.8532207217289738, 21.81201906317798134, -21.81201906317747685 ) ) ;
#20557=CARTESIAN_POINT ( 'NONE',  ( -114.4364955367318970, -20.29001642038926789, -8.064892380839017605 ) ) ;
#20558=CARTESIAN_POINT ( 'NONE',  ( -138.9613193423055861, -10.11110876497707523, -29.42718875716579774 ) ) ;
#20559=CARTESIAN_POINT ( 'NONE',  ( -138.9613198122422375, 13.65853124629189352, 27.95779845120234697 ) ) ;
#20562=CARTESIAN_POINT ( 'NONE',  ( 151.7948205124836534, -51.78348778862529400, -4.785054706299085581 ) ) ;
#20563=CARTESIAN_POINT ( 'NONE',  ( 4.995406935893297984, -39.06748935135205869, 17.50105314357158193 ) ) ;
#20564=CARTESIAN_POINT ( 'NONE',  ( -110.0513613218576410, 19.08113875878609988, 6.582668557813116550 ) ) ;
#20565=CARTESIAN_POINT ( 'NONE',  ( 130.8568914410475088, 40.00000000000011369, -5.949712681206269949 ) ) ;
#20566=CARTESIAN_POINT ( 'NONE',  ( 14.38125909742183062, -67.30136555895943218, -10.73282306403629605 ) ) ;
#20567=CARTESIAN_POINT ( 'NONE',  ( 91.82158438592158234, 17.20528682183301683, 0.000000000000000000 ) ) ;
#20568=CARTESIAN_POINT ( 'NONE',  ( -100.7734535825088358, -16.03295912088706743, -16.03295912088710296 ) ) ;
#20569=CARTESIAN_POINT ( 'NONE',  ( -259.2033419157646676, -21.55415060305824326, -35.01439189186556433 ) ) ;
#20573=CARTESIAN_POINT ( 'NONE',  ( 163.1118516004056573, 40.00000000000000711, 12.73709011382489642 ) ) ;
#20575=CARTESIAN_POINT ( 'NONE',  ( 23.40652632867980643, 46.79646383233858131, -13.79856377312498417 ) ) ;
#20576=CARTESIAN_POINT ( 'NONE',  ( -30.26275506840324070, 41.69427246844628598, 2.449293598294708485E-15 ) ) ;
#20578=CARTESIAN_POINT ( 'NONE',  ( -4.004886986945003891, -43.01537795656786045, 23.45685150724386148 ) ) ;
#20579=CARTESIAN_POINT ( 'NONE',  ( 19.06497207195980792, 54.19242893257843718, 2.449293598294708485E-15 ) ) ;
#20580=EDGE_LOOP ( 'NONE', ( #19671, #25307, #6177, #3758 ) ) ;
#20581=CARTESIAN_POINT ( 'NONE',  ( -199.9999999999999432, 39.01096890182041221, 39.01096890182058985 ) ) ;
#20582=CARTESIAN_POINT ( 'NONE',  ( -238.4067589809705794, -27.60227080167069147, 28.96627169325319429 ) ) ;
#20583=CARTESIAN_POINT ( 'NONE',  ( -4.121597284766306046, -23.43330939486645903, 42.98102224344803801 ) ) ;
#20584=CARTESIAN_POINT ( 'NONE',  ( -3.564770973659279640, 17.92368662243745092, -43.27160733161120021 ) ) ;
#20586=CARTESIAN_POINT ( 'NONE',  ( -28.75791583366071791, -38.33181286256370157, -12.03523584680476866 ) ) ;
#20588=CARTESIAN_POINT ( 'NONE',  ( -195.1685814578364386, -14.09692187700269095, 48.78510996053616822 ) ) ;
#20589=CARTESIAN_POINT ( 'NONE',  ( -91.56559293963834989, -44.31723036834885932, -12.25131212657538171 ) ) ;
#20590=CARTESIAN_POINT ( 'NONE',  ( -105.2054292635175585, -21.49321519473986442, -7.030298963786045751E-29 ) ) ;
#20591=( BOUNDED_SURFACE ( )  B_SPLINE_SURFACE ( 3, 3, ( 
 ( #2532, #22629, #12108, #6644, #20233, #4404, #4148, #12241, #12368, #8242, #20496, #20365, #12498, #18759, #10511, #10250, #3, #541, #10377, #2012, #4538, #18488, #8377, #16499, #24624, #14368, #8511, #8646, #18217, #22234 ),
 ( #18625, #16628, #12635, #24360, #4278, #16755, #24759, #6124, #22499, #14623, #20762, #14232, #24889, #18359, #138, #24494, #15024, #2931, #8911, #14758, #6907, #9044, #11161, #935, #19150, #17149, #7163, #17280, #4804, #4928 ),
 ( #805, #9296, #21157, #17401, #13288, #17020, #14889, #23154, #7039, #11288, #25540, #25156, #13039, #19277, #25283, #21021, #21409, #11040, #15155, #5058, #2804, #23409, #10915, #23282, #18891, #19408, #22888, #13164, #4667, #21284 ),
 ( #3058, #1060, #3182, #23029, #9166, #25024, #2674, #25412, #1191, #12769, #15279, #5186, #20896, #10779, #670, #8779, #16892, #6777, #12906, #19026, #3836, #7670, #5686, #1444, #19528, #7411, #25665, #7291, #23910, #1312 ),
 ( #3561, #11665, #5558, #19789, #17652, #19923, #22064, #3310, #15405, #1576, #5826, #20065, #23530, #1706, #11406, #13666, #1841, #9420, #13928, #9544, #11938, #9943, #21789, #5301, #17527, #9814, #25930, #17919, #18051, #13411 ),
 ( #26062, #15655, #9679, #25794, #7542, #21535, #13790, #23779, #17785, #15783, #15525, #21926, #23654, #5434, #13535, #3698, #21660, #3432, #11803, #19657, #7800, #11533, #15915, #24049, #18454, #6092, #3975, #22723, #16327, #16058 ),
 ( #22200, #12463, #12072, #20191, #6220, #1973, #24184, #16593, #10079, #371, #230, #4244, #8475, #18184, #8209, #6482, #12334, #26334, #8075, #14594, #22331, #4500, #10344, #24328, #16194, #16465, #2236, #24589, #24455, #8344 ) ),
 .UNSPECIFIED., .T., .F., .F. ) 
 B_SPLINE_SURFACE_WITH_KNOTS ( ( 4, 3, 4 ),
 ( 4, 2, 2, 2, 2, 2, 2, 2, 2, 2, 2, 2, 2, 2, 4 ),
 ( 0.000000000000000000, 0.5000000000000000000, 1.000000000000000000 ),
 ( 0.000000000000000000, 0.1357259735107005372, 0.1651108541090157700, 0.1944957347073310028, 0.3598804999793158710, 0.3867117631979620773, 0.4135430264166082281, 0.5789277916885930964, 0.6062785021374117456, 0.6336292125862302838, 0.8508620842112317728, 0.8814014469398914198, 0.9119408096685510667, 0.9559704048342755334, 1.000000000000000000 ),
 .UNSPECIFIED. ) 
 GEOMETRIC_REPRESENTATION_ITEM ( )  RATIONAL_B_SPLINE_SURFACE ( (
 ( 1.000000000000000000, 1.000000000000000000, 1.000000000000000000, 1.000000000000000000, 1.000000000000000000, 1.000000000000000000, 1.000000000000000000, 1.000000000000000000, 1.000000000000000000, 1.000000000000000000, 1.000000000000000000, 1.000000000000000000, 1.000000000000000000, 1.000000000000000000, 1.000000000000000000, 1.000000000000000000, 1.000000000000000000, 1.000000000000000000, 1.000000000000000000, 1.000000000000000000, 1.000000000000000000, 1.000000000000000000, 1.000000000000000000, 1.000000000000000000, 1.000000000000000000, 1.000000000000000000, 1.000000000000000000, 1.000000000000000000, 1.000000000000000000, 1.000000000000000000),
 ( 0.3333333333333333703, 0.3333333333333333703, 0.3333333333333333703, 0.3333333333333333703, 0.3333333333333333703, 0.3333333333333333703, 0.3333333333333333703, 0.3333333333333333703, 0.3333333333333333703, 0.3333333333333333703, 0.3333333333333333703, 0.3333333333333333703, 0.3333333333333333703, 0.3333333333333333703, 0.3333333333333333703, 0.3333333333333333703, 0.3333333333333333703, 0.3333333333333333703, 0.3333333333333333703, 0.3333333333333333703, 0.3333333333333333703, 0.3333333333333333703, 0.3333333333333333703, 0.3333333333333333703, 0.3333333333333333703, 0.3333333333333333703, 0.3333333333333333703, 0.3333333333333333703, 0.3333333333333333703, 0.3333333333333333703),
 ( 0.3333333333333333703, 0.3333333333333333703, 0.3333333333333333703, 0.3333333333333333703, 0.3333333333333333703, 0.3333333333333333703, 0.3333333333333333703, 0.3333333333333333703, 0.3333333333333333703, 0.3333333333333333703, 0.3333333333333333703, 0.3333333333333333703, 0.3333333333333333703, 0.3333333333333333703, 0.3333333333333333703, 0.3333333333333333703, 0.3333333333333333703, 0.3333333333333333703, 0.3333333333333333703, 0.3333333333333333703, 0.3333333333333333703, 0.3333333333333333703, 0.3333333333333333703, 0.3333333333333333703, 0.3333333333333333703, 0.3333333333333333703, 0.3333333333333333703, 0.3333333333333333703, 0.3333333333333333703, 0.3333333333333333703),
 ( 1.000000000000000000, 1.000000000000000000, 1.000000000000000000, 1.000000000000000000, 1.000000000000000000, 1.000000000000000000, 1.000000000000000000, 1.000000000000000000, 1.000000000000000000, 1.000000000000000000, 1.000000000000000000, 1.000000000000000000, 1.000000000000000000, 1.000000000000000000, 1.000000000000000000, 1.000000000000000000, 1.000000000000000000, 1.000000000000000000, 1.000000000000000000, 1.000000000000000000, 1.000000000000000000, 1.000000000000000000, 1.000000000000000000, 1.000000000000000000, 1.000000000000000000, 1.000000000000000000, 1.000000000000000000, 1.000000000000000000, 1.000000000000000000, 1.000000000000000000),
 ( 0.3333333333333333703, 0.3333333333333333703, 0.3333333333333333703, 0.3333333333333333703, 0.3333333333333333703, 0.3333333333333333703, 0.3333333333333333703, 0.3333333333333333703, 0.3333333333333333703, 0.3333333333333333703, 0.3333333333333333703, 0.3333333333333333703, 0.3333333333333333703, 0.3333333333333333703, 0.3333333333333333703, 0.3333333333333333703, 0.3333333333333333703, 0.3333333333333333703, 0.3333333333333333703, 0.3333333333333333703, 0.3333333333333333703, 0.3333333333333333703, 0.3333333333333333703, 0.3333333333333333703, 0.3333333333333333703, 0.3333333333333333703, 0.3333333333333333703, 0.3333333333333333703, 0.3333333333333333703, 0.3333333333333333703),
 ( 0.3333333333333333703, 0.3333333333333333703, 0.3333333333333333703, 0.3333333333333333703, 0.3333333333333333703, 0.3333333333333333703, 0.3333333333333333703, 0.3333333333333333703, 0.3333333333333333703, 0.3333333333333333703, 0.3333333333333333703, 0.3333333333333333703, 0.3333333333333333703, 0.3333333333333333703, 0.3333333333333333703, 0.3333333333333333703, 0.3333333333333333703, 0.3333333333333333703, 0.3333333333333333703, 0.3333333333333333703, 0.3333333333333333703, 0.3333333333333333703, 0.3333333333333333703, 0.3333333333333333703, 0.3333333333333333703, 0.3333333333333333703, 0.3333333333333333703, 0.3333333333333333703, 0.3333333333333333703, 0.3333333333333333703),
 ( 1.000000000000000000, 1.000000000000000000, 1.000000000000000000, 1.000000000000000000, 1.000000000000000000, 1.000000000000000000, 1.000000000000000000, 1.000000000000000000, 1.000000000000000000, 1.000000000000000000, 1.000000000000000000, 1.000000000000000000, 1.000000000000000000, 1.000000000000000000, 1.000000000000000000, 1.000000000000000000, 1.000000000000000000, 1.000000000000000000, 1.000000000000000000, 1.000000000000000000, 1.000000000000000000, 1.000000000000000000, 1.000000000000000000, 1.000000000000000000, 1.000000000000000000, 1.000000000000000000, 1.000000000000000000, 1.000000000000000000, 1.000000000000000000, 1.000000000000000000) ) ) 
 REPRESENTATION_ITEM ( '' )  SURFACE ( )  );
#20592=CARTESIAN_POINT ( 'NONE',  ( -189.5227851116837314, 18.00253723945986550, -43.46196956062437522 ) ) ;
#20593=CARTESIAN_POINT ( 'NONE',  ( 163.1118516004056573, -19.27778845538787422, 19.27778845538743724 ) ) ;
#20594=CARTESIAN_POINT ( 'NONE',  ( 130.8568914410475088, 4.207082182989012153, 52.36146031193425188 ) ) ;
#20595=CARTESIAN_POINT ( 'NONE',  ( -135.8532207217289738, -30.84685318188647685, -2.449293598294708485E-15 ) ) ;
#20596=CARTESIAN_POINT ( 'NONE',  ( -280.0000000000000000, 19.99999999999996092, 2.449293598294708485E-15 ) ) ;
#20597=CARTESIAN_POINT ( 'NONE',  ( -86.96347745069643054, -40.00000000000026290, 21.75974354311608749 ) ) ;
#20598=CARTESIAN_POINT ( 'NONE',  ( 14.38125909742181463, 10.73282306405862485, 67.30136555898259587 ) ) ;
#20601=CARTESIAN_POINT ( 'NONE',  ( -56.48582580120558561, -21.81201906317755146, -21.81201906317792449 ) ) ;
#20602=CARTESIAN_POINT ( 'NONE',  ( 146.6084372240433993, 24.48358557860341733, -24.48358557860313311 ) ) ;
#20603=ORIENTED_EDGE ( 'NONE', *, *, #1674, .T. ) ;
#20604=CARTESIAN_POINT ( 'NONE',  ( 130.8568914410475088, -52.36146031193419503, 4.207082182989537955 ) ) ;
#20605=CARTESIAN_POINT ( 'NONE',  ( -97.73860346103491281, 8.185503821092320109, 20.89580782302881445 ) ) ;
#20606=EDGE_CURVE ( 'NONE', #3292, #19647, #19748, .T. ) ;
#20607=CARTESIAN_POINT ( 'NONE',  ( -213.1075012329536946, -37.98287015391263566, 37.98287015391218802 ) ) ;
#20608=CARTESIAN_POINT ( 'NONE',  ( 6.371015797558896132, -44.80452650039788409, -18.55864253217484361 ) ) ;
#20610=CARTESIAN_POINT ( 'NONE',  ( -103.9474983245026039, -20.15710290851505349, 8.027156558344394455 ) ) ;
#20611=CARTESIAN_POINT ( 'NONE',  ( -82.23726319248024197, -13.38816524724604307, -15.17212319098400997 ) ) ;
#20612=VERTEX_POINT ( 'NONE', #21777 ) ;
#20615=CARTESIAN_POINT ( 'NONE',  ( -189.6939645179714375, -43.50328570201185840, -18.01965094556654989 ) ) ;
#20616=CARTESIAN_POINT ( 'NONE',  ( -162.0762913951020892, -1.777970010055771463E-13, 41.69427287682835015 ) ) ;
#20617=CARTESIAN_POINT ( 'NONE',  ( 0.2972598230769930572, 54.33493731733936016, 2.449293598294708485E-15 ) ) ;
#20621=EDGE_CURVE ( 'NONE', #17844, #25529, #15642, .T. ) ;
#20622=CARTESIAN_POINT ( 'NONE',  ( -238.4067589809705794, -1.892706720741712928E-13, 40.96449427998260973 ) ) ;
#20623=CARTESIAN_POINT ( 'NONE',  ( 163.1118516004056573, 40.00000000000000711, 12.73709011382489642 ) ) ;
#20624=CARTESIAN_POINT ( 'NONE',  ( 163.1118516004056573, 1.251511021549353291E-13, -27.26290988616872824 ) ) ;
#20626=CARTESIAN_POINT ( 'NONE',  ( -192.9588430854689705, -54.46834944099975928, -2.449293598294708485E-15 ) ) ;
#20628=CARTESIAN_POINT ( 'NONE',  ( 19.06497207195982568, -38.31983398719646061, 38.31983398719606271 ) ) ;
#20629=CARTESIAN_POINT ( 'NONE',  ( 4.995406935893290878, 1.606505379428369110E-13, -15.24977328854832592 ) ) ;
#20630=CARTESIAN_POINT ( 'NONE',  ( -4.039451493210483690, -13.82811171175408127, -46.99046209229819482 ) ) ;
#20631=CARTESIAN_POINT ( 'NONE',  ( -192.9588430854690273, 40.00000000000055422, -54.46834944101679810 ) ) ;
#20632=CARTESIAN_POINT ( 'NONE',  ( -280.0000000000000568, 39.99999999999990763, 20.00000000000015987 ) ) ;
#20633=CARTESIAN_POINT ( 'NONE',  ( 136.1360204305621551, 3.511608612530801032, -53.05693388239316022 ) ) ;
#20635=CARTESIAN_POINT ( 'NONE',  ( -114.4364955367327070, -8.644468109209471507, 20.04994829327649342 ) ) ;
#20636=CARTESIAN_POINT ( 'NONE',  ( -208.1127848780264742, -38.89260858015758515, 38.89260858015713751 ) ) ;
#20638=CARTESIAN_POINT ( 'NONE',  ( -39.84211263212320375, 32.75097567537659415, -13.56589830566843347 ) ) ;
#20639=CARTESIAN_POINT ( 'NONE',  ( -109.1264249741455785, -33.12752917269520481, -13.72187187123273233 ) ) ;
#20640=CARTESIAN_POINT ( 'NONE',  ( -213.1075012329537230, -53.71589010953668719, -40.00000000000002132 ) ) ;
#20641=ADVANCED_FACE ( 'NONE', ( #24171 ), #16043, .T. ) ;
#20642=CARTESIAN_POINT ( 'NONE',  ( -105.3895469845263193, 9.637191077568175501, 19.08279132546278944 ) ) ;
#20643=CARTESIAN_POINT ( 'NONE',  ( -208.1127848780265026, 10.60833733269551615, -10.60833733269529766 ) ) ;
#20648=CARTESIAN_POINT ( 'NONE',  ( -99.31364972220153220, 8.933506367398260650, -20.48028939131441817 ) ) ;
#20649=CARTESIAN_POINT ( 'NONE',  ( 9.006212071482861958, 14.17897189022315985, 49.32687279760999388 ) ) ;
#20652=( BOUNDED_SURFACE ( )  B_SPLINE_SURFACE ( 3, 2, ( 
 ( #11370, #19491, #1275 ),
 ( #23616, #7249, #9380 ),
 ( #11129, #23117, #5397 ),
 ( #11248, #8870, #13253 ),
 ( #16981, #1023, #23246 ),
 ( #17111, #9124, #6867 ),
 ( #13499, #25117, #4889 ),
 ( #21621, #19365, #15371 ),
 ( #5021, #17236, #1155 ),
 ( #15488, #9259, #17489 ),
 ( #21118, #12996, #17365 ),
 ( #25377, #23494, #5268 ),
 ( #13371, #21497, #15111 ),
 ( #25631, #765, #7377 ),
 ( #14983, #3396, #2895 ),
 ( #11003, #13126, #21247 ),
 ( #3021, #19113, #7129 ),
 ( #896, #9006, #25243 ) ),
 .UNSPECIFIED., .F., .F., .F. ) 
 B_SPLINE_SURFACE_WITH_KNOTS ( ( 4, 2, 2, 2, 2, 2, 2, 2, 4 ),
 ( 3, 3 ),
 ( 0.04072677041617866339, 0.04791560368711805795, 0.04971281200485290486, 0.05151002032258775176, 0.05510443695805744557, 0.06229327022899683319, 0.06409047854673168010, 0.06588768686446652700, 0.06948210349993622081 ),
 ( 0.000000000000000000, 1.000000000000000000 ),
 .UNSPECIFIED. ) 
 GEOMETRIC_REPRESENTATION_ITEM ( )  RATIONAL_B_SPLINE_SURFACE ( (
 ( 1.000000000000000000, 0.9548354694798303344, 1.000000000000000000),
 ( 1.000000000000000000, 0.9525322275551380002, 1.000000000000000000),
 ( 1.000000000000000000, 0.9507090892362719536, 1.000000000000000000),
 ( 1.000000000000000000, 0.9491274414775124901, 1.000000000000000000),
 ( 1.000000000000000000, 0.9488458707020273053, 1.000000000000000000),
 ( 1.000000000000000000, 0.9483593263061569356, 1.000000000000000000),
 ( 1.000000000000000000, 0.9481536722360313085, 1.000000000000000000),
 ( 1.000000000000000000, 0.9476504947197553763, 1.000000000000000000),
 ( 1.000000000000000000, 0.9474672091609203095, 1.000000000000000000),
 ( 1.000000000000000000, 0.9473824175298217742, 1.000000000000000000),
 ( 1.000000000000000000, 0.9479352607974392830, 1.000000000000000000),
 ( 1.000000000000000000, 0.9493585438922157449, 1.000000000000000000),
 ( 1.000000000000000000, 0.9496800154561187979, 1.000000000000000000),
 ( 1.000000000000000000, 0.9503966251880781035, 1.000000000000000000),
 ( 1.000000000000000000, 0.9507930044150058047, 1.000000000000000000),
 ( 1.000000000000000000, 0.9520783076861127903, 1.000000000000000000),
 ( 1.000000000000000000, 0.9530652557247718537, 1.000000000000000000),
 ( 1.000000000000000000, 0.9541700779530455367, 1.000000000000000000) ) ) 
 REPRESENTATION_ITEM ( '' )  SURFACE ( )  );
#20653=CARTESIAN_POINT ( 'NONE',  ( -30.26275506840324070, -27.08623969584595770, 29.48230279907789608 ) ) ;
#20655=DIRECTION ( 'NONE',  ( -0.3301743741154957168, 0.9439199556516647549, 0.000000000000000000 ) ) ;
#20658=CARTESIAN_POINT ( 'NONE',  ( -208.1127848780264742, 67.17687982760683951, 10.60833733268317403 ) ) ;
#20661=CARTESIAN_POINT ( 'NONE',  ( -199.9999999999999716, -18.59955921182013228, 46.19968414209466800 ) ) ;
#20662=CARTESIAN_POINT ( 'NONE',  ( -100.0968563617331881, -8.149320301599320970, -20.72609133243391710 ) ) ;
#20663=CARTESIAN_POINT ( 'NONE',  ( -208.1127848780264742, 40.00000000000055422, -55.00245453014380814 ) ) ;
#20664=CARTESIAN_POINT ( 'NONE',  ( 14.38125909742180220, 40.00000000000017764, -15.17850393972591760 ) ) ;
#20669=CARTESIAN_POINT ( 'NONE',  ( -187.7698581930822854, 23.34605429454593306, 42.84913646251166597 ) ) ;
#20670=CARTESIAN_POINT ( 'NONE',  ( 192.4448373802100889, 14.14213562375873678, 14.14213562375894817 ) ) ;
#20671=CARTESIAN_POINT ( 'NONE',  ( -105.2272256531192625, 2.713820371751817451, -21.35019504733632090 ) ) ;
#20672=CARTESIAN_POINT ( 'NONE',  ( 57.59792236341148453, -26.56190807104700369, 26.56190807104673723 ) ) ;
#20674=CARTESIAN_POINT ( 'NONE',  ( -208.1127848780264742, -38.89260858015704514, -38.89260858015768463 ) ) ;
#20676=CARTESIAN_POINT ( 'NONE',  ( 57.59792236341147031, 2.435789363418171760, 0.000000000000000000 ) ) ;
#20678=CARTESIAN_POINT ( 'NONE',  ( 4.995406935893289102, 10.78321810389013002, -10.78321810388986712 ) ) ;
#20679=CARTESIAN_POINT ( 'NONE',  ( 14.38125909742181285, -15.17850393972633505, 40.00000000000002132 ) ) ;
#20681=CARTESIAN_POINT ( 'NONE',  ( -280.0000000000000568, -39.99999999999987210, -20.00000000000043343 ) ) ;
#20683=CARTESIAN_POINT ( 'NONE',  ( 159.7744820660627454, -10.75261058663780034, 25.95909830917674199 ) ) ;
#20684=ORIENTED_EDGE ( 'NONE', *, *, #18676, .F. ) ;
#20685=ORIENTED_EDGE ( 'NONE', *, *, #7195, .T. ) ;
#20686=CARTESIAN_POINT ( 'NONE',  ( -135.8532207217289738, -9.153146818113595984, 40.00000000000002132 ) ) ;
#20687=AXIS2_PLACEMENT_3D ( 'NONE', #25127, #8614, #14728 ) ;
#20690=CARTESIAN_POINT ( 'NONE',  ( 57.59792236341147031, 26.56190807104720975, -26.56190807104655249 ) ) ;
#20691=CARTESIAN_POINT ( 'NONE',  ( -110.0822598093819806, -19.77208535310723292, -4.084357705420478268 ) ) ;
#20693=CIRCLE ( 'NONE', #7926, 15.00000000000000178 ) ;
#20694=CARTESIAN_POINT ( 'NONE',  ( -188.7701102708081180, -43.14144101424763278, -23.55033952083658022 ) ) ;
#20697=ADVANCED_FACE ( 'NONE', ( #3905 ), #25928, .T. ) ;
#20698=EDGE_CURVE ( 'NONE', #17509, #23238, #5815, .T. ) ;
#20700=CARTESIAN_POINT ( 'NONE',  ( 136.1360204305621551, -24.77266263493081766, -31.79587985999290112 ) ) ;
#20701=FACE_OUTER_BOUND ( 'NONE', #6789, .T. ) ;
#20703=CARTESIAN_POINT ( 'NONE',  ( 19.06497207195980792, 40.00000000000059686, -54.19242893257802507 ) ) ;
#20704=CARTESIAN_POINT ( 'NONE',  ( 200.0000000000000000, -14.14213562373122457, 42.42640687119282461 ) ) ;
#20705=CARTESIAN_POINT ( 'NONE',  ( -1.818469002956046188, 13.93708913181255049, 47.72215409237453798 ) ) ;
#20706=CARTESIAN_POINT ( 'NONE',  ( -198.0356074513804572, 10.87444709759714989, 10.87444709759722450 ) ) ;
#20707=CARTESIAN_POINT ( 'NONE',  ( -162.0762913951021176, -29.48230308784755493, -27.08623940707632372 ) ) ;
#20710=CARTESIAN_POINT ( 'NONE',  ( 192.4448373802100889, -3.692737725850373501E-14, 19.99999999996060751 ) ) ;
#20712=CARTESIAN_POINT ( 'NONE',  ( 22.17571259161255171, 47.24006242886041917, -13.86510691867242251 ) ) ;
#20713=CARTESIAN_POINT ( 'NONE',  ( -105.3755690713226585, 18.24025645688350750, -40.00000000000002132 ) ) ;
#20714=CARTESIAN_POINT ( 'NONE',  ( 57.59792236341147031, -1.722363176415032004, -1.722363176415048880 ) ) ;
#20715=CARTESIAN_POINT ( 'NONE',  ( -100.7734535825088500, -22.67402823373193499, 40.00000000000002132 ) ) ;
#20717=CARTESIAN_POINT ( 'NONE',  ( -8.720657192106740396, -41.62108041046438700, 22.53512351408631531 ) ) ;
#20719=CARTESIAN_POINT ( 'NONE',  ( 91.82158438592158234, 22.79471317813471742, 40.00000000000002132 ) ) ;
#20720=ORIENTED_EDGE ( 'NONE', *, *, #25603, .F. ) ;
#20722=CARTESIAN_POINT ( 'NONE',  ( 170.2234770963711128, -17.36149277826985937, -17.36149277826995174 ) ) ;
#20724=CARTESIAN_POINT ( 'NONE',  ( -3.696864809823408038, 23.52297716614975442, -43.10456217110547783 ) ) ;
#20726=CARTESIAN_POINT ( 'NONE',  ( -198.0356074513804572, 39.15871834505887250, 17.40982414986519089 ) ) ;
#20728=CARTESIAN_POINT ( 'NONE',  ( -87.11136440741971398, -21.34823163554633041, 2.379156564917666916 ) ) ;
#20729=CARTESIAN_POINT ( 'NONE',  ( -87.13361725327072804, 8.813415818526478339E-15, 21.49321519333429009 ) ) ;
#20730=CARTESIAN_POINT ( 'NONE',  ( -189.5227851117009266, -18.00253723946349993, 43.46196956062881611 ) ) ;
#20731=CARTESIAN_POINT ( 'NONE',  ( 0.2972598230769957217, 1.502051041545559470E-13, -14.33493731733933352 ) ) ;
#20732=CARTESIAN_POINT ( 'NONE',  ( -30.26275506840324070, 1.198031551616724366, -57.76657404653984429 ) ) ;
#20733=CARTESIAN_POINT ( 'NONE',  ( -105.4288953903213581, 9.009229104226067264, -19.35825399500005162 ) ) ;
#20734=CARTESIAN_POINT ( 'NONE',  ( -213.1075012329537230, 37.98287015391280619, -37.98287015391192512 ) ) ;
#20735=CARTESIAN_POINT ( 'NONE',  ( 170.2234770963711128, -17.36149277827010096, 17.36149277826970660 ) ) ;
#20736=CARTESIAN_POINT ( 'NONE',  ( -238.4067589809705794, -40.96449428006345528, 40.00000000000002132 ) ) ;
#20737=CARTESIAN_POINT ( 'NONE',  ( -30.26275506840324070, 41.69427246844628598, 2.449293598294708485E-15 ) ) ;
#20738=CARTESIAN_POINT ( 'NONE',  ( -135.8532207217289738, -1.208299557080134822E-13, 9.153146818113572891 ) ) ;
#20739=CARTESIAN_POINT ( 'NONE',  ( 4.995406935893289102, 10.78321810388998081, 10.78321810389001811 ) ) ;
#20740=CARTESIAN_POINT ( 'NONE',  ( -94.58360650932068836, 20.58386743644652128, -9.000712009836508543 ) ) ;
#20741=CARTESIAN_POINT ( 'NONE',  ( 19.06497207195981858, -10.03556273973377166, -66.60410523465827737 ) ) ;
#20742=CARTESIAN_POINT ( 'NONE',  ( 146.6084372240433709, 52.76785682606519146, 3.800685668858932775 ) ) ;
#20744=CARTESIAN_POINT ( 'NONE',  ( 136.1360204305621266, 3.511608612530704665, 3.511608612530695339 ) ) ;
#20745=CARTESIAN_POINT ( 'NONE',  ( -93.01741312763938652, 8.169811845848039766, 20.82169463896921968 ) ) ;
#20747=CARTESIAN_POINT ( 'NONE',  ( -280.0000000000000568, 42.42640687119274645, 14.14213562373118194 ) ) ;
#20748=CARTESIAN_POINT ( 'NONE',  ( -3.966425590329220263, -47.01685867532416552, -13.83202835294317445 ) ) ;
#20750=CARTESIAN_POINT ( 'NONE',  ( 4.995406935893288214, 15.24977328854832770, 0.000000000000000000 ) ) ;
#20755=CARTESIAN_POINT ( 'NONE',  ( 200.0000000000000000, 19.99999999999995737, 40.00000000000002132 ) ) ;
#20758=CARTESIAN_POINT ( 'NONE',  ( -259.2033419157646676, -49.83842185052040463, 6.730120644403092101 ) ) ;
#20759=CARTESIAN_POINT ( 'NONE',  ( 170.2234770963711128, -40.00000000000004263, 15.44714144992801685 ) ) ;
#20760=CARTESIAN_POINT ( 'NONE',  ( 91.82158438592156813, 39.99999999999995737, 22.79471317813484887 ) ) ;
#20762=CARTESIAN_POINT ( 'NONE',  ( -100.7734535825088500, 22.67402823373189946, -40.00000000000002132 ) ) ;
#20764=CARTESIAN_POINT ( 'NONE',  ( -105.3755690713226585, -18.24025645688353947, -40.00000000000002132 ) ) ;
#20765=CARTESIAN_POINT ( 'NONE',  ( 192.4448373802100889, -14.14213562370313682, 14.14213562370301958 ) ) ;
#20766=CARTESIAN_POINT ( 'NONE',  ( 146.5090579137181237, -12.40347562390430447, -29.94463907179419948 ) ) ;
#20767=CARTESIAN_POINT ( 'NONE',  ( -110.1018001840233893, 14.72021915949438764, -13.84057941999019725 ) ) ;
#20768=CARTESIAN_POINT ( 'NONE',  ( 14.38125909742180930, 40.00000000000060396, -55.17850393974224232 ) ) ;
#20769=CARTESIAN_POINT ( 'NONE',  ( 14.38125909742181818, -1.924622159709266762E-13, 55.17850393972636880 ) ) ;
#20770=CARTESIAN_POINT ( 'NONE',  ( 146.6084372240433709, 3.800685668858776900, -52.76785682606518435 ) ) ;
#20771=DIRECTION ( 'NONE',  ( -0.2259624731739453551, 0.9741360072993472397, 0.000000000000000000 ) ) ;
#20772=CARTESIAN_POINT ( 'NONE',  ( -114.6382724355127749, -18.98542650371856055, 11.21026131167369400 ) ) ;
#20773=CARTESIAN_POINT ( 'NONE',  ( -280.0000000000000568, -42.42640687119285303, -14.14213562373118371 ) ) ;
#20775=CARTESIAN_POINT ( 'NONE',  ( 184.8905102610680444, -14.79361573936399665, 14.79361573936367158 ) ) ;
#20776=CARTESIAN_POINT ( 'NONE',  ( 130.8888609958234213, 29.49786752803547785, -12.21841679119709312 ) ) ;
#20777=CARTESIAN_POINT ( 'NONE',  ( -198.0356074513804572, -55.37879056871328487, -40.00000000000002132 ) ) ;
#20778=CIRCLE ( 'NONE', #24160, 14.99999999999999822 ) ;
#20780=CARTESIAN_POINT ( 'NONE',  ( 192.4448373802101173, -42.42640687122053578, -14.14213562370360577 ) ) ;
#20781=ORIENTED_EDGE ( 'NONE', *, *, #24446, .T. ) ;
#20782=VERTEX_POINT ( 'NONE', #17762 ) ;
#20784=CARTESIAN_POINT ( 'NONE',  ( 110.0479209278586410, 9.419601331808891587, -22.74092928740043362 ) ) ;
#20786=CARTESIAN_POINT ( 'NONE',  ( 6.615221834190998962, 14.16446777328907736, 49.23097633542939633 ) ) ;
#20787=EDGE_LOOP ( 'NONE', ( #657, #14646, #13589, #21110 ) ) ;
#20788=ORIENTED_EDGE ( 'NONE', *, *, #7036, .T. ) ;
#20789=CARTESIAN_POINT ( 'NONE',  ( 151.7948205124836250, -23.49921654116339553, -23.49921654116350211 ) ) ;
#20791=CARTESIAN_POINT ( 'NONE',  ( -114.7824662270406151, -1.403530270408209768, 22.13040512712583308 ) ) ;
#20792=CARTESIAN_POINT ( 'NONE',  ( -162.0762913951021176, 1.198031840315997298, 57.76657433523996588 ) ) ;
#20794=CARTESIAN_POINT ( 'NONE',  ( 170.2234770963711128, 40.00000000000014211, -24.55285855007172913 ) ) ;
#20795=DIRECTION ( 'NONE',  ( 5.508077988093229047E-14, -1.000000000000000000, -1.842899034348521475E-14 ) ) ;
#20796=EDGE_CURVE ( 'NONE', #5450, #5580, #22158, .T. ) ;
#20799=CARTESIAN_POINT ( 'NONE',  ( -238.4067589809705794, 40.00000000000040501, -40.96449427990138759 ) ) ;
#20800=CARTESIAN_POINT ( 'NONE',  ( -213.1075012329537230, 40.00000000000055422, -53.71589010953623244 ) ) ;
#20805=CARTESIAN_POINT ( 'NONE',  ( -188.3392535381692312, 13.83023904993428488, 47.00481007172016490 ) ) ;
#20806=CARTESIAN_POINT ( 'NONE',  ( -192.9588430854690273, -38.51493924976957572, 18.05360324515410397 ) ) ;
#20807=CARTESIAN_POINT ( 'NONE',  ( -77.90255099906769942, -8.064892378657791738, -20.29001641120690635 ) ) ;
#20808=CARTESIAN_POINT ( 'NONE',  ( -30.26275506840323359, -1.198031551616339341, 57.76657404653985139 ) ) ;
#20810=CARTESIAN_POINT ( 'NONE',  ( -213.1075012329536946, -37.98287015391210275, -37.98287015391272092 ) ) ;
#20812=CARTESIAN_POINT ( 'NONE',  ( 19.06497207195981503, -14.19242893257840166, 0.000000000000000000 ) ) ;
#20813=CARTESIAN_POINT ( 'NONE',  ( -280.0000000000000568, 42.42640687119265408, 14.14213562373147504 ) ) ;
#20814=CARTESIAN_POINT ( 'NONE',  ( -162.0762913951021176, -1.694272876828353702, 40.00000000000002132 ) ) ;
#20817=CARTESIAN_POINT ( 'NONE',  ( 57.59792236341149163, -39.99999999999961631, -37.56421063658228832 ) ) ;
#20819=CARTESIAN_POINT ( 'NONE',  ( 156.1979191798867532, -11.34289806466604311, 27.38417834433170484 ) ) ;
#20822=CARTESIAN_POINT ( 'NONE',  ( -192.9588430854689989, 54.46834944099968823, 2.449293598294708485E-15 ) ) ;
#20823=CARTESIAN_POINT ( 'NONE',  ( 155.4809970915717088, 11.45899766888337190, 27.66446758342039658 ) ) ;
#20824=CIRCLE ( 'NONE', #14425, 15.00000000000000178 ) ;
#20825=CARTESIAN_POINT ( 'NONE',  ( -105.2055636156392495, -21.49233843345434991, -1.377569041468663436 ) ) ;
#20827=CARTESIAN_POINT ( 'NONE',  ( 200.0000000000000000, 7.347880794884121511E-14, 0.000000000000000000 ) ) ;
#20830=CARTESIAN_POINT ( 'NONE',  ( -91.56559293963834989, -16.03295912088659492, -40.53558337403696044 ) ) ;
#20831=CARTESIAN_POINT ( 'NONE',  ( 170.2234770963711128, 17.36149277826980253, 17.36149277827007253 ) ) ;
#20833=CARTESIAN_POINT ( 'NONE',  ( 151.7948205124836534, 39.99999999999970157, 33.23291073765595627 ) ) ;
#20834=CARTESIAN_POINT ( 'NONE',  ( -105.4741150117365009, 19.60045294981777531, -8.366608964619008049 ) ) ;
#20835=CARTESIAN_POINT ( 'NONE',  ( -200.0000000000000853, -24.82633483071228753, -44.86878812508721381 ) ) ;
#20836=CARTESIAN_POINT ( 'NONE',  ( 163.1118516004056573, -19.27778845538787422, 19.27778845538743724 ) ) ;
#20837=CARTESIAN_POINT ( 'NONE',  ( -280.0000000000000000, -14.14213562373108779, 14.14213562373088529 ) ) ;
#20840=CARTESIAN_POINT ( 'NONE',  ( 130.8568914410475372, 8.154165912415230659E-16, 5.949712681206690945 ) ) ;
#20841=CARTESIAN_POINT ( 'NONE',  ( 59.93546481429514472, 31.86477106155505012, -13.19882033590626058 ) ) ;
#20842=CARTESIAN_POINT ( 'NONE',  ( -105.3755690713226727, -21.75974354311652093, 0.000000000000000000 ) ) ;
#20843=CARTESIAN_POINT ( 'NONE',  ( -91.56559293963834989, -16.03295912088716335, 40.53558337403673306 ) ) ;
#20844=CARTESIAN_POINT ( 'NONE',  ( -56.48582580120559982, -9.153146818113595984, 40.00000000000002132 ) ) ;
#20845=CARTESIAN_POINT ( 'NONE',  ( 12.96694272558651839, -49.19577900139863402, 14.15914421028645798 ) ) ;
#20846=CARTESIAN_POINT ( 'NONE',  ( -56.48582580120559982, 30.84685318188643421, 40.00000000000002132 ) ) ;
#20848=CARTESIAN_POINT ( 'NONE',  ( 48.46027422359919967, -18.19770396007739066, -35.02097763790794716 ) ) ;
#20849=CARTESIAN_POINT ( 'NONE',  ( -77.58728853844743867, 17.56910682997003192, 13.48988187297745966 ) ) ;
#20850=CARTESIAN_POINT ( 'NONE',  ( -24.15343516389543055, -15.53299357113722934, 37.49996374338925165 ) ) ;
#20852=CARTESIAN_POINT ( 'NONE',  ( -4.421177063217966108, 23.37490463203949886, -42.89273859401248501 ) ) ;
#20854=CARTESIAN_POINT ( 'NONE',  ( -86.96347745069644475, -15.38646221621807442, 15.38646221621768184 ) ) ;
#20855=CARTESIAN_POINT ( 'NONE',  ( -199.9999999999999432, 14.17215463606722636, -49.28189405767596298 ) ) ;
#20856=CARTESIAN_POINT ( 'NONE',  ( -188.6013942375887495, -23.51434495930345037, 43.09289976588207338 ) ) ;
#20857=CARTESIAN_POINT ( 'NONE',  ( 130.8568914410475372, -3.326198072800416995E-13, 34.05028731879788495 ) ) ;
#20858=CARTESIAN_POINT ( 'NONE',  ( -259.2033419157646676, -35.01439189186523748, -21.55415060305881170 ) ) ;
#20859=CARTESIAN_POINT ( 'NONE',  ( 151.7948205124836250, 23.49921654116328540, 23.49921654116366554 ) ) ;
#20860=CARTESIAN_POINT ( 'NONE',  ( -259.2033419157646676, 35.01439189186559275, -21.55415060305807984 ) ) ;
#20861=CARTESIAN_POINT ( 'NONE',  ( -162.0762913951021176, 57.76657433523994456, -1.198031840315424867 ) ) ;
#20862=CARTESIAN_POINT ( 'NONE',  ( -30.26275506840324070, 1.198031551616030033, -1.198031551616006496 ) ) ;
#20863=CARTESIAN_POINT ( 'NONE',  ( -213.1075012329537230, -53.71589010950170717, 40.00000000000002132 ) ) ;
#20864=CARTESIAN_POINT ( 'NONE',  ( -192.9588430854690273, 14.46834944099966336, -40.00000000000002132 ) ) ;
#20865=CARTESIAN_POINT ( 'NONE',  ( 163.1118516004056573, -40.00000000000027711, 27.26290988616830546 ) ) ;
#20866=CARTESIAN_POINT ( 'NONE',  ( 200.0000000000000000, 14.14213562373100608, -42.42640687119291698 ) ) ;
#20869=CARTESIAN_POINT ( 'NONE',  ( -91.56559293963834989, 16.03295912088740849, -40.53558337403661938 ) ) ;
#20871=CARTESIAN_POINT ( 'NONE',  ( -183.1090696429828881, 45.18841929383577138, -13.45963186434148184 ) ) ;
#20873=CARTESIAN_POINT ( 'NONE',  ( -213.1075012329537230, 37.98287015391228749, 37.98287015391245802 ) ) ;
#20877=CARTESIAN_POINT ( 'NONE',  ( -188.2995950289364089, -13.82811170417104840, -46.99046209955525200 ) ) ;
#20878=CARTESIAN_POINT ( 'NONE',  ( 130.8568914410475372, -4.207082182992846420, 4.207082182992822439 ) ) ;
#20879=CARTESIAN_POINT ( 'NONE',  ( 13.08024833513275453, -44.78264744452988566, -18.54957993048723708 ) ) ;
#20882=ORIENTED_EDGE ( 'NONE', *, *, #8428, .F. ) ;
#20883=CARTESIAN_POINT ( 'NONE',  ( -56.48582580120559271, -9.153146818113595984, 0.000000000000000000 ) ) ;
#20884=CARTESIAN_POINT ( 'NONE',  ( -200.0000000000000000, -39.01096890182076038, 39.01096890182031274 ) ) ;
#20886=CARTESIAN_POINT ( 'NONE',  ( 21.15358250000285878, 13.91686544622536914, -47.58740525741993821 ) ) ;
#20887=CARTESIAN_POINT ( 'NONE',  ( 91.82158438592158234, 22.79471317813471742, 40.00000000000002132 ) ) ;
#20892=CARTESIAN_POINT ( 'NONE',  ( -238.4067589809705794, -57.25054294077233408, -0.6820004458489551391 ) ) ;
#20893=CARTESIAN_POINT ( 'NONE',  ( -86.96347745069643054, -40.00000000000009948, 18.24025645688337960 ) ) ;
#20894=CARTESIAN_POINT ( 'NONE',  ( 170.2234770963711128, 40.00000000000014211, -24.55285855007172913 ) ) ;
#20896=CARTESIAN_POINT ( 'NONE',  ( -86.96347745069644475, -18.24025645688354302, -2.449293598294708485E-15 ) ) ;
#20897=CARTESIAN_POINT ( 'NONE',  ( 22.17571259161159603, -13.86510691867019318, -47.24006242886260054 ) ) ;
#20899=CARTESIAN_POINT ( 'NONE',  ( 19.06497207195982924, -54.19242893257843008, -40.00000000000002132 ) ) ;
#20900=CARTESIAN_POINT ( 'NONE',  ( 130.8568914410475088, 24.07718906446891793, 32.49135343045489321 ) ) ;
#20901=CARTESIAN_POINT ( 'NONE',  ( 144.9504669809062705, -12.48392651407822740, -30.13886470195703282 ) ) ;
#20903=CARTESIAN_POINT ( 'NONE',  ( -56.48582580120559982, 40.00000000000034106, -30.84685318188602210 ) ) ;
#20904=CARTESIAN_POINT ( 'NONE',  ( 4.995406935893292655, 39.99999999999982947, 55.24977328856478209 ) ) ;
#20905=CARTESIAN_POINT ( 'NONE',  ( 19.06497207195980792, 10.03556273973433299, 10.03556273973436319 ) ) ;
#20906=CARTESIAN_POINT ( 'NONE',  ( 23.37394308801976806, 42.85717664514618264, -23.33966569535049373 ) ) ;
#20908=CARTESIAN_POINT ( 'NONE',  ( -213.1075012329537230, -66.26714140138676612, 9.698598906462487790 ) ) ;
#20909=ORIENTED_EDGE ( 'NONE', *, *, #5708, .F. ) ;
#20910=CARTESIAN_POINT ( 'NONE',  ( 192.4448373802100889, 14.14213562375873678, 14.14213562375894817 ) ) ;
#20911=CARTESIAN_POINT ( 'NONE',  ( -24.51100708737205736, 37.39427017785519780, -15.48921386273512013 ) ) ;
#20912=CARTESIAN_POINT ( 'NONE',  ( 153.3020327024397602, 28.42252382389430565, -11.77299484472932711 ) ) ;
#20913=CARTESIAN_POINT ( 'NONE',  ( -213.1075012329536946, -53.71589010951918652, -2.449293598294708485E-15 ) ) ;
#20914=CARTESIAN_POINT ( 'NONE',  ( -188.2995950289364941, -43.00522595870984333, 23.44932284465888728 ) ) ;
#20918=CARTESIAN_POINT ( 'NONE',  ( -99.29480781227090347, 8.934325994365451606, -20.48155342677145541 ) ) ;
#20919=CARTESIAN_POINT ( 'NONE',  ( -93.01854144614549114, 8.553566903984137326, -20.65013722627613646 ) ) ;
#20920=CARTESIAN_POINT ( 'NONE',  ( 22.80622392652794517, 17.87980911537470874, 43.16567765897936937 ) ) ;
#20923=EDGE_LOOP ( 'NONE', ( #14217, #13806, #9098, #4254 ) ) ;
#20924=CARTESIAN_POINT ( 'NONE',  ( -213.1075012329537230, 9.698598906462684965, 66.26714140138669507 ) ) ;
#20926=CARTESIAN_POINT ( 'NONE',  ( -105.3901353554229701, -6.689050419637368350, 20.30436174852050968 ) ) ;
#20927=CARTESIAN_POINT ( 'NONE',  ( 151.7948205124836534, -51.78348778862535795, 4.785054706298367044 ) ) ;
#20929=CARTESIAN_POINT ( 'NONE',  ( -280.0000000000000568, 39.99999999999990763, 20.00000000000015987 ) ) ;
#20930=CARTESIAN_POINT ( 'NONE',  ( -199.9999999999999716, -23.83302776610003093, 44.89135967046721731 ) ) ;
#20932=CARTESIAN_POINT ( 'NONE',  ( -30.26275506840323359, 4.336144384597734078E-13, -41.69427246844629309 ) ) ;
#20933=CARTESIAN_POINT ( 'NONE',  ( -135.8532207217289738, -1.208299557080134822E-13, 9.153146818113572891 ) ) ;
#20936=CARTESIAN_POINT ( 'NONE',  ( -87.02159731754392169, -18.50722648783487756, -10.86245144029295595 ) ) ;
#20938=CARTESIAN_POINT ( 'NONE',  ( -183.1090696430172784, 22.43564075022590032, 41.47043467732703448 ) ) ;
#20939=CARTESIAN_POINT ( 'NONE',  ( 0.2972598230770027716, -38.42060263243681817, 18.14793986248684377 ) ) ;
#20941=CARTESIAN_POINT ( 'NONE',  ( 163.1118516004056573, -9.006482792069636645, 9.006482792069567367 ) ) ;
#20942=CARTESIAN_POINT ( 'NONE',  ( -77.65695844554161908, -18.42387585928431903, 12.10528775144916125 ) ) ;
#20943=CARTESIAN_POINT ( 'NONE',  ( -238.4067589809705794, -0.6820004457337348613, -57.25054294065803617 ) ) ;
#20945=CARTESIAN_POINT ( 'NONE',  ( 130.8568914410475088, 34.05028731879790627, 40.00000000000002132 ) ) ;
#20946=CARTESIAN_POINT ( 'NONE',  ( -213.1075012329537230, 37.98287015391211696, 18.58567234101190735 ) ) ;
#20947=CARTESIAN_POINT ( 'NONE',  ( 136.1360204305621266, 35.03383547441298873, 0.000000000000000000 ) ) ;
#20949=EDGE_LOOP ( 'NONE', ( #2920, #13062 ) ) ;
#20950=CARTESIAN_POINT ( 'NONE',  ( 130.8568914410475372, 8.880724697947696879E-14, -5.949712681206690945 ) ) ;
#20955=CARTESIAN_POINT ( 'NONE',  ( 151.7948205124836250, 6.767089262349059275, 2.449293598294708485E-15 ) ) ;
#20956=CARTESIAN_POINT ( 'NONE',  ( -110.0904723790853694, -19.95170499002752962, 3.161343376076289235 ) ) ;
#20958=CARTESIAN_POINT ( 'NONE',  ( 146.6084372240433709, -39.99999999999987921, -34.62501878078319351 ) ) ;
#20961=CARTESIAN_POINT ( 'NONE',  ( -100.7734535825088500, -44.31723036834885932, -12.25131212657538171 ) ) ;
#20962=CARTESIAN_POINT ( 'NONE',  ( -91.56559293963836410, 16.03295912088692177, 16.03295912088721664 ) ) ;
#20963=CARTESIAN_POINT ( 'NONE',  ( -109.1264249741455359, -13.72187187124633212, -33.12752917268956310 ) ) ;
#20964=CARTESIAN_POINT ( 'NONE',  ( 192.4448373802101173, 39.99999999999985079, 20.00000000003984013 ) ) ;
#20965=CARTESIAN_POINT ( 'NONE',  ( -213.1075012329537230, -9.698598906450422774, -9.698598906450550672 ) ) ;
#20966=CARTESIAN_POINT ( 'NONE',  ( -192.9588430854689989, -14.46834944099973086, 0.000000000000000000 ) ) ;
#20967=CARTESIAN_POINT ( 'NONE',  ( -162.0762913951020892, 29.48230308784758691, 29.48230308784772191 ) ) ;
#20968=ADVANCED_FACE ( 'NONE', ( #13996 ), #4025, .T. ) ;
#20969=CARTESIAN_POINT ( 'NONE',  ( 130.8568914410475088, -32.49135343045460900, -24.07718906446924478 ) ) ;
#20970=CARTESIAN_POINT ( 'NONE',  ( -259.2033419157646676, 9.517827891722584255, -0.000000000000000000 ) ) ;
#20972=CARTESIAN_POINT ( 'NONE',  ( 192.4448373802100889, 1.051811698935164031E-13, -20.00000000003942091 ) ) ;
#20973=CARTESIAN_POINT ( 'NONE',  ( 14.38125909742180752, 15.17850393972634038, 0.000000000000000000 ) ) ;
#20974=CARTESIAN_POINT ( 'NONE',  ( 57.59792236341147031, -30.00663442387700641, 26.56190807104681895 ) ) ;
#20975=CARTESIAN_POINT ( 'NONE',  ( 14.38125909742180752, 15.17850393972634038, 40.00000000000002132 ) ) ;
#20977=CARTESIAN_POINT ( 'NONE',  ( 16.10036699863115217, -44.47262139759284594, 24.53427828610336903 ) ) ;
#20978=CARTESIAN_POINT ( 'NONE',  ( 170.2234770963711128, 15.44714144992819094, 2.449293598294708485E-15 ) ) ;
#20979=EDGE_LOOP ( 'NONE', ( #691, #10491, #5619, #21719 ) ) ;
#20981=CARTESIAN_POINT ( 'NONE',  ( 4.995406935893289102, 10.78321810388998081, 10.78321810389001811 ) ) ;
#20982=CARTESIAN_POINT ( 'NONE',  ( -62.69292774200316387, -11.76166271883654701, 24.97541154609807634 ) ) ;
#20983=CARTESIAN_POINT ( 'NONE',  ( -105.3755690713226727, -15.38646221621786481, -15.38646221621789856 ) ) ;
#20984=CARTESIAN_POINT ( 'NONE',  ( 21.99343714674524364, -13.87412077874951954, -47.30053030063390906 ) ) ;
#20986=CARTESIAN_POINT ( 'NONE',  ( 192.4448373802101173, 14.14213562370261279, 42.42640687122091236 ) ) ;
#20987=CARTESIAN_POINT ( 'NONE',  ( -77.58513204269964092, -21.97516623137529379, 2.423266694425164847 ) ) ;
#20988=CARTESIAN_POINT ( 'NONE',  ( -194.7884774423581007, -18.40784251727884779, 44.44046305925472495 ) ) ;
#20989=CARTESIAN_POINT ( 'NONE',  ( -213.1075012329537230, -9.698598906450422774, -9.698598906450550672 ) ) ;
#20990=CARTESIAN_POINT ( 'NONE',  ( -198.0356074513804572, -10.87444709759729911, 10.87444709759714812 ) ) ;
#20991=CARTESIAN_POINT ( 'NONE',  ( 91.82158438592158234, -40.45024623143936537, -16.11829626348475131 ) ) ;
#20992=CARTESIAN_POINT ( 'NONE',  ( 19.06497207195981147, -10.03556273973425483, -10.03556273973443247 ) ) ;
#20993=CARTESIAN_POINT ( 'NONE',  ( 4.995406935893293543, -10.78321810388990265, -10.78321810389009272 ) ) ;
#20994=CARTESIAN_POINT ( 'NONE',  ( -135.8532207217289738, 21.81201906317798134, -21.81201906317747685 ) ) ;
#20995=CARTESIAN_POINT ( 'NONE',  ( 19.06497207195979726, 38.31983398719604139, 18.24870850772803976 ) ) ;
#20996=CARTESIAN_POINT ( 'NONE',  ( -259.2033419157646676, 9.517827891722584255, -0.000000000000000000 ) ) ;
#20997=CARTESIAN_POINT ( 'NONE',  ( 146.6084372240433709, -34.62501878078303008, -40.00000000000002132 ) ) ;
#20998=CARTESIAN_POINT ( 'NONE',  ( -192.9588430854690273, 38.51493924976939098, -18.05360324515436687 ) ) ;
#21000=CARTESIAN_POINT ( 'NONE',  ( 151.7948205124836534, -33.06932595376376582, 23.49921654115996006 ) ) ;
#21001=CARTESIAN_POINT ( 'NONE',  ( -114.4364955367344834, 20.29001642038889841, -8.064892380842916708 ) ) ;
#21003=CARTESIAN_POINT ( 'NONE',  ( 136.1360204305621551, -24.77266263493126885, 31.79587985999256006 ) ) ;
#21005=CARTESIAN_POINT ( 'NONE',  ( -198.0356074513804572, -10.87444709760996986, 67.44298959253333692 ) ) ;
#21006=CARTESIAN_POINT ( 'NONE',  ( 3.869409319527063129, -44.61273074174947340, -24.63759630013054647 ) ) ;
#21009=CARTESIAN_POINT ( 'NONE',  ( -114.7826396787322665, -15.64922767586158336, -15.64922767586183738 ) ) ;
#21011=CARTESIAN_POINT ( 'NONE',  ( -114.7469200037856325, -21.93717741968544743, 2.762404124414108875 ) ) ;
#21013=CARTESIAN_POINT ( 'NONE',  ( -208.1127848780264742, 55.00245453010919050, -40.00000000000002132 ) ) ;
#21017=CARTESIAN_POINT ( 'NONE',  ( 151.7948205124835681, -4.785054706298876859, 51.78348778862533663 ) ) ;
#21018=CARTESIAN_POINT ( 'NONE',  ( 163.1118516004056573, -40.00000000000003553, 12.73709011382460687 ) ) ;
#21019=CARTESIAN_POINT ( 'NONE',  ( 184.8905102610680444, 39.99999999999999289, 19.07866798485573057 ) ) ;
#21021=CARTESIAN_POINT ( 'NONE',  ( 0.2972598230770129857, -54.33493731733936016, -40.00000000000002132 ) ) ;
#21022=CARTESIAN_POINT ( 'NONE',  ( 22.90311673802995784, -23.44499648834451122, -42.99920082299706792 ) ) ;
#21025=CARTESIAN_POINT ( 'NONE',  ( -238.4067589809705794, -40.96449428006345528, 40.00000000000002132 ) ) ;
#21027=CARTESIAN_POINT ( 'NONE',  ( -105.3755690713226585, 43.67073346367970288, 12.89780903124427702 ) ) ;
#21028=CARTESIAN_POINT ( 'NONE',  ( 127.8236149080041457, -11.91256696755843336, -28.75948073575753128 ) ) ;
#21030=CARTESIAN_POINT ( 'NONE',  ( -280.0000000000000568, 40.00000000000017764, -19.99999999999959144 ) ) ;
#21031=CARTESIAN_POINT ( 'NONE',  ( -162.0762913951020892, 1.198031840385716418, 1.198031840385750169 ) ) ;
#21032=CARTESIAN_POINT ( 'NONE',  ( 98.29820294268191105, -7.653668647302824368, -18.47759065022797031 ) ) ;
#21034=CARTESIAN_POINT ( 'NONE',  ( 200.0000000000000000, 14.14213562373083022, 42.42640687119289566 ) ) ;
#21036=CARTESIAN_POINT ( 'NONE',  ( -77.61378591600549726, 3.452311433137887242, -21.81972450369060113 ) ) ;
#21037=CARTESIAN_POINT ( 'NONE',  ( -8.197988474444796836, 42.01088836873199739, -17.40147972966091316 ) ) ;
#21039=CARTESIAN_POINT ( 'NONE',  ( -30.26275506840322649, -41.69427246844630019, -2.449293598294708485E-15 ) ) ;
#21042=CARTESIAN_POINT ( 'NONE',  ( -189.0540043420996028, 43.34487664254652373, -17.95403576473043827 ) ) ;
#21043=ORIENTED_EDGE ( 'NONE', *, *, #3001, .F. ) ;
#21044=ORIENTED_EDGE ( 'NONE', *, *, #14380, .T. ) ;
#21045=FACE_OUTER_BOUND ( 'NONE', #830, .T. ) ;
#21046=CARTESIAN_POINT ( 'NONE',  ( -88.37877758188231780, 8.026456973467151812, -20.15391234951717792 ) ) ;
#21048=ORIENTED_EDGE ( 'NONE', *, *, #21919, .T. ) ;
#21049=CARTESIAN_POINT ( 'NONE',  ( -208.1127848780264742, -17.67593391476659548, 38.89260858015730804 ) ) ;
#21051=CARTESIAN_POINT ( 'NONE',  ( -110.1003821002462786, 1.261039542895549426, 20.16525298253472442 ) ) ;
#21052=CARTESIAN_POINT ( 'NONE',  ( 163.1118516004056573, -47.56205970284957374, 9.006482792074162802 ) ) ;
#21053=CARTESIAN_POINT ( 'NONE',  ( -105.2054292635175585, 21.49321519473984665, 5.610018989487960791E-28 ) ) ;
#21054=CARTESIAN_POINT ( 'NONE',  ( -259.2033419157646676, 39.99999999999987210, 30.48217210827754542 ) ) ;
#21055=CARTESIAN_POINT ( 'NONE',  ( -193.0908841288064650, -24.29092413197462008, 44.14257353178379617 ) ) ;
#21057=CARTESIAN_POINT ( 'NONE',  ( -86.96347745069643054, -40.00000000000026290, 21.75974354311608749 ) ) ;
#21058=AXIS2_PLACEMENT_3D ( 'NONE', #7994, #22, #15977 ) ;
#21059=CARTESIAN_POINT ( 'NONE',  ( -91.56559293963834989, -2.543181659092656077E-13, 22.67402823373191723 ) ) ;
#21061=CARTESIAN_POINT ( 'NONE',  ( 23.37394308801976806, -13.80096434448233111, -46.80823611210209378 ) ) ;
#21063=CARTESIAN_POINT ( 'NONE',  ( -189.0540043421010807, 17.95403576473130869, 43.34487664254734085 ) ) ;
#21064=CARTESIAN_POINT ( 'NONE',  ( 91.82158438592158234, 12.16597498397756993, 12.16597498397776356 ) ) ;
#21066=CARTESIAN_POINT ( 'NONE',  ( -259.2033419157646676, 6.730120644403214669, 49.83842185052034068 ) ) ;
#21067=CARTESIAN_POINT ( 'NONE',  ( -77.66977424857952883, 21.51855955734878023, -4.737087604909469896 ) ) ;
#21069=CIRCLE ( 'NONE', #3225, 60.00000000000011369 ) ;
#21070=CARTESIAN_POINT ( 'NONE',  ( -91.56559293963834989, 16.03295912088740849, -40.53558337403661938 ) ) ;
#21074=CARTESIAN_POINT ( 'NONE',  ( 184.8905102610680444, -14.79361573936399665, 14.79361573936367158 ) ) ;
#21075=CARTESIAN_POINT ( 'NONE',  ( -91.56559293963836410, 22.67402823373190301, 40.00000000000002132 ) ) ;
#21078=CARTESIAN_POINT ( 'NONE',  ( 184.8905102610680444, -39.99999999999978684, -19.07866798485600768 ) ) ;
#21085=CARTESIAN_POINT ( 'NONE',  ( 4.995406935893288214, 55.24977328853207581, 40.00000000000002132 ) ) ;
#21089=CARTESIAN_POINT ( 'NONE',  ( -105.2333497862505141, -21.31134136416374147, 2.723647965523766423 ) ) ;
#21090=CARTESIAN_POINT ( 'NONE',  ( 98.29820294267528880, -14.14213562373450017, -14.14213562373441668 ) ) ;
#21093=APPLICATION_CONTEXT ( 'automotive_design' ) ;
#21094=CIRCLE ( 'NONE', #23221, 15.00000000000000355 ) ;
#21096=CARTESIAN_POINT ( 'NONE',  ( 151.7948205124836534, -23.49921654115981084, -33.06932595376387951 ) ) ;
#21097=CARTESIAN_POINT ( 'NONE',  ( -86.96347745069644475, 15.38646221621772092, 15.38646221621800336 ) ) ;
#21098=CARTESIAN_POINT ( 'NONE',  ( -114.7826396784770822, -16.62870539743747855, -14.66974995413669092 ) ) ;
#21099=CARTESIAN_POINT ( 'NONE',  ( 200.0000000000000000, 40.00000000000026290, -19.99999999999950617 ) ) ;
#21100=CARTESIAN_POINT ( 'NONE',  ( 199.9999999999999432, 14.14213562373093680, 14.14213562373114641 ) ) ;
#21101=CARTESIAN_POINT ( 'NONE',  ( -105.3755690713226869, 21.75974354311648540, -0.000000000000000000 ) ) ;
#21102=CARTESIAN_POINT ( 'NONE',  ( -30.26275506840322649, -29.48230279907810925, 29.48230279907778950 ) ) ;
#21105=CARTESIAN_POINT ( 'NONE',  ( -135.8532207217289738, 40.00000000000002842, -9.153146818113432559 ) ) ;
#21107=CARTESIAN_POINT ( 'NONE',  ( -100.7734535825088358, -22.67402823373193499, 0.000000000000000000 ) ) ;
#21108=CARTESIAN_POINT ( 'NONE',  ( 91.82158438592158234, -40.45024623143958564, 16.11829626348418998 ) ) ;
#21109=CARTESIAN_POINT ( 'NONE',  ( -208.1127848780264742, 55.00245453014418473, 40.00000000000002132 ) ) ;
#21110=ORIENTED_EDGE ( 'NONE', *, *, #25555, .T. ) ;
#21111=CARTESIAN_POINT ( 'NONE',  ( 6.011245401506787545, -44.78331514753931231, 18.54985650214110748 ) ) ;
#21112=CARTESIAN_POINT ( 'NONE',  ( 19.06497207195980792, 14.19242893257840699, -40.00000000000002132 ) ) ;
#21113=EDGE_CURVE ( 'NONE', #12221, #12267, #8985, .T. ) ;
#21114=CARTESIAN_POINT ( 'NONE',  ( 170.0000000000000284, -24.25569233607176756, -6.285860131565255138 ) ) ;
#21116=CARTESIAN_POINT ( 'NONE',  ( 91.82158438592158234, 16.11829626346139577, 16.11829626346143840 ) ) ;
#21117=CARTESIAN_POINT ( 'NONE',  ( 57.59792236341148453, -40.00000000000000000, -2.435789363418300546 ) ) ;
#21118=CARTESIAN_POINT ( 'NONE',  ( -87.11465200126595221, 21.36863955987802655, -2.590445302511781289 ) ) ;
#21119=EDGE_CURVE ( 'NONE', #23459, #14634, #7402, .T. ) ;
#21120=CARTESIAN_POINT ( 'NONE',  ( 21.15737826136113853, -13.91467835516619367, -47.57244852138559565 ) ) ;
#21122=CARTESIAN_POINT ( 'NONE',  ( 91.82158438592158234, 16.11829626348378142, 40.45024623143977749 ) ) ;
#21123=ADVANCED_FACE ( 'NONE', ( #4309 ), #24047, .T. ) ;
#21125=CARTESIAN_POINT ( 'NONE',  ( -87.08870976744344716, 3.405966936676973589, 21.20092391030562595 ) ) ;
#21126=CARTESIAN_POINT ( 'NONE',  ( -189.1288815661669958, -13.87115472123802462, 47.28031329128408800 ) ) ;
#21127=CARTESIAN_POINT ( 'NONE',  ( 146.6084372240433993, -3.357462877844280890E-13, 34.62501878078305850 ) ) ;
#21129=CARTESIAN_POINT ( 'NONE',  ( -91.56559293963834989, 16.03295912088683650, 40.53558337403684675 ) ) ;
#21131=CARTESIAN_POINT ( 'NONE',  ( -56.48582580120559982, 34.75652343174628101, -21.81201906317743067 ) ) ;
#21132=CARTESIAN_POINT ( 'NONE',  ( -135.8532207217289738, 6.472252184284096543, 6.472252184284234211 ) ) ;
#21133=CARTESIAN_POINT ( 'NONE',  ( 130.8568914410475372, 4.207082182992923691, -4.207082182992794017 ) ) ;
#21134=CARTESIAN_POINT ( 'NONE',  ( -280.0000000000000000, 14.14213562373108246, -14.14213562373078581 ) ) ;
#21135=CARTESIAN_POINT ( 'NONE',  ( -86.96347745069644475, -21.75974354311651737, 0.000000000000000000 ) ) ;
#21136=CARTESIAN_POINT ( 'NONE',  ( -56.48582580120559271, -6.472252184284187138, -6.472252184284199572 ) ) ;
#21138=CARTESIAN_POINT ( 'NONE',  ( -198.0356074513804572, -67.44298959253333692, -10.87444709761016348 ) ) ;
#21139=CARTESIAN_POINT ( 'NONE',  ( -114.4388184736442469, 20.16431396440428614, -8.352332320010020794 ) ) ;
#21141=CARTESIAN_POINT ( 'NONE',  ( -56.48582580120559982, -6.472252184284282173, 50.09629031063965243 ) ) ;
#21142=AXIS2_PLACEMENT_3D ( 'NONE', #7153, #793, #15514 ) ;
#21144=CARTESIAN_POINT ( 'NONE',  ( -192.9588430854690273, 18.05360324515418924, 38.51493924976949756 ) ) ;
#21145=CARTESIAN_POINT ( 'NONE',  ( -24.15343516395653012, -37.49996374353147388, -15.53299357101481704 ) ) ;
#21147=CARTESIAN_POINT ( 'NONE',  ( -144.0562564044143414, -29.54282788290112904, 14.68019406016581030 ) ) ;
#21149=CARTESIAN_POINT ( 'NONE',  ( -114.5450021253299866, -20.85732849908723097, -6.791646844857083032 ) ) ;
#21150=CARTESIAN_POINT ( 'NONE',  ( 0.2972598230769930017, 14.33493731733933352, -40.00000000000002132 ) ) ;
#21153=CARTESIAN_POINT ( 'NONE',  ( -135.8532207217289738, -50.09629031063973770, 6.472252184283735943 ) ) ;
#21154=CARTESIAN_POINT ( 'NONE',  ( -105.3755690713226585, 39.99999999999993605, 18.24025645688366737 ) ) ;
#21155=CARTESIAN_POINT ( 'NONE',  ( 19.06497207195980792, 39.99999999999983658, 54.19242893257857929 ) ) ;
#21157=CARTESIAN_POINT ( 'NONE',  ( -238.4067589809705794, -40.96449427990185654, -40.00000000000002132 ) ) ;
#21158=CARTESIAN_POINT ( 'NONE',  ( 19.44355705748453289, -18.20455056367453750, -43.94967286773175630 ) ) ;
#21159=CARTESIAN_POINT ( 'NONE',  ( 136.1360204305621266, 24.77266263493138965, -24.77266263493110188 ) ) ;
#21160=CARTESIAN_POINT ( 'NONE',  ( -56.48582580120559982, 9.153146818113574668, 40.00000000000002132 ) ) ;
#21161=CARTESIAN_POINT ( 'NONE',  ( 170.2234770963711128, 17.36149277827004411, -17.36149277826983095 ) ) ;
#21162=CARTESIAN_POINT ( 'NONE',  ( 136.1360204305621266, -3.419521671106983309E-13, 35.03383547441296741 ) ) ;
#21164=CARTESIAN_POINT ( 'NONE',  ( -100.7734535825088500, -40.00000000000027711, 22.67402823373149801 ) ) ;
#21166=CARTESIAN_POINT ( 'NONE',  ( 169.9999999999999716, -22.62041470344880523, -9.369682556672316309 ) ) ;
#21168=CARTESIAN_POINT ( 'NONE',  ( 14.38125909742180752, 17.55144818341448953, 39.01709431150923280 ) ) ;
#21170=CARTESIAN_POINT ( 'NONE',  ( -100.7734535825088500, 16.03295912088691821, 16.03295912088721309 ) ) ;
#21171=CARTESIAN_POINT ( 'NONE',  ( -77.90022806218905771, 20.16431395584832131, -8.352332316461433592 ) ) ;
#21172=CARTESIAN_POINT ( 'NONE',  ( 159.7744820660626885, 25.95909830917692673, -10.75261058663744507 ) ) ;
#21173=CARTESIAN_POINT ( 'NONE',  ( -56.48582580120559982, 9.153146818113574668, 40.00000000000002132 ) ) ;
#21175=CARTESIAN_POINT ( 'NONE',  ( -189.1288337602818501, 47.28029723722971767, -13.87115233298132999 ) ) ;
#21177=EDGE_LOOP ( 'NONE', ( #21849, #18818, #20346, #1592 ) ) ;
#21180=EDGE_CURVE ( 'NONE', #6050, #15177, #11515, .T. ) ;
#21186=CARTESIAN_POINT ( 'NONE',  ( -208.1127848780264742, 10.60833733270764867, 67.17687982763166588 ) ) ;
#21187=CARTESIAN_POINT ( 'NONE',  ( -105.3287628664957651, 20.69538202814367622, 5.523081874391006174 ) ) ;
#21188=CARTESIAN_POINT ( 'NONE',  ( -105.3755690713226585, 40.00000000000007816, -21.75974354311636461 ) ) ;
#21189=CARTESIAN_POINT ( 'NONE',  ( -200.0000000000000284, -47.96425349429453888, 15.65821854886114295 ) ) ;
#21191=CARTESIAN_POINT ( 'NONE',  ( 146.6084372240433709, -39.99999999999993605, -5.374981219217395356 ) ) ;
#21192=CARTESIAN_POINT ( 'NONE',  ( 14.38125909742180930, 40.00000000000060396, -55.17850393974224232 ) ) ;
#21193=CARTESIAN_POINT ( 'NONE',  ( -87.12760505690756929, 16.17310810899977724, 14.16732333546323730 ) ) ;
#21196=CARTESIAN_POINT ( 'NONE',  ( 91.82158438592158234, 12.16597498397773869, -12.16597498397759303 ) ) ;
#21197=CARTESIAN_POINT ( 'NONE',  ( -94.58366989427236149, 8.190486896678876860, 20.91926462023921829 ) ) ;
#21199=( BOUNDED_CURVE ( )  B_SPLINE_CURVE ( 3, ( #1396, #1143, #15360, #23993 ),
 .UNSPECIFIED., .F., .F. ) 
 B_SPLINE_CURVE_WITH_KNOTS ( ( 4, 4 ),
 ( 0.04745072232841010540, 0.05537094628643264571 ),
 .UNSPECIFIED. ) 
 CURVE ( )  GEOMETRIC_REPRESENTATION_ITEM ( )  RATIONAL_B_SPLINE_CURVE ( ( 0.7232313460858100784, 0.7971366613350190367, 0.8893928793064156402, 1.000000000000000000 ) ) 
 REPRESENTATION_ITEM ( '' )  );
#21200=CARTESIAN_POINT ( 'NONE',  ( -77.90255099906772784, 8.644468104261493480, 20.04994828523958361 ) ) ;
#21201=CARTESIAN_POINT ( 'NONE',  ( -213.1075012329537230, -9.698598906450557777, 9.698598906450415669 ) ) ;
#21202=CARTESIAN_POINT ( 'NONE',  ( -82.26533530497846414, -10.28306516078646915, 17.41444274466569198 ) ) ;
#21203=CARTESIAN_POINT ( 'NONE',  ( -100.7734535825088500, -40.53558337403692491, 16.03295912088671571 ) ) ;
#21205=CARTESIAN_POINT ( 'NONE',  ( 17.75917276260965849, 24.33671690504829144, 44.20478326162346860 ) ) ;
#21207=CARTESIAN_POINT ( 'NONE',  ( 151.7948205124836534, 4.785054706297857230, 51.78348778862544322 ) ) ;
#21211=ORIENTED_EDGE ( 'NONE', *, *, #18927, .F. ) ;
#21212=CARTESIAN_POINT ( 'NONE',  ( 4.995406935893306866, -39.99999999999944578, -55.24977328856505920 ) ) ;
#21215=ORIENTED_EDGE ( 'NONE', *, *, #7803, .F. ) ;
#21218=CARTESIAN_POINT ( 'NONE',  ( -213.1075012329537230, 53.71589010951910836, 2.449293598294708485E-15 ) ) ;
#21220=EDGE_CURVE ( 'NONE', #21839, #8490, #12804, .T. ) ;
#21221=CARTESIAN_POINT ( 'NONE',  ( 170.0000000000000284, -19.80854622259133890, -15.47746304364911829 ) ) ;
#21222=CIRCLE ( 'NONE', #11842, 14.99999999999999645 ) ;
#21223=CARTESIAN_POINT ( 'NONE',  ( -77.72892396114286839, -19.09609284691637754, 10.88898768917809434 ) ) ;
#21224=CARTESIAN_POINT ( 'NONE',  ( -259.2033419157646676, -1.438356298054549103E-14, -9.517827891722632216 ) ) ;
#21227=CARTESIAN_POINT ( 'NONE',  ( -56.48582580120559271, -6.472252184284276844, 6.472252184284108978 ) ) ;
#21228=CARTESIAN_POINT ( 'NONE',  ( 136.1360204305621266, -3.511608612531119000, 53.05693388239312469 ) ) ;
#21229=CARTESIAN_POINT ( 'NONE',  ( -86.84962968273566730, 19.67999904273991163, 8.151722510992470916 ) ) ;
#21230=CARTESIAN_POINT ( 'NONE',  ( 14.38125909742182529, -39.99999999999944578, -55.17850393971050238 ) ) ;
#21231=CARTESIAN_POINT ( 'NONE',  ( 170.2234770963711128, 17.36149277826980253, 17.36149277827007253 ) ) ;
#21232=CARTESIAN_POINT ( 'NONE',  ( -91.56559293963834989, -17.32597176626812185, -40.00000000000002132 ) ) ;
#21233=CARTESIAN_POINT ( 'NONE',  ( -56.48582580120558561, 6.472252184283903809, 50.09629031063968796 ) ) ;
#21236=CARTESIAN_POINT ( 'NONE',  ( 91.82158438592156813, 40.00000000000009948, -17.20528682183286051 ) ) ;
#21237=CARTESIAN_POINT ( 'NONE',  ( 192.4448373802100889, -20.00000000003938538, 0.000000000000000000 ) ) ;
#21238=CARTESIAN_POINT ( 'NONE',  ( 91.82158438592158234, -12.16597498400057198, 44.40256751092329779 ) ) ;
#21239=CARTESIAN_POINT ( 'NONE',  ( 146.6084372240433993, -34.62501878078303008, 0.000000000000000000 ) ) ;
#21240=ORIENTED_EDGE ( 'NONE', *, *, #11647, .F. ) ;
#21242=CARTESIAN_POINT ( 'NONE',  ( 3.468680969975848072, -48.91035688726934438, 14.11592159091329712 ) ) ;
#21243=CARTESIAN_POINT ( 'NONE',  ( -100.7734535825088500, 17.32597176626809699, -40.00000000000002132 ) ) ;
#21244=CARTESIAN_POINT ( 'NONE',  ( -86.86493150571114086, -8.366608963953616751, 19.60045294882772993 ) ) ;
#21245=CARTESIAN_POINT ( 'NONE',  ( -30.26275506840323715, 29.48230279907789253, 29.48230279907799556 ) ) ;
#21246=CARTESIAN_POINT ( 'NONE',  ( -86.96347745069644475, 5.999880687339585546E-14, -21.75974354311649961 ) ) ;
#21247=CARTESIAN_POINT ( 'NONE',  ( -77.79205229025097879, 20.86780749215325415, -6.766653315070159103 ) ) ;
#21248=CARTESIAN_POINT ( 'NONE',  ( -3.486753633152344989, -13.85715877881399116, -47.18604396268663947 ) ) ;
#21250=CARTESIAN_POINT ( 'NONE',  ( -105.3755690713226585, 12.89780903124349720, 43.67073346367994446 ) ) ;
#21251=FACE_OUTER_BOUND ( 'NONE', #15985, .T. ) ;
#21253=CARTESIAN_POINT ( 'NONE',  ( -199.0730705747436957, -18.57195860669628473, 44.83667434818101327 ) ) ;
#21254=CARTESIAN_POINT ( 'NONE',  ( 57.59792236341147031, -1.493297263419786540E-14, 2.435789363418160658 ) ) ;
#21256=CARTESIAN_POINT ( 'NONE',  ( 0.2972598230770048811, -10.13633138497510089, 66.70487387989852834 ) ) ;
#21257=CARTESIAN_POINT ( 'NONE',  ( -77.61421004778013355, 12.97751843348148881, -17.87698779688713913 ) ) ;
#21258=CARTESIAN_POINT ( 'NONE',  ( 192.4448373802100889, 14.14213562375873678, 14.14213562375894817 ) ) ;
#21259=CARTESIAN_POINT ( 'NONE',  ( -91.56559293963836410, 16.03295912088692177, 16.03295912088721664 ) ) ;
#21260=CARTESIAN_POINT ( 'NONE',  ( 19.06497207195980792, 66.60410523465830579, -10.03556273973354251 ) ) ;
#21261=CARTESIAN_POINT ( 'NONE',  ( 0.2972598230770011618, 10.13633138497555919, -66.70487387989845729 ) ) ;
#21262=CARTESIAN_POINT ( 'NONE',  ( 163.1118516004056573, -27.26290988616869626, -40.00000000000002132 ) ) ;
#21263=CARTESIAN_POINT ( 'NONE',  ( 200.0000000000000000, 42.42640687119288856, -14.14213562373094746 ) ) ;
#21265=CARTESIAN_POINT ( 'NONE',  ( -162.0762913951021176, -29.48230308784793152, 27.08623940707591515 ) ) ;
#21266=DIRECTION ( 'NONE',  ( 0.000000000000000000, 1.000000000000000000, 0.000000000000000000 ) ) ;
#21267=VERTEX_POINT ( 'NONE', #13560 ) ;
#21268=CARTESIAN_POINT ( 'NONE',  ( 19.06497207195981147, 38.31983398719620482, 38.31983398719633271 ) ) ;
#21269=CARTESIAN_POINT ( 'NONE',  ( -105.4741150117383057, 8.366608964593771347, 19.60045294982731789 ) ) ;
#21270=CARTESIAN_POINT ( 'NONE',  ( -4.121597284766443714, -42.98102224344790301, -23.43330939486633824 ) ) ;
#21272=CARTESIAN_POINT ( 'NONE',  ( -114.4364955367321244, -20.04994829327305084, 8.644468109216932206 ) ) ;
#21276=CARTESIAN_POINT ( 'NONE',  ( 23.32574057153124869, -23.35062444423053662, 42.87194976637110244 ) ) ;
#21277=CARTESIAN_POINT ( 'NONE',  ( 14.38125909742180752, 15.17850393972634038, -40.00000000000002132 ) ) ;
#21278=CARTESIAN_POINT ( 'NONE',  ( 23.37394308801976806, 42.85717664514618264, -23.33966569535049373 ) ) ;
#21280=CARTESIAN_POINT ( 'NONE',  ( -238.4067589809705794, -28.96627169325352469, 27.60227080167035041 ) ) ;
#21281=CARTESIAN_POINT ( 'NONE',  ( 184.8905102610680444, 40.00000000000013500, -20.92133201514430141 ) ) ;
#21282=FACE_OUTER_BOUND ( 'NONE', #13272, .T. ) ;
#21284=CARTESIAN_POINT ( 'NONE',  ( 200.0000000000000000, -19.99999999999988631, -40.00000000000002132 ) ) ;
#21285=CARTESIAN_POINT ( 'NONE',  ( 22.98934664983253029, -17.85845455615937283, -43.11412319250651137 ) ) ;
#21287=CARTESIAN_POINT ( 'NONE',  ( 91.82158438592156813, 17.20528682183302038, 40.00000000000002132 ) ) ;
#21288=CARTESIAN_POINT ( 'NONE',  ( 192.4448373802101173, 42.42640687122070631, 14.14213562370331623 ) ) ;
#21290=CARTESIAN_POINT ( 'NONE',  ( 130.8568914410475088, 39.99999999999969447, 34.05028731879830417 ) ) ;
#21292=CARTESIAN_POINT ( 'NONE',  ( 151.7948205124836534, -40.00000000000034817, 33.23291073765511072 ) ) ;
#21294=CARTESIAN_POINT ( 'NONE',  ( 144.9498910354600696, -30.13892677251539709, -12.48395222454551323 ) ) ;
#21296=CARTESIAN_POINT ( 'NONE',  ( 0.2972598230770048811, -10.13633138497510089, 66.70487387989852834 ) ) ;
#21297=EDGE_LOOP ( 'NONE', ( #18911, #22683, #6670, #994 ) ) ;
#21299=CARTESIAN_POINT ( 'NONE',  ( -4.112199523539896262, 46.96527782736888668, -13.82298295336167904 ) ) ;
#21300=CARTESIAN_POINT ( 'NONE',  ( 0.2972598230770129857, -54.33493731733938148, 40.00000000000002132 ) ) ;
#21302=DIRECTION ( 'NONE',  ( 0.000000000000000000, 0.9307566067255934605, 0.3656393565204090201 ) ) ;
#21305=ORIENTED_EDGE ( 'NONE', *, *, #9386, .T. ) ;
#21306=CARTESIAN_POINT ( 'NONE',  ( -88.39148973765156825, 8.577159256668517529, -19.92926839984427545 ) ) ;
#21307=CARTESIAN_POINT ( 'NONE',  ( 23.37394308801980713, -42.85717664514568526, -23.33966569535099822 ) ) ;
#21308=B_SPLINE_CURVE_WITH_KNOTS ( 'NONE', 3,
 ( #9602, #11995, #5741, #13847, #3896, #21982 ),
 .UNSPECIFIED., .F., .F.,
 ( 4, 2, 4 ),
 ( -0.0001324603514786740893, 0.04003846212279590228, 0.08020938459707047108 ),
 .UNSPECIFIED. ) ;
#21309=CARTESIAN_POINT ( 'NONE',  ( -94.58366989427319993, 8.190486896679173512, -20.91926462023913658 ) ) ;
#21313=CARTESIAN_POINT ( 'NONE',  ( -188.2995950289363805, 23.44932284466059969, -43.00522595870931752 ) ) ;
#21314=CARTESIAN_POINT ( 'NONE',  ( -259.2033419157646676, -35.01439189186554302, 21.55415060305832498 ) ) ;
#21316=CARTESIAN_POINT ( 'NONE',  ( -100.7734535825088358, -16.03295912088706743, -16.03295912088710296 ) ) ;
#21317=CARTESIAN_POINT ( 'NONE',  ( -192.9588430854690273, 39.99999999999980105, 54.46834944098235809 ) ) ;
#21318=CARTESIAN_POINT ( 'NONE',  ( -199.9999999999999716, -44.86878812508714276, 24.82633483071253622 ) ) ;
#21320=CARTESIAN_POINT ( 'NONE',  ( 151.7948205124836534, -40.00000000000034817, 33.23291073765511072 ) ) ;
#21321=CARTESIAN_POINT ( 'NONE',  ( 192.4448373802101173, 40.00000000000026290, -19.99999999996018474 ) ) ;
#21322=CARTESIAN_POINT ( 'NONE',  ( -77.58759120052278035, 17.31422299681156929, 13.74448509166802701 ) ) ;
#21323=CARTESIAN_POINT ( 'NONE',  ( -192.9588430854689989, -10.23066800230756890, 10.23066800230742501 ) ) ;
#21324=CARTESIAN_POINT ( 'NONE',  ( -199.9999999999998010, 24.82633483071100500, -44.86878812508844305 ) ) ;
#21325=CARTESIAN_POINT ( 'NONE',  ( -188.2995950289364089, 43.00522595870987885, -23.44932284465868477 ) ) ;
#21326=CARTESIAN_POINT ( 'NONE',  ( 104.1600437297061461, 20.63676802951782818, 8.548029200544462469 ) ) ;
#21329=CARTESIAN_POINT ( 'NONE',  ( -82.28162732581432692, -9.169756991548416281, 18.01798805100655088 ) ) ;
#21330=AXIS2_PLACEMENT_3D ( 'NONE', #3861, #22360, #5711 ) ;
#21331=CARTESIAN_POINT ( 'NONE',  ( 136.1360204305621551, -31.79587985999279454, 24.77266263493094911 ) ) ;
#21332=CARTESIAN_POINT ( 'NONE',  ( -121.8281150765456147, -10.16552078725611352, -22.46071699959419732 ) ) ;
#21333=DIRECTION ( 'NONE',  ( 0.9698969544411740751, -0.2249791741491982133, 0.09318942517732352326 ) ) ;
#21335=CARTESIAN_POINT ( 'NONE',  ( -259.2033419157646676, -6.730120644402966867, -49.83842185052038332 ) ) ;
#21339=CARTESIAN_POINT ( 'NONE',  ( 14.38125909742181818, -39.99999999999986500, -15.17850393972675604 ) ) ;
#21341=CARTESIAN_POINT ( 'NONE',  ( 23.37394308801977871, -42.85717664514601921, 23.33966569535066071 ) ) ;
#21344=CARTESIAN_POINT ( 'NONE',  ( 200.0000000000000000, 19.99999999999995737, 40.00000000000002132 ) ) ;
#21346=CARTESIAN_POINT ( 'NONE',  ( -135.8532207217289738, 6.472252184284186249, -6.472252184284142729 ) ) ;
#21350=CARTESIAN_POINT ( 'NONE',  ( -77.61378591600585253, -12.98772233503525619, 17.87002798532632042 ) ) ;
#21351=( BOUNDED_SURFACE ( )  B_SPLINE_SURFACE ( 3, 3, ( 
 ( #21570, #23566, #10957, #1097, #23193, #11200, #4974, #25579, #15566, #9457, #13451, #19063, #846, #5219, #19567, #13081, #7202, #21443, #1227, #7325, #21196, #2968, #3343, #17563, #11079, #15439, #5341, #19193, #976, #11444 ),
 ( #16235, #20236, #9719, #1744, #25835, #5726, #24363, #7978, #13830, #1614, #22237, #13967, #7840, #1879, #17822, #6, #15962, #11573, #6001, #16096, #7579, #9983, #15691, #24087, #18094, #7710, #15821, #6127, #23950, #5861 ),
 ( #10119, #14108, #20102, #21963, #22102, #13705, #4012, #11707, #12111, #2017, #18220, #3737, #11840, #9852, #3877, #8118, #24227, #3475, #19961, #17691, #25970, #23816, #26243, #14235, #19692, #1480, #9586, #5598, #11978, #21829 ),
 ( #17955, #3599, #26102, #19828, #546, #4542, #18895, #12638, #14762, #16896, #10652, #22891, #12246, #142, #8245, #8783, #12773, #2271, #20628, #18362, #24626, #25028, #8650, #6383, #20499, #4671, #6514, #410, #20765, #10380 ),
 ( #20368, #18490, #271, #2678, #16501, #6781, #22375, #2535, #8513, #2142, #16632, #10253, #14625, #12500, #10513, #10785, #6647, #18762, #14500, #24761, #6258, #20900, #4281, #22762, #4151, #674, #16363, #24497, #14371, #16758 ),
 ( #22504, #12371, #24892, #8379, #22631, #2402, #4406, #18627, #9048, #21027, #23413, #19155, #19030, #25669, #13043, #23286, #939, #809, #11165, #17153, #6911, #9424, #12910, #25287, #14893, #25418, #15028, #1064, #21288, #2808 ),
 ( #11044, #7044, #23534, #3186, #11411, #3063, #9301, #8915, #17284, #10919, #15161, #23033, #7167, #23158, #9171, #19281, #17024, #5305, #4808, #25160, #4935, #19412, #5190, #13292, #19533, #5062, #21161, #13168, #17405, #13416 ) ),
 .UNSPECIFIED., .T., .F., .T. ) 
 B_SPLINE_SURFACE_WITH_KNOTS ( ( 4, 3, 4 ),
 ( 4, 2, 2, 2, 2, 2, 2, 2, 2, 2, 2, 2, 2, 2, 4 ),
 ( 0.000000000000000000, 0.5000000000000000000, 1.000000000000000000 ),
 ( 0.000000000000000000, 0.1357259735107005372, 0.1651108541090157700, 0.1944957347073310028, 0.3598804999793158710, 0.3867117631979620773, 0.4135430264166082281, 0.5789277916885930964, 0.6062785021374117456, 0.6336292125862302838, 0.8508620842112317728, 0.8814014469398914198, 0.9119408096685510667, 0.9559704048342755334, 1.000000000000000000 ),
 .UNSPECIFIED. ) 
 GEOMETRIC_REPRESENTATION_ITEM ( )  RATIONAL_B_SPLINE_SURFACE ( (
 ( 1.000000000000000000, 1.000000000000000000, 1.000000000000000000, 1.000000000000000000, 1.000000000000000000, 1.000000000000000000, 1.000000000000000000, 1.000000000000000000, 1.000000000000000000, 1.000000000000000000, 1.000000000000000000, 1.000000000000000000, 1.000000000000000000, 1.000000000000000000, 1.000000000000000000, 1.000000000000000000, 1.000000000000000000, 1.000000000000000000, 1.000000000000000000, 1.000000000000000000, 1.000000000000000000, 1.000000000000000000, 1.000000000000000000, 1.000000000000000000, 1.000000000000000000, 1.000000000000000000, 1.000000000000000000, 1.000000000000000000, 1.000000000000000000, 1.000000000000000000),
 ( 0.3333333333333333703, 0.3333333333333333703, 0.3333333333333333703, 0.3333333333333333703, 0.3333333333333333703, 0.3333333333333333703, 0.3333333333333333703, 0.3333333333333333703, 0.3333333333333333703, 0.3333333333333333703, 0.3333333333333333703, 0.3333333333333333703, 0.3333333333333333703, 0.3333333333333333703, 0.3333333333333333703, 0.3333333333333333703, 0.3333333333333333703, 0.3333333333333333703, 0.3333333333333333703, 0.3333333333333333703, 0.3333333333333333703, 0.3333333333333333703, 0.3333333333333333703, 0.3333333333333333703, 0.3333333333333333703, 0.3333333333333333703, 0.3333333333333333703, 0.3333333333333333703, 0.3333333333333333703, 0.3333333333333333703),
 ( 0.3333333333333333703, 0.3333333333333333703, 0.3333333333333333703, 0.3333333333333333703, 0.3333333333333333703, 0.3333333333333333703, 0.3333333333333333703, 0.3333333333333333703, 0.3333333333333333703, 0.3333333333333333703, 0.3333333333333333703, 0.3333333333333333703, 0.3333333333333333703, 0.3333333333333333703, 0.3333333333333333703, 0.3333333333333333703, 0.3333333333333333703, 0.3333333333333333703, 0.3333333333333333703, 0.3333333333333333703, 0.3333333333333333703, 0.3333333333333333703, 0.3333333333333333703, 0.3333333333333333703, 0.3333333333333333703, 0.3333333333333333703, 0.3333333333333333703, 0.3333333333333333703, 0.3333333333333333703, 0.3333333333333333703),
 ( 1.000000000000000000, 1.000000000000000000, 1.000000000000000000, 1.000000000000000000, 1.000000000000000000, 1.000000000000000000, 1.000000000000000000, 1.000000000000000000, 1.000000000000000000, 1.000000000000000000, 1.000000000000000000, 1.000000000000000000, 1.000000000000000000, 1.000000000000000000, 1.000000000000000000, 1.000000000000000000, 1.000000000000000000, 1.000000000000000000, 1.000000000000000000, 1.000000000000000000, 1.000000000000000000, 1.000000000000000000, 1.000000000000000000, 1.000000000000000000, 1.000000000000000000, 1.000000000000000000, 1.000000000000000000, 1.000000000000000000, 1.000000000000000000, 1.000000000000000000),
 ( 0.3333333333333333703, 0.3333333333333333703, 0.3333333333333333703, 0.3333333333333333703, 0.3333333333333333703, 0.3333333333333333703, 0.3333333333333333703, 0.3333333333333333703, 0.3333333333333333703, 0.3333333333333333703, 0.3333333333333333703, 0.3333333333333333703, 0.3333333333333333703, 0.3333333333333333703, 0.3333333333333333703, 0.3333333333333333703, 0.3333333333333333703, 0.3333333333333333703, 0.3333333333333333703, 0.3333333333333333703, 0.3333333333333333703, 0.3333333333333333703, 0.3333333333333333703, 0.3333333333333333703, 0.3333333333333333703, 0.3333333333333333703, 0.3333333333333333703, 0.3333333333333333703, 0.3333333333333333703, 0.3333333333333333703),
 ( 0.3333333333333333703, 0.3333333333333333703, 0.3333333333333333703, 0.3333333333333333703, 0.3333333333333333703, 0.3333333333333333703, 0.3333333333333333703, 0.3333333333333333703, 0.3333333333333333703, 0.3333333333333333703, 0.3333333333333333703, 0.3333333333333333703, 0.3333333333333333703, 0.3333333333333333703, 0.3333333333333333703, 0.3333333333333333703, 0.3333333333333333703, 0.3333333333333333703, 0.3333333333333333703, 0.3333333333333333703, 0.3333333333333333703, 0.3333333333333333703, 0.3333333333333333703, 0.3333333333333333703, 0.3333333333333333703, 0.3333333333333333703, 0.3333333333333333703, 0.3333333333333333703, 0.3333333333333333703, 0.3333333333333333703),
 ( 1.000000000000000000, 1.000000000000000000, 1.000000000000000000, 1.000000000000000000, 1.000000000000000000, 1.000000000000000000, 1.000000000000000000, 1.000000000000000000, 1.000000000000000000, 1.000000000000000000, 1.000000000000000000, 1.000000000000000000, 1.000000000000000000, 1.000000000000000000, 1.000000000000000000, 1.000000000000000000, 1.000000000000000000, 1.000000000000000000, 1.000000000000000000, 1.000000000000000000, 1.000000000000000000, 1.000000000000000000, 1.000000000000000000, 1.000000000000000000, 1.000000000000000000, 1.000000000000000000, 1.000000000000000000, 1.000000000000000000, 1.000000000000000000, 1.000000000000000000) ) ) 
 REPRESENTATION_ITEM ( '' )  SURFACE ( )  );
#21352=CARTESIAN_POINT ( 'NONE',  ( -105.2054292635175727, 15.19799821370213522, 15.19799821370241943 ) ) ;
#21355=CARTESIAN_POINT ( 'NONE',  ( -87.11181970786255135, 13.17799186809413392, 17.01573394368394077 ) ) ;
#21356=CARTESIAN_POINT ( 'NONE',  ( -70.33906594972403070, -9.443630401875100944, -22.79894061986596654 ) ) ;
#21357=CARTESIAN_POINT ( 'NONE',  ( 57.59792236341147031, 1.722363176415040886, 1.722363176415060426 ) ) ;
#21358=CARTESIAN_POINT ( 'NONE',  ( -105.4741150117382631, -19.60045294982879582, -8.366608964590131592 ) ) ;
#21359=CARTESIAN_POINT ( 'NONE',  ( 163.1118516004056573, -39.99999999999986500, -12.73709011382517353 ) ) ;
#21361=CARTESIAN_POINT ( 'NONE',  ( -86.96347745069643054, -18.24025645688353947, -40.00000000000002132 ) ) ;
#21362=EDGE_CURVE ( 'NONE', #22617, #7462, #65, .T. ) ;
#21364=CARTESIAN_POINT ( 'NONE',  ( 57.59792236341148453, -26.56190807104700369, 26.56190807104673723 ) ) ;
#21365=CARTESIAN_POINT ( 'NONE',  ( -100.7734535825088500, -17.32597176626812185, -40.00000000000002132 ) ) ;
#21366=CARTESIAN_POINT ( 'NONE',  ( -110.0305071378944319, 18.66378802528556946, 7.635428997630903325 ) ) ;
#21367=CARTESIAN_POINT ( 'NONE',  ( -162.0762913951020892, -3.568845385355699554E-14, 1.694272876828323948 ) ) ;
#21368=CARTESIAN_POINT ( 'NONE',  ( -86.96347745069644475, -21.75974354311652093, -40.00000000000002132 ) ) ;
#21369=CARTESIAN_POINT ( 'NONE',  ( -162.0762913951020892, 57.76657433537918251, 1.198031840455469066 ) ) ;
#21370=CARTESIAN_POINT ( 'NONE',  ( -30.26275506840324425, 41.69427246844628598, -40.00000000000002132 ) ) ;
#21372=CARTESIAN_POINT ( 'NONE',  ( 22.90311673803729420, -42.99920082299467339, 23.44499648834695549 ) ) ;
#21373=CARTESIAN_POINT ( 'NONE',  ( -83.21262154144248768, 13.72187187061550695, -33.12752917118394436 ) ) ;
#21374=CARTESIAN_POINT ( 'NONE',  ( 146.6084372240433709, -52.76785682606516303, 3.800685668858563737 ) ) ;
#21375=CARTESIAN_POINT ( 'NONE',  ( -56.48582580120558561, -40.00000000000000000, -9.153146818113723882 ) ) ;
#21377=CARTESIAN_POINT ( 'NONE',  ( -70.30307074931239697, 8.711708294051453194, -23.14841682951314894 ) ) ;
#21380=DIRECTION ( 'NONE',  ( 1.000000000000000000, 1.836970198721025990E-16, 0.000000000000000000 ) ) ;
#21381=CARTESIAN_POINT ( 'NONE',  ( 146.6084372240433709, 3.800685668858042821, 52.76785682606522698 ) ) ;
#21382=CARTESIAN_POINT ( 'NONE',  ( -86.96347745069645896, 43.67073346367988762, -12.89780903124366418 ) ) ;
#21383=CARTESIAN_POINT ( 'NONE',  ( 57.59792236341148453, 1.722363176414758668, 54.84617931850880268 ) ) ;
#21385=CARTESIAN_POINT ( 'NONE',  ( -259.2033419157646676, 6.730120644403426944, 6.730120644403592145 ) ) ;
#21386=CARTESIAN_POINT ( 'NONE',  ( 14.38125909742180752, 17.55144818341503665, -39.01709431150898411 ) ) ;
#21387=CARTESIAN_POINT ( 'NONE',  ( 136.1360204305621551, -53.05693388239309627, -3.511608612531332163 ) ) ;
#21388=CARTESIAN_POINT ( 'NONE',  ( 184.8905102610680444, 13.49065550809826952, -13.49065550809790359 ) ) ;
#21389=CARTESIAN_POINT ( 'NONE',  ( -135.8532207217289738, -9.153146818113595984, 0.000000000000000000 ) ) ;
#21391=CARTESIAN_POINT ( 'NONE',  ( -100.7734535825088358, 6.065416334915073333E-14, -22.67402823373191723 ) ) ;
#21392=CARTESIAN_POINT ( 'NONE',  ( -105.3755690713226585, -41.18208027870611687, 15.38646221621750954 ) ) ;
#21393=CARTESIAN_POINT ( 'NONE',  ( -166.7090608787311226, 37.06260950144081079, -15.35183551249070533 ) ) ;
#21395=CARTESIAN_POINT ( 'NONE',  ( 151.7948205124836534, 33.06932595376365924, -23.49921654116018743 ) ) ;
#21396=CARTESIAN_POINT ( 'NONE',  ( -97.72675010090327419, -20.89622088363361385, -8.185591577777390881 ) ) ;
#21397=CARTESIAN_POINT ( 'NONE',  ( 22.13784119382970061, 17.95298715833905234, 43.34234508276811937 ) ) ;
#21398=CARTESIAN_POINT ( 'NONE',  ( -86.95493927446905502, -20.33927854521762058, 6.698173996902891503 ) ) ;
#21400=CARTESIAN_POINT ( 'NONE',  ( -129.2303492451636941, -24.84170067260939874, 11.67678589703593772 ) ) ;
#21402=CARTESIAN_POINT ( 'NONE',  ( 23.72853009152683157, -13.77482773664794458, 46.68009952139140495 ) ) ;
#21403=CARTESIAN_POINT ( 'NONE',  ( 169.9999999999999716, -15.47746304364925329, 19.80854622259126430 ) ) ;
#21405=CARTESIAN_POINT ( 'NONE',  ( -87.10405235694547343, 21.30065104412373245, 2.801403629797663442 ) ) ;
#21406=CARTESIAN_POINT ( 'NONE',  ( 14.38125909742180220, 39.99999999999997158, 15.17850393972647716 ) ) ;
#21407=CARTESIAN_POINT ( 'NONE',  ( 19.06497207195981147, -4.605042221739098431E-14, 14.19242893257840521 ) ) ;
#21408=CARTESIAN_POINT ( 'NONE',  ( -200.0000000000001705, -23.83166235904677777, -44.86667451853072919 ) ) ;
#21409=CARTESIAN_POINT ( 'NONE',  ( 4.995406935893307754, -55.24977328853207581, -40.00000000000002132 ) ) ;
#21410=CARTESIAN_POINT ( 'NONE',  ( 20.17262239841839389, -18.14389419515046242, -43.80323544018617099 ) ) ;
#21412=CARTESIAN_POINT ( 'NONE',  ( 14.38125909742182884, -55.17850393971007605, 40.00000000000002132 ) ) ;
#21413=CARTESIAN_POINT ( 'NONE',  ( -238.4067589809705794, -0.9644942799826262680, 0.000000000000000000 ) ) ;
#21414=CARTESIAN_POINT ( 'NONE',  ( 57.59792236341147031, 40.00000000000042633, -37.56421063658144277 ) ) ;
#21415=CARTESIAN_POINT ( 'NONE',  ( -238.4067589809705794, -39.99999999999963762, -40.96449428006383187 ) ) ;
#21416=EDGE_CURVE ( 'NONE', #23676, #19014, #6154, .T. ) ;
#21417=CARTESIAN_POINT ( 'NONE',  ( 167.0465517065776737, -23.44217192942191730, -9.710065544648454505 ) ) ;
#21419=CARTESIAN_POINT ( 'NONE',  ( 19.06497207195981147, -10.03556273973425483, -10.03556273973443247 ) ) ;
#21420=CARTESIAN_POINT ( 'NONE',  ( 15.76057515052796276, 44.53539632572124418, -18.44716516378320037 ) ) ;
#21421=CARTESIAN_POINT ( 'NONE',  ( 163.1118516004056573, -12.73709011382472589, 40.00000000000002132 ) ) ;
#21422=CARTESIAN_POINT ( 'NONE',  ( -198.9234529668597986, 49.24835336344366965, -14.16707775654091606 ) ) ;
#21424=ORIENTED_EDGE ( 'NONE', *, *, #12719, .T. ) ;
#21426=CARTESIAN_POINT ( 'NONE',  ( -135.8532207217289738, 6.472252184284186249, -6.472252184284142729 ) ) ;
#21427=CARTESIAN_POINT ( 'NONE',  ( 144.9504669809064126, 12.48392651407853471, -30.13886470195694400 ) ) ;
#21433=CARTESIAN_POINT ( 'NONE',  ( 146.6084372240433993, 3.800685668858676980, 3.800685668858667210 ) ) ;
#21434=CARTESIAN_POINT ( 'NONE',  ( -121.8281150760332991, -23.07023398566525074, -8.694016612792475840 ) ) ;
#21435=CARTESIAN_POINT ( 'NONE',  ( 57.59792236341147031, 1.908507979671054758E-14, -2.435789363418160658 ) ) ;
#21436=CARTESIAN_POINT ( 'NONE',  ( 21.15358250000287654, -13.91686544622502097, 47.58740525742008032 ) ) ;
#21438=CARTESIAN_POINT ( 'NONE',  ( 0.2972598230770030492, -39.99999999999987210, -14.33493731733975451 ) ) ;
#21439=CARTESIAN_POINT ( 'NONE',  ( 200.0000000000000000, 40.00000000000026290, -19.99999999999950617 ) ) ;
#21440=CARTESIAN_POINT ( 'NONE',  ( -82.24986055077694402, 16.41205588405924942, 11.76386043655782032 ) ) ;
#21441=CARTESIAN_POINT ( 'NONE',  ( 199.9999999999999432, 14.14213562373113398, -14.14213562373094923 ) ) ;
#21442=CARTESIAN_POINT ( 'NONE',  ( 130.8568914410475372, 1.429239637432775288E-13, -34.05028731879788495 ) ) ;
#21443=CARTESIAN_POINT ( 'NONE',  ( 14.38125909742181285, -10.73282306404727393, 10.73282306404716380 ) ) ;
#21444=CARTESIAN_POINT ( 'NONE',  ( 118.9130007099547299, 25.80693111732287548, 10.68958087202344664 ) ) ;
#21445=EDGE_CURVE ( 'NONE', #17458, #22617, #7099, .T. ) ;
#21446=CARTESIAN_POINT ( 'NONE',  ( 98.29820294271928560, -12.26677183925107428, -16.01749940821211382 ) ) ;
#21447=CARTESIAN_POINT ( 'NONE',  ( 14.38125909742181285, -10.73282306404727393, 10.73282306404716380 ) ) ;
#21448=CARTESIAN_POINT ( 'NONE',  ( -82.25988539630567686, -17.04081484590923168, 10.82485991172919526 ) ) ;
#21449=CARTESIAN_POINT ( 'NONE',  ( 19.06497207195981858, 10.03556273973424062, 66.60410523465820631 ) ) ;
#21450=( BOUNDED_SURFACE ( )  B_SPLINE_SURFACE ( 3, 3, ( 
 ( #638, #2903, #24854, #20989, #24993, #14726, #8878, #6745, #4635, #7135, #18721, #14857, #12601, #23124, #12736, #2638, #2771, #22992, #10880, #10747, #19120, #9130, #903, #18858, #5028, #25250, #22858, #772, #506, #13136 ),
 ( #8743, #8612, #16988, #4768, #25124, #17245, #14990, #25383, #9015, #17120, #15249, #23379, #21382, #13761, #25764, #11773, #25510, #19892, #1281, #9782, #15622, #3278, #17373, #21758, #13259, #5404, #7770, #9389, #11376, #3154 ),
 ( #13504, #19497, #21626, #5154, #3402, #5274, #11504, #23624, #19628, #1413, #17884, #23745, #3665, #17496, #11255, #11632, #9514, #26033, #23500, #15751, #21888, #5526, #1677, #25637, #15885, #19374, #23879, #13633, #1161, #17754 ),
 ( #9265, #7259, #15377, #13379, #17619, #7514, #21506, #3531, #7383, #19754, #15494, #1544, #9649, #25895, #7635, #5656, #1942, #18019, #6315, #18424, #5929, #1810, #24423, #14435, #8311, #24297, #22436, #20430, #3805, #10050 ),
 ( #16434, #22564, #4213, #12041, #16299, #9913, #6065, #18156, #26168, #20299, #26303, #16027, #18561, #22032, #8046, #24011, #8182, #24152, #14036, #14167, #16162, #22300, #22170, #14302, #12435, #6189, #3944, #202, #10318, #7908 ),
 ( #4077, #8444, #11909, #20161, #20032, #12178, #2076, #10183, #4343, #18287, #24560, #73, #5791, #2209, #12303, #13899, #20563, #2334, #10448, #340, #5002, #12703, #21228, #746, #14698, #2467, #6846, #24693, #16831, #19223 ),
 ( #875, #24966, #6713, #14827, #4607, #22959, #16563, #4738, #16693, #12846, #8715, #20962, #2743, #3000, #8850, #15090, #22830, #6448, #23099, #10847, #11107, #8582, #8986, #6976, #16960, #13107, #20831, #23224, #14564, #17091 ) ),
 .UNSPECIFIED., .T., .F., .T. ) 
 B_SPLINE_SURFACE_WITH_KNOTS ( ( 4, 3, 4 ),
 ( 4, 2, 2, 2, 2, 2, 2, 2, 2, 2, 2, 2, 2, 2, 4 ),
 ( 0.000000000000000000, 0.5000000000000000000, 1.000000000000000000 ),
 ( 0.000000000000000000, 0.1357259735107005372, 0.1651108541090157700, 0.1944957347073310028, 0.3598804999793158710, 0.3867117631979620773, 0.4135430264166082281, 0.5789277916885930964, 0.6062785021374117456, 0.6336292125862302838, 0.8508620842112317728, 0.8814014469398914198, 0.9119408096685510667, 0.9559704048342755334, 1.000000000000000000 ),
 .UNSPECIFIED. ) 
 GEOMETRIC_REPRESENTATION_ITEM ( )  RATIONAL_B_SPLINE_SURFACE ( (
 ( 1.000000000000000000, 1.000000000000000000, 1.000000000000000000, 1.000000000000000000, 1.000000000000000000, 1.000000000000000000, 1.000000000000000000, 1.000000000000000000, 1.000000000000000000, 1.000000000000000000, 1.000000000000000000, 1.000000000000000000, 1.000000000000000000, 1.000000000000000000, 1.000000000000000000, 1.000000000000000000, 1.000000000000000000, 1.000000000000000000, 1.000000000000000000, 1.000000000000000000, 1.000000000000000000, 1.000000000000000000, 1.000000000000000000, 1.000000000000000000, 1.000000000000000000, 1.000000000000000000, 1.000000000000000000, 1.000000000000000000, 1.000000000000000000, 1.000000000000000000),
 ( 0.3333333333333333703, 0.3333333333333333703, 0.3333333333333333703, 0.3333333333333333703, 0.3333333333333333703, 0.3333333333333333703, 0.3333333333333333703, 0.3333333333333333703, 0.3333333333333333703, 0.3333333333333333703, 0.3333333333333333703, 0.3333333333333333703, 0.3333333333333333703, 0.3333333333333333703, 0.3333333333333333703, 0.3333333333333333703, 0.3333333333333333703, 0.3333333333333333703, 0.3333333333333333703, 0.3333333333333333703, 0.3333333333333333703, 0.3333333333333333703, 0.3333333333333333703, 0.3333333333333333703, 0.3333333333333333703, 0.3333333333333333703, 0.3333333333333333703, 0.3333333333333333703, 0.3333333333333333703, 0.3333333333333333703),
 ( 0.3333333333333333703, 0.3333333333333333703, 0.3333333333333333703, 0.3333333333333333703, 0.3333333333333333703, 0.3333333333333333703, 0.3333333333333333703, 0.3333333333333333703, 0.3333333333333333703, 0.3333333333333333703, 0.3333333333333333703, 0.3333333333333333703, 0.3333333333333333703, 0.3333333333333333703, 0.3333333333333333703, 0.3333333333333333703, 0.3333333333333333703, 0.3333333333333333703, 0.3333333333333333703, 0.3333333333333333703, 0.3333333333333333703, 0.3333333333333333703, 0.3333333333333333703, 0.3333333333333333703, 0.3333333333333333703, 0.3333333333333333703, 0.3333333333333333703, 0.3333333333333333703, 0.3333333333333333703, 0.3333333333333333703),
 ( 1.000000000000000000, 1.000000000000000000, 1.000000000000000000, 1.000000000000000000, 1.000000000000000000, 1.000000000000000000, 1.000000000000000000, 1.000000000000000000, 1.000000000000000000, 1.000000000000000000, 1.000000000000000000, 1.000000000000000000, 1.000000000000000000, 1.000000000000000000, 1.000000000000000000, 1.000000000000000000, 1.000000000000000000, 1.000000000000000000, 1.000000000000000000, 1.000000000000000000, 1.000000000000000000, 1.000000000000000000, 1.000000000000000000, 1.000000000000000000, 1.000000000000000000, 1.000000000000000000, 1.000000000000000000, 1.000000000000000000, 1.000000000000000000, 1.000000000000000000),
 ( 0.3333333333333333703, 0.3333333333333333703, 0.3333333333333333703, 0.3333333333333333703, 0.3333333333333333703, 0.3333333333333333703, 0.3333333333333333703, 0.3333333333333333703, 0.3333333333333333703, 0.3333333333333333703, 0.3333333333333333703, 0.3333333333333333703, 0.3333333333333333703, 0.3333333333333333703, 0.3333333333333333703, 0.3333333333333333703, 0.3333333333333333703, 0.3333333333333333703, 0.3333333333333333703, 0.3333333333333333703, 0.3333333333333333703, 0.3333333333333333703, 0.3333333333333333703, 0.3333333333333333703, 0.3333333333333333703, 0.3333333333333333703, 0.3333333333333333703, 0.3333333333333333703, 0.3333333333333333703, 0.3333333333333333703),
 ( 0.3333333333333333703, 0.3333333333333333703, 0.3333333333333333703, 0.3333333333333333703, 0.3333333333333333703, 0.3333333333333333703, 0.3333333333333333703, 0.3333333333333333703, 0.3333333333333333703, 0.3333333333333333703, 0.3333333333333333703, 0.3333333333333333703, 0.3333333333333333703, 0.3333333333333333703, 0.3333333333333333703, 0.3333333333333333703, 0.3333333333333333703, 0.3333333333333333703, 0.3333333333333333703, 0.3333333333333333703, 0.3333333333333333703, 0.3333333333333333703, 0.3333333333333333703, 0.3333333333333333703, 0.3333333333333333703, 0.3333333333333333703, 0.3333333333333333703, 0.3333333333333333703, 0.3333333333333333703, 0.3333333333333333703),
 ( 1.000000000000000000, 1.000000000000000000, 1.000000000000000000, 1.000000000000000000, 1.000000000000000000, 1.000000000000000000, 1.000000000000000000, 1.000000000000000000, 1.000000000000000000, 1.000000000000000000, 1.000000000000000000, 1.000000000000000000, 1.000000000000000000, 1.000000000000000000, 1.000000000000000000, 1.000000000000000000, 1.000000000000000000, 1.000000000000000000, 1.000000000000000000, 1.000000000000000000, 1.000000000000000000, 1.000000000000000000, 1.000000000000000000, 1.000000000000000000, 1.000000000000000000, 1.000000000000000000, 1.000000000000000000, 1.000000000000000000, 1.000000000000000000, 1.000000000000000000) ) ) 
 REPRESENTATION_ITEM ( '' )  SURFACE ( )  );
#21451=CARTESIAN_POINT ( 'NONE',  ( 4.995406935893312195, -67.35176059882525124, -10.78321810390210445 ) ) ;
#21453=CARTESIAN_POINT ( 'NONE',  ( -109.1264249741456211, -33.12752917268984731, 13.72187187124577434 ) ) ;
#21454=ORIENTED_EDGE ( 'NONE', *, *, #4933, .T. ) ;
#21455=CARTESIAN_POINT ( 'NONE',  ( -208.1127848780265026, 38.89260858015777700, -38.89260858015687461 ) ) ;
#21461=FACE_OUTER_BOUND ( 'NONE', #17390, .T. ) ;
#21464=CARTESIAN_POINT ( 'NONE',  ( -135.8532207217289738, 39.99999999999989342, 30.84685318188660474 ) ) ;
#21467=CARTESIAN_POINT ( 'NONE',  ( -280.0000000000000000, 1.839446121267387017E-14, -20.00000000000001421 ) ) ;
#21471=B_SPLINE_CURVE_WITH_KNOTS ( 'NONE', 3,
 ( #7486, #21733, #15597, #19603, #13353, #17471, #22006, #3776 ),
 .UNSPECIFIED., .F., .F.,
 ( 4, 2, 2, 4 ),
 ( 0.008473926331994447239, 0.01052499632799544851, 0.01257606632399645152, 0.01667820631599845754 ),
 .UNSPECIFIED. ) ;
#21472=CARTESIAN_POINT ( 'NONE',  ( -77.90255099906777048, 8.644468104261289199, 20.04994828523966177 ) ) ;
#21473=CARTESIAN_POINT ( 'NONE',  ( 136.1360204305621266, -24.77266263493151044, 24.77266263493093135 ) ) ;
#21474=CARTESIAN_POINT ( 'NONE',  ( 91.82158438592159655, 12.16597498400091304, -44.40256751092321963 ) ) ;
#21476=CARTESIAN_POINT ( 'NONE',  ( -56.48582580120557850, -39.99999999999970868, -30.84685318188687120 ) ) ;
#21478=CARTESIAN_POINT ( 'NONE',  ( -280.0000000000000000, 19.99999999999996092, -0.000000000000000000 ) ) ;
#21479=CARTESIAN_POINT ( 'NONE',  ( 91.82158438592159655, -22.79471317813468545, -40.00000000000002132 ) ) ;
#21480=CARTESIAN_POINT ( 'NONE',  ( 14.38125909742180752, 17.55144818341448953, 39.01709431150923280 ) ) ;
#21481=CARTESIAN_POINT ( 'NONE',  ( -30.26275506840323004, -41.69427246844627888, -40.00000000000002132 ) ) ;
#21483=CARTESIAN_POINT ( 'NONE',  ( 192.4448373802101173, 39.99999999999998579, 19.99999999996075317 ) ) ;
#21484=CARTESIAN_POINT ( 'NONE',  ( -96.94475454970501005, -20.58449551012127898, 9.001119816584967737 ) ) ;
#21485=CARTESIAN_POINT ( 'NONE',  ( -114.7831050401054682, 22.13388504846499671, -0.1750307869482046752 ) ) ;
#21486=CARTESIAN_POINT ( 'NONE',  ( -192.9588430854689989, 38.51493924976929861, 38.51493924976947625 ) ) ;
#21487=CARTESIAN_POINT ( 'NONE',  ( -91.56559293963834989, 17.32597176626809699, -40.00000000000002132 ) ) ;
#21490=CARTESIAN_POINT ( 'NONE',  ( 23.58679727197035092, -42.79169916605200541, 23.29637218065948545 ) ) ;
#21494=( BOUNDED_SURFACE ( )  B_SPLINE_SURFACE ( 3, 2, ( 
 ( #17214, #25481, #21472 ),
 ( #19345, #7108, #23350 ),
 ( #5127, #13232, #1254 ),
 ( #21355, #3124, #9238 ),
 ( #7230, #23474, #5246 ),
 ( #13350, #9358, #17468 ) ),
 .UNSPECIFIED., .F., .F., .F. ) 
 B_SPLINE_SURFACE_WITH_KNOTS ( ( 4, 2, 4 ),
 ( 3, 3 ),
 ( 0.04143177204337192970, 0.04845749460347205384, 0.05548321716357218492 ),
 ( 0.000000000000000000, 1.000000000000000000 ),
 .UNSPECIFIED. ) 
 GEOMETRIC_REPRESENTATION_ITEM ( )  RATIONAL_B_SPLINE_SURFACE ( (
 ( 1.000000000000000000, 0.9541700779530459808, 1.000000000000000000),
 ( 1.000000000000000000, 0.9520119500059182061, 1.000000000000000000),
 ( 1.000000000000000000, 0.9503149744749778138, 1.000000000000000000),
 ( 1.000000000000000000, 0.9480088402726788432, 1.000000000000000000),
 ( 1.000000000000000000, 0.9474362538696746716, 1.000000000000000000),
 ( 1.000000000000000000, 0.9474350314971542453, 1.000000000000000000) ) ) 
 REPRESENTATION_ITEM ( '' )  SURFACE ( )  );
#21495=CARTESIAN_POINT ( 'NONE',  ( -162.0762913951021176, 1.198031840315997298, 57.76657433523996588 ) ) ;
#21496=CARTESIAN_POINT ( 'NONE',  ( -162.0762913951021176, -40.00000000000005684, 1.694272876828184504 ) ) ;
#21497=CARTESIAN_POINT ( 'NONE',  ( -82.25907871058393539, 19.72177579145719051, -4.317081979949474402 ) ) ;
#21499=CIRCLE ( 'NONE', #10026, 15.00000000000000000 ) ;
#21501=AXIS2_PLACEMENT_3D ( 'NONE', #16650, #16777, #2828 ) ;
#21502=CARTESIAN_POINT ( 'NONE',  ( -24.15343516389538081, 15.53299357102992495, -37.49996374344652139 ) ) ;
#21505=CARTESIAN_POINT ( 'NONE',  ( -213.1075012329537230, 37.98287015391211696, 18.58567234101190735 ) ) ;
#21506=CARTESIAN_POINT ( 'NONE',  ( -192.9588430854689705, -38.51493924976909966, -38.51493924976973915 ) ) ;
#21507=CARTESIAN_POINT ( 'NONE',  ( 163.1118516004056573, 47.56205970284957374, 9.006482792074494981 ) ) ;
#21509=CARTESIAN_POINT ( 'NONE',  ( 0.2972598230770100991, -38.42060263243632079, -38.42060263243699580 ) ) ;
#21510=CARTESIAN_POINT ( 'NONE',  ( 151.7948205124836534, 23.49921654116056047, -33.06932595376338213 ) ) ;
#21511=CARTESIAN_POINT ( 'NONE',  ( -100.7734535825088500, -16.03295912088659492, -40.53558337403696044 ) ) ;
#21512=CARTESIAN_POINT ( 'NONE',  ( 199.9999999999999432, 14.14213562373110911, -14.14213562373072364 ) ) ;
#21513=CARTESIAN_POINT ( 'NONE',  ( -238.4067589809705794, -0.6820004457913680929, 0.6820004457913170226 ) ) ;
#21515=CARTESIAN_POINT ( 'NONE',  ( 4.995406935893290878, -5.232665749138292703E-14, 15.24977328854832592 ) ) ;
#21516=CARTESIAN_POINT ( 'NONE',  ( 130.8568914410475088, -4.207082182990058428, 52.36146031193416661 ) ) ;
#21517=CARTESIAN_POINT ( 'NONE',  ( 130.8568914410475088, 5.949712681206712261, 40.00000000000002132 ) ) ;
#21519=CARTESIAN_POINT ( 'NONE',  ( -198.0356074513804572, 67.44298959253333692, 10.87444709760969452 ) ) ;
#21520=CARTESIAN_POINT ( 'NONE',  ( -100.0753760173618900, -20.72827493166393609, -8.149786832858609387 ) ) ;
#21521=CARTESIAN_POINT ( 'NONE',  ( -53.37769371643637584, -10.11111068828991577, -29.42719939405419893 ) ) ;
#21522=CARTESIAN_POINT ( 'NONE',  ( -3.838270362648686707, -43.19795333834416340, -17.89317813949888603 ) ) ;
#21524=CARTESIAN_POINT ( 'NONE',  ( -129.2303492453802676, -25.82246949215104337, 9.309000511570687308 ) ) ;
#21526=CARTESIAN_POINT ( 'NONE',  ( 23.84827734669550736, -13.76599369847126830, 46.63681169410619276 ) ) ;
#21528=CARTESIAN_POINT ( 'NONE',  ( 90.71511022964570259, 8.335579106121171478, -21.46756116452269580 ) ) ;
#21530=CARTESIAN_POINT ( 'NONE',  ( -87.01512800814687409, 20.72591320789969771, 5.554844834155465705 ) ) ;
#21531=CARTESIAN_POINT ( 'NONE',  ( 91.82158438592156813, 40.00000000000009948, -17.20528682183286051 ) ) ;
#21534=CARTESIAN_POINT ( 'NONE',  ( 21.15737826136114208, 47.57244852138565960, -13.91467835516647789 ) ) ;
#21535=CARTESIAN_POINT ( 'NONE',  ( -198.0356074513804572, -15.37879056873074290, 40.00000000000002132 ) ) ;
#21536=CARTESIAN_POINT ( 'NONE',  ( -129.2920262390587993, 10.46331600574958642, -25.26067940841951298 ) ) ;
#21538=CARTESIAN_POINT ( 'NONE',  ( 163.1118516004056573, 27.26290988616876021, 40.00000000000002132 ) ) ;
#21539=CARTESIAN_POINT ( 'NONE',  ( -105.3755690713226869, 21.75974354311648540, -0.000000000000000000 ) ) ;
#21541=CARTESIAN_POINT ( 'NONE',  ( 130.8568914410475372, -3.326198072800416995E-13, 34.05028731879788495 ) ) ;
#21542=CARTESIAN_POINT ( 'NONE',  ( 0.2972598230770103767, -39.99999999999945288, -54.33493731733979359 ) ) ;
#21543=CARTESIAN_POINT ( 'NONE',  ( 100.8632772039314744, -19.41886981475201068, -8.043559243227951683 ) ) ;
#21544=ORIENTED_EDGE ( 'NONE', *, *, #6629, .T. ) ;
#21546=CARTESIAN_POINT ( 'NONE',  ( 3.468680969975556305, 44.56630890487243590, -24.60338114558966183 ) ) ;
#21547=CARTESIAN_POINT ( 'NONE',  ( -56.48582580120558561, -30.84685318188645908, 40.00000000000002132 ) ) ;
#21549=CARTESIAN_POINT ( 'NONE',  ( -188.9524464571040880, 43.19209889639678579, -23.58788642769180655 ) ) ;
#21551=ORIENTED_EDGE ( 'NONE', *, *, #4274, .F. ) ;
#21553=CARTESIAN_POINT ( 'NONE',  ( -259.2033419157646676, 6.730120644403521979, -6.730120644403498886 ) ) ;
#21554=CARTESIAN_POINT ( 'NONE',  ( 130.1167162091014120, 12.15076864148467628, -29.33455044752955132 ) ) ;
#21559=CARTESIAN_POINT ( 'NONE',  ( 130.8568914410475372, 4.207082182992862407, 4.207082182992856190 ) ) ;
#21561=FACE_OUTER_BOUND ( 'NONE', #18948, .T. ) ;
#21562=CARTESIAN_POINT ( 'NONE',  ( 18.90082769090740200, -14.00978943384292208, 48.20711988125824377 ) ) ;
#21564=CARTESIAN_POINT ( 'NONE',  ( -53.37686176745754096, 13.65870576116527957, -27.95807077219528480 ) ) ;
#21565=CARTESIAN_POINT ( 'NONE',  ( 130.8568914410475088, -39.99999999999992895, -5.949712681207114606 ) ) ;
#21566=CARTESIAN_POINT ( 'NONE',  ( 0.2972598230769956662, 40.00000000000058975, -54.33493731733894094 ) ) ;
#21568=CARTESIAN_POINT ( 'NONE',  ( 192.4448373802100889, 14.14213562375893574, -14.14213562375874922 ) ) ;
#21569=CARTESIAN_POINT ( 'NONE',  ( 136.1360204305621266, 1.473277640373554421E-13, -35.03383547441296741 ) ) ;
#21570=CARTESIAN_POINT ( 'NONE',  ( -280.0000000000000000, 14.14213562373098299, -14.14213562373088706 ) ) ;
#21571=CARTESIAN_POINT ( 'NONE',  ( 141.7948666911895259, 30.38861427224621536, 12.58737617328915448 ) ) ;
#21573=CARTESIAN_POINT ( 'NONE',  ( -100.7734535825088500, 16.03295912088713848, -16.03295912088698927 ) ) ;
#21574=CARTESIAN_POINT ( 'NONE',  ( -100.7734535825088500, -39.99999999999995737, -22.67402823373205578 ) ) ;
#21575=CARTESIAN_POINT ( 'NONE',  ( 130.8568914410475088, -52.36146031193419503, 4.207082182989537955 ) ) ;
#21576=CARTESIAN_POINT ( 'NONE',  ( 170.2234770963711128, -39.20704971665404059, 17.36149277826957160 ) ) ;
#21577=CARTESIAN_POINT ( 'NONE',  ( -121.8281150758381557, -8.694016608770111176, -23.07023398735807262 ) ) ;
#21579=EDGE_CURVE ( 'NONE', #6963, #9873, #450, .T. ) ;
#21581=CARTESIAN_POINT ( 'NONE',  ( 19.06497207195981858, 10.03556273973516078, -66.60410523465806421 ) ) ;
#21583=CARTESIAN_POINT ( 'NONE',  ( 170.0000000000001137, 3.062538285712881336, 24.95097643317000191 ) ) ;
#21586=CARTESIAN_POINT ( 'NONE',  ( 91.82158438592158234, -1.633484621919921769E-13, 17.20528682183300262 ) ) ;
#21588=CARTESIAN_POINT ( 'NONE',  ( -70.35386311724839459, 8.707385196241270719, 23.12931224237960848 ) ) ;
#21591=CARTESIAN_POINT ( 'NONE',  ( -91.56559293963836410, -12.25131212657462321, -44.31723036834905827 ) ) ;
#21592=CARTESIAN_POINT ( 'NONE',  ( 4.995406935893292655, 39.99999999999982947, 55.24977328856478209 ) ) ;
#21594=CARTESIAN_POINT ( 'NONE',  ( -86.86493150571118349, -19.77569912839183885, -7.943527260495956810 ) ) ;
#21597=CARTESIAN_POINT ( 'NONE',  ( 136.1360204305621551, -40.00000000000001421, 4.966164525586921563 ) ) ;
#21599=CARTESIAN_POINT ( 'NONE',  ( 146.6084372240433709, 40.00000000000003553, 5.374981219217116468 ) ) ;
#21601=CARTESIAN_POINT ( 'NONE',  ( -7.769366557097388437, -22.72119856428940210, -41.90323276218089887 ) ) ;
#21602=CARTESIAN_POINT ( 'NONE',  ( 146.6084372240433709, 52.76785682606523409, -3.800685668858194255 ) ) ;
#21603=FACE_OUTER_BOUND ( 'NONE', #252, .T. ) ;
#21604=CARTESIAN_POINT ( 'NONE',  ( 19.06497207195982924, -39.99999999999945288, -54.19242893257885640 ) ) ;
#21605=CARTESIAN_POINT ( 'NONE',  ( 169.9999999999999432, -24.25569233607180308, 6.285860131565189413 ) ) ;
#21606=CARTESIAN_POINT ( 'NONE',  ( -162.0762913951021176, -1.694272876828353702, 40.00000000000002132 ) ) ;
#21607=CARTESIAN_POINT ( 'NONE',  ( -259.2033419157646676, -30.48217210827743884, -40.00000000000002132 ) ) ;
#21608=CARTESIAN_POINT ( 'NONE',  ( -162.0762913951020892, -1.198031840385783919, 1.198031840385741731 ) ) ;
#21609=CARTESIAN_POINT ( 'NONE',  ( -280.0000000000000568, 19.99999999999996092, -40.00000000000002132 ) ) ;
#21610=CARTESIAN_POINT ( 'NONE',  ( 0.4311942631276012294, -44.08816696360405274, -24.25071831022401625 ) ) ;
#21612=CARTESIAN_POINT ( 'NONE',  ( -238.4067589809705794, -3.369206980223063916E-14, -0.9644942799825824142 ) ) ;
#21613=CARTESIAN_POINT ( 'NONE',  ( -238.4067589809705794, 57.25054294077225592, 0.6820004458485544596 ) ) ;
#21614=CARTESIAN_POINT ( 'NONE',  ( -280.0000000000000000, 19.99999999999996092, 2.449293598294708485E-15 ) ) ;
#21617=CARTESIAN_POINT ( 'NONE',  ( 36.66494225461514844, -39.17447069114134450, 16.22659705900260718 ) ) ;
#21619=CARTESIAN_POINT ( 'NONE',  ( 14.38125909742181108, 39.01709431150907648, 39.01709431150921858 ) ) ;
#21620=CARTESIAN_POINT ( 'NONE',  ( -198.0356074513804572, -9.007331120208026888E-14, 15.37879056873070560 ) ) ;
#21621=CARTESIAN_POINT ( 'NONE',  ( -87.12536333654861664, 21.43930114797831621, 1.600202314776014489 ) ) ;
#21622=DIRECTION ( 'NONE',  ( 5.551115123125783491E-15, 0.3995982397861026492, 0.9166903767138872006 ) ) ;
#21624=CARTESIAN_POINT ( 'NONE',  ( -87.04313178894965120, -4.721723262651171815, -20.90674919797856646 ) ) ;
#21625=CARTESIAN_POINT ( 'NONE',  ( -135.8532207217289738, 21.81201906317729566, 34.75652343174635917 ) ) ;
#21626=CARTESIAN_POINT ( 'NONE',  ( -238.4067589809705794, -0.6820004457337348613, -57.25054294065803617 ) ) ;
#21627=EDGE_CURVE ( 'NONE', #14909, #25810, #10868, .T. ) ;
#21628=CARTESIAN_POINT ( 'NONE',  ( -110.1016741620976518, 20.19284057200533056, -0.4456461246811765919 ) ) ;
#21629=CARTESIAN_POINT ( 'NONE',  ( -86.86493150571115507, 7.943527260496353826, 19.77569912839162569 ) ) ;
#21630=CARTESIAN_POINT ( 'NONE',  ( 200.0000000000000000, 42.42640687119310172, -14.14213562373052646 ) ) ;
#21631=CARTESIAN_POINT ( 'NONE',  ( 4.995406935893287326, 17.50105314357225694, -39.06748935135176026 ) ) ;
#21632=CARTESIAN_POINT ( 'NONE',  ( 146.6084372240433709, -24.48358557860284179, -32.08495691632087699 ) ) ;
#21633=CARTESIAN_POINT ( 'NONE',  ( -162.0762913951020892, 29.48230308784799902, -29.48230308784730980 ) ) ;
#21635=CARTESIAN_POINT ( 'NONE',  ( 4.995406935893288214, 15.24977328854832770, 0.000000000000000000 ) ) ;
#21638=CARTESIAN_POINT ( 'NONE',  ( -162.0762913951021176, -40.00000000000005684, 1.694272876828184504 ) ) ;
#21639=B_SPLINE_CURVE_WITH_KNOTS ( 'NONE', 3,
 ( #5281, #1289, #7521, #11511, #25644, #15385, #26040, #26175 ),
 .UNSPECIFIED., .F., .F.,
 ( 4, 2, 2, 4 ),
 ( 0.008396560128413051854, 0.01250087472273852390, 0.01455303201990126340, 0.01660518931706400289 ),
 .UNSPECIFIED. ) ;
#21640=CARTESIAN_POINT ( 'NONE',  ( 4.995406935893293543, -10.78321810388990265, -10.78321810389009272 ) ) ;
#21641=CARTESIAN_POINT ( 'NONE',  ( -56.48582580120559982, -9.153146818113595984, 40.00000000000002132 ) ) ;
#21643=CARTESIAN_POINT ( 'NONE',  ( -86.96347745069644475, 41.18208027870598187, -15.38646221621779731 ) ) ;
#21644=( BOUNDED_SURFACE ( )  B_SPLINE_SURFACE ( 3, 3, ( 
 ( #10172, #3933, #10036, #16553, #6438, #20554, #18145, #16684, #14290, #5916, #24681, #8297, #467, #6178, #16285, #2456, #22426, #2199, #18681, #6306, #14555, #4201, #14423, #22555, #20422, #10566, #24283, #22685, #4334, #2323 ),
 ( #16423, #12030, #12554, #8570, #14024, #10432, #14157, #10308, #20686, #20150, #22152, #26293, #24413, #22289, #18549, #8032, #18414, #1931, #8171, #16152, #18277, #6052, #330, #62, #4063, #4461, #8433, #12166, #20287, #2066 ),
 ( #189, #3115, #9228, #865, #14686, #10976, #8974, #22819, #16949, #2734, #2596, #24815, #22949, #6835, #10839, #10710, #21085, #18955, #16817, #19334, #4595, #736, #6567, #17083, #24957, #14816, #14954, #8842, #23089, #21344 ),
 ( #599, #18819, #12835, #21218, #12693, #13225, #20822, #15215, #6703, #7102, #25084, #8706, #19086, #25217, #17207, #4860, #6966, #15082, #12965, #11220, #4728, #9099, #23215, #4994, #20955, #23342, #1120, #13100, #2869, #2992 ),
 ( #11097, #19212, #995, #25345, #5118, #21809, #9834, #25951, #18073, #3582, #3857, #6110, #19941, #2124, #21945, #25816, #9967, #3721, #11685, #22347, #12094, #7693, #19811, #26224, #8095, #1993, #17939, #16078, #14087, #23800 ),
 ( #20085, #7562, #26085, #11823, #1597, #17674, #15805, #7820, #1726, #9698, #13949, #15936, #17805, #12225, #15675, #24069, #5581, #1864, #23930, #5705, #5845, #22084, #11960, #14218, #13688, #5979, #22218, #13811, #20215, #3994 ),
 ( #24206, #10099, #7960, #18201, #16215, #24346, #20347, #22354, #4131, #10232, #22742, #8362, #4524, #20883, #4792, #18610, #20750, #10636, #2519, #8766, #12484, #16880, #23017, #16611, #123, #6241, #12757, #14482, #8228, #14354 ) ),
 .UNSPECIFIED., .T., .F., .F. ) 
 B_SPLINE_SURFACE_WITH_KNOTS ( ( 4, 3, 4 ),
 ( 4, 2, 2, 2, 2, 2, 2, 2, 2, 2, 2, 2, 2, 2, 4 ),
 ( 0.000000000000000000, 0.5000000000000000000, 1.000000000000000000 ),
 ( 0.000000000000000000, 0.1357259735107005372, 0.1651108541090157700, 0.1944957347073310028, 0.3598804999793158710, 0.3867117631979620773, 0.4135430264166082281, 0.5789277916885930964, 0.6062785021374117456, 0.6336292125862302838, 0.8508620842112317728, 0.8814014469398914198, 0.9119408096685510667, 0.9559704048342755334, 1.000000000000000000 ),
 .UNSPECIFIED. ) 
 GEOMETRIC_REPRESENTATION_ITEM ( )  RATIONAL_B_SPLINE_SURFACE ( (
 ( 1.000000000000000000, 1.000000000000000000, 1.000000000000000000, 1.000000000000000000, 1.000000000000000000, 1.000000000000000000, 1.000000000000000000, 1.000000000000000000, 1.000000000000000000, 1.000000000000000000, 1.000000000000000000, 1.000000000000000000, 1.000000000000000000, 1.000000000000000000, 1.000000000000000000, 1.000000000000000000, 1.000000000000000000, 1.000000000000000000, 1.000000000000000000, 1.000000000000000000, 1.000000000000000000, 1.000000000000000000, 1.000000000000000000, 1.000000000000000000, 1.000000000000000000, 1.000000000000000000, 1.000000000000000000, 1.000000000000000000, 1.000000000000000000, 1.000000000000000000),
 ( 0.3333333333333333703, 0.3333333333333333703, 0.3333333333333333703, 0.3333333333333333703, 0.3333333333333333703, 0.3333333333333333703, 0.3333333333333333703, 0.3333333333333333703, 0.3333333333333333703, 0.3333333333333333703, 0.3333333333333333703, 0.3333333333333333703, 0.3333333333333333703, 0.3333333333333333703, 0.3333333333333333703, 0.3333333333333333703, 0.3333333333333333703, 0.3333333333333333703, 0.3333333333333333703, 0.3333333333333333703, 0.3333333333333333703, 0.3333333333333333703, 0.3333333333333333703, 0.3333333333333333703, 0.3333333333333333703, 0.3333333333333333703, 0.3333333333333333703, 0.3333333333333333703, 0.3333333333333333703, 0.3333333333333333703),
 ( 0.3333333333333333703, 0.3333333333333333703, 0.3333333333333333703, 0.3333333333333333703, 0.3333333333333333703, 0.3333333333333333703, 0.3333333333333333703, 0.3333333333333333703, 0.3333333333333333703, 0.3333333333333333703, 0.3333333333333333703, 0.3333333333333333703, 0.3333333333333333703, 0.3333333333333333703, 0.3333333333333333703, 0.3333333333333333703, 0.3333333333333333703, 0.3333333333333333703, 0.3333333333333333703, 0.3333333333333333703, 0.3333333333333333703, 0.3333333333333333703, 0.3333333333333333703, 0.3333333333333333703, 0.3333333333333333703, 0.3333333333333333703, 0.3333333333333333703, 0.3333333333333333703, 0.3333333333333333703, 0.3333333333333333703),
 ( 1.000000000000000000, 1.000000000000000000, 1.000000000000000000, 1.000000000000000000, 1.000000000000000000, 1.000000000000000000, 1.000000000000000000, 1.000000000000000000, 1.000000000000000000, 1.000000000000000000, 1.000000000000000000, 1.000000000000000000, 1.000000000000000000, 1.000000000000000000, 1.000000000000000000, 1.000000000000000000, 1.000000000000000000, 1.000000000000000000, 1.000000000000000000, 1.000000000000000000, 1.000000000000000000, 1.000000000000000000, 1.000000000000000000, 1.000000000000000000, 1.000000000000000000, 1.000000000000000000, 1.000000000000000000, 1.000000000000000000, 1.000000000000000000, 1.000000000000000000),
 ( 0.3333333333333333703, 0.3333333333333333703, 0.3333333333333333703, 0.3333333333333333703, 0.3333333333333333703, 0.3333333333333333703, 0.3333333333333333703, 0.3333333333333333703, 0.3333333333333333703, 0.3333333333333333703, 0.3333333333333333703, 0.3333333333333333703, 0.3333333333333333703, 0.3333333333333333703, 0.3333333333333333703, 0.3333333333333333703, 0.3333333333333333703, 0.3333333333333333703, 0.3333333333333333703, 0.3333333333333333703, 0.3333333333333333703, 0.3333333333333333703, 0.3333333333333333703, 0.3333333333333333703, 0.3333333333333333703, 0.3333333333333333703, 0.3333333333333333703, 0.3333333333333333703, 0.3333333333333333703, 0.3333333333333333703),
 ( 0.3333333333333333703, 0.3333333333333333703, 0.3333333333333333703, 0.3333333333333333703, 0.3333333333333333703, 0.3333333333333333703, 0.3333333333333333703, 0.3333333333333333703, 0.3333333333333333703, 0.3333333333333333703, 0.3333333333333333703, 0.3333333333333333703, 0.3333333333333333703, 0.3333333333333333703, 0.3333333333333333703, 0.3333333333333333703, 0.3333333333333333703, 0.3333333333333333703, 0.3333333333333333703, 0.3333333333333333703, 0.3333333333333333703, 0.3333333333333333703, 0.3333333333333333703, 0.3333333333333333703, 0.3333333333333333703, 0.3333333333333333703, 0.3333333333333333703, 0.3333333333333333703, 0.3333333333333333703, 0.3333333333333333703),
 ( 1.000000000000000000, 1.000000000000000000, 1.000000000000000000, 1.000000000000000000, 1.000000000000000000, 1.000000000000000000, 1.000000000000000000, 1.000000000000000000, 1.000000000000000000, 1.000000000000000000, 1.000000000000000000, 1.000000000000000000, 1.000000000000000000, 1.000000000000000000, 1.000000000000000000, 1.000000000000000000, 1.000000000000000000, 1.000000000000000000, 1.000000000000000000, 1.000000000000000000, 1.000000000000000000, 1.000000000000000000, 1.000000000000000000, 1.000000000000000000, 1.000000000000000000, 1.000000000000000000, 1.000000000000000000, 1.000000000000000000, 1.000000000000000000, 1.000000000000000000) ) ) 
 REPRESENTATION_ITEM ( '' )  SURFACE ( )  );
#21645=CARTESIAN_POINT ( 'NONE',  ( -8.311322960495319379, 41.20580916678637351, 17.06800500544055765 ) ) ;
#21646=CARTESIAN_POINT ( 'NONE',  ( 23.58679727196754428, 13.78527791281921644, 46.73132340480187707 ) ) ;
#21647=CARTESIAN_POINT ( 'NONE',  ( -77.90255099906875103, -20.29001641120621002, -8.064892378658361949 ) ) ;
#21648=ORIENTED_EDGE ( 'NONE', *, *, #1426, .T. ) ;
#21649=CARTESIAN_POINT ( 'NONE',  ( -188.3610564113219823, -47.01267209787972234, 13.83140491817315976 ) ) ;
#21651=CARTESIAN_POINT ( 'NONE',  ( 25.88393124174215743, -22.82896322165249359, 42.08451360837295852 ) ) ;
#21652=AXIS2_PLACEMENT_3D ( 'NONE', #13744, #21870, #9369 ) ;
#21653=CARTESIAN_POINT ( 'NONE',  ( -111.5098000082168710, 19.36828941575083363, 8.022608155968326216 ) ) ;
#21656=CARTESIAN_POINT ( 'NONE',  ( 170.2234770963711128, 40.00000000000000000, 15.44714144992830462 ) ) ;
#21657=CARTESIAN_POINT ( 'NONE',  ( -86.86493150571119770, -7.943527260496137110, 19.77569912839176425 ) ) ;
#21658=EDGE_CURVE ( 'NONE', #1858, #12216, #4754, .T. ) ;
#21659=CARTESIAN_POINT ( 'NONE',  ( -199.9999999999999432, -14.52307781036537193, -48.92947633520097384 ) ) ;
#21660=CARTESIAN_POINT ( 'NONE',  ( 4.995406935893294431, -15.24977328854832415, 40.00000000000002132 ) ) ;
#21661=CARTESIAN_POINT ( 'NONE',  ( -144.0562696874938524, 10.50947022281075860, -31.27040355056193022 ) ) ;
#21664=CARTESIAN_POINT ( 'NONE',  ( -105.3755690713226585, 21.75974354311648185, 40.00000000000002132 ) ) ;
#21665=CARTESIAN_POINT ( 'NONE',  ( -135.8532207217289738, 9.153146818113548022, -40.00000000000002132 ) ) ;
#21666=CARTESIAN_POINT ( 'NONE',  ( 184.8905102610680444, -20.92133201514440799, 0.000000000000000000 ) ) ;
#21667=CARTESIAN_POINT ( 'NONE',  ( -208.1127848780264742, 40.00000000000014211, -15.00245453012627728 ) ) ;
#21669=CARTESIAN_POINT ( 'NONE',  ( 137.0932223649025161, -30.33046076074802855, -12.56328820012686798 ) ) ;
#21671=EDGE_CURVE ( 'NONE', #12165, #12221, #7285, .T. ) ;
#21674=CARTESIAN_POINT ( 'NONE',  ( 6.762329110785001873, 44.82519229649617643, -18.56720258520260813 ) ) ;
#21675=CARTESIAN_POINT ( 'NONE',  ( 91.82158438592159655, -22.79471317813468900, 40.00000000000002132 ) ) ;
#21677=CARTESIAN_POINT ( 'NONE',  ( -163.5815475687391825, -38.33196416462971712, 12.03526863292968230 ) ) ;
#21678=CARTESIAN_POINT ( 'NONE',  ( -88.37877758185140920, -8.575405935195258067, 19.92653024451507093 ) ) ;
#21679=EDGE_LOOP ( 'NONE', ( #14515, #16776, #24843, #8395 ) ) ;
#21681=CARTESIAN_POINT ( 'NONE',  ( 155.1206158682454657, 11.51471166709257865, -27.79897307351022917 ) ) ;
#21683=CARTESIAN_POINT ( 'NONE',  ( -102.4068193528164841, 8.088405365068929598, -20.44188272012819496 ) ) ;
#21686=CARTESIAN_POINT ( 'NONE',  ( -196.0240758340695777, 14.12332442061101467, 48.96019759410229000 ) ) ;
#21687=CARTESIAN_POINT ( 'NONE',  ( 192.4448373802101173, -14.14213562375886291, 42.42640687116498555 ) ) ;
#21689=CARTESIAN_POINT ( 'NONE',  ( -213.1075012329537230, -8.703598725189323045E-14, 13.71589010951911902 ) ) ;
#21690=CARTESIAN_POINT ( 'NONE',  ( -4.039451493210485467, -13.82811171175474207, 46.99046209229799587 ) ) ;
#21692=CARTESIAN_POINT ( 'NONE',  ( -28.75704569508430808, 18.59466133783093866, -35.61514925947727050 ) ) ;
#21693=CARTESIAN_POINT ( 'NONE',  ( -192.9588430854689989, 1.161019517985663313E-13, -14.46834944099969533 ) ) ;
#21694=CARTESIAN_POINT ( 'NONE',  ( -91.56559293963834989, 1.671088883502053755E-13, -17.32597176626811120 ) ) ;
#21695=CARTESIAN_POINT ( 'NONE',  ( -199.9999999999999716, -46.88040655664269707, -17.27712336974166618 ) ) ;
#21696=CARTESIAN_POINT ( 'NONE',  ( 184.8905102610680444, 14.79361573936396113, -14.79361573936377461 ) ) ;
#21697=CARTESIAN_POINT ( 'NONE',  ( -199.9999999999999432, 15.63350978565376082, -47.95319408140855444 ) ) ;
#21698=CARTESIAN_POINT ( 'NONE',  ( -195.1686598214383537, 14.09692385498526690, 48.78512304065124994 ) ) ;
#21700=CARTESIAN_POINT ( 'NONE',  ( -77.79405973474324298, 19.55084590669568456, -9.945757298482792663 ) ) ;
#21701=CARTESIAN_POINT ( 'NONE',  ( 199.9999999999999432, 14.14213562373113398, -14.14213562373094923 ) ) ;
#21702=CARTESIAN_POINT ( 'NONE',  ( -208.1127848780265026, -9.061048840815752106E-14, 15.00245453012669472 ) ) ;
#21703=CARTESIAN_POINT ( 'NONE',  ( -208.1127848780264742, 10.60833733270764867, 67.17687982763166588 ) ) ;
#21704=CARTESIAN_POINT ( 'NONE',  ( 136.1360204305621266, -3.511608612530630058, -3.511608612530719764 ) ) ;
#21706=CARTESIAN_POINT ( 'NONE',  ( 21.16156876808018339, 23.80729322913559898, 43.48822901267189422 ) ) ;
#21708=CARTESIAN_POINT ( 'NONE',  ( -213.1075012329537230, 37.98287015391280619, -37.98287015391192512 ) ) ;
#21709=LINE ( 'NONE', #3487, #13684 ) ;
#21711=EDGE_LOOP ( 'NONE', ( #8934, #9346, #8704, #19133 ) ) ;
#21713=CARTESIAN_POINT ( 'NONE',  ( -162.0762913951020892, -1.202636532414034422E-14, -1.694272876828323948 ) ) ;
#21715=CARTESIAN_POINT ( 'NONE',  ( -39.84211263215726007, 13.56589830558360532, 32.75097567529046927 ) ) ;
#21717=AXIS2_PLACEMENT_3D ( 'NONE', #25325, #12817, #5101 ) ;
#21718=ORIENTED_EDGE ( 'NONE', *, *, #10945, .T. ) ;
#21719=ORIENTED_EDGE ( 'NONE', *, *, #21579, .T. ) ;
#21720=CIRCLE ( 'NONE', #12366, 14.99999999999999467 ) ;
#21721=CARTESIAN_POINT ( 'NONE',  ( 91.82158438592158234, 22.79471317813472453, -40.00000000000002132 ) ) ;
#21722=CARTESIAN_POINT ( 'NONE',  ( 130.8568914410475372, 24.07718906447243867, -24.07718906447216156 ) ) ;
#21723=CARTESIAN_POINT ( 'NONE',  ( 192.4448373802101173, 39.99999999999998579, 19.99999999996075317 ) ) ;
#21724=CARTESIAN_POINT ( 'NONE',  ( -114.7539998840383504, -17.50311857019343620, -13.57334797814988470 ) ) ;
#21726=CARTESIAN_POINT ( 'NONE',  ( -109.1264249741489323, 33.12752917269099839, -13.72187187124618646 ) ) ;
#21727=CARTESIAN_POINT ( 'NONE',  ( 57.59792236341147742, -1.230234673553095937E-13, 37.56421063658186199 ) ) ;
#21729=CARTESIAN_POINT ( 'NONE',  ( -192.9588430854689989, -8.596193650988133061E-14, 14.46834944099969533 ) ) ;
#21731=CARTESIAN_POINT ( 'NONE',  ( -77.90255099906774205, -8.644468104261530783, -20.04994828523958006 ) ) ;
#21732=CARTESIAN_POINT ( 'NONE',  ( -259.2033419157646676, 6.730120644403918995, -49.83842185052024831 ) ) ;
#21733=CARTESIAN_POINT ( 'NONE',  ( -105.2054292635175727, -21.49321519473986442, 0.6800022380102618280 ) ) ;
#21734=CARTESIAN_POINT ( 'NONE',  ( 151.7948205124836534, -40.00000000000034817, 33.23291073765511072 ) ) ;
#21736=CARTESIAN_POINT ( 'NONE',  ( -91.56559293963836410, 22.67402823373190301, 40.00000000000002132 ) ) ;
#21737=CARTESIAN_POINT ( 'NONE',  ( 184.8905102610680444, 20.92133201514447194, -40.00000000000002132 ) ) ;
#21738=CARTESIAN_POINT ( 'NONE',  ( 19.06497207195981147, -10.03556273973439517, 10.03556273973429214 ) ) ;
#21739=CARTESIAN_POINT ( 'NONE',  ( -259.2033419157646676, -30.48217210827743884, -40.00000000000002132 ) ) ;
#21740=CARTESIAN_POINT ( 'NONE',  ( 4.990269915386285504, -44.75621547178040771, -24.74342916192413355 ) ) ;
#21741=EDGE_CURVE ( 'NONE', #19209, #8230, #16195, .T. ) ;
#21742=CARTESIAN_POINT ( 'NONE',  ( -280.0000000000000568, 39.99999999999976552, 20.00000000000043343 ) ) ;
#21743=CARTESIAN_POINT ( 'NONE',  ( 19.06497207195980792, 66.60410523465817789, 10.03556273973446800 ) ) ;
#21744=CARTESIAN_POINT ( 'NONE',  ( 151.7948205124836534, 6.767089262349062828, -40.00000000000002132 ) ) ;
#21746=CARTESIAN_POINT ( 'NONE',  ( 23.37583784646189500, -42.85659535397651609, 23.33923448557682789 ) ) ;
#21749=CARTESIAN_POINT ( 'NONE',  ( -105.3755690713226585, 41.18208027870598187, -15.38646221621779731 ) ) ;
#21750=CARTESIAN_POINT ( 'NONE',  ( 4.995406935893298872, -1.944352046434030652E-13, 55.24977328854835434 ) ) ;
#21751=CARTESIAN_POINT ( 'NONE',  ( 184.8905102610680444, 13.49065550809757497, 43.07788698682593065 ) ) ;
#21752=CARTESIAN_POINT ( 'NONE',  ( 163.1118516004056573, 12.73709011382478806, -40.00000000000002132 ) ) ;
#21756=CARTESIAN_POINT ( 'NONE',  ( -82.28162732594363149, 6.256644183661008718, -19.22463888481380323 ) ) ;
#21757=CARTESIAN_POINT ( 'NONE',  ( 57.59792236341147031, 26.56190807104652052, 30.00663442387728708 ) ) ;
#21758=CARTESIAN_POINT ( 'NONE',  ( 146.6084372240433709, 52.76785682606523409, -3.800685668858194255 ) ) ;
#21760=FACE_OUTER_BOUND ( 'NONE', #21177, .T. ) ;
#21761=CARTESIAN_POINT ( 'NONE',  ( 14.38125909742180752, 17.55144818341503665, -39.01709431150898411 ) ) ;
#21763=CARTESIAN_POINT ( 'NONE',  ( 146.6084372240433709, 24.48358557860356655, -32.08495691632035118 ) ) ;
#21764=CARTESIAN_POINT ( 'NONE',  ( -135.8532207217289738, -6.472252184283586729, -50.09629031063973770 ) ) ;
#21765=CARTESIAN_POINT ( 'NONE',  ( 57.59792236341147031, -1.722363176415055985, 1.722363176415024677 ) ) ;
#21767=CARTESIAN_POINT ( 'NONE',  ( 192.4448373802100889, -14.14213562375876698, -14.14213562375885047 ) ) ;
#21769=CARTESIAN_POINT ( 'NONE',  ( -238.4067589809705794, -40.00000000000007105, 0.9644942799824426372 ) ) ;
#21770=CARTESIAN_POINT ( 'NONE',  ( 136.1360204305621266, -3.511608612530682905, 3.511608612530666917 ) ) ;
#21771=CARTESIAN_POINT ( 'NONE',  ( -198.0356074513804572, -10.87444709759714634, -10.87444709759729911 ) ) ;
#21772=CARTESIAN_POINT ( 'NONE',  ( 0.2972598230769930017, 14.33493731733933352, 40.00000000000002132 ) ) ;
#21774=CARTESIAN_POINT ( 'NONE',  ( -198.0356074513804572, 10.87444709759714989, 10.87444709759722450 ) ) ;
#21775=CARTESIAN_POINT ( 'NONE',  ( 1.066297917906484427, 43.20144851603839697, 17.89462588950527788 ) ) ;
#21777=CARTESIAN_POINT ( 'NONE',  ( 98.29820294267436509, 14.14213562374297695, -14.14213562372651189 ) ) ;
#21779=CARTESIAN_POINT ( 'NONE',  ( -188.3610564113329247, -43.02325945309097932, 23.46269903113408262 ) ) ;
#21781=CARTESIAN_POINT ( 'NONE',  ( 67.90397382967701390, -10.29861769470937638, 30.27708616521051255 ) ) ;
#21782=CARTESIAN_POINT ( 'NONE',  ( 22.50777602749652218, 17.91321921095766712, -43.24633676485946410 ) ) ;
#21785=DIRECTION ( 'NONE',  ( 0.000000000000000000, 1.000000000000000000, 0.000000000000000000 ) ) ;
#21786=CARTESIAN_POINT ( 'NONE',  ( -100.7734535825088500, 40.00000000000008527, -22.67402823373177512 ) ) ;
#21787=CARTESIAN_POINT ( 'NONE',  ( -77.55640685868800688, -1.385213842686960017, 22.13135000840288313 ) ) ;
#21789=CARTESIAN_POINT ( 'NONE',  ( 136.1360204305621551, -4.966164525587043244, 40.00000000000002132 ) ) ;
#21790=CARTESIAN_POINT ( 'NONE',  ( -185.5190930961335027, 17.55874694104972988, -42.39056500340850420 ) ) ;
#21792=CARTESIAN_POINT ( 'NONE',  ( 98.29820294267396719, -17.94316440882807129, -8.858778887858122175 ) ) ;
#21793=CARTESIAN_POINT ( 'NONE',  ( 0.2972598230769983307, -14.33493731733933352, 0.000000000000000000 ) ) ;
#21794=CARTESIAN_POINT ( 'NONE',  ( 91.82158438592158234, -17.20528682183298486, 40.00000000000002132 ) ) ;
#21795=CARTESIAN_POINT ( 'NONE',  ( 14.38125909742182529, -39.99999999999944578, -55.17850393971050238 ) ) ;
#21796=CARTESIAN_POINT ( 'NONE',  ( 91.82158438592158234, -1.633484621919921769E-13, 17.20528682183300262 ) ) ;
#21797=CARTESIAN_POINT ( 'NONE',  ( 151.7948205124836250, 23.49921654116328540, 23.49921654116366554 ) ) ;
#21798=ORIENTED_EDGE ( 'NONE', *, *, #1588, .F. ) ;
#21799=CARTESIAN_POINT ( 'NONE',  ( -109.1264249741451948, 33.12752917270486819, -13.72187187121119401 ) ) ;
#21800=CARTESIAN_POINT ( 'NONE',  ( -56.48582580120559271, 9.153146818113576444, -0.000000000000000000 ) ) ;
#21802=CARTESIAN_POINT ( 'NONE',  ( -86.86578273022546171, -8.153770686795279943, 19.68494377654078420 ) ) ;
#21804=ORIENTED_EDGE ( 'NONE', *, *, #1849, .T. ) ;
#21805=ORIENTED_EDGE ( 'NONE', *, *, #1775, .T. ) ;
#21806=CARTESIAN_POINT ( 'NONE',  ( -105.4741150117382915, -19.60045294982753461, 8.366608964593266862 ) ) ;
#21807=CARTESIAN_POINT ( 'NONE',  ( 23.72853009152644788, -46.68009952139126995, -13.77482773664812221 ) ) ;
#21809=CARTESIAN_POINT ( 'NONE',  ( -198.0356074513804572, 55.37879056874818673, -40.00000000000002132 ) ) ;
#21810=CARTESIAN_POINT ( 'NONE',  ( -94.58360650939697223, -20.91945674498037278, 8.190527749779679567 ) ) ;
#21812=ORIENTED_EDGE ( 'NONE', *, *, #15991, .T. ) ;
#21815=CARTESIAN_POINT ( 'NONE',  ( -105.3755690713226585, 41.18208027870598187, -15.38646221621779731 ) ) ;
#21817=CARTESIAN_POINT ( 'NONE',  ( -200.0000000000000284, 30.70179486994630835, -44.88127304974036491 ) ) ;
#21818=CARTESIAN_POINT ( 'NONE',  ( 130.8568914410475372, 1.429239637432775288E-13, -34.05028731879788495 ) ) ;
#21821=ADVANCED_FACE ( 'NONE', ( #12229 ), #2259, .T. ) ;
#21824=CARTESIAN_POINT ( 'NONE',  ( 163.1118516004056573, -2.556006622855449647E-13, 27.26290988616872824 ) ) ;
#21825=CARTESIAN_POINT ( 'NONE',  ( -208.1127848780265026, 1.189126717069624012E-13, -15.00245453012669472 ) ) ;
#21826=CARTESIAN_POINT ( 'NONE',  ( -200.0000000000000000, -44.98788141756672587, -22.84381638316556717 ) ) ;
#21827=CARTESIAN_POINT ( 'NONE',  ( -198.0356074513804572, -39.15871834505905724, -17.40982414986491733 ) ) ;
#21828=CARTESIAN_POINT ( 'NONE',  ( -238.4067589809705794, -0.9644942799826263791, -40.00000000000002132 ) ) ;
#21829=CARTESIAN_POINT ( 'NONE',  ( 200.0000000000000000, -42.42640687119269671, -14.14213562373124766 ) ) ;
#21830=CARTESIAN_POINT ( 'NONE',  ( -83.21262154144251610, 13.72187187061548741, -33.12752917118393015 ) ) ;
#21832=CARTESIAN_POINT ( 'NONE',  ( 98.29820294268191105, -7.653668647302825256, -18.47759065022797031 ) ) ;
#21833=CARTESIAN_POINT ( 'NONE',  ( -86.96347745069645896, 39.99999999999977973, 21.75974354311691883 ) ) ;
#21834=CARTESIAN_POINT ( 'NONE',  ( -213.1075012329537230, -40.00000000000025580, 53.71589010953650956 ) ) ;
#21835=CARTESIAN_POINT ( 'NONE',  ( -192.9588430854690273, 10.23066800231970319, 66.79921049724369198 ) ) ;
#21836=CARTESIAN_POINT ( 'NONE',  ( 200.0000000000000000, -14.14213562373122457, 42.42640687119282461 ) ) ;
#21837=CARTESIAN_POINT ( 'NONE',  ( -188.2652746676490096, -13.82569223135675607, -46.97858116094653269 ) ) ;
#21838=CARTESIAN_POINT ( 'NONE',  ( 163.1118516004056573, 19.27778845538780317, -19.27778845538757224 ) ) ;
#21839=VERTEX_POINT ( 'NONE', #8232 ) ;
#21840=CARTESIAN_POINT ( 'NONE',  ( -208.1127848780264742, 10.60833733268383483, -67.17687982760675425 ) ) ;
#21841=CARTESIAN_POINT ( 'NONE',  ( -56.48582580120559271, 9.153146818113576444, -0.000000000000000000 ) ) ;
#21843=CARTESIAN_POINT ( 'NONE',  ( 192.4448373802100889, 14.14213562370330379, -14.14213562370292365 ) ) ;
#21844=CARTESIAN_POINT ( 'NONE',  ( -87.12809909138003661, 1.359879344810606350, 21.45715697400068578 ) ) ;
#21848=CARTESIAN_POINT ( 'NONE',  ( -4.558244102844902557, 13.79151199599537669, 46.81081390833295330 ) ) ;
#21849=ORIENTED_EDGE ( 'NONE', *, *, #4630, .F. ) ;
#21850=ORIENTED_EDGE ( 'NONE', *, *, #17579, .T. ) ;
#21851=CARTESIAN_POINT ( 'NONE',  ( 130.8568914410475088, 5.949712681206719367, -40.00000000000002132 ) ) ;
#21852=CARTESIAN_POINT ( 'NONE',  ( -280.0000000000000000, 14.14213562373098299, -14.14213562373088706 ) ) ;
#21853=CARTESIAN_POINT ( 'NONE',  ( -213.1075012329537230, 39.99999999999979394, 53.71589010950180665 ) ) ;
#21854=CARTESIAN_POINT ( 'NONE',  ( -96.94475454970458372, -20.92018922306581530, -8.190683501986224968 ) ) ;
#21857=CARTESIAN_POINT ( 'NONE',  ( 130.8568914410475088, 39.99999999999969447, 34.05028731879830417 ) ) ;
#21860=CARTESIAN_POINT ( 'NONE',  ( -3.977426076247836839, -17.87762021094878406, -43.16039317622803395 ) ) ;
#21861=CARTESIAN_POINT ( 'NONE',  ( -192.9588430854690273, 18.05360324515473280, -38.51493924976924177 ) ) ;
#21862=CARTESIAN_POINT ( 'NONE',  ( 151.7948205124836250, -23.49921654116371883, 23.49921654116317526 ) ) ;
#21863=CARTESIAN_POINT ( 'NONE',  ( 91.82158438592156813, -16.11829626348402655, -40.45024623143966380 ) ) ;
#21864=CARTESIAN_POINT ( 'NONE',  ( 200.0000000000000000, -40.00000000000019185, 19.99999999999968381 ) ) ;
#21865=CARTESIAN_POINT ( 'NONE',  ( -105.2274517607688011, -21.34875776644186374, -2.715151009218549127 ) ) ;
#21866=CARTESIAN_POINT ( 'NONE',  ( 91.82158438592158234, 17.20528682183301683, 0.000000000000000000 ) ) ;
#21867=CARTESIAN_POINT ( 'NONE',  ( -100.7734535825088358, -17.32597176626813251, -2.449293598294708485E-15 ) ) ;
#21868=CARTESIAN_POINT ( 'NONE',  ( 130.8568914410475372, 24.07718906447243867, -24.07718906447216156 ) ) ;
#21869=CARTESIAN_POINT ( 'NONE',  ( -280.0000000000000568, -20.00000000000006395, -40.00000000000002132 ) ) ;
#21870=DIRECTION ( 'NONE',  ( 0.9698969544411792931, 0.09318942517728809327, 0.2249791741491908026 ) ) ;
#21871=CARTESIAN_POINT ( 'NONE',  ( -114.7484189202600930, 21.94394827837179918, 2.980060266884688946 ) ) ;
#21872=CARTESIAN_POINT ( 'NONE',  ( -86.96347745069644475, 41.18208027870598187, -15.38646221621779731 ) ) ;
#21873=CARTESIAN_POINT ( 'NONE',  ( 136.1360204305621551, 4.966164525587085876, 40.00000000000002132 ) ) ;
#21875=( BOUNDED_CURVE ( )  B_SPLINE_CURVE ( 3, ( #24775, #2823, #12924, #10526 ),
 .UNSPECIFIED., .F., .T. ) 
 B_SPLINE_CURVE_WITH_KNOTS ( ( 4, 4 ),
 ( 0.01388163286937179816, 0.02359082919310010601 ),
 .UNSPECIFIED. ) 
 CURVE ( )  GEOMETRIC_REPRESENTATION_ITEM ( )  RATIONAL_B_SPLINE_CURVE ( ( 1.000000000000000000, 0.8672072324488975248, 0.7608653435686167921, 0.6809743333591576908 ) ) 
 REPRESENTATION_ITEM ( '' )  );
#21877=DIRECTION ( 'NONE',  ( 0.000000000000000000, 1.000000000000000000, 0.000000000000000000 ) ) ;
#21878=CARTESIAN_POINT ( 'NONE',  ( -135.8532207217289738, 21.81201906317777883, -34.75652343174605363 ) ) ;
#21879=CARTESIAN_POINT ( 'NONE',  ( 146.6084372240433709, -40.00000000000001421, 5.374981219216829587 ) ) ;
#21880=AXIS2_PLACEMENT_3D ( 'NONE', #14702, #16963, #22833 ) ;
#21881=CARTESIAN_POINT ( 'NONE',  ( -280.0000000000000000, -14.14213562373118549, 14.14213562373078936 ) ) ;
#21882=CARTESIAN_POINT ( 'NONE',  ( -238.4067589809705794, 0.9644942799825386714, 0.000000000000000000 ) ) ;
#21883=CARTESIAN_POINT ( 'NONE',  ( 136.1360204305621551, 4.966164525587093870, -40.00000000000002132 ) ) ;
#21884=CARTESIAN_POINT ( 'NONE',  ( -188.2995950289364089, -43.00522595870943832, -23.44932284466036521 ) ) ;
#21887=CARTESIAN_POINT ( 'NONE',  ( -238.4067589809705794, 28.96627169325285678, 27.60227080167094726 ) ) ;
#21888=CARTESIAN_POINT ( 'NONE',  ( 91.82158438592159655, 12.16597498400091304, -44.40256751092321963 ) ) ;
#21890=CARTESIAN_POINT ( 'NONE',  ( 4.995406935893293543, -10.78321810389005364, 10.78321810388994173 ) ) ;
#21891=CARTESIAN_POINT ( 'NONE',  ( -77.65695844553741267, 18.42387585929312976, -12.10528775143868252 ) ) ;
#21892=CARTESIAN_POINT ( 'NONE',  ( -198.0356074513804288, -39.15871834505882276, -39.15871834505946936 ) ) ;
#21893=CARTESIAN_POINT ( 'NONE',  ( 0.2972598230770100991, -38.42060263243632079, -38.42060263243699580 ) ) ;
#21894=CARTESIAN_POINT ( 'NONE',  ( 4.995406935893294431, -17.50105314357144337, -39.06748935135212264 ) ) ;
#21895=CARTESIAN_POINT ( 'NONE',  ( 91.82158438592158234, -40.45024623143936537, -16.11829626348475131 ) ) ;
#21896=CARTESIAN_POINT ( 'NONE',  ( 136.1360204305621266, -35.03383547441293899, 0.000000000000000000 ) ) ;
#21899=CARTESIAN_POINT ( 'NONE',  ( 136.1360204305621266, 1.473277640373554421E-13, -35.03383547441296741 ) ) ;
#21900=CARTESIAN_POINT ( 'NONE',  ( -86.96347745069645896, 43.67073346367970288, 12.89780903124427702 ) ) ;
#21902=CARTESIAN_POINT ( 'NONE',  ( 151.7948205124836250, 23.49921654116328540, 23.49921654116366554 ) ) ;
#21904=CARTESIAN_POINT ( 'NONE',  ( 57.59792236341147031, -2.435789363418150000, 40.00000000000002132 ) ) ;
#21907=CARTESIAN_POINT ( 'NONE',  ( -100.7734535825088500, 12.25131212657490209, -44.31723036834897300 ) ) ;
#21908=CARTESIAN_POINT ( 'NONE',  ( -63.45572741887768586, 25.09195535024256785, 10.39342821253069893 ) ) ;
#21910=CARTESIAN_POINT ( 'NONE',  ( -198.0356074513804572, 15.37879056873067007, 0.000000000000000000 ) ) ;
#21911=EDGE_CURVE ( 'NONE', #24911, #10231, #10534, .T. ) ;
#21913=VERTEX_POINT ( 'NONE', #19018 ) ;
#21915=CARTESIAN_POINT ( 'NONE',  ( -3.762763306026911447, 23.50897034858851242, -43.08566851766582317 ) ) ;
#21917=CARTESIAN_POINT ( 'NONE',  ( -4.022465846214220875, -23.45302613997613861, 43.01021959554137908 ) ) ;
#21919=EDGE_CURVE ( 'NONE', #23643, #17137, #3460, .T. ) ;
#21920=CARTESIAN_POINT ( 'NONE',  ( 16.38602454705335276, 24.50452114746028087, -44.43226271088839496 ) ) ;
#21924=CARTESIAN_POINT ( 'NONE',  ( -121.8281150759179212, -8.694016608775745780, 23.07023398738753173 ) ) ;
#21925=CARTESIAN_POINT ( 'NONE',  ( 14.38125909742181108, 39.01709431150961649, -39.01709431150867147 ) ) ;
#21926=CARTESIAN_POINT ( 'NONE',  ( -91.56559293963836410, 22.67402823373190301, 40.00000000000002132 ) ) ;
#21927=CARTESIAN_POINT ( 'NONE',  ( 44.82887508592131098, -18.94256811217822900, -36.15717056695913101 ) ) ;
#21928=CARTESIAN_POINT ( 'NONE',  ( -238.4067589809705794, 0.9644942799825386714, 0.000000000000000000 ) ) ;
#21929=CARTESIAN_POINT ( 'NONE',  ( -162.0762913951020892, 1.198031840385732849, -1.198031840385733515 ) ) ;
#21930=CARTESIAN_POINT ( 'NONE',  ( 151.7948205124836250, 33.23291073765556547, 0.000000000000000000 ) ) ;
#21931=CARTESIAN_POINT ( 'NONE',  ( -208.1127848780265026, 15.00245453012665564, 0.000000000000000000 ) ) ;
#21932=CARTESIAN_POINT ( 'NONE',  ( 146.6084372240433709, -39.99999999999993605, -5.374981219217395356 ) ) ;
#21933=CARTESIAN_POINT ( 'NONE',  ( 98.29820294267355507, -10.02182676110716208, 17.32045324916611406 ) ) ;
#21934=CARTESIAN_POINT ( 'NONE',  ( -135.8532207217289738, 6.472252184284096543, 6.472252184284234211 ) ) ;
#21937=CARTESIAN_POINT ( 'NONE',  ( -100.7734535825088500, 22.67402823373189591, -0.000000000000000000 ) ) ;
#21938=CARTESIAN_POINT ( 'NONE',  ( -102.4309680866254268, -8.087567261749121883, 20.43798635335615899 ) ) ;
#21942=CARTESIAN_POINT ( 'NONE',  ( 19.06497207195981858, -38.31983398719616218, -18.24870850772777331 ) ) ;
#21943=CARTESIAN_POINT ( 'NONE',  ( 44.65795722955357405, -36.73450905827150592, -15.21593185916488622 ) ) ;
#21944=ORIENTED_EDGE ( 'NONE', *, *, #15341, .F. ) ;
#21945=CARTESIAN_POINT ( 'NONE',  ( -30.26275506840324425, 41.69427246844628598, -40.00000000000002132 ) ) ;
#21947=EDGE_LOOP ( 'NONE', ( #5583, #19164, #25710, #16081, #13676, #14647, #11554 ) ) ;
#21950=CARTESIAN_POINT ( 'NONE',  ( 200.0000000000000000, -14.14213562373106114, 42.42640687119278908 ) ) ;
#21951=CARTESIAN_POINT ( 'NONE',  ( -199.9999999999998579, 44.86878812508723513, -24.82633483071237634 ) ) ;
#21954=CARTESIAN_POINT ( 'NONE',  ( -162.0762913951020892, -3.568845385355699554E-14, 1.694272876828323948 ) ) ;
#21955=CARTESIAN_POINT ( 'NONE',  ( 163.1118516004056573, -27.26290988616869626, 0.000000000000000000 ) ) ;
#21958=CARTESIAN_POINT ( 'NONE',  ( -105.3755690713226727, 5.661656051307470077E-14, -21.75974354311649961 ) ) ;
#21959=CARTESIAN_POINT ( 'NONE',  ( -135.8532207217289738, -1.208299557080134822E-13, 9.153146818113572891 ) ) ;
#21960=CARTESIAN_POINT ( 'NONE',  ( 170.0000000000000284, -6.285860131565133457, -24.25569233607183506 ) ) ;
#21961=CARTESIAN_POINT ( 'NONE',  ( 136.1360204305621266, -3.511608612530682905, 3.511608612530666917 ) ) ;
#21962=CARTESIAN_POINT ( 'NONE',  ( 14.38125909742181285, -15.17850393972633505, -40.00000000000002132 ) ) ;
#21963=CARTESIAN_POINT ( 'NONE',  ( -213.1075012329537230, -66.26714140138676612, 9.698598906462487790 ) ) ;
#21966=B_SPLINE_CURVE_WITH_KNOTS ( 'NONE', 3,
 ( #17929, #7421, #25805, #23540, #3447, #13940, #5696, #13801 ),
 .UNSPECIFIED., .F., .F.,
 ( 4, 2, 2, 4 ),
 ( -5.298247996737306503E-05, 0.001923793760064214722, 0.003900570000095802611, 0.007854122480158971450 ),
 .UNSPECIFIED. ) ;
#21967=CARTESIAN_POINT ( 'NONE',  ( -1.818469002956083935, -47.72215409237453088, 13.93708913181261799 ) ) ;
#21968=CARTESIAN_POINT ( 'NONE',  ( 146.6084372240433993, -3.357462877844280890E-13, 34.62501878078305850 ) ) ;
#21969=CARTESIAN_POINT ( 'NONE',  ( 0.2972598230770030492, -40.00000000000007816, 14.33493731733919496 ) ) ;
#21970=CARTESIAN_POINT ( 'NONE',  ( -30.26275506840325136, 57.76657404653985139, 1.198031551616126178 ) ) ;
#21971=CARTESIAN_POINT ( 'NONE',  ( -86.96347745069644475, 15.38646221621772092, 15.38646221621800336 ) ) ;
#21972=CARTESIAN_POINT ( 'NONE',  ( -188.8753834511965692, -17.93496043754474556, -43.29882472894647094 ) ) ;
#21973=CARTESIAN_POINT ( 'NONE',  ( 170.0000000000000000, -2.301191124287261779E-13, 24.95097643317000546 ) ) ;
#21975=CARTESIAN_POINT ( 'NONE',  ( 130.8568914410475088, -24.07718906446864793, -32.49135343045505664 ) ) ;
#21976=CARTESIAN_POINT ( 'NONE',  ( 130.8568914410475372, 24.07718906447243867, -24.07718906447216156 ) ) ;
#21977=CARTESIAN_POINT ( 'NONE',  ( -30.26275506840324070, -1.694272468446265112, 0.000000000000000000 ) ) ;
#21979=CARTESIAN_POINT ( 'NONE',  ( -87.13361725327071383, 16.19487519257939212, 14.20112123283741745 ) ) ;
#21980=CARTESIAN_POINT ( 'NONE',  ( -259.2033419157646676, -6.730120644402966867, -49.83842185052038332 ) ) ;
#21981=B_SPLINE_CURVE_WITH_KNOTS ( 'NONE', 3,
 ( #18026, #1420, #23753, #7643, #23507, #15758 ),
 .UNSPECIFIED., .F., .F.,
 ( 4, 2, 4 ),
 ( 0.0003134551847831237793, 0.004478723513730584541, 0.008643991842678043838 ),
 .UNSPECIFIED. ) ;
#21982=CARTESIAN_POINT ( 'NONE',  ( 23.37394308801977871, -42.85717664514601921, 23.33966569535066071 ) ) ;
#21986=CARTESIAN_POINT ( 'NONE',  ( -105.2502153031278880, -17.39736479739720920, 12.58638139385545607 ) ) ;
#21987=CARTESIAN_POINT ( 'NONE',  ( -3.417371742524983880, 17.93997298316174493, 43.31092608455620763 ) ) ;
#21988=B_SPLINE_CURVE_WITH_KNOTS ( 'NONE', 3,
 ( #24789, #4963, #25056, #21187, #8945, #6543, #12938, #21053 ),
 .UNSPECIFIED., .F., .F.,
 ( 4, 2, 2, 4 ),
 ( 1.822044248639793593E-14, 0.002116768774648846146, 0.004233537549279472491, 0.008467075098540726916 ),
 .UNSPECIFIED. ) ;
#21991=CARTESIAN_POINT ( 'NONE',  ( -105.3755690713226727, -15.38646221621786481, -15.38646221621789856 ) ) ;
#21993=CARTESIAN_POINT ( 'NONE',  ( -208.1127848780264742, 39.99999999999979394, 55.00245453010936103 ) ) ;
#21994=ADVANCED_BREP_SHAPE_REPRESENTATION ( '', ( #8606, #21058 ), #17620 ) ;
#21997=CARTESIAN_POINT ( 'NONE',  ( -86.96347745069644475, -2.438961472018186339E-13, 21.75974354311649961 ) ) ;
#22002=CARTESIAN_POINT ( 'NONE',  ( -83.21262154144251610, -33.12752917118416462, -13.72187187061499536 ) ) ;
#22003=CARTESIAN_POINT ( 'NONE',  ( -3.417371742523256373, -17.93997298316167033, -43.31092608455676185 ) ) ;
#22004=CARTESIAN_POINT ( 'NONE',  ( 91.82158438592159655, -16.11829626346125011, -16.11829626346154853 ) ) ;
#22006=CARTESIAN_POINT ( 'NONE',  ( -105.3841681040961475, -20.33889746609128579, 6.699016078410943820 ) ) ;
#22007=CARTESIAN_POINT ( 'NONE',  ( -135.8532207217289738, -21.81201906317788186, 21.81201906317762962 ) ) ;
#22008=CARTESIAN_POINT ( 'NONE',  ( -86.96347745069643054, -40.00000000000026290, 21.75974354311608749 ) ) ;
#22010=CARTESIAN_POINT ( 'NONE',  ( 192.4448373802100889, 14.14213562375873678, 14.14213562375894817 ) ) ;
#22011=CARTESIAN_POINT ( 'NONE',  ( 192.4448373802100889, -19.99999999996057198, -2.449293598294708485E-15 ) ) ;
#22012=CARTESIAN_POINT ( 'NONE',  ( -100.7734535825088500, 44.31723036834890905, 12.25131212657507795 ) ) ;
#22013=CARTESIAN_POINT ( 'NONE',  ( 163.1118516004056573, -12.73709011382471878, -40.00000000000002132 ) ) ;
#22014=CARTESIAN_POINT ( 'NONE',  ( -105.2599799664448312, 17.55584898455461840, 12.33876530776534786 ) ) ;
#22015=CARTESIAN_POINT ( 'NONE',  ( -208.1127848780265026, 1.189126717069624012E-13, -15.00245453012669472 ) ) ;
#22017=CARTESIAN_POINT ( 'NONE',  ( -213.1075012329537230, 9.698598906450410340, 9.698598906450483170 ) ) ;
#22018=EDGE_CURVE ( 'NONE', #16948, #8230, #24190, .T. ) ;
#22019=CARTESIAN_POINT ( 'NONE',  ( -162.0762913951020892, 1.694272876828294194, 0.000000000000000000 ) ) ;
#22021=CARTESIAN_POINT ( 'NONE',  ( 22.86726691379450926, -43.14849715852140122, 17.87269271907627655 ) ) ;
#22022=FACE_OUTER_BOUND ( 'NONE', #11591, .T. ) ;
#22023=CARTESIAN_POINT ( 'NONE',  ( 146.6084372240433709, 32.08495691632064961, -24.48358557860320417 ) ) ;
#22024=CARTESIAN_POINT ( 'NONE',  ( 170.2234770963711128, -39.99999999999991473, -24.55285855007201334 ) ) ;
#22025=CARTESIAN_POINT ( 'NONE',  ( 163.1118516004056573, -19.27778845538787422, 19.27778845538743724 ) ) ;
#22026=CARTESIAN_POINT ( 'NONE',  ( 163.1118516004056573, -27.26290988616869626, 0.000000000000000000 ) ) ;
#22027=CARTESIAN_POINT ( 'NONE',  ( -100.7734535825088358, -22.67402823373193499, 0.000000000000000000 ) ) ;
#22031=CARTESIAN_POINT ( 'NONE',  ( -213.1075012329537230, 37.98287015391280619, -37.98287015391192512 ) ) ;
#22032=CARTESIAN_POINT ( 'NONE',  ( -56.48582580120558561, -50.09629031063971638, 6.472252184283745713 ) ) ;
#22033=CARTESIAN_POINT ( 'NONE',  ( -188.2995950289364941, -13.82811170417257607, 46.99046209955427855 ) ) ;
#22034=CARTESIAN_POINT ( 'NONE',  ( -82.23729782343656325, 15.18297044031445431, -13.37626936639568598 ) ) ;
#22035=CARTESIAN_POINT ( 'NONE',  ( -192.9588430854689705, -38.51493924976909966, -38.51493924976973915 ) ) ;
#22036=B_SPLINE_CURVE_WITH_KNOTS ( 'NONE', 3,
 ( #11990, #2028, #9498, #14383, #20380, #3385 ),
 .UNSPECIFIED., .F., .F.,
 ( 4, 2, 4 ),
 ( 0.000000000000000000, 0.004519197161541735688, 0.009038394323083471377 ),
 .UNSPECIFIED. ) ;
#22037=CARTESIAN_POINT ( 'NONE',  ( 146.6084372240433993, -3.800685668858596156, -3.800685668858692967 ) ) ;
#22038=CARTESIAN_POINT ( 'NONE',  ( -53.37769371643646110, 10.11111068829013249, 29.42719939405408169 ) ) ;
#22039=CARTESIAN_POINT ( 'NONE',  ( -91.56559293963834989, -16.03295912088728414, 16.03295912088688269 ) ) ;
#22044=CARTESIAN_POINT ( 'NONE',  ( -208.1127848780264742, -40.00000000000011369, 15.00245453012655439 ) ) ;
#22045=CARTESIAN_POINT ( 'NONE',  ( -259.2033419157646676, 6.730120644403521979, -6.730120644403498886 ) ) ;
#22047=CARTESIAN_POINT ( 'NONE',  ( 4.995406935893288214, 55.24977328853207581, 40.00000000000002132 ) ) ;
#22048=ORIENTED_EDGE ( 'NONE', *, *, #24365, .F. ) ;
#22050=CARTESIAN_POINT ( 'NONE',  ( 2.985930184390671371, 43.42223633017472650, 17.98607919652674170 ) ) ;
#22051=CARTESIAN_POINT ( 'NONE',  ( 60.14720761598005083, 10.94158980372334078, 33.22245024487595089 ) ) ;
#22052=CARTESIAN_POINT ( 'NONE',  ( -105.2274517607689290, -2.715151009219458622, 21.34875776644108569 ) ) ;
#22053=VERTEX_POINT ( 'NONE', #8900 ) ;
#22054=CARTESIAN_POINT ( 'NONE',  ( -190.7345856381647877, -47.78725959878028107, 13.94676320011207515 ) ) ;
#22056=CARTESIAN_POINT ( 'NONE',  ( 17.91733029164682023, -14.04577174279065943, 48.44632265249130398 ) ) ;
#22058=CARTESIAN_POINT ( 'NONE',  ( 22.01478053666848211, 13.87318432395317203, -47.29427690643910154 ) ) ;
#22062=CARTESIAN_POINT ( 'NONE',  ( -151.4802930567624912, -11.09498731346505451, 33.96623840860532084 ) ) ;
#22063=CARTESIAN_POINT ( 'NONE',  ( -105.3755690713226727, 12.89780903124418998, -12.89780903124389155 ) ) ;
#22064=CARTESIAN_POINT ( 'NONE',  ( -192.9588430854690273, -54.46834944098226572, 40.00000000000002132 ) ) ;
#22065=CARTESIAN_POINT ( 'NONE',  ( -121.8281150762304748, 8.694016615518547653, -23.07023398454548868 ) ) ;
#22066=CARTESIAN_POINT ( 'NONE',  ( -86.96347745069644475, 12.89780903124349898, 43.67073346367994446 ) ) ;
#22067=CARTESIAN_POINT ( 'NONE',  ( 98.29850319125813485, -18.22532005591201809, -8.262390927758364256 ) ) ;
#22068=CARTESIAN_POINT ( 'NONE',  ( 136.1360204305621266, 35.03383547441298873, 0.000000000000000000 ) ) ;
#22069=CARTESIAN_POINT ( 'NONE',  ( -259.2033419157646676, 30.48217210827734647, 40.00000000000002132 ) ) ;
#22070=CARTESIAN_POINT ( 'NONE',  ( 19.06497207195981858, 5.735870351258996432E-13, -54.19242893257843008 ) ) ;
#22071=CARTESIAN_POINT ( 'NONE',  ( 4.995406935893290878, 1.606505379428369110E-13, -15.24977328854832592 ) ) ;
#22073=CARTESIAN_POINT ( 'NONE',  ( 57.59792236341147031, 30.00663442387720181, -26.56190807104661289 ) ) ;
#22075=CARTESIAN_POINT ( 'NONE',  ( -77.90255099906769942, -20.29001641120661859, 8.064892378658379712 ) ) ;
#22076=CARTESIAN_POINT ( 'NONE',  ( 192.4448373802100889, 20.00000000003945644, 0.000000000000000000 ) ) ;
#22081=CARTESIAN_POINT ( 'NONE',  ( 146.6084372240433709, -3.800685668858344801, -52.76785682606520567 ) ) ;
#22082=CARTESIAN_POINT ( 'NONE',  ( 23.48902902575148488, -42.82177761400719618, -23.31625887490651650 ) ) ;
#22084=CARTESIAN_POINT ( 'NONE',  ( 130.8568914410475088, -34.05028731879786363, -40.00000000000002132 ) ) ;
#22085=CARTESIAN_POINT ( 'NONE',  ( -102.4294859497687327, -20.29697089191209969, 8.407280618541118855 ) ) ;
#22089=DIRECTION ( 'NONE',  ( 0.9352143328345118301, -0.3271292286605502753, 0.1355013631549612796 ) ) ;
#22090=CARTESIAN_POINT ( 'NONE',  ( -213.1075012329537230, 37.98287015391236565, -18.58567234101138510 ) ) ;
#22091=CARTESIAN_POINT ( 'NONE',  ( -183.6285492668830557, -41.87133366545522506, -17.34367427884065549 ) ) ;
#22092=CARTESIAN_POINT ( 'NONE',  ( -259.2033419157646676, -1.564921101325656229E-13, 30.48217210827739621 ) ) ;
#22093=CARTESIAN_POINT ( 'NONE',  ( -135.8532207217289738, -9.153146818113595984, 0.000000000000000000 ) ) ;
#22095=CYLINDRICAL_SURFACE ( 'NONE', #919, 30.00000000000003908 ) ;
#22096=CARTESIAN_POINT ( 'NONE',  ( 170.2234770963711128, 1.169953928977015745E-13, -24.55285855007187124 ) ) ;
#22098=CARTESIAN_POINT ( 'NONE',  ( -91.56559293963834989, -40.00000000000027711, 22.67402823373149801 ) ) ;
#22100=CARTESIAN_POINT ( 'NONE',  ( -100.7734535825088500, 16.03295912088683295, 40.53558337403684675 ) ) ;
#22101=CARTESIAN_POINT ( 'NONE',  ( 184.8905102610680444, 20.92133201514447194, -40.00000000000002132 ) ) ;
#22102=CARTESIAN_POINT ( 'NONE',  ( -208.1127848780264742, -67.17687982763172272, 10.60833733270744617 ) ) ;
#22104=AXIS2_PLACEMENT_3D ( 'NONE', #15452, #1893, #13983 ) ;
#22106=CARTESIAN_POINT ( 'NONE',  ( -259.2033419157646676, -40.00000000000003553, -9.517827891722768996 ) ) ;
#22107=CARTESIAN_POINT ( 'NONE',  ( -198.0356074513804572, 39.15871834505912119, -17.40982414986464377 ) ) ;
#22108=CARTESIAN_POINT ( 'NONE',  ( -135.8532207217289738, 6.472252184284096543, 6.472252184284234211 ) ) ;
#22109=CARTESIAN_POINT ( 'NONE',  ( -188.3066136396867307, -13.82848859481001647, -46.99300418776059729 ) ) ;
#22110=CARTESIAN_POINT ( 'NONE',  ( -86.96347745069644475, 15.38646221621793586, -15.38646221621778842 ) ) ;
#22111=ORIENTED_EDGE ( 'NONE', *, *, #2485, .T. ) ;
#22112=CARTESIAN_POINT ( 'NONE',  ( -280.0000000000000000, -14.14213562373118549, 14.14213562373078936 ) ) ;
#22114=CARTESIAN_POINT ( 'NONE',  ( 192.4448373802100889, 14.14213562375893574, -14.14213562375874922 ) ) ;
#22115=CARTESIAN_POINT ( 'NONE',  ( -100.7734535825088500, 22.67402823373189591, -0.000000000000000000 ) ) ;
#22117=CARTESIAN_POINT ( 'NONE',  ( 91.82158438592158234, -12.16597498399995203, -44.40256751092347542 ) ) ;
#22122=CARTESIAN_POINT ( 'NONE',  ( -6.342283169555448907, 23.00001740814278506, 42.32555349774906972 ) ) ;
#22125=CARTESIAN_POINT ( 'NONE',  ( -213.1075012329537230, 9.698598906450410340, 9.698598906450483170 ) ) ;
#22127=CARTESIAN_POINT ( 'NONE',  ( -86.96347745069644475, -15.38646221621786125, -15.38646221621789856 ) ) ;
#22130=CARTESIAN_POINT ( 'NONE',  ( 85.88436428469954365, 10.32541753206531432, -22.72801546669109385 ) ) ;
#22133=CARTESIAN_POINT ( 'NONE',  ( -4.039451493210490796, -23.44932283416679297, 43.00522595894000943 ) ) ;
#22135=CARTESIAN_POINT ( 'NONE',  ( -166.3490444791740401, 19.13701437391346616, 36.43931842066525917 ) ) ;
#22136=CARTESIAN_POINT ( 'NONE',  ( -4.082462733454488735, -13.82507958736516684, -46.97557262069201300 ) ) ;
#22137=CARTESIAN_POINT ( 'NONE',  ( 170.2234770963711128, -39.20704971665404059, 17.36149277826957160 ) ) ;
#22138=CARTESIAN_POINT ( 'NONE',  ( 98.29820294267862835, 15.90088694521858415, -12.38338430224807851 ) ) ;
#22139=CARTESIAN_POINT ( 'NONE',  ( -192.9588430854689705, -38.51493924976963967, 38.51493924976919914 ) ) ;
#22140=CARTESIAN_POINT ( 'NONE',  ( 151.7948205124836250, -3.202120068677277203E-13, 33.23291073765553705 ) ) ;
#22141=CARTESIAN_POINT ( 'NONE',  ( 151.7948205124836250, 33.23291073765556547, 0.000000000000000000 ) ) ;
#22142=CARTESIAN_POINT ( 'NONE',  ( -135.8532207217289738, -30.84685318188647685, -2.449293598294708485E-15 ) ) ;
#22145=CARTESIAN_POINT ( 'NONE',  ( -100.7734535825088500, -17.32597176626813251, 40.00000000000002132 ) ) ;
#22147=CARTESIAN_POINT ( 'NONE',  ( -97.72675010090206627, 20.89622088363370622, -8.185591577777238115 ) ) ;
#22148=CARTESIAN_POINT ( 'NONE',  ( -91.56559293963836410, 40.00000000000019185, -17.32597176626768487 ) ) ;
#22149=CARTESIAN_POINT ( 'NONE',  ( 4.995406935893289102, 10.78321810388998081, 10.78321810389001811 ) ) ;
#22150=CARTESIAN_POINT ( 'NONE',  ( -162.0762913951021176, 1.694272876828294194, -40.00000000000002132 ) ) ;
#22152=CARTESIAN_POINT ( 'NONE',  ( -100.7734535825088500, -22.67402823373193499, 40.00000000000002132 ) ) ;
#22154=CARTESIAN_POINT ( 'NONE',  ( 118.9130007099547299, 10.68958087202317131, 25.80693111732301048 ) ) ;
#22156=CARTESIAN_POINT ( 'NONE',  ( -198.0356074513804572, 67.44298959253333692, 10.87444709760969452 ) ) ;
#22157=CARTESIAN_POINT ( 'NONE',  ( -105.3755690713226585, -40.00000000000010658, 18.24025645688337249 ) ) ;
#22158=CIRCLE ( 'NONE', #24711, 40.00000000000003553 ) ;
#22159=ADVANCED_FACE ( 'NONE', ( #18614 ), #8755, .T. ) ;
#22160=CARTESIAN_POINT ( 'NONE',  ( -30.26275506840324070, 1.694272468446254232, 0.000000000000000000 ) ) ;
#22168=B_SPLINE_CURVE_WITH_KNOTS ( 'NONE', 3,
 ( #24583, #14461, #20586, #17558, #22592, #14854 ),
 .UNSPECIFIED., .F., .F.,
 ( 4, 2, 4 ),
 ( -5.998621906156382924E-08, 0.03938016914544737596, 0.07876039827711382724 ),
 .UNSPECIFIED. ) ;
#22169=CARTESIAN_POINT ( 'NONE',  ( 91.82158438592158234, 16.11829626346161604, -16.11829626346121103 ) ) ;
#22170=CARTESIAN_POINT ( 'NONE',  ( 136.1360204305621551, -31.79587985999279454, 24.77266263493094911 ) ) ;
#22171=CARTESIAN_POINT ( 'NONE',  ( -105.4894168351564048, 19.67999904371083275, 8.151722511394638104 ) ) ;
#22172=CARTESIAN_POINT ( 'NONE',  ( -259.2033419157646676, -1.473088368616265084E-13, 9.517827891722632216 ) ) ;
#22173=CARTESIAN_POINT ( 'NONE',  ( -259.2033419157646676, -21.55415060305872998, 35.01439189186525880 ) ) ;
#22174=CARTESIAN_POINT ( 'NONE',  ( 151.7948205124836250, -23.49921654116371883, 23.49921654116317526 ) ) ;
#22175=CARTESIAN_POINT ( 'NONE',  ( 184.8905102610680444, -43.07788698682556827, -13.49065550809859104 ) ) ;
#22176=CARTESIAN_POINT ( 'NONE',  ( -198.0356074513804572, -39.15871834505905724, -17.40982414986491733 ) ) ;
#22179=CARTESIAN_POINT ( 'NONE',  ( -162.0762913951021176, -40.00000000000019895, 41.69427287672974813 ) ) ;
#22182=CARTESIAN_POINT ( 'NONE',  ( 8.209392600929815487, 44.89226883836261806, -24.84362085272430676 ) ) ;
#22183=CARTESIAN_POINT ( 'NONE',  ( 4.995406935893288214, 55.24977328854835434, 2.449293598294708485E-15 ) ) ;
#22186=CARTESIAN_POINT ( 'NONE',  ( 51.52267038239544661, 34.28362880217498798, 14.20074401722577839 ) ) ;
#22188=CARTESIAN_POINT ( 'NONE',  ( 151.7948205124836250, -33.23291073765550863, 0.000000000000000000 ) ) ;
#22190=CARTESIAN_POINT ( 'NONE',  ( -189.1288337602858860, -43.24060467048573031, 23.62383291543415709 ) ) ;
#22192=CARTESIAN_POINT ( 'NONE',  ( 11.59303701482094517, -18.58252782966835781, 44.86219070952759580 ) ) ;
#22193=CARTESIAN_POINT ( 'NONE',  ( 23.54890483848243221, 23.30407993985267012, -42.80335737019193942 ) ) ;
#22196=CARTESIAN_POINT ( 'NONE',  ( 137.0939645874030930, -30.33050608226204758, 12.56330697291239140 ) ) ;
#22197=CARTESIAN_POINT ( 'NONE',  ( -200.0000000000000000, 60.00000000000009948, 0.000000000000000000 ) ) ;
#22198=( BOUNDED_SURFACE ( )  B_SPLINE_SURFACE ( 3, 3, ( 
 ( #21881, #8036, #24004, #9508, #3658, #5647, #7763, #5784, #3525, #26296, #19884, #5921, #1667, #3796, #5520, #17613, #25886, #7629, #18147, #13753, #24287, #19622, #18012, #13891, #1407, #22025, #25757, #11899, #9775, #26026 ),
 ( #26159, #16155, #22292, #7505, #6056, #15742, #20023, #1803, #7901, #9642, #17745, #1935, #14160, #1537, #15615, #9906, #20153, #3938, #17876, #16020, #24145, #23739, #23872, #13625, #14029, #12034, #10040, #21751, #11626, #19747 ),
 ( #2202, #8174, #12428, #18416, #6181, #22821, #20290, #10311, #4069, #332, #14294, #4204, #14426, #191, #22557, #469, #16289, #24683, #8573, #8301, #2069, #16686, #10436, #24817, #24553, #18280, #12171, #12296, #14557, #4336 ),
 ( #16426, #66, #22429, #6570, #14690, #24416, #18552, #6308, #20556, #10176, #20423, #2325, #8437, #16555, #6441, #22688, #4463, #2458, #12557, #20690, #10570, #18684, #4598, #12696, #19977, #22251, #1758, #20116, #21843, #25849 ),
 ( #8132, #21980, #14249, #1495, #7993, #5878, #17706, #13984, #7593, #1894, #17969, #15976, #3613, #5612, #15705, #14123, #4027, #16249, #24104, #24377, #22117, #9601, #12125, #2031, #20250, #3894, #6141, #16112, #10133, #7724 ),
 ( #9867, #26257, #24242, #23829, #13846, #13718, #6014, #18236, #7855, #11724, #21, #25984, #26116, #19843, #22389, #4166, #1628, #9735, #12259, #17837, #9999, #15835, #23965, #3751, #11994, #18107, #5740, #11857, #20780, #4686 ),
 ( #16774, #156, #23047, #8529, #20643, #24776, #560, #8665, #10667, #2159, #4558, #24512, #4822, #8798, #16377, #20383, #12514, #14778, #2418, #12654, #14386, #18377, #8393, #16515, #689, #14514, #6796, #10267, #24907, #6529 ) ),
 .UNSPECIFIED., .T., .F., .F. ) 
 B_SPLINE_SURFACE_WITH_KNOTS ( ( 4, 3, 4 ),
 ( 4, 2, 2, 2, 2, 2, 2, 2, 2, 2, 2, 2, 2, 2, 4 ),
 ( 0.000000000000000000, 0.5000000000000000000, 1.000000000000000000 ),
 ( 0.000000000000000000, 0.1357259735107005372, 0.1651108541090157700, 0.1944957347073310028, 0.3598804999793158710, 0.3867117631979620773, 0.4135430264166082281, 0.5789277916885930964, 0.6062785021374117456, 0.6336292125862302838, 0.8508620842112317728, 0.8814014469398914198, 0.9119408096685510667, 0.9559704048342755334, 1.000000000000000000 ),
 .UNSPECIFIED. ) 
 GEOMETRIC_REPRESENTATION_ITEM ( )  RATIONAL_B_SPLINE_SURFACE ( (
 ( 1.000000000000000000, 1.000000000000000000, 1.000000000000000000, 1.000000000000000000, 1.000000000000000000, 1.000000000000000000, 1.000000000000000000, 1.000000000000000000, 1.000000000000000000, 1.000000000000000000, 1.000000000000000000, 1.000000000000000000, 1.000000000000000000, 1.000000000000000000, 1.000000000000000000, 1.000000000000000000, 1.000000000000000000, 1.000000000000000000, 1.000000000000000000, 1.000000000000000000, 1.000000000000000000, 1.000000000000000000, 1.000000000000000000, 1.000000000000000000, 1.000000000000000000, 1.000000000000000000, 1.000000000000000000, 1.000000000000000000, 1.000000000000000000, 1.000000000000000000),
 ( 0.3333333333333333703, 0.3333333333333333703, 0.3333333333333333703, 0.3333333333333333703, 0.3333333333333333703, 0.3333333333333333703, 0.3333333333333333703, 0.3333333333333333703, 0.3333333333333333703, 0.3333333333333333703, 0.3333333333333333703, 0.3333333333333333703, 0.3333333333333333703, 0.3333333333333333703, 0.3333333333333333703, 0.3333333333333333703, 0.3333333333333333703, 0.3333333333333333703, 0.3333333333333333703, 0.3333333333333333703, 0.3333333333333333703, 0.3333333333333333703, 0.3333333333333333703, 0.3333333333333333703, 0.3333333333333333703, 0.3333333333333333703, 0.3333333333333333703, 0.3333333333333333703, 0.3333333333333333703, 0.3333333333333333703),
 ( 0.3333333333333333703, 0.3333333333333333703, 0.3333333333333333703, 0.3333333333333333703, 0.3333333333333333703, 0.3333333333333333703, 0.3333333333333333703, 0.3333333333333333703, 0.3333333333333333703, 0.3333333333333333703, 0.3333333333333333703, 0.3333333333333333703, 0.3333333333333333703, 0.3333333333333333703, 0.3333333333333333703, 0.3333333333333333703, 0.3333333333333333703, 0.3333333333333333703, 0.3333333333333333703, 0.3333333333333333703, 0.3333333333333333703, 0.3333333333333333703, 0.3333333333333333703, 0.3333333333333333703, 0.3333333333333333703, 0.3333333333333333703, 0.3333333333333333703, 0.3333333333333333703, 0.3333333333333333703, 0.3333333333333333703),
 ( 1.000000000000000000, 1.000000000000000000, 1.000000000000000000, 1.000000000000000000, 1.000000000000000000, 1.000000000000000000, 1.000000000000000000, 1.000000000000000000, 1.000000000000000000, 1.000000000000000000, 1.000000000000000000, 1.000000000000000000, 1.000000000000000000, 1.000000000000000000, 1.000000000000000000, 1.000000000000000000, 1.000000000000000000, 1.000000000000000000, 1.000000000000000000, 1.000000000000000000, 1.000000000000000000, 1.000000000000000000, 1.000000000000000000, 1.000000000000000000, 1.000000000000000000, 1.000000000000000000, 1.000000000000000000, 1.000000000000000000, 1.000000000000000000, 1.000000000000000000),
 ( 0.3333333333333333703, 0.3333333333333333703, 0.3333333333333333703, 0.3333333333333333703, 0.3333333333333333703, 0.3333333333333333703, 0.3333333333333333703, 0.3333333333333333703, 0.3333333333333333703, 0.3333333333333333703, 0.3333333333333333703, 0.3333333333333333703, 0.3333333333333333703, 0.3333333333333333703, 0.3333333333333333703, 0.3333333333333333703, 0.3333333333333333703, 0.3333333333333333703, 0.3333333333333333703, 0.3333333333333333703, 0.3333333333333333703, 0.3333333333333333703, 0.3333333333333333703, 0.3333333333333333703, 0.3333333333333333703, 0.3333333333333333703, 0.3333333333333333703, 0.3333333333333333703, 0.3333333333333333703, 0.3333333333333333703),
 ( 0.3333333333333333703, 0.3333333333333333703, 0.3333333333333333703, 0.3333333333333333703, 0.3333333333333333703, 0.3333333333333333703, 0.3333333333333333703, 0.3333333333333333703, 0.3333333333333333703, 0.3333333333333333703, 0.3333333333333333703, 0.3333333333333333703, 0.3333333333333333703, 0.3333333333333333703, 0.3333333333333333703, 0.3333333333333333703, 0.3333333333333333703, 0.3333333333333333703, 0.3333333333333333703, 0.3333333333333333703, 0.3333333333333333703, 0.3333333333333333703, 0.3333333333333333703, 0.3333333333333333703, 0.3333333333333333703, 0.3333333333333333703, 0.3333333333333333703, 0.3333333333333333703, 0.3333333333333333703, 0.3333333333333333703),
 ( 1.000000000000000000, 1.000000000000000000, 1.000000000000000000, 1.000000000000000000, 1.000000000000000000, 1.000000000000000000, 1.000000000000000000, 1.000000000000000000, 1.000000000000000000, 1.000000000000000000, 1.000000000000000000, 1.000000000000000000, 1.000000000000000000, 1.000000000000000000, 1.000000000000000000, 1.000000000000000000, 1.000000000000000000, 1.000000000000000000, 1.000000000000000000, 1.000000000000000000, 1.000000000000000000, 1.000000000000000000, 1.000000000000000000, 1.000000000000000000, 1.000000000000000000, 1.000000000000000000, 1.000000000000000000, 1.000000000000000000, 1.000000000000000000, 1.000000000000000000) ) ) 
 REPRESENTATION_ITEM ( '' )  SURFACE ( )  );
#22199=CARTESIAN_POINT ( 'NONE',  ( -280.0000000000000000, 14.14213562373108246, -14.14213562373078581 ) ) ;
#22200=CARTESIAN_POINT ( 'NONE',  ( -280.0000000000000000, 19.99999999999996092, -0.000000000000000000 ) ) ;
#22201=CARTESIAN_POINT ( 'NONE',  ( -188.2871287166302636, 13.82723289751406703, -46.98614659774629843 ) ) ;
#22202=CARTESIAN_POINT ( 'NONE',  ( 170.0000000000000853, -9.369682556672300322, 22.62041470344878746 ) ) ;
#22203=CARTESIAN_POINT ( 'NONE',  ( 98.29820294267378245, -17.32045324915796769, -10.02182676112147774 ) ) ;
#22204=CARTESIAN_POINT ( 'NONE',  ( 19.06497207195981503, -14.19242893257840166, 0.000000000000000000 ) ) ;
#22205=CARTESIAN_POINT ( 'NONE',  ( 0.2972598230769930572, 14.33493731733933352, 0.000000000000000000 ) ) ;
#22206=CARTESIAN_POINT ( 'NONE',  ( -259.2033419157646676, -39.99999999999975131, -30.48217210827782608 ) ) ;
#22207=CARTESIAN_POINT ( 'NONE',  ( -162.0762913951020892, 57.76657433537918251, 1.198031840455469066 ) ) ;
#22209=CARTESIAN_POINT ( 'NONE',  ( 170.2234770963711128, 17.36149277826980253, 17.36149277827007253 ) ) ;
#22210=ORIENTED_EDGE ( 'NONE', *, *, #17029, .T. ) ;
#22211=CARTESIAN_POINT ( 'NONE',  ( 91.82158438592158234, -40.45024623143958564, 16.11829626348418998 ) ) ;
#22212=CARTESIAN_POINT ( 'NONE',  ( -86.86493150571116928, -7.943527260496078490, 19.77569912839177135 ) ) ;
#22213=ORIENTED_EDGE ( 'NONE', *, *, #21911, .T. ) ;
#22215=CARTESIAN_POINT ( 'NONE',  ( 184.8905102610680444, -13.49065550809780412, -43.07788698682583828 ) ) ;
#22216=CARTESIAN_POINT ( 'NONE',  ( 22.33254948916634319, -43.29223140031879780, -17.93222939140903449 ) ) ;
#22218=CARTESIAN_POINT ( 'NONE',  ( 170.2234770963711128, -24.55285855007184281, -40.00000000000002132 ) ) ;
#22223=CARTESIAN_POINT ( 'NONE',  ( 200.0000000000000000, 42.42640687119288856, -14.14213562373094746 ) ) ;
#22224=CARTESIAN_POINT ( 'NONE',  ( -188.4265466358226035, -43.04237830659937458, -23.47687925214709637 ) ) ;
#22225=CARTESIAN_POINT ( 'NONE',  ( -56.48582580120558561, -40.00000000000000000, -9.153146818113723882 ) ) ;
#22226=CARTESIAN_POINT ( 'NONE',  ( 130.8568914410475372, -34.05028731879786363, 0.000000000000000000 ) ) ;
#22229=CARTESIAN_POINT ( 'NONE',  ( 91.82158438592159655, -39.99999999999994316, -17.20528682183314118 ) ) ;
#22230=CARTESIAN_POINT ( 'NONE',  ( -238.4067589809705794, -40.00000000000021316, 40.96449427990166470 ) ) ;
#22231=CARTESIAN_POINT ( 'NONE',  ( -56.48582580120559271, -1.062504017861011783E-13, 9.153146818113587102 ) ) ;
#22232=CARTESIAN_POINT ( 'NONE',  ( 146.6084372240433709, 40.00000000000017053, -34.62501878078291639 ) ) ;
#22234=CARTESIAN_POINT ( 'NONE',  ( 199.9999999999999432, 20.00000000000013856, 0.000000000000000000 ) ) ;
#22235=CARTESIAN_POINT ( 'NONE',  ( -100.7734535825088500, -40.53558337403669753, -16.03295912088728770 ) ) ;
#22236=CARTESIAN_POINT ( 'NONE',  ( -100.7734535825088500, 22.67402823373189591, -0.000000000000000000 ) ) ;
#22237=CARTESIAN_POINT ( 'NONE',  ( -100.7734535825088500, -12.25131212657462498, -44.31723036834905827 ) ) ;
#22240=CARTESIAN_POINT ( 'NONE',  ( 151.7948205124836250, 23.49921654116328540, 23.49921654116366554 ) ) ;
#22241=CARTESIAN_POINT ( 'NONE',  ( -208.1127848780265026, -2.327190355601776466E-13, 55.00245453012672670 ) ) ;
#22242=CARTESIAN_POINT ( 'NONE',  ( 199.9999999999999432, 14.14213562373090838, 14.14213562373092437 ) ) ;
#22243=CARTESIAN_POINT ( 'NONE',  ( -213.1075012329537230, -9.698598906450422774, -9.698598906450550672 ) ) ;
#22244=CARTESIAN_POINT ( 'NONE',  ( -190.7346372395361129, -13.94676542151222343, -47.78727444209329889 ) ) ;
#22245=CARTESIAN_POINT ( 'NONE',  ( -280.0000000000000568, -14.14213562373078226, -42.42640687119295251 ) ) ;
#22246=ORIENTED_EDGE ( 'NONE', *, *, #17665, .F. ) ;
#22247=CARTESIAN_POINT ( 'NONE',  ( -56.48582580120559982, -34.75652343174584047, -21.81201906317815187 ) ) ;
#22249=CARTESIAN_POINT ( 'NONE',  ( 14.38125909742181285, -15.17850393972633505, 0.000000000000000000 ) ) ;
#22250=CARTESIAN_POINT ( 'NONE',  ( -86.84962968273566730, 19.67999904273991163, 8.151722510992470916 ) ) ;
#22251=CARTESIAN_POINT ( 'NONE',  ( 163.1118516004056573, 9.006482792069759213, -9.006482792069505194 ) ) ;
#22255=CARTESIAN_POINT ( 'NONE',  ( 23.23639021239535651, -23.37084785298091916, 42.89921396172186974 ) ) ;
#22257=CARTESIAN_POINT ( 'NONE',  ( -4.082462733456166504, 23.44093842354227419, 42.99255347688187356 ) ) ;
#22258=ORIENTED_EDGE ( 'NONE', *, *, #2836, .T. ) ;
#22260=CARTESIAN_POINT ( 'NONE',  ( -100.7734535825088358, -16.03295912088706743, -16.03295912088710296 ) ) ;
#22262=CARTESIAN_POINT ( 'NONE',  ( -114.4364955367327212, -8.064892380842954012, -20.29001642038816300 ) ) ;
#22265=CARTESIAN_POINT ( 'NONE',  ( 17.75917276260960875, 44.20478326162373151, -24.33671690504812801 ) ) ;
#22266=ADVANCED_FACE ( 'NONE', ( #7128 ), #6730, .T. ) ;
#22267=CARTESIAN_POINT ( 'NONE',  ( -100.7734535825088500, 39.99999999999976552, 22.67402823373233645 ) ) ;
#22269=CARTESIAN_POINT ( 'NONE',  ( -77.70091844760044353, -21.35079699648278861, -5.501606197251263985 ) ) ;
#22271=B_SPLINE_CURVE_WITH_KNOTS ( 'NONE', 3,
 ( #13904, #16167, #22038, #17889, #22569, #3810 ),
 .UNSPECIFIED., .F., .F.,
 ( 4, 2, 4 ),
 ( 0.000000000000000000, 0.03937634048170812057, 0.07875268096341624113 ),
 .UNSPECIFIED. ) ;
#22273=CARTESIAN_POINT ( 'NONE',  ( -114.4364955367302912, 8.644468109216418839, 20.04994829327247530 ) ) ;
#22274=CARTESIAN_POINT ( 'NONE',  ( -4.004886986944679705, -13.82996668233299431, -47.00296421444959805 ) ) ;
#22275=CARTESIAN_POINT ( 'NONE',  ( -198.0356074513804288, -39.15871834505882276, -39.15871834505946936 ) ) ;
#22276=CARTESIAN_POINT ( 'NONE',  ( -100.0753760173601279, 20.41987330121804334, -8.894334231739408736 ) ) ;
#22277=CARTESIAN_POINT ( 'NONE',  ( -259.2033419157646676, -49.83842185052031937, -6.730120644403796426 ) ) ;
#22278=CARTESIAN_POINT ( 'NONE',  ( 130.8568914410475088, -40.00000000000036238, 34.05028731879746573 ) ) ;
#22279=CARTESIAN_POINT ( 'NONE',  ( -162.0762913951021176, 27.08623940707639477, -29.48230308784743059 ) ) ;
#22280=CARTESIAN_POINT ( 'NONE',  ( 200.0000000000000000, -19.99999999999989342, 40.00000000000002132 ) ) ;
#22282=CARTESIAN_POINT ( 'NONE',  ( 146.6084372240433993, -5.374981219216945938, -2.449293598294708485E-15 ) ) ;
#22283=CARTESIAN_POINT ( 'NONE',  ( -110.0830815298113095, 11.16636597695389987, 16.82107498772007759 ) ) ;
#22284=CARTESIAN_POINT ( 'NONE',  ( -91.56559293963836410, 39.99999999999976552, 22.67402823373234000 ) ) ;
#22285=CARTESIAN_POINT ( 'NONE',  ( 146.6084372240433993, -24.48358557860319706, -24.48358557860330720 ) ) ;
#22286=CARTESIAN_POINT ( 'NONE',  ( 91.82158438592158234, -17.20528682183298486, 0.000000000000000000 ) ) ;
#22287=VERTEX_POINT ( 'NONE', #23435 ) ;
#22289=CARTESIAN_POINT ( 'NONE',  ( -56.48582580120559982, -9.153146818113595984, 40.00000000000002132 ) ) ;
#22290=CARTESIAN_POINT ( 'NONE',  ( 146.5090579137182090, 12.40347562390415348, 29.94463907179425988 ) ) ;
#22291=CARTESIAN_POINT ( 'NONE',  ( -91.56559293963834989, -40.00000000000009948, 17.32597176626796553 ) ) ;
#22292=CARTESIAN_POINT ( 'NONE',  ( -238.4067589809705794, 28.96627169325285678, 27.60227080167094726 ) ) ;
#22293=CARTESIAN_POINT ( 'NONE',  ( 146.6084372240433993, -34.62501878078303008, 0.000000000000000000 ) ) ;
#22294=CARTESIAN_POINT ( 'NONE',  ( -196.0240701155048271, -44.60678452943326988, -24.63338802315930565 ) ) ;
#22296=CARTESIAN_POINT ( 'NONE',  ( -190.1760961841080757, 13.92889018282242830, -47.67020129349042179 ) ) ;
#22299=CARTESIAN_POINT ( 'NONE',  ( -30.26275506840325136, 57.76657404653985139, -1.198031551615314161 ) ) ;
#22300=CARTESIAN_POINT ( 'NONE',  ( 130.8568914410475088, -32.49135343045495006, 24.07718906446878648 ) ) ;
#22301=CARTESIAN_POINT ( 'NONE',  ( -109.1264249741455927, -13.72187187124634278, -33.12752917268957020 ) ) ;
#22302=CARTESIAN_POINT ( 'NONE',  ( -82.30220482034332008, 18.51665893431357901, -7.992411108784951423 ) ) ;
#22303=CARTESIAN_POINT ( 'NONE',  ( 170.2234770963711128, -10.92277846919187034, -10.92277846919209594 ) ) ;
#22304=CARTESIAN_POINT ( 'NONE',  ( -87.02146317964813704, 10.86006974120160962, -18.50839211081806823 ) ) ;
#22305=CARTESIAN_POINT ( 'NONE',  ( -192.9588430854689989, 10.23066800230742679, 10.23066800230749607 ) ) ;
#22306=CARTESIAN_POINT ( 'NONE',  ( 19.06497207195981858, -38.31983398719616218, -18.24870850772777331 ) ) ;
#22308=ADVANCED_FACE ( 'NONE', ( #21561 ), #9444, .T. ) ;
#22310=CARTESIAN_POINT ( 'NONE',  ( -135.8532207217289738, 39.99999999999989342, 30.84685318188660474 ) ) ;
#22311=( BOUNDED_SURFACE ( )  B_SPLINE_SURFACE ( 3, 2, ( 
 ( #18606, #22736, #12346 ),
 ( #20475, #16479, #10226 ),
 ( #8761, #385, #12218 ),
 ( #8492, #20340, #24605 ),
 ( #18335, #24340, #22477 ),
 ( #18468, #114, #20605 ),
 ( #16339, #6625, #8358 ),
 ( #8221, #2657, #24471 ),
 ( #6359, #6234, #20745 ),
 ( #4387, #14349, #4650 ),
 ( #14478, #12479, #16738 ),
 ( #10493, #12617, #654 ) ),
 .UNSPECIFIED., .F., .F., .F. ) 
 B_SPLINE_SURFACE_WITH_KNOTS ( ( 4, 2, 2, 2, 2, 4 ),
 ( 3, 3 ),
 ( 0.006022589392325605230, 0.01254516766564424401, 0.01580645680230356384, 0.01906774593896288367, 0.02559032421228152332, 0.03211290248560016297 ),
 ( 0.000000000000000000, 1.000000000000000000 ),
 .UNSPECIFIED. ) 
 GEOMETRIC_REPRESENTATION_ITEM ( )  RATIONAL_B_SPLINE_SURFACE ( (
 ( 1.000000000000000000, 0.9998834880171258988, 1.000000000000000000),
 ( 1.000000000000000000, 0.9998139205012247510, 1.000000000000000000),
 ( 1.000000000000000000, 0.9997315632444677691, 1.000000000000000000),
 ( 1.000000000000000000, 0.9996405464946958030, 1.000000000000000000),
 ( 1.000000000000000000, 0.9996155081776924023, 1.000000000000000000),
 ( 1.000000000000000000, 0.9995814087511104562, 1.000000000000000000),
 ( 1.000000000000000000, 0.9995724100939918921, 1.000000000000000000),
 ( 1.000000000000000000, 0.9995726760936894939, 1.000000000000000000),
 ( 1.000000000000000000, 0.9996103361817947341, 1.000000000000000000),
 ( 1.000000000000000000, 0.9997312749795597142, 1.000000000000000000),
 ( 1.000000000000000000, 0.9998135910915183500, 1.000000000000000000),
 ( 1.000000000000000000, 0.9998834880173385065, 1.000000000000000000) ) ) 
 REPRESENTATION_ITEM ( '' )  SURFACE ( )  );
#22313=CARTESIAN_POINT ( 'NONE',  ( 23.46661716383107077, 42.82867125331087266, -23.32081713244353693 ) ) ;
#22314=CARTESIAN_POINT ( 'NONE',  ( 200.0000000000000000, 19.99999999999996447, -40.00000000000002132 ) ) ;
#22315=ORIENTED_EDGE ( 'NONE', *, *, #21627, .F. ) ;
#22316=CARTESIAN_POINT ( 'NONE',  ( 3.854700064722255792, -24.62824689551980839, -44.60002223906906238 ) ) ;
#22317=CARTESIAN_POINT ( 'NONE',  ( -62.79433447042003280, -24.94280497468228930, 11.74096317481567731 ) ) ;
#22318=CARTESIAN_POINT ( 'NONE',  ( -105.4741150117366431, -7.943527260727707429, 19.77569912956141707 ) ) ;
#22321=CARTESIAN_POINT ( 'NONE',  ( 23.09861257792924505, 23.40165480222934846, -42.94075326233378576 ) ) ;
#22322=B_SPLINE_CURVE_WITH_KNOTS ( 'NONE', 3,
 ( #23177, #20517, #20784, #14519, #4562, #4425, #2555, #10671, #7309, #21554, #25562, #960, #15423, #23673, #9314, #5453, #25684, #23550, #21427, #25305, #23798, #17546, #19549, #13554, #5321, #21681, #7432, #19674, #7182, #25814, #13061, #1335, #17421, #2953 ),
 .UNSPECIFIED., .F., .F.,
 ( 4, 2, 2, 2, 2, 2, 2, 2, 2, 2, 2, 2, 2, 2, 2, 2, 4 ),
 ( -5.298243351203664762E-05, 0.01887868273877483377, 0.02834451532491826659, 0.03071097347145414561, 0.03307743161799002463, 0.03544388976452590018, 0.03781034791106178267, 0.04254326420413354071, 0.04727618049720529875, 0.04964263864374118124, 0.05200909679027704985, 0.05674201308334873156, 0.05910847122988461405, 0.06029170030315258999, 0.06147492937642056593, 0.06620784566949247663, 0.07567367825563631190 ),
 .UNSPECIFIED. ) ;
#22324=CARTESIAN_POINT ( 'NONE',  ( 2.332272417612619719, -24.49123061639008370, 44.41409500755982975 ) ) ;
#22325=CARTESIAN_POINT ( 'NONE',  ( 22.37977766477551356, 23.55755712319015061, -43.15105302556542455 ) ) ;
#22327=CARTESIAN_POINT ( 'NONE',  ( 73.43438319820711513, -28.18283897611635069, 9.843172589489940449 ) ) ;
#22328=CARTESIAN_POINT ( 'NONE',  ( 153.3020327024398171, -28.42252382389432341, 11.77299484472919922 ) ) ;
#22329=CARTESIAN_POINT ( 'NONE',  ( 130.8568914410475372, 1.429239637432775288E-13, -34.05028731879788495 ) ) ;
#22330=CARTESIAN_POINT ( 'NONE',  ( -86.96347745069644475, 12.89780903124419353, -12.89780903124389333 ) ) ;
#22331=CARTESIAN_POINT ( 'NONE',  ( 91.82158438592158234, 17.20528682183301683, 0.000000000000000000 ) ) ;
#22332=AXIS2_PLACEMENT_3D ( 'NONE', #1932, #21877, #25883 ) ;
#22334=CARTESIAN_POINT ( 'NONE',  ( -187.7699188115417996, 23.34606611631939899, -42.84915433765981874 ) ) ;
#22335=CARTESIAN_POINT ( 'NONE',  ( 14.38125909742180752, 10.73282306404735387, -10.73282306404708919 ) ) ;
#22336=CARTESIAN_POINT ( 'NONE',  ( -86.96347745069645896, 21.75974354311648895, -0.000000000000000000 ) ) ;
#22337=CARTESIAN_POINT ( 'NONE',  ( 151.7948205124836534, -6.767089262349000656, -40.00000000000002132 ) ) ;
#22338=CARTESIAN_POINT ( 'NONE',  ( 91.82158438592158234, 22.79471317813472098, 2.449293598294708485E-15 ) ) ;
#22339=CARTESIAN_POINT ( 'NONE',  ( -259.2033419157646676, 2.741182173978444749E-13, -30.48217210827739621 ) ) ;
#22340=CARTESIAN_POINT ( 'NONE',  ( -198.0356074513804572, 67.44298959253333692, 10.87444709760969452 ) ) ;
#22341=CARTESIAN_POINT ( 'NONE',  ( 98.29820294273281434, -7.653668647304240125, 18.47759065023114644 ) ) ;
#22342=CARTESIAN_POINT ( 'NONE',  ( -100.7734535825088500, 44.31723036834907958, -12.25131212657445801 ) ) ;
#22344=CARTESIAN_POINT ( 'NONE',  ( 163.1118516004056573, -19.27778845538761132, -19.27778845538770724 ) ) ;
#22345=CIRCLE ( 'NONE', #15114, 15.00000000000000178 ) ;
#22346=CARTESIAN_POINT ( 'NONE',  ( -193.0908841288066071, -14.03723590834271739, -48.38979025835740799 ) ) ;
#22347=CARTESIAN_POINT ( 'NONE',  ( 57.59792236341147031, 37.56421063658187620, -40.00000000000002132 ) ) ;
#22349=ORIENTED_EDGE ( 'NONE', *, *, #18883, .T. ) ;
#22350=CARTESIAN_POINT ( 'NONE',  ( -86.96347745069645896, -12.89780903124382938, -43.67073346367985920 ) ) ;
#22351=CARTESIAN_POINT ( 'NONE',  ( 67.90397382950679628, -28.69135535083399802, -14.12691053321092483 ) ) ;
#22352=EDGE_CURVE ( 'NONE', #19642, #5232, #15257, .T. ) ;
#22353=ORIENTED_EDGE ( 'NONE', *, *, #6054, .T. ) ;
#22354=CARTESIAN_POINT ( 'NONE',  ( -162.0762913951020892, 1.694272876828294194, 0.000000000000000000 ) ) ;
#22355=CARTESIAN_POINT ( 'NONE',  ( -97.73860346101268703, -20.89580782307320206, 8.185503820996688162 ) ) ;
#22360=DIRECTION ( 'NONE',  ( 0.9352143328346287365, -0.1355013631592235090, -0.3271292286584503994 ) ) ;
#22361=CARTESIAN_POINT ( 'NONE',  ( 199.9999999999999432, -14.14213562373096345, -14.14213562373104871 ) ) ;
#22362=CARTESIAN_POINT ( 'NONE',  ( -187.3037411061945079, -46.64555264106432730, -13.75782484033866915 ) ) ;
#22363=( BOUNDED_SURFACE ( )  B_SPLINE_SURFACE ( 3, 3, ( 
 ( #9451, #5592, #17557, #17816, #13825, #18087, #2266, #16090, #8374, #21958, #2136, #249, #11835, #8110, #1738, #14229, #12104, #12364, #1875, #20229, #13962, #9847, #16496, #5993, #2008, #22369, #22096, #14100, #16227, #20362 ),
 ( #15955, #19954, #9978, #26238, #10374, #24220, #24621, #3732, #10246, #24357, #17950, #6121, #26097, #4145, #10113, #18213, #24082, #7833, #5856, #8239, #22229, #12238, #4005, #3871, #18356, #11972, #6252, #22496, #14365, #135 ),
 ( #6376, #16357, #4275, #20493, #24491, #18485, #266, #20097, #7972, #405, #10912, #19023, #20893, #8508, #4925, #12632, #14755, #2397, #25153, #932, #12495, #18622, #2928, #17146, #6774, #21018, #20759, #538, #12766, #14886 ),
 ( #2670, #4401, #20622, #10508, #802, #23026, #12902, #11037, #8643, #18888, #2801, #8907, #4801, #22626, #25021, #16625, #25280, #19147, #24756, #14495, #667, #4664, #6509, #10646, #14620, #17017, #9041, #13036, #6904, #22757 ),
 ( #23151, #4535, #6641, #10775, #16752, #18756, #2529, #24886, #15021, #21154, #22885, #8776, #16889, #15402, #7034, #17649, #9417, #1572, #7288, #3179, #11530, #15522, #3558, #23650, #25790, #9676, #21656, #9293, #7539, #11402 ),
 ( #23527, #17398, #11662, #19525, #5055, #25537, #1187, #3306, #1309, #25409, #21786, #5298, #1440, #13408, #25662, #1057, #13161, #21406, #11285, #13663, #21531, #19786, #15151, #13532, #17524, #23279, #7408, #21281, #5431, #3429 ),
 ( #3054, #19654, #17782, #11159, #9541, #15652, #23776, #5554, #19274, #9163, #5182, #13285, #17275, #7160, #23406, #15276, #19405, #8207, #10212, #26202, #24326, #22329, #5683, #11936, #11801, #4105, #12205, #5956, #19921, #16325 ) ),
 .UNSPECIFIED., .T., .F., .F. ) 
 B_SPLINE_SURFACE_WITH_KNOTS ( ( 4, 3, 4 ),
 ( 4, 2, 2, 2, 2, 2, 2, 2, 2, 2, 2, 2, 2, 2, 4 ),
 ( 0.000000000000000000, 0.5000000000000000000, 1.000000000000000000 ),
 ( 0.000000000000000000, 0.1357259735107005372, 0.1651108541090157700, 0.1944957347073310028, 0.3598804999793158710, 0.3867117631979620773, 0.4135430264166082281, 0.5789277916885930964, 0.6062785021374117456, 0.6336292125862302838, 0.8508620842112317728, 0.8814014469398914198, 0.9119408096685510667, 0.9559704048342755334, 1.000000000000000000 ),
 .UNSPECIFIED. ) 
 GEOMETRIC_REPRESENTATION_ITEM ( )  RATIONAL_B_SPLINE_SURFACE ( (
 ( 1.000000000000000000, 1.000000000000000000, 1.000000000000000000, 1.000000000000000000, 1.000000000000000000, 1.000000000000000000, 1.000000000000000000, 1.000000000000000000, 1.000000000000000000, 1.000000000000000000, 1.000000000000000000, 1.000000000000000000, 1.000000000000000000, 1.000000000000000000, 1.000000000000000000, 1.000000000000000000, 1.000000000000000000, 1.000000000000000000, 1.000000000000000000, 1.000000000000000000, 1.000000000000000000, 1.000000000000000000, 1.000000000000000000, 1.000000000000000000, 1.000000000000000000, 1.000000000000000000, 1.000000000000000000, 1.000000000000000000, 1.000000000000000000, 1.000000000000000000),
 ( 0.3333333333333333703, 0.3333333333333333703, 0.3333333333333333703, 0.3333333333333333703, 0.3333333333333333703, 0.3333333333333333703, 0.3333333333333333703, 0.3333333333333333703, 0.3333333333333333703, 0.3333333333333333703, 0.3333333333333333703, 0.3333333333333333703, 0.3333333333333333703, 0.3333333333333333703, 0.3333333333333333703, 0.3333333333333333703, 0.3333333333333333703, 0.3333333333333333703, 0.3333333333333333703, 0.3333333333333333703, 0.3333333333333333703, 0.3333333333333333703, 0.3333333333333333703, 0.3333333333333333703, 0.3333333333333333703, 0.3333333333333333703, 0.3333333333333333703, 0.3333333333333333703, 0.3333333333333333703, 0.3333333333333333703),
 ( 0.3333333333333333703, 0.3333333333333333703, 0.3333333333333333703, 0.3333333333333333703, 0.3333333333333333703, 0.3333333333333333703, 0.3333333333333333703, 0.3333333333333333703, 0.3333333333333333703, 0.3333333333333333703, 0.3333333333333333703, 0.3333333333333333703, 0.3333333333333333703, 0.3333333333333333703, 0.3333333333333333703, 0.3333333333333333703, 0.3333333333333333703, 0.3333333333333333703, 0.3333333333333333703, 0.3333333333333333703, 0.3333333333333333703, 0.3333333333333333703, 0.3333333333333333703, 0.3333333333333333703, 0.3333333333333333703, 0.3333333333333333703, 0.3333333333333333703, 0.3333333333333333703, 0.3333333333333333703, 0.3333333333333333703),
 ( 1.000000000000000000, 1.000000000000000000, 1.000000000000000000, 1.000000000000000000, 1.000000000000000000, 1.000000000000000000, 1.000000000000000000, 1.000000000000000000, 1.000000000000000000, 1.000000000000000000, 1.000000000000000000, 1.000000000000000000, 1.000000000000000000, 1.000000000000000000, 1.000000000000000000, 1.000000000000000000, 1.000000000000000000, 1.000000000000000000, 1.000000000000000000, 1.000000000000000000, 1.000000000000000000, 1.000000000000000000, 1.000000000000000000, 1.000000000000000000, 1.000000000000000000, 1.000000000000000000, 1.000000000000000000, 1.000000000000000000, 1.000000000000000000, 1.000000000000000000),
 ( 0.3333333333333333703, 0.3333333333333333703, 0.3333333333333333703, 0.3333333333333333703, 0.3333333333333333703, 0.3333333333333333703, 0.3333333333333333703, 0.3333333333333333703, 0.3333333333333333703, 0.3333333333333333703, 0.3333333333333333703, 0.3333333333333333703, 0.3333333333333333703, 0.3333333333333333703, 0.3333333333333333703, 0.3333333333333333703, 0.3333333333333333703, 0.3333333333333333703, 0.3333333333333333703, 0.3333333333333333703, 0.3333333333333333703, 0.3333333333333333703, 0.3333333333333333703, 0.3333333333333333703, 0.3333333333333333703, 0.3333333333333333703, 0.3333333333333333703, 0.3333333333333333703, 0.3333333333333333703, 0.3333333333333333703),
 ( 0.3333333333333333703, 0.3333333333333333703, 0.3333333333333333703, 0.3333333333333333703, 0.3333333333333333703, 0.3333333333333333703, 0.3333333333333333703, 0.3333333333333333703, 0.3333333333333333703, 0.3333333333333333703, 0.3333333333333333703, 0.3333333333333333703, 0.3333333333333333703, 0.3333333333333333703, 0.3333333333333333703, 0.3333333333333333703, 0.3333333333333333703, 0.3333333333333333703, 0.3333333333333333703, 0.3333333333333333703, 0.3333333333333333703, 0.3333333333333333703, 0.3333333333333333703, 0.3333333333333333703, 0.3333333333333333703, 0.3333333333333333703, 0.3333333333333333703, 0.3333333333333333703, 0.3333333333333333703, 0.3333333333333333703),
 ( 1.000000000000000000, 1.000000000000000000, 1.000000000000000000, 1.000000000000000000, 1.000000000000000000, 1.000000000000000000, 1.000000000000000000, 1.000000000000000000, 1.000000000000000000, 1.000000000000000000, 1.000000000000000000, 1.000000000000000000, 1.000000000000000000, 1.000000000000000000, 1.000000000000000000, 1.000000000000000000, 1.000000000000000000, 1.000000000000000000, 1.000000000000000000, 1.000000000000000000, 1.000000000000000000, 1.000000000000000000, 1.000000000000000000, 1.000000000000000000, 1.000000000000000000, 1.000000000000000000, 1.000000000000000000, 1.000000000000000000, 1.000000000000000000, 1.000000000000000000) ) ) 
 REPRESENTATION_ITEM ( '' )  SURFACE ( )  );
#22364=CARTESIAN_POINT ( 'NONE',  ( -192.9588430854690273, -40.00000000000024158, 54.46834944101708231 ) ) ;
#22365=CARTESIAN_POINT ( 'NONE',  ( -280.0000000000000568, 19.99999999999995737, 40.00000000000002132 ) ) ;
#22369=CARTESIAN_POINT ( 'NONE',  ( 163.1118516004056573, 1.251511021549353291E-13, -27.26290988616872824 ) ) ;
#22370=CARTESIAN_POINT ( 'NONE',  ( 184.8905102610680444, -3.509827109981123710E-14, 19.07866798485558490 ) ) ;
#22371=CARTESIAN_POINT ( 'NONE',  ( 192.4448373802101173, 40.00000000000012790, -20.00000000003928236 ) ) ;
#22373=CARTESIAN_POINT ( 'NONE',  ( -91.56559293963834989, -12.25131212657492874, 12.25131212657477953 ) ) ;
#22374=CARTESIAN_POINT ( 'NONE',  ( -213.1075012329537230, -13.71589010951915810, -40.00000000000002132 ) ) ;
#22375=CARTESIAN_POINT ( 'NONE',  ( -192.9588430854690273, -10.23066800229550388, 66.79921049721887982 ) ) ;
#22376=CARTESIAN_POINT ( 'NONE',  ( -89.92902785008669753, -8.734793929541526225, 20.17328762787284546 ) ) ;
#22377=CARTESIAN_POINT ( 'NONE',  ( 22.82385994800819162, -47.01156385802200788, 13.83113328680604681 ) ) ;
#22378=CARTESIAN_POINT ( 'NONE',  ( -56.48582580120560692, 39.99999999999991473, 9.153146818114004546 ) ) ;
#22379=CARTESIAN_POINT ( 'NONE',  ( -208.1127848780264742, 39.99999999999979394, 55.00245453010936103 ) ) ;
#22380=CARTESIAN_POINT ( 'NONE',  ( 136.1360204305621266, 3.511608612530704665, 3.511608612530695339 ) ) ;
#22381=CARTESIAN_POINT ( 'NONE',  ( -259.2033419157646676, 6.730120644403426944, 6.730120644403592145 ) ) ;
#22382=CARTESIAN_POINT ( 'NONE',  ( -189.5227851116908084, -18.00253723945785822, -43.46196956062684791 ) ) ;
#22383=CARTESIAN_POINT ( 'NONE',  ( -105.3755690713226585, -12.89780903124383471, -43.67073346367985920 ) ) ;
#22385=CARTESIAN_POINT ( 'NONE',  ( 192.4448373802101173, -42.42640687122053578, -14.14213562370360577 ) ) ;
#22387=CARTESIAN_POINT ( 'NONE',  ( 170.2234770963711128, 24.55285855007190321, 0.000000000000000000 ) ) ;
#22389=CARTESIAN_POINT ( 'NONE',  ( -30.26275506840324070, -27.08623969584554558, -29.48230279907826912 ) ) ;
#22390=CARTESIAN_POINT ( 'NONE',  ( -200.4318156386407850, -24.83634777282063766, -44.88237417767277293 ) ) ;
#22394=CARTESIAN_POINT ( 'NONE',  ( 22.26816181513970250, -23.58015273002475709, 43.18156009806490658 ) ) ;
#22395=CARTESIAN_POINT ( 'NONE',  ( -6.342283169556221623, 13.66521761902655818, 46.19215417243774624 ) ) ;
#22397=ORIENTED_EDGE ( 'NONE', *, *, #536, .F. ) ;
#22399=CARTESIAN_POINT ( 'NONE',  ( 151.7948205124836534, -33.23291073765550863, -40.00000000000002132 ) ) ;
#22403=CARTESIAN_POINT ( 'NONE',  ( 146.6084372240433709, 40.00000000000010658, -5.374981219216549810 ) ) ;
#22408=CARTESIAN_POINT ( 'NONE',  ( -114.4388184736404952, 8.352332320009658417, 20.16431396440389534 ) ) ;
#22409=CARTESIAN_POINT ( 'NONE',  ( -4.004886986945149552, -23.45685150724343160, -43.01537795656791019 ) ) ;
#22410=CARTESIAN_POINT ( 'NONE',  ( -198.0356074513804572, -67.44298959253333692, -10.87444709761016348 ) ) ;
#22412=CARTESIAN_POINT ( 'NONE',  ( -99.29480781227051978, 20.48155342677154067, -8.934325994365337920 ) ) ;
#22413=CARTESIAN_POINT ( 'NONE',  ( -30.26275506840322294, -57.76657404653985139, 1.198031551615709844 ) ) ;
#22414=CARTESIAN_POINT ( 'NONE',  ( 98.29820294267423719, -14.14213562374330024, 14.14213562372619926 ) ) ;
#22415=CARTESIAN_POINT ( 'NONE',  ( 136.1360204305621266, 24.77266263493104148, 24.77266263493145004 ) ) ;
#22416=CARTESIAN_POINT ( 'NONE',  ( -105.3755690713226585, -18.24025645688355013, 40.00000000000002132 ) ) ;
#22418=CARTESIAN_POINT ( 'NONE',  ( -30.26275506840323004, -41.69427246844629309, 40.00000000000002132 ) ) ;
#22419=CARTESIAN_POINT ( 'NONE',  ( -105.2331094975916130, 16.94275695785337277, 13.19829893673040644 ) ) ;
#22420=CARTESIAN_POINT ( 'NONE',  ( 200.0000000000000000, 39.99999999999985079, 20.00000000000052225 ) ) ;
#22421=CARTESIAN_POINT ( 'NONE',  ( 0.2972598230769886718, 38.42060263243669027, -18.14793986248710667 ) ) ;
#22422=CARTESIAN_POINT ( 'NONE',  ( -213.1075012329537230, 13.71589010951907817, -40.00000000000002132 ) ) ;
#22424=EDGE_CURVE ( 'NONE', #13885, #17229, #18784, .T. ) ;
#22426=CARTESIAN_POINT ( 'NONE',  ( 4.995406935893288214, 15.24977328854832770, 0.000000000000000000 ) ) ;
#22427=CARTESIAN_POINT ( 'NONE',  ( -103.9474983245023481, -8.027156558344637816, -20.15710290851495756 ) ) ;
#22428=CARTESIAN_POINT ( 'NONE',  ( 57.59792236341147031, 39.99999999999990763, 37.56421063658199699 ) ) ;
#22429=CARTESIAN_POINT ( 'NONE',  ( -238.4067589809705794, 28.96627169325354956, -28.96627169325289231 ) ) ;
#22431=CARTESIAN_POINT ( 'NONE',  ( -192.1167141818822017, -43.95739236919489912, -24.15421809699812172 ) ) ;
#22435=CARTESIAN_POINT ( 'NONE',  ( -162.0762913951020892, 29.48230308784799902, -29.48230308784730980 ) ) ;
#22436=CARTESIAN_POINT ( 'NONE',  ( 170.2234770963711128, -10.92277846919187034, -10.92277846919209594 ) ) ;
#22437=DIRECTION ( 'NONE',  ( 0.9698969544411725208, -0.09318942517750300469, -0.2249791741491306285 ) ) ;
#22438=CARTESIAN_POINT ( 'NONE',  ( 146.6084372240433993, -3.357462877844280890E-13, 34.62501878078305850 ) ) ;
#22439=CARTESIAN_POINT ( 'NONE',  ( -280.0000000000000568, -42.42640687119305198, 14.14213562373058686 ) ) ;
#22441=CARTESIAN_POINT ( 'NONE',  ( 57.59792236341147031, -1.722363176415032004, -1.722363176415048880 ) ) ;
#22442=CARTESIAN_POINT ( 'NONE',  ( 0.2972598230770027716, -38.42060263243656237, -18.14793986248737667 ) ) ;
#22443=DIRECTION ( 'NONE',  ( 1.000000000000000000, 1.836970198721030181E-16, 0.000000000000000000 ) ) ;
#22445=CARTESIAN_POINT ( 'NONE',  ( 57.59792236341147742, -1.230234673553095937E-13, 37.56421063658186199 ) ) ;
#22447=CARTESIAN_POINT ( 'NONE',  ( 23.35901252181229637, 46.81387818480130392, -13.80180065670237788 ) ) ;
#22448=CARTESIAN_POINT ( 'NONE',  ( -259.2033419157646676, -9.517827891722680178, -40.00000000000002132 ) ) ;
#22449=ORIENTED_EDGE ( 'NONE', *, *, #22352, .T. ) ;
#22450=CARTESIAN_POINT ( 'NONE',  ( 21.16156876808018339, -23.80729322913531121, -43.48822901267205054 ) ) ;
#22451=CARTESIAN_POINT ( 'NONE',  ( -4.260882601032360384, -42.93997571557835613, 23.40615483283719556 ) ) ;
#22453=CARTESIAN_POINT ( 'NONE',  ( -105.3755690713226727, 18.24025645688350750, 2.449293598294708485E-15 ) ) ;
#22455=CARTESIAN_POINT ( 'NONE',  ( -192.1131556193065819, -48.19965519933759168, -14.00853984552894360 ) ) ;
#22456=CARTESIAN_POINT ( 'NONE',  ( 163.1118516004056573, -19.27778845538761132, -19.27778845538770724 ) ) ;
#22457=CARTESIAN_POINT ( 'NONE',  ( 22.01478053666890133, -13.87318432395561807, 47.29427690643639437 ) ) ;
#22458=CARTESIAN_POINT ( 'NONE',  ( -1.624577210452443854, 18.12534649864440084, -43.75845733971287643 ) ) ;
#22462=CARTESIAN_POINT ( 'NONE',  ( -166.7090905288631291, -15.35183918172718442, 37.06261835973858609 ) ) ;
#22463=CARTESIAN_POINT ( 'NONE',  ( -198.0356074513804572, 10.87444709761036066, -67.44298959253325165 ) ) ;
#22464=CARTESIAN_POINT ( 'NONE',  ( -86.95492400940779021, -6.698385205267455511, 20.33918296375446744 ) ) ;
#22465=( BOUNDED_CURVE ( )  B_SPLINE_CURVE ( 3, ( #14291, #10310, #21221, #23469 ),
 .UNSPECIFIED., .F., .F. ) 
 B_SPLINE_CURVE_WITH_KNOTS ( ( 4, 4 ),
 ( 0.004183487405659318259, 0.01388163286937179816 ),
 .UNSPECIFIED. ) 
 CURVE ( )  GEOMETRIC_REPRESENTATION_ITEM ( )  RATIONAL_B_SPLINE_CURVE ( ( 0.6809743333591583569, 0.7608653435686173472, 0.8672072324488978579, 1.000000000000000000 ) ) 
 REPRESENTATION_ITEM ( '' )  );
#22466=CARTESIAN_POINT ( 'NONE',  ( -190.5535808404945044, 18.10342626500584728, -43.70553721440292350 ) ) ;
#22467=CARTESIAN_POINT ( 'NONE',  ( 130.8568914410475088, 4.207082182989012153, 52.36146031193425188 ) ) ;
#22468=CARTESIAN_POINT ( 'NONE',  ( -86.96347745069644475, -15.38646221621807442, 15.38646221621768184 ) ) ;
#22469=CARTESIAN_POINT ( 'NONE',  ( 57.59792236341148453, -37.56421063658185489, -2.449293598294708485E-15 ) ) ;
#22470=CARTESIAN_POINT ( 'NONE',  ( -192.9588430854690273, 54.46834944098218756, -40.00000000000002132 ) ) ;
#22471=CARTESIAN_POINT ( 'NONE',  ( -238.4067589809705794, -3.369206980223063916E-14, -0.9644942799825824142 ) ) ;
#22472=CARTESIAN_POINT ( 'NONE',  ( 146.6084372240433709, -24.48358557860329299, 32.08495691632052882 ) ) ;
#22474=CARTESIAN_POINT ( 'NONE',  ( -86.96347745069644475, -12.89780903124395195, -12.89780903124416511 ) ) ;
#22476=CARTESIAN_POINT ( 'NONE',  ( -208.1127848780265026, 10.60833733269537049, 10.60833733269544510 ) ) ;
#22477=CARTESIAN_POINT ( 'NONE',  ( -99.31364972219382992, 8.164808577079744722, 20.79869444143179891 ) ) ;
#22478=VERTEX_POINT ( 'NONE', #1096 ) ;
#22479=CARTESIAN_POINT ( 'NONE',  ( 4.995406935893310418, -67.35176059880237176, 10.78321810387813429 ) ) ;
#22480=CARTESIAN_POINT ( 'NONE',  ( 2.692156443669315724, -44.48799183653559197, -18.42752958144988895 ) ) ;
#22482=CARTESIAN_POINT ( 'NONE',  ( -96.93773665438737908, -20.92028269119444062, 8.190703376740682273 ) ) ;
#22488=CARTESIAN_POINT ( 'NONE',  ( 151.7948205124836250, -23.49921654116339553, -23.49921654116350211 ) ) ;
#22489=CARTESIAN_POINT ( 'NONE',  ( -166.3490736461147605, -36.43932733827825388, -19.13702016920204230 ) ) ;
#22490=ADVANCED_FACE ( 'NONE', ( #25449 ), #9756, .T. ) ;
#22491=CARTESIAN_POINT ( 'NONE',  ( -100.7734535825088500, -40.00000000000009948, 17.32597176626796909 ) ) ;
#22492=CARTESIAN_POINT ( 'NONE',  ( 170.2234770963711128, -24.55285855007184281, 40.00000000000002132 ) ) ;
#22495=EDGE_CURVE ( 'NONE', #14842, #18547, #12472, .T. ) ;
#22496=CARTESIAN_POINT ( 'NONE',  ( 184.8905102610680444, -39.99999999999991473, -20.92133201514458207 ) ) ;
#22497=CARTESIAN_POINT ( 'NONE',  ( -135.8532207217289738, -1.351063376314938213E-13, 30.84685318188645553 ) ) ;
#22498=CARTESIAN_POINT ( 'NONE',  ( -213.1075012329537230, 39.99999999999992895, 13.71589010951925935 ) ) ;
#22499=CARTESIAN_POINT ( 'NONE',  ( -135.8532207217289738, 9.153146818113548022, -40.00000000000002132 ) ) ;
#22500=CARTESIAN_POINT ( 'NONE',  ( 146.6084372240433993, -3.800685668858652999, 3.800685668858636568 ) ) ;
#22502=CARTESIAN_POINT ( 'NONE',  ( 19.06497207195982924, -54.19242893257843008, -2.449293598294708485E-15 ) ) ;
#22503=EDGE_CURVE ( 'NONE', #3292, #6406, #7032, .T. ) ;
#22504=CARTESIAN_POINT ( 'NONE',  ( -280.0000000000000568, 42.42640687119274645, 14.14213562373118194 ) ) ;
#22505=CARTESIAN_POINT ( 'NONE',  ( -175.9234132812216842, 12.95567001274190133, 42.70618379781711837 ) ) ;
#22507=CARTESIAN_POINT ( 'NONE',  ( 163.1118516004056573, 39.99999999999976552, 27.26290988616914746 ) ) ;
#22508=CARTESIAN_POINT ( 'NONE',  ( 130.8568914410475088, -40.00000000000001421, 5.949712681206549725 ) ) ;
#22509=CARTESIAN_POINT ( 'NONE',  ( -100.7734535825088500, 40.53558337403677569, -16.03295912088699993 ) ) ;
#22510=CARTESIAN_POINT ( 'NONE',  ( 85.88436334084022405, -10.32541289738165524, 22.72801779375535958 ) ) ;
#22512=CARTESIAN_POINT ( 'NONE',  ( -192.9588430854690273, -66.79921049724377724, 10.23066800231950069 ) ) ;
#22514=CARTESIAN_POINT ( 'NONE',  ( -30.26275506840324070, 1.198031551616030033, -1.198031551616006496 ) ) ;
#22516=CARTESIAN_POINT ( 'NONE',  ( 91.82158438592156813, 17.20528682183302038, -40.00000000000002132 ) ) ;
#22520=ORIENTED_EDGE ( 'NONE', *, *, #543, .T. ) ;
#22523=CARTESIAN_POINT ( 'NONE',  ( 23.37583784646054141, 23.33923448557714053, 42.85659535397683584 ) ) ;
#22526=( BOUNDED_SURFACE ( )  B_SPLINE_SURFACE ( 3, 3, ( 
 ( #16126, #26273, #9616, #20130, #25861, #26130, #1909, #26001, #15849, #8147, #23979, #17982, #21997, #3631, #11871, #11600, #19857, #3910, #9881, #1776, #3767, #19991, #7871, #10013, #1643, #9751, #4042, #2044, #15993, #35 ),
 ( #5892, #7606, #15721, #14000, #18121, #8011, #24256, #6029, #1509, #14136, #22267, #23846, #24390, #12141, #20265, #10151, #5625, #18254, #16261, #13731, #13596, #21857, #3502, #6157, #16662, #24528, #22532, #22664, #18525, #4436 ),
 ( #307, #14794, #20799, #2711, #20663, #577, #18391, #8546, #4573, #22925, #2571, #4179, #2298, #14266, #16531, #4313, #24929, #24794, #10545, #12670, #20528, #10816, #18656, #22403, #8684, #18796, #2175, #10685, #10282, #443 ),
 ( #12273, #6546, #20401, #14655, #12530, #2433, #12810, #16792, #22796, #24659, #6679, #16399, #4706, #14402, #20932, #168, #18929, #711, #8815, #16926, #8274, #6284, #12403, #10408, #6416, #8409, #14533, #19309, #25445, #23187 ),
 ( #3093, #7197, #972, #10952, #15434, #4967, #25317, #12942, #9326, #11439, #23064, #2844, #13445, #1353, #17313, #5214, #13076, #11074, #23318, #15312, #19058, #21565, #23438, #21191, #19188, #7320, #13318, #3338, #13198, #19435 ),
 ( #9076, #1222, #23561, #25574, #2963, #17182, #5093, #11195, #17437, #11319, #25060, #15190, #21057, #7076, #840, #21438, #19561, #5336, #9452, #6812, #14928, #1092, #4836, #8950, #21320, #9201, #3212, #17059, #25192, #6940 ),
 ( #15058, #10340, #12459, #6216, #18449, #7446, #21693, #3469, #4369, #8340, #23811, #16190, #14328, #226, #5593, #9713, #11568, #19686, #12203, #18315, #15686, #16323, #11701, #23685, #98, #21824, #1475, #2361, #13699, #25965 ) ),
 .UNSPECIFIED., .T., .F., .F. ) 
 B_SPLINE_SURFACE_WITH_KNOTS ( ( 4, 3, 4 ),
 ( 4, 2, 2, 2, 2, 2, 2, 2, 2, 2, 2, 2, 2, 2, 4 ),
 ( 0.000000000000000000, 0.5000000000000000000, 1.000000000000000000 ),
 ( 0.000000000000000000, 0.1357259735107005372, 0.1651108541090157700, 0.1944957347073310028, 0.3598804999793158710, 0.3867117631979620773, 0.4135430264166082281, 0.5789277916885930964, 0.6062785021374117456, 0.6336292125862302838, 0.8508620842112317728, 0.8814014469398914198, 0.9119408096685510667, 0.9559704048342755334, 1.000000000000000000 ),
 .UNSPECIFIED. ) 
 GEOMETRIC_REPRESENTATION_ITEM ( )  RATIONAL_B_SPLINE_SURFACE ( (
 ( 1.000000000000000000, 1.000000000000000000, 1.000000000000000000, 1.000000000000000000, 1.000000000000000000, 1.000000000000000000, 1.000000000000000000, 1.000000000000000000, 1.000000000000000000, 1.000000000000000000, 1.000000000000000000, 1.000000000000000000, 1.000000000000000000, 1.000000000000000000, 1.000000000000000000, 1.000000000000000000, 1.000000000000000000, 1.000000000000000000, 1.000000000000000000, 1.000000000000000000, 1.000000000000000000, 1.000000000000000000, 1.000000000000000000, 1.000000000000000000, 1.000000000000000000, 1.000000000000000000, 1.000000000000000000, 1.000000000000000000, 1.000000000000000000, 1.000000000000000000),
 ( 0.3333333333333333703, 0.3333333333333333703, 0.3333333333333333703, 0.3333333333333333703, 0.3333333333333333703, 0.3333333333333333703, 0.3333333333333333703, 0.3333333333333333703, 0.3333333333333333703, 0.3333333333333333703, 0.3333333333333333703, 0.3333333333333333703, 0.3333333333333333703, 0.3333333333333333703, 0.3333333333333333703, 0.3333333333333333703, 0.3333333333333333703, 0.3333333333333333703, 0.3333333333333333703, 0.3333333333333333703, 0.3333333333333333703, 0.3333333333333333703, 0.3333333333333333703, 0.3333333333333333703, 0.3333333333333333703, 0.3333333333333333703, 0.3333333333333333703, 0.3333333333333333703, 0.3333333333333333703, 0.3333333333333333703),
 ( 0.3333333333333333703, 0.3333333333333333703, 0.3333333333333333703, 0.3333333333333333703, 0.3333333333333333703, 0.3333333333333333703, 0.3333333333333333703, 0.3333333333333333703, 0.3333333333333333703, 0.3333333333333333703, 0.3333333333333333703, 0.3333333333333333703, 0.3333333333333333703, 0.3333333333333333703, 0.3333333333333333703, 0.3333333333333333703, 0.3333333333333333703, 0.3333333333333333703, 0.3333333333333333703, 0.3333333333333333703, 0.3333333333333333703, 0.3333333333333333703, 0.3333333333333333703, 0.3333333333333333703, 0.3333333333333333703, 0.3333333333333333703, 0.3333333333333333703, 0.3333333333333333703, 0.3333333333333333703, 0.3333333333333333703),
 ( 1.000000000000000000, 1.000000000000000000, 1.000000000000000000, 1.000000000000000000, 1.000000000000000000, 1.000000000000000000, 1.000000000000000000, 1.000000000000000000, 1.000000000000000000, 1.000000000000000000, 1.000000000000000000, 1.000000000000000000, 1.000000000000000000, 1.000000000000000000, 1.000000000000000000, 1.000000000000000000, 1.000000000000000000, 1.000000000000000000, 1.000000000000000000, 1.000000000000000000, 1.000000000000000000, 1.000000000000000000, 1.000000000000000000, 1.000000000000000000, 1.000000000000000000, 1.000000000000000000, 1.000000000000000000, 1.000000000000000000, 1.000000000000000000, 1.000000000000000000),
 ( 0.3333333333333333703, 0.3333333333333333703, 0.3333333333333333703, 0.3333333333333333703, 0.3333333333333333703, 0.3333333333333333703, 0.3333333333333333703, 0.3333333333333333703, 0.3333333333333333703, 0.3333333333333333703, 0.3333333333333333703, 0.3333333333333333703, 0.3333333333333333703, 0.3333333333333333703, 0.3333333333333333703, 0.3333333333333333703, 0.3333333333333333703, 0.3333333333333333703, 0.3333333333333333703, 0.3333333333333333703, 0.3333333333333333703, 0.3333333333333333703, 0.3333333333333333703, 0.3333333333333333703, 0.3333333333333333703, 0.3333333333333333703, 0.3333333333333333703, 0.3333333333333333703, 0.3333333333333333703, 0.3333333333333333703),
 ( 0.3333333333333333703, 0.3333333333333333703, 0.3333333333333333703, 0.3333333333333333703, 0.3333333333333333703, 0.3333333333333333703, 0.3333333333333333703, 0.3333333333333333703, 0.3333333333333333703, 0.3333333333333333703, 0.3333333333333333703, 0.3333333333333333703, 0.3333333333333333703, 0.3333333333333333703, 0.3333333333333333703, 0.3333333333333333703, 0.3333333333333333703, 0.3333333333333333703, 0.3333333333333333703, 0.3333333333333333703, 0.3333333333333333703, 0.3333333333333333703, 0.3333333333333333703, 0.3333333333333333703, 0.3333333333333333703, 0.3333333333333333703, 0.3333333333333333703, 0.3333333333333333703, 0.3333333333333333703, 0.3333333333333333703),
 ( 1.000000000000000000, 1.000000000000000000, 1.000000000000000000, 1.000000000000000000, 1.000000000000000000, 1.000000000000000000, 1.000000000000000000, 1.000000000000000000, 1.000000000000000000, 1.000000000000000000, 1.000000000000000000, 1.000000000000000000, 1.000000000000000000, 1.000000000000000000, 1.000000000000000000, 1.000000000000000000, 1.000000000000000000, 1.000000000000000000, 1.000000000000000000, 1.000000000000000000, 1.000000000000000000, 1.000000000000000000, 1.000000000000000000, 1.000000000000000000, 1.000000000000000000, 1.000000000000000000, 1.000000000000000000, 1.000000000000000000, 1.000000000000000000, 1.000000000000000000) ) ) 
 REPRESENTATION_ITEM ( '' )  SURFACE ( )  );
#22527=CARTESIAN_POINT ( 'NONE',  ( -259.2033419157646676, -9.517827891722680178, 0.000000000000000000 ) ) ;
#22529=CARTESIAN_POINT ( 'NONE',  ( -199.9999999999999716, -44.86878812508714276, 24.82633483071253622 ) ) ;
#22530=CARTESIAN_POINT ( 'NONE',  ( -97.73860346099715457, -8.185503821079883835, -20.89580782303697859 ) ) ;
#22532=CARTESIAN_POINT ( 'NONE',  ( 170.2234770963711128, 39.99999999999980105, 24.55285855007229401 ) ) ;
#22533=CARTESIAN_POINT ( 'NONE',  ( 170.2234770963711128, -2.259079968736224833E-13, 24.55285855007187124 ) ) ;
#22537=CARTESIAN_POINT ( 'NONE',  ( -184.9729924864046779, 22.80024897326492450, 42.02333070177070340 ) ) ;
#22538=CARTESIAN_POINT ( 'NONE',  ( 17.65190074000382126, -24.35922420887711226, -44.23515346911565871 ) ) ;
#22539=CARTESIAN_POINT ( 'NONE',  ( 4.995406935893312195, -67.35176059882525124, -10.78321810390210445 ) ) ;
#22540=CARTESIAN_POINT ( 'NONE',  ( -200.0000000000000284, 20.93268228684348387, 45.36622447512526435 ) ) ;
#22541=CARTESIAN_POINT ( 'NONE',  ( -213.1075012329537230, 18.58567234101121102, 37.98287015391247223 ) ) ;
#22543=CARTESIAN_POINT ( 'NONE',  ( 184.8905102610680444, 14.79361573936375507, 14.79361573936398067 ) ) ;
#22544=CARTESIAN_POINT ( 'NONE',  ( -100.7734535825088500, 22.67402823373189946, 40.00000000000002132 ) ) ;
#22545=CARTESIAN_POINT ( 'NONE',  ( -162.0762913951020892, 1.198031840385732849, -1.198031840385733515 ) ) ;
#22546=CARTESIAN_POINT ( 'NONE',  ( -162.0762913951020607, -41.69427287682838568, -2.449293598294708485E-15 ) ) ;
#22547=CARTESIAN_POINT ( 'NONE',  ( -99.29480781227073294, 20.80016781325170427, -8.165122821357643446 ) ) ;
#22548=CARTESIAN_POINT ( 'NONE',  ( 14.38125909742180220, 40.00000000000017764, -15.17850393972591760 ) ) ;
#22549=CARTESIAN_POINT ( 'NONE',  ( 192.4448373802101173, 14.14213562370320076, -42.42640687122072762 ) ) ;
#22550=CARTESIAN_POINT ( 'NONE',  ( -100.7734535825088358, -22.67402823373193499, 0.000000000000000000 ) ) ;
#22554=VERTEX_POINT ( 'NONE', #1844 ) ;
#22555=CARTESIAN_POINT ( 'NONE',  ( 146.6084372240433993, -34.62501878078303008, 0.000000000000000000 ) ) ;
#22556=CARTESIAN_POINT ( 'NONE',  ( 158.3379117892987722, 10.98149362779600935, 26.51167085133962686 ) ) ;
#22557=CARTESIAN_POINT ( 'NONE',  ( -30.26275506840325136, 57.76657404653985139, -1.198031551615314161 ) ) ;
#22558=CARTESIAN_POINT ( 'NONE',  ( -114.4940140763995373, -20.58897208713957738, -7.440456728211662707 ) ) ;
#22559=CARTESIAN_POINT ( 'NONE',  ( 199.9999999999999432, -20.00000000000006750, 0.000000000000000000 ) ) ;
#22560=LINE ( 'NONE', #24687, #1171 ) ;
#22563=CARTESIAN_POINT ( 'NONE',  ( 192.4448373802101173, -14.14213562375826605, -42.42640687116518450 ) ) ;
#22564=CARTESIAN_POINT ( 'NONE',  ( -259.2033419157646676, -49.83842185052040463, 6.730120644403092101 ) ) ;
#22566=CARTESIAN_POINT ( 'NONE',  ( 57.59792236341147031, 40.00000000000042633, -37.56421063658144277 ) ) ;
#22567=CARTESIAN_POINT ( 'NONE',  ( -192.9588430854690273, -38.51493924976957572, 18.05360324515410397 ) ) ;
#22569=CARTESIAN_POINT ( 'NONE',  ( -16.41532015099270225, 12.95569205221179487, 42.70629200725615959 ) ) ;
#22570=CARTESIAN_POINT ( 'NONE',  ( -162.0762913951020892, 1.198031840385716418, 1.198031840385750169 ) ) ;
#22571=CARTESIAN_POINT ( 'NONE',  ( -100.7734535825088500, -40.53558337403669753, -16.03295912088728770 ) ) ;
#22574=CARTESIAN_POINT ( 'NONE',  ( 57.59792236341147031, 39.99999999999990763, 37.56421063658199699 ) ) ;
#22576=CARTESIAN_POINT ( 'NONE',  ( 25.62979979003352682, 42.16299361907574905, -22.88075396656789806 ) ) ;
#22577=CARTESIAN_POINT ( 'NONE',  ( 130.8568914410475372, 5.949712681206715814, 2.449293598294708485E-15 ) ) ;
#22578=CARTESIAN_POINT ( 'NONE',  ( 19.06497207195981503, -14.19242893257840166, 0.000000000000000000 ) ) ;
#22579=CARTESIAN_POINT ( 'NONE',  ( 151.7948205124836250, -23.49921654116339553, -23.49921654116350211 ) ) ;
#22580=CARTESIAN_POINT ( 'NONE',  ( -5.152948516943141044, -46.60473671797108608, 13.74948675458158753 ) ) ;
#22582=CARTESIAN_POINT ( 'NONE',  ( -105.3755690713226585, 18.24025645688349684, 40.00000000000002132 ) ) ;
#22584=ORIENTED_EDGE ( 'NONE', *, *, #24446, .F. ) ;
#22585=CARTESIAN_POINT ( 'NONE',  ( 4.990269915386266852, 24.74342916192447817, -44.75621547178034376 ) ) ;
#22587=CARTESIAN_POINT ( 'NONE',  ( -135.8532207217289738, -6.472252184284190690, -6.472252184284188914 ) ) ;
#22590=CARTESIAN_POINT ( 'NONE',  ( -3.434479974377871780, 17.93814274724503122, -43.30650750418230643 ) ) ;
#22592=CARTESIAN_POINT ( 'NONE',  ( -65.65510974524528365, -24.89665924127696783, -9.107311025939324622 ) ) ;
#22593=CARTESIAN_POINT ( 'NONE',  ( 159.7744820660626885, -25.95909830917692673, 10.75261058663734026 ) ) ;
#22594=CARTESIAN_POINT ( 'NONE',  ( -189.2667921706068626, -17.97629039507247484, 43.39860407294408873 ) ) ;
#22595=CARTESIAN_POINT ( 'NONE',  ( -213.1075012329537230, 9.698598906450543566, -9.698598906450348167 ) ) ;
#22596=CARTESIAN_POINT ( 'NONE',  ( 170.0000000000000000, 24.25569233607184216, 6.285860131565298659 ) ) ;
#22598=CARTESIAN_POINT ( 'NONE',  ( -195.1685814578629561, 14.09692187699488031, -48.78510996054859561 ) ) ;
#22599=CARTESIAN_POINT ( 'NONE',  ( 146.6084372240433709, 3.800685668858042821, 52.76785682606522698 ) ) ;
#22600=CARTESIAN_POINT ( 'NONE',  ( 14.38125909742180752, 10.73282306404735387, -10.73282306404708919 ) ) ;
#22601=CARTESIAN_POINT ( 'NONE',  ( 4.995406935893309530, -55.24977328856464709, 40.00000000000002132 ) ) ;
#22602=CARTESIAN_POINT ( 'NONE',  ( 136.1360204305621551, 4.966164525587085876, 40.00000000000002132 ) ) ;
#22603=CARTESIAN_POINT ( 'NONE',  ( -192.9588430854690273, -39.99999999999991473, -14.46834944100011633 ) ) ;
#22604=CARTESIAN_POINT ( 'NONE',  ( -56.48582580120559271, 21.81201906317768291, 21.81201906317777173 ) ) ;
#22605=CARTESIAN_POINT ( 'NONE',  ( -162.0762913951020892, -29.48230308784744125, -29.48230308784792442 ) ) ;
#22609=CARTESIAN_POINT ( 'NONE',  ( -238.4067589809705794, 0.6820004457912757223, 0.6820004457913219076 ) ) ;
#22610=CARTESIAN_POINT ( 'NONE',  ( -189.4799804244526626, -13.88847367996405069, -47.39666776706570062 ) ) ;
#22612=CARTESIAN_POINT ( 'NONE',  ( -238.4067589809705794, -0.6820004458488042598, 57.25054294077229855 ) ) ;
#22613=CARTESIAN_POINT ( 'NONE',  ( -3.117754532602394324, -43.38723640139033222, -17.97158175134525493 ) ) ;
#22614=ORIENTED_EDGE ( 'NONE', *, *, #25555, .F. ) ;
#22615=CARTESIAN_POINT ( 'NONE',  ( -93.02511667906844650, -20.82219708225688493, 8.169918093965387484 ) ) ;
#22616=CARTESIAN_POINT ( 'NONE',  ( -87.02160135033209087, -10.86113943608616239, -18.50856326151600939 ) ) ;
#22617=VERTEX_POINT ( 'NONE', #20196 ) ;
#22621=CARTESIAN_POINT ( 'NONE',  ( -190.7346372394394791, -47.78727444206358399, -13.94676542151541021 ) ) ;
#22622=CARTESIAN_POINT ( 'NONE',  ( 163.1118516004056573, -39.99999999999990052, -27.26290988616886679 ) ) ;
#22623=CARTESIAN_POINT ( 'NONE',  ( 146.6084372240433709, 5.374981219216996564, 40.00000000000002132 ) ) ;
#22626=CARTESIAN_POINT ( 'NONE',  ( -56.48582580120558561, -1.205267837095813407E-13, 30.84685318188644132 ) ) ;
#22627=CARTESIAN_POINT ( 'NONE',  ( 151.7948205124836534, 40.00000000000002842, 6.767089262349174739 ) ) ;
#22629=CARTESIAN_POINT ( 'NONE',  ( -259.2033419157646676, 9.517827891722584255, -0.000000000000000000 ) ) ;
#22630=CARTESIAN_POINT ( 'NONE',  ( 130.8568914410475088, -5.949712681206664300, -40.00000000000002132 ) ) ;
#22631=CARTESIAN_POINT ( 'NONE',  ( -208.1127848780264742, 17.67593391476624021, 38.89260858015742883 ) ) ;
#22632=CARTESIAN_POINT ( 'NONE',  ( -208.1127848780265026, 1.189126717069624012E-13, -15.00245453012669472 ) ) ;
#22634=CARTESIAN_POINT ( 'NONE',  ( -208.1127848780264742, 40.00000000000055422, -55.00245453014380814 ) ) ;
#22635=CARTESIAN_POINT ( 'NONE',  ( -198.0356074513804572, -2.321818583541004323E-13, 55.37879056873073580 ) ) ;
#22637=CARTESIAN_POINT ( 'NONE',  ( -138.9613193425335282, -29.42718875726419014, -10.11110876495210675 ) ) ;
#22639=CARTESIAN_POINT ( 'NONE',  ( -100.7734535825088500, -40.53558337403669753, -16.03295912088728770 ) ) ;
#22640=ORIENTED_EDGE ( 'NONE', *, *, #18344, .T. ) ;
#22641=CARTESIAN_POINT ( 'NONE',  ( 163.1118516004056573, -19.27778845538787422, 19.27778845538743724 ) ) ;
#22643=CARTESIAN_POINT ( 'NONE',  ( -259.2033419157646676, -30.48217210827744239, -2.449293598294708485E-15 ) ) ;
#22645=CARTESIAN_POINT ( 'NONE',  ( -114.5523123854248553, 19.58652998792704736, -9.959192389756811536 ) ) ;
#22646=CARTESIAN_POINT ( 'NONE',  ( -198.0356074513804572, 15.37879056873067007, 0.000000000000000000 ) ) ;
#22648=EDGE_LOOP ( 'NONE', ( #15711, #3325, #4858, #23926, #1859, #1722, #19979, #3821, #13939 ) ) ;
#22650=CARTESIAN_POINT ( 'NONE',  ( -88.37877758184959021, 8.575405934490602178, -19.92653024479352908 ) ) ;
#22651=CARTESIAN_POINT ( 'NONE',  ( 11.38508063393684466, 24.83994849155569540, 44.88728980639523769 ) ) ;
#22652=ADVANCED_FACE ( 'NONE', ( #8078 ), #18787, .T. ) ;
#22653=VERTEX_POINT ( 'NONE', #8449 ) ;
#22654=VERTEX_POINT ( 'NONE', #345 ) ;
#22655=CARTESIAN_POINT ( 'NONE',  ( -192.9588430854690273, -18.05360324515454096, 38.51493924976936967 ) ) ;
#22659=EDGE_CURVE ( 'NONE', #4726, #8524, #7355, .T. ) ;
#22660=CARTESIAN_POINT ( 'NONE',  ( -192.9588430854689989, 10.23066800230742679, 10.23066800230749607 ) ) ;
#22661=CARTESIAN_POINT ( 'NONE',  ( -208.1127848780264742, 38.89260858015732936, -17.67593391476642140 ) ) ;
#22662=CARTESIAN_POINT ( 'NONE',  ( -199.9999999999997726, -24.82633483071077762, 44.86878812508861358 ) ) ;
#22664=CARTESIAN_POINT ( 'NONE',  ( 184.8905102610680444, 39.99999999999983658, 20.92133201514485563 ) ) ;
#22665=CARTESIAN_POINT ( 'NONE',  ( -162.0762913951020892, -1.202636532414034422E-14, -1.694272876828323948 ) ) ;
#22669=CARTESIAN_POINT ( 'NONE',  ( -187.8778500559390636, 17.82355023088775070, 43.02985669704477090 ) ) ;
#22670=CARTESIAN_POINT ( 'NONE',  ( 0.2972598230769976091, -10.13633138497465147, -10.13633138497482733 ) ) ;
#22671=CARTESIAN_POINT ( 'NONE',  ( -105.4741150117365009, 19.60045294981777531, -8.366608964619008049 ) ) ;
#22672=CARTESIAN_POINT ( 'NONE',  ( 130.8568914410475088, 24.07718906446891793, 32.49135343045489321 ) ) ;
#22674=CARTESIAN_POINT ( 'NONE',  ( -238.4067589809705794, -28.96627169325303797, -28.96627169325349627 ) ) ;
#22676=CARTESIAN_POINT ( 'NONE',  ( -86.96347745069645896, 21.75974354311648895, -0.000000000000000000 ) ) ;
#22677=PLANE ( 'NONE',  #13417 ) ;
#22678=CARTESIAN_POINT ( 'NONE',  ( -105.3755690713226869, 21.75974354311648540, -0.000000000000000000 ) ) ;
#22680=CARTESIAN_POINT ( 'NONE',  ( 170.2234770963711128, 40.00000000000021316, -15.44714144992773797 ) ) ;
#22682=CARTESIAN_POINT ( 'NONE',  ( 155.1206158682454657, -11.51471166709265503, 27.79897307351014746 ) ) ;
#22683=ORIENTED_EDGE ( 'NONE', *, *, #7052, .F. ) ;
#22685=CARTESIAN_POINT ( 'NONE',  ( 184.8905102610680444, -20.92133201514440799, 0.000000000000000000 ) ) ;
#22686=ADVANCED_FACE ( 'NONE', ( #24698 ), #13864, .T. ) ;
#22687=CARTESIAN_POINT ( 'NONE',  ( 164.1122551457367251, 10.10009781492405523, 24.38379312608499561 ) ) ;
#22688=CARTESIAN_POINT ( 'NONE',  ( 0.2972598230769959993, 38.42060263243713081, -38.42060263243619289 ) ) ;
#22689=CARTESIAN_POINT ( 'NONE',  ( -114.7538884075660235, -21.97380054625780232, -2.777513412063746578 ) ) ;
#22690=CARTESIAN_POINT ( 'NONE',  ( -193.0908841288064934, -44.14257353178373222, -24.29092413197459521 ) ) ;
#22691=CARTESIAN_POINT ( 'NONE',  ( -114.4364955367322949, 8.644468109217019247, 20.04994829327305794 ) ) ;
#22693=CARTESIAN_POINT ( 'NONE',  ( 163.1118516004056573, -19.27778845539181063, -37.29075403953176959 ) ) ;
#22695=CARTESIAN_POINT ( 'NONE',  ( -109.1264249741459622, 13.72187187123908814, -33.12752917269256159 ) ) ;
#22696=CARTESIAN_POINT ( 'NONE',  ( 170.2234770963711128, 39.99999999999980105, 24.55285855007229401 ) ) ;
#22697=CARTESIAN_POINT ( 'NONE',  ( -91.56559293963836410, 16.03295912088692177, 16.03295912088721664 ) ) ;
#22698=CARTESIAN_POINT ( 'NONE',  ( 146.6084372240433993, 34.62501878078308692, 0.000000000000000000 ) ) ;
#22699=CARTESIAN_POINT ( 'NONE',  ( 170.2234770963711128, -17.36149277827010096, 17.36149277826970660 ) ) ;
#22700=CARTESIAN_POINT ( 'NONE',  ( 130.8568914410475372, 24.07718906447243867, -24.07718906447216156 ) ) ;
#22703=CARTESIAN_POINT ( 'NONE',  ( 170.2234770963711128, -40.00000000000004263, 15.44714144992801685 ) ) ;
#22705=CARTESIAN_POINT ( 'NONE',  ( 19.94008347559388028, 47.92933869853938234, -13.96811062196751863 ) ) ;
#22706=CARTESIAN_POINT ( 'NONE',  ( -105.3755690713226585, -21.75974354311652448, -40.00000000000002132 ) ) ;
#22707=CARTESIAN_POINT ( 'NONE',  ( -56.48582580120559271, -6.472252184284187138, -6.472252184284199572 ) ) ;
#22708=CARTESIAN_POINT ( 'NONE',  ( -162.0762913951021176, 41.69427287672986182, 40.00000000000002132 ) ) ;
#22709=CARTESIAN_POINT ( 'NONE',  ( -7.233308327735402443, -42.27575367454439714, 17.51119053154051031 ) ) ;
#22710=CARTESIAN_POINT ( 'NONE',  ( -208.1127848780264742, 55.00245453014418473, 40.00000000000002132 ) ) ;
#22712=CARTESIAN_POINT ( 'NONE',  ( 21.98945382326336428, 23.63684424402695328, -43.25809532770859533 ) ) ;
#22713=CARTESIAN_POINT ( 'NONE',  ( -213.1075012329537230, -18.58567234101155208, 37.98287015391234434 ) ) ;
#22715=CARTESIAN_POINT ( 'NONE',  ( 6.202588567995411140, 14.15973318134927439, -49.19971320597417730 ) ) ;
#22717=CARTESIAN_POINT ( 'NONE',  ( -192.9588430854689989, 10.23066800230756712, -10.23066800230735396 ) ) ;
#22718=CARTESIAN_POINT ( 'NONE',  ( -77.62874474886855580, -21.73921449502670811, 3.805079090745403736 ) ) ;
#22720=CARTESIAN_POINT ( 'NONE',  ( -188.6890294954570493, -23.53287096354458185, 43.11788624869836184 ) ) ;
#22721=CARTESIAN_POINT ( 'NONE',  ( 192.4448373802101173, -39.99999999999977973, -19.99999999996102673 ) ) ;
#22722=CARTESIAN_POINT ( 'NONE',  ( -56.48582580120559271, -6.472252184284276844, 6.472252184284108978 ) ) ;
#22723=CARTESIAN_POINT ( 'NONE',  ( 184.8905102610680444, 20.92133201514447194, 40.00000000000002132 ) ) ;
#22724=CARTESIAN_POINT ( 'NONE',  ( -190.0144721488044581, 13.91469502168346040, -47.57279682960905376 ) ) ;
#22725=CARTESIAN_POINT ( 'NONE',  ( 4.995406935893286438, 67.35176059880245703, -10.78321810387767066 ) ) ;
#22726=CARTESIAN_POINT ( 'NONE',  ( 200.0000000000000000, 14.14213562373041455, 42.42640687119311593 ) ) ;
#22728=CARTESIAN_POINT ( 'NONE',  ( 192.4448373802101173, -19.99999999996056843, -40.00000000000002132 ) ) ;
#22729=CARTESIAN_POINT ( 'NONE',  ( -105.3755690713226585, 18.24025645688349684, 40.00000000000002132 ) ) ;
#22730=CARTESIAN_POINT ( 'NONE',  ( -162.0762913951021176, -40.00000000000003553, -1.694272876828743168 ) ) ;
#22731=CARTESIAN_POINT ( 'NONE',  ( 57.59792236341147031, 26.56190807104693619, -30.00663442387692115 ) ) ;
#22732=CARTESIAN_POINT ( 'NONE',  ( 146.6084372240433993, -3.800685668858596156, -3.800685668858692967 ) ) ;
#22733=CARTESIAN_POINT ( 'NONE',  ( -105.3755690713226727, 15.38646221621793231, -15.38646221621779020 ) ) ;
#22734=ORIENTED_EDGE ( 'NONE', *, *, #12425, .T. ) ;
#22735=CARTESIAN_POINT ( 'NONE',  ( -86.96347745069644475, -43.67073346367983788, 12.89780903124397149 ) ) ;
#22736=CARTESIAN_POINT ( 'NONE',  ( -105.4732637872234449, 8.153770687239065396, 19.68494377761417979 ) ) ;
#22738=CARTESIAN_POINT ( 'NONE',  ( 192.4448373802100889, -14.14213562370313682, 14.14213562370301958 ) ) ;
#22739=CARTESIAN_POINT ( 'NONE',  ( -3.336279363873598580, -43.33179396957120133, -17.94861674415379937 ) ) ;
#22742=CARTESIAN_POINT ( 'NONE',  ( -100.7734535825088358, -22.67402823373193499, 0.000000000000000000 ) ) ;
#22743=CARTESIAN_POINT ( 'NONE',  ( -199.9999999999997726, -24.82633483071077762, 44.86878812508861358 ) ) ;
#22745=ORIENTED_EDGE ( 'NONE', *, *, #11104, .T. ) ;
#22746=( BOUNDED_SURFACE ( )  B_SPLINE_SURFACE ( 3, 2, ( 
 ( #5637, #21366, #5258 ),
 ( #23729, #19738, #11616 ),
 ( #2060, #16010, #54 ),
 ( #16143, #24277, #16545 ),
 ( #22014, #2316, #14282 ),
 ( #2192, #18407, #6046 ),
 ( #22419, #10424, #26146 ),
 ( #3785, #12025, #18542 ),
 ( #8165, #14151, #20546 ),
 ( #8289, #24544, #11887 ),
 ( #18001, #5773, #3927 ),
 ( #10029, #22283, #20008 ),
 ( #4057, #18139, #12159 ),
 ( #1793, #26287, #7890 ),
 ( #10300, #20145, #182 ),
 ( #24406, #20281, #16416 ),
 ( #14417, #24136, #8026 ),
 ( #6299, #5908, #10166 ) ),
 .UNSPECIFIED., .F., .F., .T. ) 
 B_SPLINE_SURFACE_WITH_KNOTS ( ( 4, 2, 2, 2, 2, 2, 2, 2, 4 ),
 ( 3, 3 ),
 ( 0.04072677052481911419, 0.04791560376915927899, 0.04971281208024432019, 0.05151002039132936139, 0.05510443701349943685, 0.06229327025783959471, 0.06409047856892463590, 0.06588768688000967710, 0.06948210350217975950 ),
 ( 0.000000000000000000, 1.000000000000000000 ),
 .UNSPECIFIED. ) 
 GEOMETRIC_REPRESENTATION_ITEM ( )  RATIONAL_B_SPLINE_SURFACE ( (
 ( 1.000000000000000000, 0.9548354691836614672, 1.000000000000000000),
 ( 1.000000000000000000, 0.9525322272685073921, 1.000000000000000000),
 ( 1.000000000000000000, 0.9507090889564540070, 1.000000000000000000),
 ( 1.000000000000000000, 0.9491274412103997138, 1.000000000000000000),
 ( 1.000000000000000000, 0.9488458704368275543, 1.000000000000000000),
 ( 1.000000000000000000, 0.9483593260462360730, 1.000000000000000000),
 ( 1.000000000000000000, 0.9481536719786518574, 1.000000000000000000),
 ( 1.000000000000000000, 0.9476504944683689091, 1.000000000000000000),
 ( 1.000000000000000000, 0.9474672089150538712, 1.000000000000000000),
 ( 1.000000000000000000, 0.9473824172973602797, 1.000000000000000000),
 ( 1.000000000000000000, 0.9479352605727494607, 1.000000000000000000),
 ( 1.000000000000000000, 0.9493585436777139952, 1.000000000000000000),
 ( 1.000000000000000000, 0.9496800152430581177, 1.000000000000000000),
 ( 1.000000000000000000, 0.9503966249792042964, 1.000000000000000000),
 ( 1.000000000000000000, 0.9507930042074207444, 1.000000000000000000),
 ( 1.000000000000000000, 0.9520783074840074578, 1.000000000000000000),
 ( 1.000000000000000000, 0.9530652555250912483, 1.000000000000000000),
 ( 1.000000000000000000, 0.9541700777564556812, 1.000000000000000000) ) ) 
 REPRESENTATION_ITEM ( '' )  SURFACE ( )  );
#22747=VECTOR ( 'NONE', #6557, 1000.000000000000000 ) ;
#22749=CARTESIAN_POINT ( 'NONE',  ( 12.01361943528961085, 14.17591515420136972, -49.30661675909291830 ) ) ;
#22750=CARTESIAN_POINT ( 'NONE',  ( -56.48582580120558561, -1.205267837095813407E-13, 30.84685318188644132 ) ) ;
#22751=CARTESIAN_POINT ( 'NONE',  ( -86.96347745069644475, 18.24025645688350750, 40.00000000000002132 ) ) ;
#22755=AXIS2_PLACEMENT_3D ( 'NONE', #25766, #19376, #19123 ) ;
#22756=CARTESIAN_POINT ( 'NONE',  ( -56.48582580120558561, -50.09629031063971638, 6.472252184283745713 ) ) ;
#22757=CARTESIAN_POINT ( 'NONE',  ( 199.9999999999999432, -3.553951640073651008E-14, 19.99999999999992539 ) ) ;
#22758=CARTESIAN_POINT ( 'NONE',  ( -56.48582580120560692, 40.00000000000004263, -9.153146818113443217 ) ) ;
#22761=CARTESIAN_POINT ( 'NONE',  ( 91.82158438592159655, -22.79471317813468545, -40.00000000000002132 ) ) ;
#22762=CARTESIAN_POINT ( 'NONE',  ( 146.6084372240433709, 24.48358557860311180, 32.08495691632071356 ) ) ;
#22764=CARTESIAN_POINT ( 'NONE',  ( -110.1003821002792620, 15.15067674040053092, -13.36729751623248497 ) ) ;
#22765=CARTESIAN_POINT ( 'NONE',  ( -259.2033419157646676, 40.00000000000029843, -30.48217210827696988 ) ) ;
#22766=CARTESIAN_POINT ( 'NONE',  ( 57.59792236341149163, -40.00000000000014211, 37.56421063658172699 ) ) ;
#22768=CARTESIAN_POINT ( 'NONE',  ( 73.43468099484965705, -12.96803874020848468, 26.88834960806370233 ) ) ;
#22770=CARTESIAN_POINT ( 'NONE',  ( -91.56559293963834989, -12.25131212657492874, 12.25131212657477953 ) ) ;
#22772=CARTESIAN_POINT ( 'NONE',  ( -188.2995950289363805, 23.44932284466059969, -43.00522595870931752 ) ) ;
#22773=CARTESIAN_POINT ( 'NONE',  ( 137.0939645874030361, 30.33050608226201206, -12.56330697291247844 ) ) ;
#22774=CARTESIAN_POINT ( 'NONE',  ( 57.59792236341147031, 2.435789363418170872, -40.00000000000002132 ) ) ;
#22775=CARTESIAN_POINT ( 'NONE',  ( -86.86493150571121191, -19.77569912839188149, -7.943527260495856446 ) ) ;
#22783=CARTESIAN_POINT ( 'NONE',  ( -86.86493150571128297, 7.943527260495892861, -19.77569912839186372 ) ) ;
#22784=CARTESIAN_POINT ( 'NONE',  ( 23.37583784646053786, 13.80085822091002790, 46.80752016581961072 ) ) ;
#22786=ORIENTED_EDGE ( 'NONE', *, *, #14776, .F. ) ;
#22787=CARTESIAN_POINT ( 'NONE',  ( 170.2234770963711128, -17.36149277826985937, -17.36149277826995174 ) ) ;
#22789=CARTESIAN_POINT ( 'NONE',  ( -105.2276019244893916, -17.02339403573614263, -13.16689311108276783 ) ) ;
#22791=CARTESIAN_POINT ( 'NONE',  ( -86.96347745069644475, -15.38646221621796073, 41.18208027870593924 ) ) ;
#22793=CARTESIAN_POINT ( 'NONE',  ( -109.0492076899303555, 7.884024499252893476E-13, -35.99236577015783212 ) ) ;
#22796=CARTESIAN_POINT ( 'NONE',  ( -135.8532207217289738, 3.005970985514575011E-13, -30.84685318188645553 ) ) ;
#22797=CARTESIAN_POINT ( 'NONE',  ( 57.59792236341146321, 40.00000000000000711, 2.435789363418579434 ) ) ;
#22801=CARTESIAN_POINT ( 'NONE',  ( -173.7925187076908458, 12.78856575072571644, 41.93431653926056413 ) ) ;
#22802=CARTESIAN_POINT ( 'NONE',  ( 200.0000000000000000, -42.42640687119290988, 14.14213562373064903 ) ) ;
#22803=CARTESIAN_POINT ( 'NONE',  ( -97.72675010090438263, 8.987772175319268086, 20.56394680065916347 ) ) ;
#22804=CARTESIAN_POINT ( 'NONE',  ( 0.2972598230770048811, -10.13633138497510089, 66.70487387989852834 ) ) ;
#22806=CARTESIAN_POINT ( 'NONE',  ( -86.96347745069645896, 43.67073346367988762, -12.89780903124366418 ) ) ;
#22808=CARTESIAN_POINT ( 'NONE',  ( -56.48582580120559982, 9.153146818113574668, 40.00000000000002132 ) ) ;
#22810=CARTESIAN_POINT ( 'NONE',  ( 146.6084372240433709, 3.800685668858042821, 52.76785682606522698 ) ) ;
#22811=CARTESIAN_POINT ( 'NONE',  ( 91.82158438592158234, 17.20528682183301683, 0.000000000000000000 ) ) ;
#22813=CARTESIAN_POINT ( 'NONE',  ( 146.6084372240433709, -39.99999999999993605, -5.374981219217395356 ) ) ;
#22815=CARTESIAN_POINT ( 'NONE',  ( 158.3379117892986869, -10.98149362779657601, 26.51167085133944923 ) ) ;
#22816=EDGE_LOOP ( 'NONE', ( #11487, #5116, #13776, #15635 ) ) ;
#22819=CARTESIAN_POINT ( 'NONE',  ( -162.0762913951021176, 41.69427287672986182, 40.00000000000002132 ) ) ;
#22820=CARTESIAN_POINT ( 'NONE',  ( 149.5797498300189261, 12.18602109748300855, 29.41965740490887526 ) ) ;
#22821=CARTESIAN_POINT ( 'NONE',  ( -198.0356074513804572, 67.44298959250878056, -10.87444709758402261 ) ) ;
#22822=CARTESIAN_POINT ( 'NONE',  ( -114.7755410848894968, -22.09261867841506799, 1.384971738882752268 ) ) ;
#22825=CARTESIAN_POINT ( 'NONE',  ( -126.6834156231701769, -9.107266674874638923, 24.89646324320183979 ) ) ;
#22826=CARTESIAN_POINT ( 'NONE',  ( -86.95488169845610571, 6.698970622310091549, -20.33891803571749435 ) ) ;
#22829=CARTESIAN_POINT ( 'NONE',  ( 200.0000000000000000, -14.14213562373046784, -42.42640687119298804 ) ) ;
#22830=CARTESIAN_POINT ( 'NONE',  ( 4.995406935893293543, -10.78321810388990265, -10.78321810389009272 ) ) ;
#22832=CARTESIAN_POINT ( 'NONE',  ( 146.6084372240433709, 39.99999999999968026, 34.62501878078347772 ) ) ;
#22833=DIRECTION ( 'NONE',  ( 0.2259624731720737134, 0.9741360072997814479, 0.000000000000000000 ) ) ;
#22835=CARTESIAN_POINT ( 'NONE',  ( 136.1360204305621266, -24.77266263493116583, -24.77266263493127951 ) ) ;
#22837=EDGE_CURVE ( 'NONE', #6926, #7299, #12454, .T. ) ;
#22838=CARTESIAN_POINT ( 'NONE',  ( -259.2033419157646676, -21.55415060305854524, 21.55415060305827524 ) ) ;
#22839=CARTESIAN_POINT ( 'NONE',  ( -213.1075012329537230, -13.71589010951915810, 0.000000000000000000 ) ) ;
#22841=CARTESIAN_POINT ( 'NONE',  ( 14.38125909742180930, 39.99999999999982947, 55.17850393971022527 ) ) ;
#22842=CARTESIAN_POINT ( 'NONE',  ( 22.72189371635671051, 43.05215026464217232, -23.48424859981733448 ) ) ;
#22843=CARTESIAN_POINT ( 'NONE',  ( 192.4448373802101173, -20.00000000003938538, -40.00000000000002132 ) ) ;
#22844=CARTESIAN_POINT ( 'NONE',  ( -135.8532207217289738, -6.472252184284287502, 50.09629031063965243 ) ) ;
#22845=CARTESIAN_POINT ( 'NONE',  ( -86.96347745069644475, 18.24025645688350750, 40.00000000000002132 ) ) ;
#22846=CARTESIAN_POINT ( 'NONE',  ( -4.439300432583282330, -46.85201324744756590, 13.79990882516902317 ) ) ;
#22847=CARTESIAN_POINT ( 'NONE',  ( 146.6084372240433709, 5.374981219216996564, 40.00000000000002132 ) ) ;
#22849=CARTESIAN_POINT ( 'NONE',  ( 98.29820294268191105, -7.653668647302824368, -18.47759065022797031 ) ) ;
#22851=CARTESIAN_POINT ( 'NONE',  ( -5.296937277128574095, -17.72975434250267313, 42.80341339121885369 ) ) ;
#22852=CARTESIAN_POINT ( 'NONE',  ( -4.810655158401165643, 17.78437748361197990, -42.93528531927893255 ) ) ;
#22854=CARTESIAN_POINT ( 'NONE',  ( -105.3755690713226727, -15.38646221621807619, 15.38646221621768362 ) ) ;
#22856=CARTESIAN_POINT ( 'NONE',  ( -87.10560006382534937, 2.727320883003452767, 21.31071338414146865 ) ) ;
#22857=CARTESIAN_POINT ( 'NONE',  ( -188.2871287166303773, -13.82723289751392137, 46.98614659774630553 ) ) ;
#22858=CARTESIAN_POINT ( 'NONE',  ( 170.2234770963711128, 17.36149277826980253, 17.36149277827007253 ) ) ;
#22859=CARTESIAN_POINT ( 'NONE',  ( 163.1118516004056573, -47.56205970284945295, -9.006482792074823607 ) ) ;
#22860=CARTESIAN_POINT ( 'NONE',  ( -192.9588430854689989, -10.23066800230742501, -10.23066800230756712 ) ) ;
#22861=CARTESIAN_POINT ( 'NONE',  ( 192.4448373802100889, 14.14213562375873678, 14.14213562375894817 ) ) ;
#22862=CARTESIAN_POINT ( 'NONE',  ( 192.4448373802100889, 14.14213562370330379, -14.14213562370292365 ) ) ;
#22863=CARTESIAN_POINT ( 'NONE',  ( -100.7734535825088358, -16.03295912088728770, 16.03295912088687913 ) ) ;
#22864=CARTESIAN_POINT ( 'NONE',  ( 57.59792236341148453, -37.56421063658185489, -40.00000000000002132 ) ) ;
#22865=CARTESIAN_POINT ( 'NONE',  ( -56.48582580120559271, -9.153146818113595984, 0.000000000000000000 ) ) ;
#22866=CARTESIAN_POINT ( 'NONE',  ( -259.2033419157646676, -1.473088368616265084E-13, 9.517827891722632216 ) ) ;
#22867=CARTESIAN_POINT ( 'NONE',  ( -198.0356074513804572, 39.15871834505912119, -17.40982414986464377 ) ) ;
#22868=CARTESIAN_POINT ( 'NONE',  ( -99.31267923334560521, 20.62886818714807191, -8.544756979537151409 ) ) ;
#22869=CARTESIAN_POINT ( 'NONE',  ( 91.82158438592159655, -16.11829626346125011, -16.11829626346154853 ) ) ;
#22870=CARTESIAN_POINT ( 'NONE',  ( 192.4448373802101173, 42.42640687122070631, 14.14213562370331623 ) ) ;
#22872=CARTESIAN_POINT ( 'NONE',  ( -238.4067589809705794, 57.25054294077225592, 0.6820004458485544596 ) ) ;
#22873=CARTESIAN_POINT ( 'NONE',  ( -188.7701102708080612, -13.85300071690466872, -47.15821026576311681 ) ) ;
#22874=CARTESIAN_POINT ( 'NONE',  ( -213.1075012329537230, 18.58567234101121102, 37.98287015391247223 ) ) ;
#22875=CARTESIAN_POINT ( 'NONE',  ( -4.076660308449338466, -42.99426297939334773, -23.44206949513785787 ) ) ;
#22877=CARTESIAN_POINT ( 'NONE',  ( -105.2054292635175727, 15.19799821370213522, 15.19799821370241943 ) ) ;
#22878=CARTESIAN_POINT ( 'NONE',  ( -114.4364955367319823, -8.644468109212290585, -20.04994829327477035 ) ) ;
#22880=CARTESIAN_POINT ( 'NONE',  ( 17.76569288431003812, 14.04863394049499981, -48.46476365406677189 ) ) ;
#22881=CARTESIAN_POINT ( 'NONE',  ( -105.3755690713226727, 18.24025645688350750, 2.449293598294708485E-15 ) ) ;
#22884=CARTESIAN_POINT ( 'NONE',  ( 4.995406935893297984, -39.06748935135205869, 17.50105314357158193 ) ) ;
#22885=CARTESIAN_POINT ( 'NONE',  ( -100.7734535825088500, 39.99999999999994316, 17.32597176626825686 ) ) ;
#22886=CARTESIAN_POINT ( 'NONE',  ( -100.7734535825088500, 40.00000000000008527, -22.67402823373177512 ) ) ;
#22887=CARTESIAN_POINT ( 'NONE',  ( -1.258540240222682849, 47.88180740053044815, -13.96099832920784145 ) ) ;
#22888=CARTESIAN_POINT ( 'NONE',  ( 170.2234770963711128, -15.44714144992812699, -40.00000000000002132 ) ) ;
#22890=CARTESIAN_POINT ( 'NONE',  ( -198.0356074513804572, -55.37879056871328487, -40.00000000000002132 ) ) ;
#22891=CARTESIAN_POINT ( 'NONE',  ( -91.56559293963834989, -12.25131212657492874, 12.25131212657477953 ) ) ;
#22892=FACE_OUTER_BOUND ( 'NONE', #20787, .T. ) ;
#22893=ADVANCED_FACE ( 'NONE', ( #14847 ), #6415, .T. ) ;
#22894=CARTESIAN_POINT ( 'NONE',  ( -105.2958943009977446, 11.44501736924781099, -18.12177707671771998 ) ) ;
#22895=CARTESIAN_POINT ( 'NONE',  ( -162.0762913951021176, 40.00000000000042633, -41.69427287672947102 ) ) ;
#22896=CARTESIAN_POINT ( 'NONE',  ( -91.56559293963836410, 39.99999999999994316, 17.32597176626825330 ) ) ;
#22900=CARTESIAN_POINT ( 'NONE',  ( -238.4067589809705794, -28.96627169325343942, 28.96627169325309126 ) ) ;
#22901=ORIENTED_EDGE ( 'NONE', *, *, #11242, .T. ) ;
#22902=CARTESIAN_POINT ( 'NONE',  ( -91.56559293963836410, 16.03295912088692177, 16.03295912088721664 ) ) ;
#22903=CARTESIAN_POINT ( 'NONE',  ( -189.2428623074473819, 23.64699222226093411, -43.27185639470894074 ) ) ;
#22904=CARTESIAN_POINT ( 'NONE',  ( 149.5797498300188977, 29.41965740490885750, -12.18602109748323592 ) ) ;
#22905=CARTESIAN_POINT ( 'NONE',  ( 130.8568914410475088, 34.05028731879790627, -40.00000000000002132 ) ) ;
#22907=CARTESIAN_POINT ( 'NONE',  ( -105.2274175719510367, 13.17695787001530761, 17.01505826703009205 ) ) ;
#22908=CARTESIAN_POINT ( 'NONE',  ( -200.0000000000000000, -60.00000000000011369, 7.960204194457800407E-15 ) ) ;
#22909=EDGE_LOOP ( 'NONE', ( #6566, #3456, #5701, #22640 ) ) ;
#22910=ORIENTED_EDGE ( 'NONE', *, *, #4274, .T. ) ;
#22911=CARTESIAN_POINT ( 'NONE',  ( 23.37394308801977871, -13.80096434448300613, 46.80823611210190904 ) ) ;
#22913=CARTESIAN_POINT ( 'NONE',  ( 23.38399212876434419, 13.80022400692476836, 46.80460545930715455 ) ) ;
#22916=CARTESIAN_POINT ( 'NONE',  ( 146.6084372240433709, -52.76785682606516303, 3.800685668858563737 ) ) ;
#22918=CARTESIAN_POINT ( 'NONE',  ( -110.0960685945546231, -2.528047301428510085, 20.07406508575495607 ) ) ;
#22919=CARTESIAN_POINT ( 'NONE',  ( 136.1360204305621551, -24.77266263493126885, 31.79587985999256006 ) ) ;
#22920=CARTESIAN_POINT ( 'NONE',  ( -280.0000000000000000, -14.14213562373098831, -14.14213562373098654 ) ) ;
#22921=CARTESIAN_POINT ( 'NONE',  ( -100.7734535825088500, 40.00000000000008527, -22.67402823373177512 ) ) ;
#22922=CARTESIAN_POINT ( 'NONE',  ( -200.0000000000000000, -19.96680831879894669, 45.63305559644814480 ) ) ;
#22925=CARTESIAN_POINT ( 'NONE',  ( -105.3755690713226585, 40.00000000000019185, -18.24025645688310249 ) ) ;
#22926=CARTESIAN_POINT ( 'NONE',  ( -198.0356074513804572, 40.00000000000056843, -55.37879056871282302 ) ) ;
#22928=CARTESIAN_POINT ( 'NONE',  ( -87.11144460356582897, -17.02335282540412109, -13.16693477525666367 ) ) ;
#22931=CARTESIAN_POINT ( 'NONE',  ( -188.3120147333419254, 13.82877842034795712, 46.99495896211607260 ) ) ;
#22932=CARTESIAN_POINT ( 'NONE',  ( -198.0356074513804572, -10.87444709759714634, -10.87444709759729911 ) ) ;
#22934=CARTESIAN_POINT ( 'NONE',  ( 151.7948205124836250, -4.785054706301671068, 4.785054706301645311 ) ) ;
#22936=CARTESIAN_POINT ( 'NONE',  ( 0.2972598230769923355, 18.14793986248751168, -38.42060263243650553 ) ) ;
#22937=CARTESIAN_POINT ( 'NONE',  ( -200.0000000000000568, 47.96425349429458151, -15.65821854886104880 ) ) ;
#22938=DIRECTION ( 'NONE',  ( -0.01051738777840045304, 0.3656191333263374976, 0.9307051272556827737 ) ) ;
#22939=CARTESIAN_POINT ( 'NONE',  ( -91.56559293963834989, 12.25131212657428748, 44.31723036834913643 ) ) ;
#22940=CARTESIAN_POINT ( 'NONE',  ( -192.9588430854690273, -14.46834944099973264, 40.00000000000002132 ) ) ;
#22944=CARTESIAN_POINT ( 'NONE',  ( 184.8905102610680444, 2.362515690532070066E-13, -19.07866798485558490 ) ) ;
#22946=CARTESIAN_POINT ( 'NONE',  ( 118.9130007099545878, -10.68958087202361718, 25.80693111732275113 ) ) ;
#22947=VERTEX_POINT ( 'NONE', #14790 ) ;
#22948=ORIENTED_EDGE ( 'NONE', *, *, #25089, .F. ) ;
#22949=CARTESIAN_POINT ( 'NONE',  ( -86.96347745069644475, 18.24025645688350750, 40.00000000000002132 ) ) ;
#22952=CARTESIAN_POINT ( 'NONE',  ( -105.3394646353531954, -20.62740382080770729, -5.712077376962630737 ) ) ;
#22953=DIRECTION ( 'NONE',  ( 0.9698969544411814026, 0.09318942518809772424, -0.2249791741447042526 ) ) ;
#22954=CARTESIAN_POINT ( 'NONE',  ( 91.82158438592158234, 7.693928927950222250E-14, -17.20528682183300262 ) ) ;
#22958=CARTESIAN_POINT ( 'NONE',  ( -238.4067589809705794, 0.6820004457912851592, -0.6820004457913123597 ) ) ;
#22959=CARTESIAN_POINT ( 'NONE',  ( -198.0356074513804572, -10.87444709759714634, -10.87444709759729911 ) ) ;
#22960=CYLINDRICAL_SURFACE ( 'NONE', #13134, 69.99999999999994316 ) ;
#22961=CARTESIAN_POINT ( 'NONE',  ( 91.82158438592156813, 39.99999999999986500, 17.20528682183341473 ) ) ;
#22962=CARTESIAN_POINT ( 'NONE',  ( 0.2972598230769976091, -10.13633138497465147, -10.13633138497482733 ) ) ;
#22963=CARTESIAN_POINT ( 'NONE',  ( -198.0356074513804572, -15.37879056873074290, 0.000000000000000000 ) ) ;
#22964=CARTESIAN_POINT ( 'NONE',  ( -135.8532207217289738, -6.472252184284287502, 50.09629031063965243 ) ) ;
#22965=CARTESIAN_POINT ( 'NONE',  ( 19.06497207195982568, -38.31983398719646061, 38.31983398719606271 ) ) ;
#22969=CARTESIAN_POINT ( 'NONE',  ( 130.8568914410475372, 1.429239637432775288E-13, -34.05028731879788495 ) ) ;
#22970=CARTESIAN_POINT ( 'NONE',  ( 44.46627453574045319, 36.79413088008411137, -15.24062802596003507 ) ) ;
#22971=CARTESIAN_POINT ( 'NONE',  ( 130.8568914410475372, -34.05028731879786363, 0.000000000000000000 ) ) ;
#22972=CARTESIAN_POINT ( 'NONE',  ( 91.82158438592158234, -12.16597498397761967, -12.16597498397768007 ) ) ;
#22973=CARTESIAN_POINT ( 'NONE',  ( 184.8905102610680444, -20.92133201514440799, 40.00000000000002132 ) ) ;
#22976=CARTESIAN_POINT ( 'NONE',  ( -2.004660104900875872, -43.67474423982626774, 18.09067139730424500 ) ) ;
#22977=CARTESIAN_POINT ( 'NONE',  ( 151.7948205124836534, -33.23291073765550863, 40.00000000000002132 ) ) ;
#22978=ORIENTED_EDGE ( 'NONE', *, *, #25921, .T. ) ;
#22980=EDGE_CURVE ( 'NONE', #2033, #16316, #19560, .T. ) ;
#22981=CARTESIAN_POINT ( 'NONE',  ( -162.0762913951020892, 1.198031840385716418, 1.198031840385750169 ) ) ;
#22982=CARTESIAN_POINT ( 'NONE',  ( -4.061681315507533974, -23.44498947467614514, 42.99867639910929995 ) ) ;
#22983=CARTESIAN_POINT ( 'NONE',  ( 19.06497207195980792, 10.03556273973433299, 10.03556273973436319 ) ) ;
#22984=EDGE_CURVE ( 'NONE', #18786, #14909, #21988, .T. ) ;
#22986=CARTESIAN_POINT ( 'NONE',  ( -4.022465846214347884, 13.82902411340800519, -46.99661175925213996 ) ) ;
#22988=CARTESIAN_POINT ( 'NONE',  ( 192.4448373802100889, -14.14213562375896061, 14.14213562375865330 ) ) ;
#22991=CARTESIAN_POINT ( 'NONE',  ( -188.4702232936913333, -13.83721295434360421, 47.05182887786764923 ) ) ;
#22992=CARTESIAN_POINT ( 'NONE',  ( 14.38125909742181285, -10.73282306404712472, -10.73282306404731301 ) ) ;
#22993=CARTESIAN_POINT ( 'NONE',  ( 163.1118516004056573, 19.27778845539212327, 37.29075403953164169 ) ) ;
#22994=CARTESIAN_POINT ( 'NONE',  ( 0.2972598230769938343, 10.13633138497486286, -10.13633138497461594 ) ) ;
#22995=CARTESIAN_POINT ( 'NONE',  ( -135.8532207217289738, 34.75652343174625258, -21.81201906317744132 ) ) ;
#22996=DIRECTION ( 'NONE',  ( 0.7071067811865440200, 0.7071067811865511255, 0.000000000000000000 ) ) ;
#22997=CARTESIAN_POINT ( 'NONE',  ( 163.1118516004056573, 37.29075403953132906, 19.27778845539275565 ) ) ;
#22998=CARTESIAN_POINT ( 'NONE',  ( -198.0356074513804572, 39.15871834505887250, 17.40982414986519089 ) ) ;
#22999=CARTESIAN_POINT ( 'NONE',  ( -192.9588430854689989, -14.46834944099973086, 0.000000000000000000 ) ) ;
#23000=CARTESIAN_POINT ( 'NONE',  ( 19.06497207195980792, 14.19242893257840699, -40.00000000000002132 ) ) ;
#23001=CARTESIAN_POINT ( 'NONE',  ( 19.06497207195980792, 66.60410523465817789, 10.03556273973446800 ) ) ;
#23003=CARTESIAN_POINT ( 'NONE',  ( -100.7734535825088358, -12.25131212657475643, -12.25131212657495539 ) ) ;
#23005=CARTESIAN_POINT ( 'NONE',  ( -187.3036811847820786, 42.71162014089968295, -23.25512365539639958 ) ) ;
#23007=CARTESIAN_POINT ( 'NONE',  ( 130.8568914410475088, -24.07718906446910623, 32.49135343045471558 ) ) ;
#23010=AXIS2_PLACEMENT_3D ( 'NONE', #5077, #17416, #21302 ) ;
#23011=CARTESIAN_POINT ( 'NONE',  ( -93.02511667906952653, -20.82219708225693466, -8.169918093965536698 ) ) ;
#23014=CARTESIAN_POINT ( 'NONE',  ( 136.1360204305621266, -3.511608612530682905, 3.511608612530666917 ) ) ;
#23015=CARTESIAN_POINT ( 'NONE',  ( 4.155455573178285178, -44.65020969900605508, -18.49472242011575673 ) ) ;
#23016=ORIENTED_EDGE ( 'NONE', *, *, #1673, .F. ) ;
#23017=CARTESIAN_POINT ( 'NONE',  ( 136.1360204305621266, -35.03383547441293899, 0.000000000000000000 ) ) ;
#23018=CARTESIAN_POINT ( 'NONE',  ( -87.13361725327074225, -15.19799821270840035, -15.19799821270843765 ) ) ;
#23021=CARTESIAN_POINT ( 'NONE',  ( 19.06497207195980792, 54.19242893257843718, 2.449293598294708485E-15 ) ) ;
#23025=CARTESIAN_POINT ( 'NONE',  ( 151.7948205124836534, -33.06932595376376582, 23.49921654115996006 ) ) ;
#23026=CARTESIAN_POINT ( 'NONE',  ( -198.0356074513804572, -2.321818583541004323E-13, 55.37879056873073580 ) ) ;
#23027=CARTESIAN_POINT ( 'NONE',  ( -135.8532207217289738, 39.99999999999989342, 30.84685318188660474 ) ) ;
#23029=CARTESIAN_POINT ( 'NONE',  ( -213.1075012329536946, -53.71589010951918652, -2.449293598294708485E-15 ) ) ;
#23030=CARTESIAN_POINT ( 'NONE',  ( 22.86726691379337595, -17.87269271907613444, -43.14849715852183465 ) ) ;
#23031=CARTESIAN_POINT ( 'NONE',  ( 170.2234770963711128, 17.36149277827004411, -17.36149277826983095 ) ) ;
#23032=CARTESIAN_POINT ( 'NONE',  ( 184.8905102610680444, -19.07866798485555293, -2.449293598294708485E-15 ) ) ;
#23033=CARTESIAN_POINT ( 'NONE',  ( -91.56559293963836410, 16.03295912088714203, -16.03295912088699282 ) ) ;
#23034=CARTESIAN_POINT ( 'NONE',  ( 125.5832160019860169, -11.61997419108375063, -28.05309928653998242 ) ) ;
#23035=CARTESIAN_POINT ( 'NONE',  ( -114.5444905533168338, 9.939131763671985809, -19.55376799566989732 ) ) ;
#23036=CARTESIAN_POINT ( 'NONE',  ( -280.0000000000000000, 1.605030083646939673E-13, -20.00000000000001421 ) ) ;
#23037=CARTESIAN_POINT ( 'NONE',  ( -100.7734535825088358, -16.03295912088706743, -16.03295912088710296 ) ) ;
#23038=CARTESIAN_POINT ( 'NONE',  ( -105.2054292635175585, 21.49321519473984665, 5.610018989487960791E-28 ) ) ;
#23040=CARTESIAN_POINT ( 'NONE',  ( -86.96347745069644475, -12.89780903124413491, 12.89780903124398037 ) ) ;
#23042=CARTESIAN_POINT ( 'NONE',  ( -56.48582580120559271, 6.472252184284121412, 6.472252184284244869 ) ) ;
#23043=CARTESIAN_POINT ( 'NONE',  ( -17.28139728232450878, 39.07633224428969498, -20.85871090880913670 ) ) ;
#23045=CARTESIAN_POINT ( 'NONE',  ( -86.96347745069644475, -18.24025645688354302, -2.449293598294708485E-15 ) ) ;
#23046=CARTESIAN_POINT ( 'NONE',  ( -114.7537493279933187, 13.57142477590316254, -17.50316801958423341 ) ) ;
#23047=CARTESIAN_POINT ( 'NONE',  ( -238.4067589809705794, 0.6820004457912851592, -0.6820004457913123597 ) ) ;
#23055=ORIENTED_EDGE ( 'NONE', *, *, #25999, .F. ) ;
#23056=CARTESIAN_POINT ( 'NONE',  ( -162.0762913951021176, 1.198031840315997298, 57.76657433523996588 ) ) ;
#23058=CARTESIAN_POINT ( 'NONE',  ( -114.7755410848759112, 1.384971738882062819, 22.09261867840957194 ) ) ;
#23059=CARTESIAN_POINT ( 'NONE',  ( 199.9999999999999432, -14.14213562373096345, -14.14213562373104871 ) ) ;
#23061=CARTESIAN_POINT ( 'NONE',  ( -105.3755690713226585, 39.99999999999993605, 18.24025645688366737 ) ) ;
#23063=CARTESIAN_POINT ( 'NONE',  ( -86.86578273022547592, -8.153770686795120071, -19.68494377654086236 ) ) ;
#23064=CARTESIAN_POINT ( 'NONE',  ( -100.7734535825088500, -39.99999999999986500, -17.32597176626853397 ) ) ;
#23065=CARTESIAN_POINT ( 'NONE',  ( 130.8568914410475372, -3.326198072800416995E-13, 34.05028731879788495 ) ) ;
#23066=CARTESIAN_POINT ( 'NONE',  ( -87.10945906665416771, 16.83914111323053220, 13.33429271096284729 ) ) ;
#23070=CARTESIAN_POINT ( 'NONE',  ( -190.0144222803081675, 23.79986276084134289, 43.47820992357743819 ) ) ;
#23071=CARTESIAN_POINT ( 'NONE',  ( -162.0762913951020892, -1.198031840385767266, -1.198031840385758384 ) ) ;
#23072=CARTESIAN_POINT ( 'NONE',  ( -89.92902785008925548, 8.734793929541238455, 20.17328762787341034 ) ) ;
#23073=CARTESIAN_POINT ( 'NONE',  ( 19.06497207195981858, -10.03556273973469715, 66.60410523465813526 ) ) ;
#23074=CARTESIAN_POINT ( 'NONE',  ( -82.30220482034327745, -18.51665893431350085, 7.992411108785186791 ) ) ;
#23075=CARTESIAN_POINT ( 'NONE',  ( -100.7734535825088500, 16.03295912088740494, -40.53558337403661938 ) ) ;
#23077=CARTESIAN_POINT ( 'NONE',  ( 170.2234770963711128, 24.55285855007190676, 40.00000000000002132 ) ) ;
#23078=CARTESIAN_POINT ( 'NONE',  ( -56.48582580120559982, 21.81201906317729922, 34.75652343174635917 ) ) ;
#23079=CARTESIAN_POINT ( 'NONE',  ( -100.7734535825088500, 22.67402823373189946, 40.00000000000002132 ) ) ;
#23081=VERTEX_POINT ( 'NONE', #17053 ) ;
#23082=CARTESIAN_POINT ( 'NONE',  ( -192.9588430854690273, -39.99999999999991473, -14.46834944100011633 ) ) ;
#23083=CARTESIAN_POINT ( 'NONE',  ( -105.4741150117383341, -8.366608964593364561, -19.60045294982747777 ) ) ;
#23085=CARTESIAN_POINT ( 'NONE',  ( 130.1167162091012983, -12.15076864148480418, 29.33455044752945895 ) ) ;
#23089=CARTESIAN_POINT ( 'NONE',  ( 192.4448373802101173, 19.99999999996063949, 40.00000000000002132 ) ) ;
#23090=ADVANCED_FACE ( 'NONE', ( #15811 ), #5714, .T. ) ;
#23093=CARTESIAN_POINT ( 'NONE',  ( -105.2833435977218812, -20.98775841734472181, -4.389626034958370226 ) ) ;
#23094=CARTESIAN_POINT ( 'NONE',  ( 151.7948205124836250, -23.49921654116339553, -23.49921654116350211 ) ) ;
#23095=CARTESIAN_POINT ( 'NONE',  ( -280.0000000000000568, -40.00000000000000000, -20.00000000000015277 ) ) ;
#23098=CARTESIAN_POINT ( 'NONE',  ( -198.0356074513804572, -17.40982414986427429, -39.15871834505933435 ) ) ;
#23099=CARTESIAN_POINT ( 'NONE',  ( 19.06497207195981147, -10.03556273973425483, -10.03556273973443247 ) ) ;
#23101=CARTESIAN_POINT ( 'NONE',  ( 163.1118516004056573, 1.658263919738574066E-13, -12.73709011382475254 ) ) ;
#23102=CARTESIAN_POINT ( 'NONE',  ( 163.1118516004056573, 19.27778845538753316, 19.27778845538783870 ) ) ;
#23103=CARTESIAN_POINT ( 'NONE',  ( 17.75917311731579673, 14.04884443869898014, 48.46615948699193410 ) ) ;
#23104=CARTESIAN_POINT ( 'NONE',  ( -192.9588430854690273, -10.23066800229550388, 66.79921049721887982 ) ) ;
#23107=CARTESIAN_POINT ( 'NONE',  ( 0.2972598230769957217, -4.999556039334937811E-14, 14.33493731733933352 ) ) ;
#23108=CARTESIAN_POINT ( 'NONE',  ( 19.06497207195980792, 14.19242893257840699, -40.00000000000002132 ) ) ;
#23109=CARTESIAN_POINT ( 'NONE',  ( -198.0356074513804572, 10.87444709758468875, 67.44298959250869530 ) ) ;
#23110=CARTESIAN_POINT ( 'NONE',  ( -86.96347745069644475, -21.75974354311652093, 40.00000000000002132 ) ) ;
#23112=CARTESIAN_POINT ( 'NONE',  ( 11.28112952475396469, -44.87390167240484118, 18.58737866931859983 ) ) ;
#23113=CARTESIAN_POINT ( 'NONE',  ( -86.96347745069644475, -21.75974354311652093, -40.00000000000002132 ) ) ;
#23114=CARTESIAN_POINT ( 'NONE',  ( 170.0000000000000000, -24.95097643316997704, 0.000000000000000000 ) ) ;
#23115=CARTESIAN_POINT ( 'NONE',  ( -280.0000000000000000, 14.14213562373088351, 14.14213562373098654 ) ) ;
#23116=CARTESIAN_POINT ( 'NONE',  ( 14.38125909742181818, -40.00000000000007816, 15.17850393972619649 ) ) ;
#23117=CARTESIAN_POINT ( 'NONE',  ( -82.26903151907711731, 19.50325165503522840, 5.351754661224573439 ) ) ;
#23118=CARTESIAN_POINT ( 'NONE',  ( -39.81953879993444190, 16.38089232947213958, -32.18669035976384407 ) ) ;
#23120=CARTESIAN_POINT ( 'NONE',  ( -192.9588430854690273, 38.51493924976913519, 18.05360324515490333 ) ) ;
#23121=CARTESIAN_POINT ( 'NONE',  ( -82.26531528646586366, -19.58553546193898853, 5.040628272971080293 ) ) ;
#23123=CARTESIAN_POINT ( 'NONE',  ( -195.5008451366654469, -18.44412755964216899, 44.52806290062937222 ) ) ;
#23124=CARTESIAN_POINT ( 'NONE',  ( -56.48582580120559271, 6.472252184284121412, 6.472252184284244869 ) ) ;
#23126=CARTESIAN_POINT ( 'NONE',  ( -91.56559293963836410, 16.03295912088714203, -16.03295912088699282 ) ) ;
#23127=CARTESIAN_POINT ( 'NONE',  ( -162.0762913951020892, 1.198031840385732849, -1.198031840385733515 ) ) ;
#23128=CARTESIAN_POINT ( 'NONE',  ( -192.9588430854690273, 18.05360324515473280, -38.51493924976924177 ) ) ;
#23129=CARTESIAN_POINT ( 'NONE',  ( -56.48582580120559982, 34.75652343174628101, -21.81201906317743067 ) ) ;
#23130=CARTESIAN_POINT ( 'NONE',  ( 0.2972598230769959993, 38.42060263243713081, -38.42060263243619289 ) ) ;
#23131=CARTESIAN_POINT ( 'NONE',  ( 14.38125909742181108, 39.01709431150961649, -39.01709431150867147 ) ) ;
#23132=CARTESIAN_POINT ( 'NONE',  ( 57.59792236341147031, 37.56421063658187620, -40.00000000000002132 ) ) ;
#23133=CARTESIAN_POINT ( 'NONE',  ( -100.7734535825088358, -16.03295912088706743, -16.03295912088710296 ) ) ;
#23135=CARTESIAN_POINT ( 'NONE',  ( -91.56559293963836410, -12.25131212657524138, 44.31723036834888774 ) ) ;
#23137=CARTESIAN_POINT ( 'NONE',  ( -188.8753211508393690, 43.29880796194926518, -17.93495349242721204 ) ) ;
#23138=EDGE_LOOP ( 'NONE', ( #4062, #4816, #22048, #21215 ) ) ;
#23139=CARTESIAN_POINT ( 'NONE',  ( 200.0000000000000000, -14.14213562373106114, 42.42640687119278908 ) ) ;
#23140=CARTESIAN_POINT ( 'NONE',  ( -87.13361725327074225, -15.19799821270840390, -15.19799821270844120 ) ) ;
#23141=CARTESIAN_POINT ( 'NONE',  ( -30.26275506840322649, -29.48230279907810925, 29.48230279907778950 ) ) ;
#23142=CARTESIAN_POINT ( 'NONE',  ( -77.90022806219018037, -20.16431395584817210, -8.352332316461392736 ) ) ;
#23144=CARTESIAN_POINT ( 'NONE',  ( -105.3942160150412519, 19.19970061689178564, 9.473065214623858310 ) ) ;
#23147=CARTESIAN_POINT ( 'NONE',  ( -198.0356074513804572, 55.37879056873070027, 2.449293598294708485E-15 ) ) ;
#23148=CARTESIAN_POINT ( 'NONE',  ( 83.11963132832433132, 9.001241435325864515, -24.42551322443806683 ) ) ;
#23150=CARTESIAN_POINT ( 'NONE',  ( 163.1118516004056573, -37.29075403953166301, 19.27778845539196695 ) ) ;
#23151=CARTESIAN_POINT ( 'NONE',  ( -280.0000000000000568, 39.99999999999990763, 20.00000000000015987 ) ) ;
#23152=CARTESIAN_POINT ( 'NONE',  ( 146.6084372240433709, 40.00000000000003553, 5.374981219217116468 ) ) ;
#23154=CARTESIAN_POINT ( 'NONE',  ( -162.0762913951020892, -41.69427287672991866, -40.00000000000002132 ) ) ;
#23155=CARTESIAN_POINT ( 'NONE',  ( 27.55177309529138441, -22.48880744266456588, -41.56868263114530748 ) ) ;
#23156=CARTESIAN_POINT ( 'NONE',  ( -91.56559293963836410, 16.03295912088714203, -16.03295912088699282 ) ) ;
#23157=CARTESIAN_POINT ( 'NONE',  ( -86.96347745069643054, -18.24025645688353947, 40.00000000000002132 ) ) ;
#23158=CARTESIAN_POINT ( 'NONE',  ( -56.48582580120559271, 6.472252184284211118, -6.472252184284153387 ) ) ;
#23159=CARTESIAN_POINT ( 'NONE',  ( 146.6084372240433993, -3.357462877844280890E-13, 34.62501878078305850 ) ) ;
#23160=CARTESIAN_POINT ( 'NONE',  ( -114.7248266913118897, 17.87714126013195326, -12.97729011815941469 ) ) ;
#23161=CARTESIAN_POINT ( 'NONE',  ( -208.1127848780264742, -39.99999999999990763, -15.00245453012711394 ) ) ;
#23162=CARTESIAN_POINT ( 'NONE',  ( -198.0356074513804572, 10.87444709759714989, 10.87444709759722450 ) ) ;
#23165=CARTESIAN_POINT ( 'NONE',  ( -162.0762913951021176, 27.08623940707598265, 29.48230308784781428 ) ) ;
#23168=CARTESIAN_POINT ( 'NONE',  ( -86.94949953272028154, 19.08279132442754644, -9.637191076863791395 ) ) ;
#23169=CARTESIAN_POINT ( 'NONE',  ( -70.35386311751949506, 22.51194464734792433, -10.19784241718953588 ) ) ;
#23170=CARTESIAN_POINT ( 'NONE',  ( 156.1979191798868101, 27.38417834433190379, -11.34289806466565764 ) ) ;
#23171=CARTESIAN_POINT ( 'NONE',  ( -259.2033419157646676, 9.517827891722582478, 40.00000000000002132 ) ) ;
#23173=CARTESIAN_POINT ( 'NONE',  ( -197.4154352061690645, 49.11380478896982282, -14.14666496776101212 ) ) ;
#23175=ORIENTED_EDGE ( 'NONE', *, *, #11555, .F. ) ;
#23177=CARTESIAN_POINT ( 'NONE',  ( 98.29820294267312875, 7.653668647304333383, -18.47759065023115355 ) ) ;
#23178=CARTESIAN_POINT ( 'NONE',  ( -190.1760717698206520, 43.55712811720382405, -23.85870456570982157 ) ) ;
#23182=CARTESIAN_POINT ( 'NONE',  ( 163.1118516004056573, -19.27778845538761132, -19.27778845538770724 ) ) ;
#23183=CARTESIAN_POINT ( 'NONE',  ( 192.4448373802100889, -14.14213562375876698, -14.14213562375885047 ) ) ;
#23184=CARTESIAN_POINT ( 'NONE',  ( 163.1118516004056573, 40.00000000000000711, 12.73709011382489642 ) ) ;
#23185=CARTESIAN_POINT ( 'NONE',  ( -99.21568817060988010, 6.094032021297641100E-14, -22.67402823373191723 ) ) ;
#23187=CARTESIAN_POINT ( 'NONE',  ( 199.9999999999999432, 2.486775779033024914E-13, -19.99999999999992539 ) ) ;
#23189=CARTESIAN_POINT ( 'NONE',  ( -259.2033419157646676, -39.99999999999975131, -30.48217210827782608 ) ) ;
#23190=CARTESIAN_POINT ( 'NONE',  ( -82.25253345620868117, 16.60364765899479167, 11.48998332232444852 ) ) ;
#23191=CARTESIAN_POINT ( 'NONE',  ( -199.9999999999999147, -14.17215463606695280, 49.28189405767609088 ) ) ;
#23193=CARTESIAN_POINT ( 'NONE',  ( -208.1127848780265026, -10.60833733269551971, 10.60833733269537049 ) ) ;
#23194=CARTESIAN_POINT ( 'NONE',  ( -162.0762913951021176, -29.48230308784793152, 27.08623940707591515 ) ) ;
#23195=CARTESIAN_POINT ( 'NONE',  ( -188.7701069479165881, -47.15820909662600968, 13.85300054332501851 ) ) ;
#23196=CARTESIAN_POINT ( 'NONE',  ( 170.0000000000000000, 3.122849337825751958E-14, 0.000000000000000000 ) ) ;
#23197=CARTESIAN_POINT ( 'NONE',  ( -77.90255099906769942, 20.29001641120678201, -8.064892378658056415 ) ) ;
#23199=CARTESIAN_POINT ( 'NONE',  ( 0.2972598230770100991, -38.42060263243632079, -38.42060263243699580 ) ) ;
#23200=CARTESIAN_POINT ( 'NONE',  ( -200.0000000000000000, 48.59548038928832625, -14.89048929005512001 ) ) ;
#23201=CARTESIAN_POINT ( 'NONE',  ( 23.37394308801977871, 23.33966569535068203, 42.85717664514594816 ) ) ;
#23203=CARTESIAN_POINT ( 'NONE',  ( -91.56559293963834989, 40.53558337403654832, 16.03295912088756481 ) ) ;
#23206=ORIENTED_EDGE ( 'NONE', *, *, #17937, .T. ) ;
#23207=CARTESIAN_POINT ( 'NONE',  ( 4.995406935893298872, 5.820775922023080204E-13, -55.24977328854835434 ) ) ;
#23212=VERTEX_POINT ( 'NONE', #5330 ) ;
#23215=CARTESIAN_POINT ( 'NONE',  ( 136.1360204305621266, 4.966164525587089429, 2.449293598294708485E-15 ) ) ;
#23217=CARTESIAN_POINT ( 'NONE',  ( -77.90255099906769942, -20.04994828523962269, 8.644468104261498809 ) ) ;
#23218=( BOUNDED_SURFACE ( )  B_SPLINE_SURFACE ( 3, 2, ( 
 ( #19298, #9190, #17303 ),
 ( #23427, #3199, #11307 ),
 ( #19426, #13809, #26352 ),
 ( #22351, #24344, #20345 ),
 ( #6108, #14216, #13686 ),
 ( #1861, #21943, #4129 ),
 ( #20213, #3992, #3719 ),
 ( #11958, #11821, #15803 ),
 ( #19939, #9696, #7958 ),
 ( #24067, #12091, #5977 ),
 ( #26083, #9832, #21807 ),
 ( #7818, #18071, #1724 ),
 ( #22082, #9965, #23928 ),
 ( #8093, #14085, #1991 ),
 ( #15934, #3580, #5843 ),
 ( #12223, #26222, #20083 ),
 ( #17936, #121, #10097 ),
 ( #13947, #3855, #19809 ),
 ( #17803, #18199, #2122 ),
 ( #25949, #5703, #16076 ),
 ( #24204, #22216, #16213 ),
 ( #1595, #10230, #16344 ),
 ( #18339, #8226, #5579 ),
 ( #11683, #7690, #12892 ),
 ( #6628, #12481, #10495 ),
 ( #24607, #24742, #10901 ),
 ( #24476, #656, #2517 ),
 ( #19013, #20879, #10764 ),
 ( #8763, #10632, #6763 ),
 ( #4788, #18608, #791 ),
 ( #4652, #18743, #14352 ),
 ( #387, #524, #8496 ),
 ( #12349, #20608, #10360 ),
 ( #21006, #23015, #16878 ),
 ( #6238, #22480, #4259 ),
 ( #16609, #12620, #6497 ),
 ( #8629, #8895, #2788 ),
 ( #14745, #22613, #20478 ),
 ( #6361, #2251, #14608 ),
 ( #2383, #22739, #18470 ),
 ( #4522, #251, #20748 ),
 ( #24873, #25010, #4389 ),
 ( #14875, #16740, #8360 ),
 ( #14480, #12755, #16481 ),
 ( #22875, #2659, #18876 ),
 ( #21270, #3044, #11521 ),
 ( #7151, #5172, #1299 ),
 ( #17136, #21522, #3171 ),
 ( #17514, #25269, #11392 ),
 ( #7399, #9409, #5420 ),
 ( #25653, #15512, #25143 ),
 ( #13276, #7019, #23642 ),
 ( #5290, #15393, #15140 ),
 ( #23396, #23270, #921 ),
 ( #5045, #21145, #19394 ),
 ( #9150, #23518, #17389 ),
 ( #11151, #19266, #6894 ),
 ( #1048, #13521, #13152 ),
 ( #3419, #17265, #25400 ),
 ( #3296, #23142, #21647 ) ),
 .UNSPECIFIED., .F., .F., .F. ) 
 B_SPLINE_SURFACE_WITH_KNOTS ( ( 4, 2, 2, 2, 2, 2, 2, 2, 2, 2, 2, 2, 2, 2, 2, 2, 2, 2, 2, 2, 2, 2, 2, 2, 2, 2, 2, 2, 2, 4 ),
 ( 3, 3 ),
 ( -6.934549977324728988E-05, 0.02465257023823467716, 0.04937448597624260332, 0.07409640171425052602, 0.08027688064875250495, 0.08066316058215888818, 0.08085630054886207285, 0.08090458554053786555, 0.08095287053221367213, 0.08104944051556525753, 0.08182200038237799622, 0.08336712011600350136, 0.08645735958325448389, 0.09263783851775647671, 0.09881831745225845565, 0.1019085569195094521, 0.1049987963867604346, 0.1111792753212624274, 0.1173597542557644063, 0.1177460341891707896, 0.1179391741558739742, 0.1179874591475497669, 0.1180357441392255735, 0.1181323141225771589, 0.1189048739893898976, 0.1204499937230154027, 0.1235402331902663853, 0.1482621489282743010, 0.1729840646662822445, 0.1977059804042901603 ),
 ( 0.000000000000000000, 1.000000000000000000 ),
 .UNSPECIFIED. ) 
 GEOMETRIC_REPRESENTATION_ITEM ( )  RATIONAL_B_SPLINE_SURFACE ( (
 ( 1.000000000000000000, 1.000000000000000000, 1.000000000000000000),
 ( 1.000000000000000000, 0.9999975583951711267, 1.000000000000000000),
 ( 1.000000000000000000, 0.9982436956960243357, 1.000000000000000000),
 ( 1.000000000000000000, 0.9910288481552835815, 1.000000000000000000),
 ( 1.000000000000000000, 0.9855714588524815412, 1.000000000000000000),
 ( 1.000000000000000000, 0.9705958323307124491, 1.000000000000000000),
 ( 1.000000000000000000, 0.9610788543728796540, 1.000000000000000000),
 ( 1.000000000000000000, 0.9462867046313782060, 1.000000000000000000),
 ( 1.000000000000000000, 0.9431828180755336133, 1.000000000000000000),
 ( 1.000000000000000000, 0.9397240291170312343, 1.000000000000000000),
 ( 1.000000000000000000, 0.9395199791396151578, 1.000000000000000000),
 ( 1.000000000000000000, 0.9392130141387098341, 1.000000000000000000),
 ( 1.000000000000000000, 0.9391105441324959502, 1.000000000000000000),
 ( 1.000000000000000000, 0.9389822709566335579, 1.000000000000000000),
 ( 1.000000000000000000, 0.9389566070380604978, 1.000000000000000000),
 ( 1.000000000000000000, 0.9389052606279734148, 1.000000000000000000),
 ( 1.000000000000000000, 0.9388799835492064316, 1.000000000000000000),
 ( 1.000000000000000000, 0.9388039637710021701, 1.000000000000000000),
 ( 1.000000000000000000, 0.9387533729070449695, 1.000000000000000000),
 ( 1.000000000000000000, 0.9382988607466934416, 1.000000000000000000),
 ( 1.000000000000000000, 0.9379005790853075508, 1.000000000000000000),
 ( 1.000000000000000000, 0.9367237203702429849, 1.000000000000000000),
 ( 1.000000000000000000, 0.9359625442026195952, 1.000000000000000000),
 ( 1.000000000000000000, 0.9337619511408732365, 1.000000000000000000),
 ( 1.000000000000000000, 0.9324064515427972211, 1.000000000000000000),
 ( 1.000000000000000000, 0.9287106072117489175, 1.000000000000000000),
 ( 1.000000000000000000, 0.9267422912951360781, 1.000000000000000000),
 ( 1.000000000000000000, 0.9239539123014891553, 1.000000000000000000),
 ( 1.000000000000000000, 0.9231338493909951870, 1.000000000000000000),
 ( 1.000000000000000000, 0.9228496048506062976, 1.000000000000000000),
 ( 1.000000000000000000, 0.9229135694615097085, 1.000000000000000000),
 ( 1.000000000000000000, 0.9233494155302127693, 1.000000000000000000),
 ( 1.000000000000000000, 0.9237209353787610988, 1.000000000000000000),
 ( 1.000000000000000000, 0.9252744993865242851, 1.000000000000000000),
 ( 1.000000000000000000, 0.9268968421605615626, 1.000000000000000000),
 ( 1.000000000000000000, 0.9311673748452381494, 1.000000000000000000),
 ( 1.000000000000000000, 0.9338157035272729445, 1.000000000000000000),
 ( 1.000000000000000000, 0.9370733336298818772, 1.000000000000000000),
 ( 1.000000000000000000, 0.9372665829346543687, 1.000000000000000000),
 ( 1.000000000000000000, 0.9375588533504843891, 1.000000000000000000),
 ( 1.000000000000000000, 0.9376566762263829347, 1.000000000000000000),
 ( 1.000000000000000000, 0.9377794499114591176, 1.000000000000000000),
 ( 1.000000000000000000, 0.9378038842964694366, 1.000000000000000000),
 ( 1.000000000000000000, 0.9378536652368906212, 1.000000000000000000),
 ( 1.000000000000000000, 0.9378785472098781772, 1.000000000000000000),
 ( 1.000000000000000000, 0.9379531676447521171, 1.000000000000000000),
 ( 1.000000000000000000, 0.9380028806225367832, 1.000000000000000000),
 ( 1.000000000000000000, 0.9384499917948696535, 1.000000000000000000),
 ( 1.000000000000000000, 0.9388452506063797998, 1.000000000000000000),
 ( 1.000000000000000000, 0.9400245377240861178, 1.000000000000000000),
 ( 1.000000000000000000, 0.9408020798628555781, 1.000000000000000000),
 ( 1.000000000000000000, 0.9431089717075972212, 1.000000000000000000),
 ( 1.000000000000000000, 0.9446123105951095278, 1.000000000000000000),
 ( 1.000000000000000000, 0.9578370004751587397, 1.000000000000000000),
 ( 1.000000000000000000, 0.9674308273347622666, 1.000000000000000000),
 ( 1.000000000000000000, 0.9828254127553104347, 1.000000000000000000),
 ( 1.000000000000000000, 0.9886239107120774472, 1.000000000000000000),
 ( 1.000000000000000000, 0.9967564037641253316, 1.000000000000000000),
 ( 1.000000000000000000, 0.9990872413564623189, 1.000000000000000000),
 ( 1.000000000000000000, 0.9997813423572990965, 1.000000000000000000) ) ) 
 REPRESENTATION_ITEM ( '' )  SURFACE ( )  );
#23219=FACE_OUTER_BOUND ( 'NONE', #9056, .T. ) ;
#23221=AXIS2_PLACEMENT_3D ( 'NONE', #15127, #17251, #2502 ) ;
#23223=CARTESIAN_POINT ( 'NONE',  ( -77.90255099906777048, -8.064892378658553795, -20.29001641120655464 ) ) ;
#23224=CARTESIAN_POINT ( 'NONE',  ( 184.8905102610680444, 14.79361573936375507, 14.79361573936398067 ) ) ;
#23225=CARTESIAN_POINT ( 'NONE',  ( -77.55640685876515761, -15.64922766773196905, -15.64922766773223195 ) ) ;
#23226=CARTESIAN_POINT ( 'NONE',  ( 184.8905102610680444, 2.362515690532070066E-13, -19.07866798485558490 ) ) ;
#23227=CARTESIAN_POINT ( 'NONE',  ( -96.93773665438786225, -8.190703376741039321, 20.92028269119429496 ) ) ;
#23228=CARTESIAN_POINT ( 'NONE',  ( -30.26275506840324070, -1.694272468446265112, 0.000000000000000000 ) ) ;
#23229=CARTESIAN_POINT ( 'NONE',  ( 163.1118516004056573, -37.29075403953139300, -19.27778845539249630 ) ) ;
#23233=CARTESIAN_POINT ( 'NONE',  ( 200.0000000000000000, 39.99999999999999289, 20.00000000000007105 ) ) ;
#23235=CARTESIAN_POINT ( 'NONE',  ( 4.995406935893288214, 15.24977328854832770, 0.000000000000000000 ) ) ;
#23236=CARTESIAN_POINT ( 'NONE',  ( -192.9588430854690273, -18.05360324515454096, 38.51493924976936967 ) ) ;
#23237=CARTESIAN_POINT ( 'NONE',  ( 199.9999999999999432, -20.00000000000006750, 0.000000000000000000 ) ) ;
#23238=VERTEX_POINT ( 'NONE', #1345 ) ;
#23239=CARTESIAN_POINT ( 'NONE',  ( 22.72189371636348554, -43.05215026464009043, 23.48424859981480495 ) ) ;
#23240=CARTESIAN_POINT ( 'NONE',  ( -238.4067589809705794, 40.96449428006337001, -40.00000000000002132 ) ) ;
#23242=AXIS2_PLACEMENT_3D ( 'NONE', #12779, #16764, #12915 ) ;
#23244=CARTESIAN_POINT ( 'NONE',  ( 146.6084372240433993, 3.800685668858676980, 3.800685668858667210 ) ) ;
#23245=CARTESIAN_POINT ( 'NONE',  ( -208.1127848780264742, -40.00000000000011369, 15.00245453012655439 ) ) ;
#23246=CARTESIAN_POINT ( 'NONE',  ( -77.62680886784242773, 21.74967759987069371, 3.755764534306124336 ) ) ;
#23247=CARTESIAN_POINT ( 'NONE',  ( 23.37394308801976806, -13.80096434448233111, -46.80823611210209378 ) ) ;
#23249=CARTESIAN_POINT ( 'NONE',  ( -135.8532207217289738, -6.472252184284280396, 6.472252184284099208 ) ) ;
#23250=CARTESIAN_POINT ( 'NONE',  ( -86.86493150571051558, -19.77569912838786337, 7.943527260504712473 ) ) ;
#23252=CARTESIAN_POINT ( 'NONE',  ( -238.4067589809705794, -0.6820004457913680929, 0.6820004457913170226 ) ) ;
#23253=CARTESIAN_POINT ( 'NONE',  ( 163.1118516004056573, -2.556006622855449647E-13, 27.26290988616872824 ) ) ;
#23254=CARTESIAN_POINT ( 'NONE',  ( -208.1127848780265026, -10.60833733269551971, 10.60833733269537049 ) ) ;
#23255=CARTESIAN_POINT ( 'NONE',  ( -87.02115643451061544, 10.85297647555737299, -18.51269039639787906 ) ) ;
#23256=CARTESIAN_POINT ( 'NONE',  ( -198.0356074513804572, 17.40982414986501325, -39.15871834505897198 ) ) ;
#23257=CARTESIAN_POINT ( 'NONE',  ( 57.59792236341147031, 1.722363176415040886, 1.722363176415060426 ) ) ;
#23258=CARTESIAN_POINT ( 'NONE',  ( -86.96347745069644475, 41.18208027870576871, 15.38646221621837107 ) ) ;
#23259=CARTESIAN_POINT ( 'NONE',  ( -30.26275506840324070, 1.198031551616724366, -57.76657404653984429 ) ) ;
#23260=CARTESIAN_POINT ( 'NONE',  ( 91.82158438592158234, 22.79471317813472453, -40.00000000000002132 ) ) ;
#23261=CARTESIAN_POINT ( 'NONE',  ( -280.0000000000000000, -14.14213562373098831, -14.14213562373098654 ) ) ;
#23263=CARTESIAN_POINT ( 'NONE',  ( -213.1075012329537230, -8.703598725189323045E-14, 13.71589010951911902 ) ) ;
#23264=CARTESIAN_POINT ( 'NONE',  ( -198.0356074513804572, -39.15871834505931304, 17.40982414986437377 ) ) ;
#23265=CARTESIAN_POINT ( 'NONE',  ( -187.3036811847508716, 46.64553187114688626, -13.75782060302973164 ) ) ;
#23267=CARTESIAN_POINT ( 'NONE',  ( -56.48582580120559271, 21.81201906317768291, 21.81201906317777173 ) ) ;
#23268=CARTESIAN_POINT ( 'NONE',  ( -99.29480781227208297, -20.80016781325152664, -8.165122821357817529 ) ) ;
#23269=CARTESIAN_POINT ( 'NONE',  ( 0.2972598230769923355, 18.14793986248697166, 38.42060263243675422 ) ) ;
#23270=CARTESIAN_POINT ( 'NONE',  ( -16.37606550806730610, -39.75508062642441587, -16.46709356883193109 ) ) ;
#23272=CARTESIAN_POINT ( 'NONE',  ( -166.3490444791802929, -36.43931842067700444, 19.13701437385558535 ) ) ;
#23274=CARTESIAN_POINT ( 'NONE',  ( 23.54890483848385330, -23.30407993985125259, 42.80335737019169073 ) ) ;
#23275=CARTESIAN_POINT ( 'NONE',  ( 170.2234770963711128, -24.55285855007184281, -40.00000000000002132 ) ) ;
#23276=CARTESIAN_POINT ( 'NONE',  ( 44.65795722941690116, 15.21593185910654000, -36.73450905838434721 ) ) ;
#23278=CARTESIAN_POINT ( 'NONE',  ( -56.48582580120559982, -21.81201906317804173, 34.75652343174591152 ) ) ;
#23279=CARTESIAN_POINT ( 'NONE',  ( 163.1118516004056573, 40.00000000000014921, -27.26290988616858968 ) ) ;
#23281=CARTESIAN_POINT ( 'NONE',  ( -200.0000000000000853, -24.82633483071228753, -44.86878812508721381 ) ) ;
#23282=CARTESIAN_POINT ( 'NONE',  ( 146.6084372240433709, -5.374981219216942385, -40.00000000000002132 ) ) ;
#23283=CARTESIAN_POINT ( 'NONE',  ( 22.75856136761844795, -17.88529938203868497, -43.17893233522190144 ) ) ;
#23285=CARTESIAN_POINT ( 'NONE',  ( -208.1127848780264742, -15.00245453012673202, 40.00000000000002132 ) ) ;
#23286=CARTESIAN_POINT ( 'NONE',  ( 0.2972598230769923355, 18.14793986248697166, 38.42060263243675422 ) ) ;
#23287=CARTESIAN_POINT ( 'NONE',  ( 0.2972598230769956662, 40.00000000000058975, -54.33493731733894094 ) ) ;
#23288=CARTESIAN_POINT ( 'NONE',  ( -114.4364955367327354, 8.644468109209578088, -20.04994829327644723 ) ) ;
#23289=CARTESIAN_POINT ( 'NONE',  ( -135.8532207217289738, -40.00000000000014211, 9.153146818113153671 ) ) ;
#23291=CARTESIAN_POINT ( 'NONE',  ( 164.1121284987796969, -24.38383377897543980, -10.10011465390285323 ) ) ;
#23293=CARTESIAN_POINT ( 'NONE',  ( -198.0356074513804572, -10.87444709760996986, 67.44298959253333692 ) ) ;
#23294=ORIENTED_EDGE ( 'NONE', *, *, #25019, .F. ) ;
#23296=CARTESIAN_POINT ( 'NONE',  ( -4.915070467874492088, 46.68718905935151753, -13.76630780994186765 ) ) ;
#23297=CARTESIAN_POINT ( 'NONE',  ( 91.82158438592156813, 17.20528682183302038, 40.00000000000002132 ) ) ;
#23299=CARTESIAN_POINT ( 'NONE',  ( -200.4317933031551320, 49.29858032309928717, -14.17468109412842914 ) ) ;
#23302=ORIENTED_EDGE ( 'NONE', *, *, #23310, .F. ) ;
#23303=CARTESIAN_POINT ( 'NONE',  ( 0.2972598230769976091, -10.13633138497479180, 10.13633138497468522 ) ) ;
#23305=CARTESIAN_POINT ( 'NONE',  ( 146.6084372240433993, 1.478241399363601114E-13, -34.62501878078305850 ) ) ;
#23310=EDGE_CURVE ( 'NONE', #11587, #17229, #10150, .T. ) ;
#23311=CARTESIAN_POINT ( 'NONE',  ( 91.82158438592158234, -12.16597498400057198, 44.40256751092329779 ) ) ;
#23313=CARTESIAN_POINT ( 'NONE',  ( 0.2972598230769956662, 39.99999999999983658, 54.33493731733950938 ) ) ;
#23318=CARTESIAN_POINT ( 'NONE',  ( 19.06497207195982924, -39.99999999999945288, -54.19242893257885640 ) ) ;
#23319=CARTESIAN_POINT ( 'NONE',  ( 130.8568914410475372, 8.880724697947696879E-14, -5.949712681206690945 ) ) ;
#23320=CARTESIAN_POINT ( 'NONE',  ( 14.38125909742181285, -10.73282306404727393, 10.73282306404716380 ) ) ;
#23322=CARTESIAN_POINT ( 'NONE',  ( -200.4317933031552457, 14.17468109412838295, 49.29858032309917348 ) ) ;
#23324=AXIS2_PLACEMENT_3D ( 'NONE', #18049, #3834, #3695 ) ;
#23327=CARTESIAN_POINT ( 'NONE',  ( -82.25678930351507745, -16.86921253968544221, 11.09265870503258000 ) ) ;
#23328=( BOUNDED_SURFACE ( )  B_SPLINE_SURFACE ( 3, 3, ( 
 ( #17995, #20002, #9892, #11132, #17242, #8874, #22717, #18991, #23249, #22854, #6475, #13002, #20854, #25120, #10605, #14852, #10743, #18717, #2767, #10876, #13131, #6872, #4494, #14589, #12597, #14986, #14722, #4629, #22988, #18854 ),
 ( #4893, #634, #502, #6602, #24850, #20726, #23120, #8609, #2634, #21250, #2494, #19116, #16718, #12732, #12868, #8740, #16858, #5024, #24989, #6997, #21122, #768, #15118, #6740, #4764, #3025, #16984, #19246, #20986, #1028 ),
 ( #2900, #11006, #899, #9010, #17116, #25246, #9127, #25686, #12206, #9942, #18050, #5685, #26203, #20327, #17784, #7939, #1705, #16057, #20064, #24048, #12071, #5825, #13789, #13927, #10078, #6219, #3835, #25929, #11937, #1840 ),
 ( #22199, #24327, #14066, #5957, #3974, #2104, #4107, #17918, #24183, #22063, #20190, #14332, #22330, #23909, #10213, #1972, #15914, #21925, #1575, #18318, #4243, #18183, #26333, #8074, #9678, #101, #16193, #9813, #6091, #14198 ),
 ( #8208, #16326, #24454, #7669, #3697, #22463, #12333, #15782, #11802, #26061, #19922, #7799, #2773, #4770, #20732, #18860, #16863, #229, #6481, #12602, #14464, #4499, #2500, #8880, #2364, #10611, #4372, #8343, #12875, #6876 ),
 ( #774, #20858, #10343, #4899, #18453, #2641, #10478, #18592, #18723, #14593, #507, #20589, #10749, #16991, #12738, #370, #24588, #25126, #8613, #16464, #20991, #16724, #24855, #6607, #14727, #22859, #6748, #14992, #6344, #20461 ),
 ( #641, #4636, #10883, #22595, #12462, #18997, #8745, #23127, #8474, #2235, #16592, #24724, #24995, #22722, #14860, #22994, #15379, #3280, #3156, #23502, #11137, #2905, #1415, #9267, #23382, #7137, #19631, #19499, #5156, #5276 ) ),
 .UNSPECIFIED., .T., .F., .T. ) 
 B_SPLINE_SURFACE_WITH_KNOTS ( ( 4, 3, 4 ),
 ( 4, 2, 2, 2, 2, 2, 2, 2, 2, 2, 2, 2, 2, 2, 4 ),
 ( 0.000000000000000000, 0.5000000000000000000, 1.000000000000000000 ),
 ( 0.000000000000000000, 0.1357259735107005372, 0.1651108541090157700, 0.1944957347073310028, 0.3598804999793158710, 0.3867117631979620773, 0.4135430264166082281, 0.5789277916885930964, 0.6062785021374117456, 0.6336292125862302838, 0.8508620842112317728, 0.8814014469398914198, 0.9119408096685510667, 0.9559704048342755334, 1.000000000000000000 ),
 .UNSPECIFIED. ) 
 GEOMETRIC_REPRESENTATION_ITEM ( )  RATIONAL_B_SPLINE_SURFACE ( (
 ( 1.000000000000000000, 1.000000000000000000, 1.000000000000000000, 1.000000000000000000, 1.000000000000000000, 1.000000000000000000, 1.000000000000000000, 1.000000000000000000, 1.000000000000000000, 1.000000000000000000, 1.000000000000000000, 1.000000000000000000, 1.000000000000000000, 1.000000000000000000, 1.000000000000000000, 1.000000000000000000, 1.000000000000000000, 1.000000000000000000, 1.000000000000000000, 1.000000000000000000, 1.000000000000000000, 1.000000000000000000, 1.000000000000000000, 1.000000000000000000, 1.000000000000000000, 1.000000000000000000, 1.000000000000000000, 1.000000000000000000, 1.000000000000000000, 1.000000000000000000),
 ( 0.3333333333333333703, 0.3333333333333333703, 0.3333333333333333703, 0.3333333333333333703, 0.3333333333333333703, 0.3333333333333333703, 0.3333333333333333703, 0.3333333333333333703, 0.3333333333333333703, 0.3333333333333333703, 0.3333333333333333703, 0.3333333333333333703, 0.3333333333333333703, 0.3333333333333333703, 0.3333333333333333703, 0.3333333333333333703, 0.3333333333333333703, 0.3333333333333333703, 0.3333333333333333703, 0.3333333333333333703, 0.3333333333333333703, 0.3333333333333333703, 0.3333333333333333703, 0.3333333333333333703, 0.3333333333333333703, 0.3333333333333333703, 0.3333333333333333703, 0.3333333333333333703, 0.3333333333333333703, 0.3333333333333333703),
 ( 0.3333333333333333703, 0.3333333333333333703, 0.3333333333333333703, 0.3333333333333333703, 0.3333333333333333703, 0.3333333333333333703, 0.3333333333333333703, 0.3333333333333333703, 0.3333333333333333703, 0.3333333333333333703, 0.3333333333333333703, 0.3333333333333333703, 0.3333333333333333703, 0.3333333333333333703, 0.3333333333333333703, 0.3333333333333333703, 0.3333333333333333703, 0.3333333333333333703, 0.3333333333333333703, 0.3333333333333333703, 0.3333333333333333703, 0.3333333333333333703, 0.3333333333333333703, 0.3333333333333333703, 0.3333333333333333703, 0.3333333333333333703, 0.3333333333333333703, 0.3333333333333333703, 0.3333333333333333703, 0.3333333333333333703),
 ( 1.000000000000000000, 1.000000000000000000, 1.000000000000000000, 1.000000000000000000, 1.000000000000000000, 1.000000000000000000, 1.000000000000000000, 1.000000000000000000, 1.000000000000000000, 1.000000000000000000, 1.000000000000000000, 1.000000000000000000, 1.000000000000000000, 1.000000000000000000, 1.000000000000000000, 1.000000000000000000, 1.000000000000000000, 1.000000000000000000, 1.000000000000000000, 1.000000000000000000, 1.000000000000000000, 1.000000000000000000, 1.000000000000000000, 1.000000000000000000, 1.000000000000000000, 1.000000000000000000, 1.000000000000000000, 1.000000000000000000, 1.000000000000000000, 1.000000000000000000),
 ( 0.3333333333333333703, 0.3333333333333333703, 0.3333333333333333703, 0.3333333333333333703, 0.3333333333333333703, 0.3333333333333333703, 0.3333333333333333703, 0.3333333333333333703, 0.3333333333333333703, 0.3333333333333333703, 0.3333333333333333703, 0.3333333333333333703, 0.3333333333333333703, 0.3333333333333333703, 0.3333333333333333703, 0.3333333333333333703, 0.3333333333333333703, 0.3333333333333333703, 0.3333333333333333703, 0.3333333333333333703, 0.3333333333333333703, 0.3333333333333333703, 0.3333333333333333703, 0.3333333333333333703, 0.3333333333333333703, 0.3333333333333333703, 0.3333333333333333703, 0.3333333333333333703, 0.3333333333333333703, 0.3333333333333333703),
 ( 0.3333333333333333703, 0.3333333333333333703, 0.3333333333333333703, 0.3333333333333333703, 0.3333333333333333703, 0.3333333333333333703, 0.3333333333333333703, 0.3333333333333333703, 0.3333333333333333703, 0.3333333333333333703, 0.3333333333333333703, 0.3333333333333333703, 0.3333333333333333703, 0.3333333333333333703, 0.3333333333333333703, 0.3333333333333333703, 0.3333333333333333703, 0.3333333333333333703, 0.3333333333333333703, 0.3333333333333333703, 0.3333333333333333703, 0.3333333333333333703, 0.3333333333333333703, 0.3333333333333333703, 0.3333333333333333703, 0.3333333333333333703, 0.3333333333333333703, 0.3333333333333333703, 0.3333333333333333703, 0.3333333333333333703),
 ( 1.000000000000000000, 1.000000000000000000, 1.000000000000000000, 1.000000000000000000, 1.000000000000000000, 1.000000000000000000, 1.000000000000000000, 1.000000000000000000, 1.000000000000000000, 1.000000000000000000, 1.000000000000000000, 1.000000000000000000, 1.000000000000000000, 1.000000000000000000, 1.000000000000000000, 1.000000000000000000, 1.000000000000000000, 1.000000000000000000, 1.000000000000000000, 1.000000000000000000, 1.000000000000000000, 1.000000000000000000, 1.000000000000000000, 1.000000000000000000, 1.000000000000000000, 1.000000000000000000, 1.000000000000000000, 1.000000000000000000, 1.000000000000000000, 1.000000000000000000) ) ) 
 REPRESENTATION_ITEM ( '' )  SURFACE ( )  );
#23329=CARTESIAN_POINT ( 'NONE',  ( 200.0000000000000000, -42.42640687119290988, 14.14213562373064903 ) ) ;
#23332=VERTEX_POINT ( 'NONE', #9321 ) ;
#23333=CARTESIAN_POINT ( 'NONE',  ( -91.56559293963834989, -16.03295912088659492, -40.53558337403696044 ) ) ;
#23336=ORIENTED_EDGE ( 'NONE', *, *, #379, .F. ) ;
#23337=CARTESIAN_POINT ( 'NONE',  ( 91.82158438592158234, 2.580785920671402147E-13, -22.79471317813470321 ) ) ;
#23340=ORIENTED_EDGE ( 'NONE', *, *, #22659, .F. ) ;
#23341=ORIENTED_EDGE ( 'NONE', *, *, #10932, .T. ) ;
#23342=CARTESIAN_POINT ( 'NONE',  ( 163.1118516004056573, 12.73709011382478273, 2.449293598294708485E-15 ) ) ;
#23343=CARTESIAN_POINT ( 'NONE',  ( -100.0957100001013913, -20.56213589528242736, -8.517115559121256396 ) ) ;
#23344=AXIS2_PLACEMENT_3D ( 'NONE', #20963, #10986, #2744 ) ;
#23345=PRODUCT_DEFINITION_CONTEXT ( 'detailed design', #24315, 'design' ) ;
#23347=CARTESIAN_POINT ( 'NONE',  ( -138.9613193425336988, -10.11110876495216537, 29.42718875726419014 ) ) ;
#23348=CARTESIAN_POINT ( 'NONE',  ( -198.0356074513804572, -9.007331120208026888E-14, 15.37879056873070560 ) ) ;
#23350=CARTESIAN_POINT ( 'NONE',  ( -77.78738561284504271, 9.951797149076110571, 19.58913667614457310 ) ) ;
#23351=CARTESIAN_POINT ( 'NONE',  ( 57.59792236341147031, -1.722363176415055985, 1.722363176415024677 ) ) ;
#23352=CARTESIAN_POINT ( 'NONE',  ( -213.1075012329537230, -9.698598906462304825, -66.26714140138675191 ) ) ;
#23353=CARTESIAN_POINT ( 'NONE',  ( -114.7826396787322665, -15.64922767586157981, -15.64922767586183383 ) ) ;
#23354=CARTESIAN_POINT ( 'NONE',  ( 146.6084372240433993, 8.568076647504290689E-14, -5.374981219216972583 ) ) ;
#23356=CARTESIAN_POINT ( 'NONE',  ( 163.1118516004056573, 27.26290988616876021, -40.00000000000002132 ) ) ;
#23357=CARTESIAN_POINT ( 'NONE',  ( 19.06497207195982924, -66.60410523465823474, 10.03556273973400081 ) ) ;
#23358=CARTESIAN_POINT ( 'NONE',  ( 192.4448373802101173, 20.00000000003945644, -40.00000000000002132 ) ) ;
#23360=CARTESIAN_POINT ( 'NONE',  ( -105.3755690713226585, 40.00000000000007816, -21.75974354311636461 ) ) ;
#23361=CARTESIAN_POINT ( 'NONE',  ( 151.7948205124836534, -33.23291073765550863, -40.00000000000002132 ) ) ;
#23362=CARTESIAN_POINT ( 'NONE',  ( 14.38125909742181285, -17.55144818341476309, 39.01709431150910490 ) ) ;
#23363=CARTESIAN_POINT ( 'NONE',  ( 151.7948205124836250, 6.767089262349059275, 2.449293598294708485E-15 ) ) ;
#23366=CARTESIAN_POINT ( 'NONE',  ( -4.004886986944963922, -47.00296421444941330, 13.82996668233338156 ) ) ;
#23367=CARTESIAN_POINT ( 'NONE',  ( -162.0762913951020892, 41.69427287692678163, -40.00000000000002132 ) ) ;
#23368=CARTESIAN_POINT ( 'NONE',  ( -87.10563802237723507, -13.14174799571811825, 16.99650074895399854 ) ) ;
#23370=CARTESIAN_POINT ( 'NONE',  ( -100.7734535825088500, -16.03295912088716335, 40.53558337403673306 ) ) ;
#23371=CARTESIAN_POINT ( 'NONE',  ( -100.7734535825088358, 6.065416334915073333E-14, -22.67402823373191723 ) ) ;
#23373=CARTESIAN_POINT ( 'NONE',  ( -8.255580677153719904, 13.52904896325820339, -45.52720393890008665 ) ) ;
#23375=EDGE_CURVE ( 'NONE', #12261, #3577, #18149, .T. ) ;
#23377=CARTESIAN_POINT ( 'NONE',  ( -77.58512834294195670, -2.776851935584524256, -21.97396063739902061 ) ) ;
#23378=CARTESIAN_POINT ( 'NONE',  ( 0.2972598230769886718, 38.42060263243643448, 18.14793986248763957 ) ) ;
#23379=CARTESIAN_POINT ( 'NONE',  ( -91.56559293963836410, 44.31723036834908669, -12.25131212657445801 ) ) ;
#23381=CARTESIAN_POINT ( 'NONE',  ( 91.82158438592159655, 12.16597498400028776, 44.40256751092339016 ) ) ;
#23382=CARTESIAN_POINT ( 'NONE',  ( 151.7948205124836250, -23.49921654116371883, 23.49921654116317526 ) ) ;
#23383=CARTESIAN_POINT ( 'NONE',  ( -208.1127848780264742, 17.67593391476678377, -38.89260858015718014 ) ) ;
#23384=CARTESIAN_POINT ( 'NONE',  ( 136.1360204305621266, 53.05693388239320285, -3.511608612530223716 ) ) ;
#23385=CARTESIAN_POINT ( 'NONE',  ( -91.56559293963834989, -44.31723036834885932, -12.25131212657538171 ) ) ;
#23386=CARTESIAN_POINT ( 'NONE',  ( -259.2033419157646676, 21.55415060305860209, -21.55415060305812602 ) ) ;
#23387=CARTESIAN_POINT ( 'NONE',  ( -105.3755690713226585, -21.75974354311652448, -40.00000000000002132 ) ) ;
#23389=CARTESIAN_POINT ( 'NONE',  ( -86.96347745069644475, 5.999880687339585546E-14, -21.75974354311649961 ) ) ;
#23390=CARTESIAN_POINT ( 'NONE',  ( 170.2234770963711128, -39.20704971665404059, 17.36149277826957160 ) ) ;
#23391=FACE_OUTER_BOUND ( 'NONE', #15807, .T. ) ;
#23393=CARTESIAN_POINT ( 'NONE',  ( 14.38125909742181108, 39.01709431150907648, 39.01709431150921858 ) ) ;
#23394=CARTESIAN_POINT ( 'NONE',  ( -196.0240759113457045, 24.63338926175158861, 44.60678620512894099 ) ) ;
#23395=CARTESIAN_POINT ( 'NONE',  ( 9.006212071497531113, 24.85331907609986501, 44.90541342374595501 ) ) ;
#23396=CARTESIAN_POINT ( 'NONE',  ( -16.87994666116949460, -39.19724034060761397, -20.93785811911747530 ) ) ;
#23397=ORIENTED_EDGE ( 'NONE', *, *, #306, .T. ) ;
#23398=CARTESIAN_POINT ( 'NONE',  ( -184.9729924864286659, -42.02333070177691354, 22.80024897330345368 ) ) ;
#23401=CARTESIAN_POINT ( 'NONE',  ( 23.10188454848764650, -23.40120037233781147, 42.94013537404170222 ) ) ;
#23403=CARTESIAN_POINT ( 'NONE',  ( 73.43374752933530658, 26.88866000079776342, -12.96823637283455355 ) ) ;
#23405=CARTESIAN_POINT ( 'NONE',  ( -86.94483050222758891, 20.27470715367157794, 6.877769850676278551 ) ) ;
#23406=CARTESIAN_POINT ( 'NONE',  ( -30.26275506840324070, -1.147469862568086380E-14, 1.694272468446259783 ) ) ;
#23407=CARTESIAN_POINT ( 'NONE',  ( -86.95456146551094889, -6.703401383518407641, 20.33691291319591699 ) ) ;
#23409=CARTESIAN_POINT ( 'NONE',  ( 130.8568914410475088, -5.949712681206664300, -40.00000000000002132 ) ) ;
#23410=CARTESIAN_POINT ( 'NONE',  ( 23.35901252181223597, -13.80180065670210432, -46.81387818480128260 ) ) ;
#23412=CARTESIAN_POINT ( 'NONE',  ( 4.995406935893309530, -55.24977328856464709, 40.00000000000002132 ) ) ;
#23413=CARTESIAN_POINT ( 'NONE',  ( -100.7734535825088500, 44.31723036834890905, 12.25131212657507795 ) ) ;
#23415=CARTESIAN_POINT ( 'NONE',  ( 19.06497207195979726, 40.00000000000017053, -14.19242893257798599 ) ) ;
#23416=CARTESIAN_POINT ( 'NONE',  ( -30.26275506840324070, -40.00000000000001421, -1.694272468446678559 ) ) ;
#23420=CARTESIAN_POINT ( 'NONE',  ( -77.56334768864770979, 1.373422545953698615, -22.09347816142257059 ) ) ;
#23421=CARTESIAN_POINT ( 'NONE',  ( -0.5869797817588224831, 43.96874597319774836, -18.21245090264383393 ) ) ;
#23422=CARTESIAN_POINT ( 'NONE',  ( 200.0000000000000000, -19.99999999999989342, 40.00000000000002132 ) ) ;
#23423=CARTESIAN_POINT ( 'NONE',  ( -189.1288337602927641, 43.24060467048765588, -23.62383291543576647 ) ) ;
#23426=CARTESIAN_POINT ( 'NONE',  ( 91.82158438592158234, 12.16597498397773869, -12.16597498397759303 ) ) ;
#23427=CARTESIAN_POINT ( 'NONE',  ( 90.71511022959295190, -21.07400258556058503, -9.285713565094647848 ) ) ;
#23429=EDGE_LOOP ( 'NONE', ( #1466, #24608, #19083, #8972 ) ) ;
#23433=CARTESIAN_POINT ( 'NONE',  ( -86.96347745069644475, 41.18208027870598187, -15.38646221621779731 ) ) ;
#23434=CARTESIAN_POINT ( 'NONE',  ( -114.4364955367326502, -20.04994829327650052, -8.644468109209421769 ) ) ;
#23435=CARTESIAN_POINT ( 'NONE',  ( 23.37394308801977871, -46.80823611210205115, 13.80096434448272724 ) ) ;
#23436=CARTESIAN_POINT ( 'NONE',  ( -188.7701102708081748, -23.55033952083662285, 43.14144101424771804 ) ) ;
#23438=CARTESIAN_POINT ( 'NONE',  ( 136.1360204305621551, -39.99999999999994316, -4.966164525587488221 ) ) ;
#23439=CARTESIAN_POINT ( 'NONE',  ( -135.8532207217289738, 3.005970985514575011E-13, -30.84685318188645553 ) ) ;
#23441=CARTESIAN_POINT ( 'NONE',  ( -198.0356074513804572, -67.44298959250878056, 10.87444709758448447 ) ) ;
#23442=CARTESIAN_POINT ( 'NONE',  ( 170.2234770963711128, 40.00000000000014211, -24.55285855007172913 ) ) ;
#23443=FACE_OUTER_BOUND ( 'NONE', #4945, .T. ) ;
#23444=CARTESIAN_POINT ( 'NONE',  ( -100.0753760173605258, 8.149786832858509911, 20.72827493166407464 ) ) ;
#23445=ADVANCED_FACE ( 'NONE', ( #23806 ), #25475, .T. ) ;
#23448=CARTESIAN_POINT ( 'NONE',  ( -77.56593252305926001, 22.07939426011869344, 1.556858787764804353 ) ) ;
#23449=CARTESIAN_POINT ( 'NONE',  ( -56.48582580120559271, 21.81201906317768291, 21.81201906317777173 ) ) ;
#23451=CARTESIAN_POINT ( 'NONE',  ( -30.26275506840324070, -29.48230279907817675, 27.08623969584564151 ) ) ;
#23452=CARTESIAN_POINT ( 'NONE',  ( -187.7699188115162769, -13.79076593539094553, -46.80708926513509027 ) ) ;
#23453=CARTESIAN_POINT ( 'NONE',  ( -105.2054292635175727, 15.19799821370213522, 15.19799821370241943 ) ) ;
#23454=EDGE_LOOP ( 'NONE', ( #19202, #16151, #23206, #13342 ) ) ;
#23455=CARTESIAN_POINT ( 'NONE',  ( 4.995406935893297984, 10.78321810390233892, -67.35176059882522281 ) ) ;
#23456=ADVANCED_FACE ( 'NONE', ( #25858 ), #20014, .T. ) ;
#23459=VERTEX_POINT ( 'NONE', #13207 ) ;
#23461=CARTESIAN_POINT ( 'NONE',  ( 199.9999999999999432, -1.727494763561684666E-13, 20.00000000000010303 ) ) ;
#23464=CARTESIAN_POINT ( 'NONE',  ( 22.27781863250965344, -43.19367102557750115, 23.58928354728861976 ) ) ;
#23467=CARTESIAN_POINT ( 'NONE',  ( -208.1127848780264742, -38.89260858015728672, -17.67593391476669851 ) ) ;
#23468=CARTESIAN_POINT ( 'NONE',  ( -213.1075012329537230, 39.99999999999992895, 13.71589010951925935 ) ) ;
#23469=CARTESIAN_POINT ( 'NONE',  ( 169.9999999999674571, -17.64300463372919836, -17.64300463252165585 ) ) ;
#23471=DIRECTION ( 'NONE',  ( -1.836970198721030181E-16, 1.000000000000000000, 0.000000000000000000 ) ) ;
#23472=CARTESIAN_POINT ( 'NONE',  ( -192.9588430854689989, -8.596193650988133061E-14, 14.46834944099969533 ) ) ;
#23474=CARTESIAN_POINT ( 'NONE',  ( -82.23726319252905625, 13.38816311965448946, 15.17212531852062085 ) ) ;
#23475=CARTESIAN_POINT ( 'NONE',  ( 199.9999999999999432, -14.14213562373115884, 14.14213562373085153 ) ) ;
#23476=CARTESIAN_POINT ( 'NONE',  ( 91.82158438592156813, 40.45024623143973486, -16.11829626348390931 ) ) ;
#23478=CARTESIAN_POINT ( 'NONE',  ( 199.9999999999999432, 2.486775779033024914E-13, -19.99999999999992539 ) ) ;
#23479=CARTESIAN_POINT ( 'NONE',  ( 98.29820294273291381, -18.47759065023123526, -7.653668647304108674 ) ) ;
#23480=CARTESIAN_POINT ( 'NONE',  ( 146.6084372240433709, 34.62501878078307982, 40.00000000000002132 ) ) ;
#23481=CARTESIAN_POINT ( 'NONE',  ( 57.59792236341147031, 2.435789363418170872, -40.00000000000002132 ) ) ;
#23482=CARTESIAN_POINT ( 'NONE',  ( -208.1127848780264742, 17.67593391476624021, 38.89260858015742883 ) ) ;
#23483=CARTESIAN_POINT ( 'NONE',  ( -56.48582580120558561, -30.84685318188645553, -40.00000000000002132 ) ) ;
#23484=CARTESIAN_POINT ( 'NONE',  ( -30.26275506840325136, 40.00000000000001421, 1.694272468446399227 ) ) ;
#23485=CARTESIAN_POINT ( 'NONE',  ( 170.2234770963711128, -2.259079968736224833E-13, 24.55285855007187124 ) ) ;
#23486=CARTESIAN_POINT ( 'NONE',  ( 4.995406935893287326, 67.35176059882533650, 10.78321810390163549 ) ) ;
#23487=ADVANCED_FACE ( 'NONE', ( #11082, #19196 ), #6948, .T. ) ;
#23488=CARTESIAN_POINT ( 'NONE',  ( -259.2033419157646676, 30.48217210827735713, -40.00000000000002132 ) ) ;
#23490=CARTESIAN_POINT ( 'NONE',  ( 22.17571259161115194, -43.20787961119348353, 23.59965736305207429 ) ) ;
#23491=CARTESIAN_POINT ( 'NONE',  ( -87.13361725327075646, -15.19799821270861706, 15.19799821270823159 ) ) ;
#23492=CARTESIAN_POINT ( 'NONE',  ( 184.8905102610680444, -14.79361573936389540, 41.77492675555996016 ) ) ;
#23494=CARTESIAN_POINT ( 'NONE',  ( -82.25596499887640789, 19.79010929774564076, -3.998483074826426176 ) ) ;
#23495=CARTESIAN_POINT ( 'NONE',  ( -24.53392603775155578, 12.34411287782940292, -39.81639166318235823 ) ) ;
#23499=CARTESIAN_POINT ( 'NONE',  ( -259.2033419157646676, 21.55415060305790931, 35.01439189186571355 ) ) ;
#23500=CARTESIAN_POINT ( 'NONE',  ( 19.06497207195981858, -10.03556273973377166, -66.60410523465827737 ) ) ;
#23501=CARTESIAN_POINT ( 'NONE',  ( 57.59792236341147031, 30.00663442387683588, 26.56190807104703211 ) ) ;
#23502=CARTESIAN_POINT ( 'NONE',  ( 57.59792236341147031, -1.722363176415055985, 1.722363176415024677 ) ) ;
#23503=CARTESIAN_POINT ( 'NONE',  ( 57.59792236341147031, 30.00663442387720181, -26.56190807104661289 ) ) ;
#23504=CARTESIAN_POINT ( 'NONE',  ( -208.1127848780264742, -38.89260858015704514, -38.89260858015768463 ) ) ;
#23505=CARTESIAN_POINT ( 'NONE',  ( 91.82158438592158234, -12.16597498399995203, -44.40256751092347542 ) ) ;
#23506=CARTESIAN_POINT ( 'NONE',  ( -192.9588430854690273, 10.23066800229588758, -66.79921049721882298 ) ) ;
#23507=CARTESIAN_POINT ( 'NONE',  ( -114.7826396787323091, -1.398623183117054136, -22.13135001986807993 ) ) ;
#23509=CARTESIAN_POINT ( 'NONE',  ( -30.26275506840324070, -1.147469862568086380E-14, 1.694272468446259783 ) ) ;
#23510=CARTESIAN_POINT ( 'NONE',  ( 163.1118516004056573, -9.006482792074626431, 47.56205970284951690 ) ) ;
#23511=CARTESIAN_POINT ( 'NONE',  ( -208.1127848780264742, 55.00245453014418473, 40.00000000000002132 ) ) ;
#23513=CARTESIAN_POINT ( 'NONE',  ( -162.0762913951021176, 29.48230308784768638, -27.08623940707612121 ) ) ;
#23514=B_SPLINE_CURVE_WITH_KNOTS ( 'NONE', 3,
 ( #13426, #4951, #954, #11422, #7177, #9061 ),
 .UNSPECIFIED., .F., .F.,
 ( 4, 2, 4 ),
 ( 0.000000000000000000, 0.004168007559015109859, 0.008336015118030219717 ),
 .UNSPECIFIED. ) ;
#23515=( BOUNDED_CURVE ( )  B_SPLINE_CURVE ( 3, ( #23114, #4886, #21114, #3018 ),
 .UNSPECIFIED., .F., .F. ) 
 B_SPLINE_CURVE_WITH_KNOTS ( ( 4, 4 ),
 ( 0.01388163287021749320, 0.02359082919309987009 ),
 .UNSPECIFIED. ) 
 CURVE ( )  GEOMETRIC_REPRESENTATION_ITEM ( )  RATIONAL_B_SPLINE_CURVE ( ( 1.000000000000000000, 0.8672072324488975248, 0.7608653435686167921, 0.6809743333591576908 ) ) 
 REPRESENTATION_ITEM ( '' )  );
#23516=CARTESIAN_POINT ( 'NONE',  ( -87.02159130206896975, -18.50869357302490315, -10.86091765595724468 ) ) ;
#23517=CARTESIAN_POINT ( 'NONE',  ( 23.64688638900135587, 23.28414885118118249, 42.77321027809743725 ) ) ;
#23518=CARTESIAN_POINT ( 'NONE',  ( -39.58644176650890500, -32.83087322311865819, -13.59899295362217764 ) ) ;
#23520=CARTESIAN_POINT ( 'NONE',  ( -183.1090696430980529, -41.47043467734991395, 22.43564075026454319 ) ) ;
#23522=CARTESIAN_POINT ( 'NONE',  ( 45.01779936585140263, -12.15764947731424250, 38.89115870265484176 ) ) ;
#23526=CARTESIAN_POINT ( 'NONE',  ( -99.29480781227181296, -20.48155342677142698, -8.934325994365357460 ) ) ;
#23527=CARTESIAN_POINT ( 'NONE',  ( -280.0000000000000568, 40.00000000000004263, -19.99999999999987210 ) ) ;
#23528=DIRECTION ( 'NONE',  ( 0.9698969544100581874, -0.09318942523027390346, 0.2249791742614079271 ) ) ;
#23529=CARTESIAN_POINT ( 'NONE',  ( -199.9999999999999716, -14.89048929005484467, -48.59548038928831915 ) ) ;
#23530=CARTESIAN_POINT ( 'NONE',  ( -86.96347745069643054, -18.24025645688353947, 40.00000000000002132 ) ) ;
#23531=CARTESIAN_POINT ( 'NONE',  ( 83.01683444512164556, -9.947410331075138501, -24.01517293243385609 ) ) ;
#23533=CARTESIAN_POINT ( 'NONE',  ( -135.8532207217289738, 9.153146818113548022, 40.00000000000002132 ) ) ;
#23534=CARTESIAN_POINT ( 'NONE',  ( -238.4067589809705794, -0.6820004457913680929, 0.6820004457913170226 ) ) ;
#23535=CARTESIAN_POINT ( 'NONE',  ( 192.4448373802100889, -1.741373372144848397E-13, 20.00000000003942091 ) ) ;
#23536=CARTESIAN_POINT ( 'NONE',  ( 184.8905102610680444, -39.99999999999978684, -19.07866798485600768 ) ) ;
#23539=EDGE_LOOP ( 'NONE', ( #22948, #14086, #15337, #13524, #16648, #13648, #19702, #8091 ) ) ;
#23540=CARTESIAN_POINT ( 'NONE',  ( 98.29820294267349823, 10.02182676112789217, -17.32045324915450379 ) ) ;
#23541=CARTESIAN_POINT ( 'NONE',  ( -3.494657986428189922, 43.29048295385600653, -17.93150516116771342 ) ) ;
#23542=CARTESIAN_POINT ( 'NONE',  ( -86.96347745069645896, 21.75974354311648895, 40.00000000000002132 ) ) ;
#23545=CARTESIAN_POINT ( 'NONE',  ( -192.1963514251025913, 43.96876056338943783, -24.16258207727797824 ) ) ;
#23548=ORIENTED_EDGE ( 'NONE', *, *, #21119, .F. ) ;
#23549=CARTESIAN_POINT ( 'NONE',  ( 151.7948205124836250, 23.49921654116361225, -23.49921654116333514 ) ) ;
#23550=CARTESIAN_POINT ( 'NONE',  ( 144.1620285550791891, 12.51613133675877876, -30.21661402164554744 ) ) ;
#23551=CARTESIAN_POINT ( 'NONE',  ( -188.2995950289364089, 43.00522595870987885, -23.44932284465868477 ) ) ;
#23554=CARTESIAN_POINT ( 'NONE',  ( -192.1166648175283740, 14.00295691731063386, 48.16216898722862538 ) ) ;
#23555=CARTESIAN_POINT ( 'NONE',  ( -198.0356074513804572, 39.15871834505901461, 39.15871834505919935 ) ) ;
#23557=CARTESIAN_POINT ( 'NONE',  ( -238.4067589809705794, -4.716212492215116094E-14, 0.9644942799825824142 ) ) ;
#23561=CARTESIAN_POINT ( 'NONE',  ( -238.4067589809705794, -40.00000000000005684, -0.9644942799830014124 ) ) ;
#23562=CARTESIAN_POINT ( 'NONE',  ( 170.2234770963711128, 40.00000000000021316, -15.44714144992773797 ) ) ;
#23563=CARTESIAN_POINT ( 'NONE',  ( -86.84055334702942730, 19.72499881414481493, 8.026593896031025466 ) ) ;
#23564=CARTESIAN_POINT ( 'NONE',  ( 151.7948205124836250, 23.49921654116361225, -23.49921654116333514 ) ) ;
#23565=CARTESIAN_POINT ( 'NONE',  ( -198.0356074513804572, -9.007331120208026888E-14, 15.37879056873070560 ) ) ;
#23566=CARTESIAN_POINT ( 'NONE',  ( -259.2033419157646676, 6.730120644403521979, -6.730120644403498886 ) ) ;
#23567=CARTESIAN_POINT ( 'NONE',  ( -109.1264249741457490, -13.72187187121248364, 33.12752917270315578 ) ) ;
#23568=B_SPLINE_CURVE_WITH_KNOTS ( 'NONE', 3,
 ( #13133, #2769, #8876, #10878, #18993, #3026, #25509, #1030, #17753, #11503 ),
 .UNSPECIFIED., .F., .F.,
 ( 4, 2, 2, 2, 4 ),
 ( 0.7921542097164080420, 0.8508620842112317728, 0.8814014469398914198, 0.9119408096685510667, 0.9406682828395580565 ),
 .UNSPECIFIED. ) ;
#23571=CARTESIAN_POINT ( 'NONE',  ( -82.28266731793512179, -17.99064928892019211, 9.155589012557189932 ) ) ;
#23572=CARTESIAN_POINT ( 'NONE',  ( 0.2972598230770011618, 10.13633138497462305, 66.70487387989858519 ) ) ;
#23573=CARTESIAN_POINT ( 'NONE',  ( -100.7734535825088500, -12.25131212657524316, 44.31723036834888774 ) ) ;
#23575=DIRECTION ( 'NONE',  ( 0.2259624730582988905, 0.9741360073261728925, 0.000000000000000000 ) ) ;
#23577=CARTESIAN_POINT ( 'NONE',  ( 136.1360204305621266, 3.511608612530757068, -3.511608612530642937 ) ) ;
#23581=CARTESIAN_POINT ( 'NONE',  ( -86.96347745069643054, -40.00000000000026290, 21.75974354311608749 ) ) ;
#23583=CARTESIAN_POINT ( 'NONE',  ( -70.35386311745469357, 10.19784241653377777, 22.51194464762888003 ) ) ;
#23586=CARTESIAN_POINT ( 'NONE',  ( -192.9588430854689989, -10.23066800230756890, 10.23066800230742501 ) ) ;
#23587=CARTESIAN_POINT ( 'NONE',  ( 192.4448373802100889, -3.692737725850373501E-14, 19.99999999996060751 ) ) ;
#23588=CARTESIAN_POINT ( 'NONE',  ( -105.2054292635175869, 15.19799821370233062, -15.19799821370219206 ) ) ;
#23589=EDGE_CURVE ( 'NONE', #9969, #9873, #5429, .T. ) ;
#23591=CARTESIAN_POINT ( 'NONE',  ( 130.8568914410475088, -40.00000000000001421, 5.949712681206549725 ) ) ;
#23594=CARTESIAN_POINT ( 'NONE',  ( 19.06497207195981147, -4.605042221739098431E-14, 14.19242893257840521 ) ) ;
#23596=CARTESIAN_POINT ( 'NONE',  ( 19.06497207195980792, 10.03556273973447155, -10.03556273973422286 ) ) ;
#23597=CARTESIAN_POINT ( 'NONE',  ( -162.0762913951021176, 27.08623940707639477, -29.48230308784743059 ) ) ;
#23599=CARTESIAN_POINT ( 'NONE',  ( 19.06497207195981858, 5.735870351258996432E-13, -54.19242893257843008 ) ) ;
#23601=CARTESIAN_POINT ( 'NONE',  ( 146.6084372240433709, -5.374981219216948602, 40.00000000000002132 ) ) ;
#23602=CARTESIAN_POINT ( 'NONE',  ( -259.2033419157646676, 9.517827891722582478, -40.00000000000002132 ) ) ;
#23603=CARTESIAN_POINT ( 'NONE',  ( 4.995406935893287326, 17.50105314357170627, 39.06748935135200895 ) ) ;
#23604=CARTESIAN_POINT ( 'NONE',  ( 184.8905102610680444, 20.92133201514447549, 0.000000000000000000 ) ) ;
#23605=CARTESIAN_POINT ( 'NONE',  ( -105.3841681040955933, 6.699016078400306107, 20.33889746609499838 ) ) ;
#23607=CARTESIAN_POINT ( 'NONE',  ( 130.8568914410475372, -3.326198072800416995E-13, 34.05028731879788495 ) ) ;
#23608=CARTESIAN_POINT ( 'NONE',  ( 199.9999999999999432, 14.14213562373090838, 14.14213562373092437 ) ) ;
#23609=CARTESIAN_POINT ( 'NONE',  ( -100.7734535825088500, 17.32597176626809699, -40.00000000000002132 ) ) ;
#23611=CARTESIAN_POINT ( 'NONE',  ( 25.62979979008006381, -45.99287499155195746, 13.63460241477595325 ) ) ;
#23613=ADVANCED_FACE ( 'NONE', ( #25839 ), #2157, .T. ) ;
#23614=CARTESIAN_POINT ( 'NONE',  ( -213.1075012329537230, 9.698598906462684965, 66.26714140138669507 ) ) ;
#23616=CARTESIAN_POINT ( 'NONE',  ( -86.93367134006987840, 20.20393068805329762, 7.058177991699935205 ) ) ;
#23619=EDGE_CURVE ( 'NONE', #25051, #13654, #10199, .T. ) ;
#23620=CARTESIAN_POINT ( 'NONE',  ( -77.78739057084328579, -20.88856886083027575, -6.814681957699006531 ) ) ;
#23622=CARTESIAN_POINT ( 'NONE',  ( -87.05569247515344955, -4.389928423847803352, -20.98769100332471638 ) ) ;
#23623=CARTESIAN_POINT ( 'NONE',  ( -162.0762913951020892, 1.198031840385732849, -1.198031840385733515 ) ) ;
#23624=CARTESIAN_POINT ( 'NONE',  ( -162.0762913951020892, -1.198031840315659124, -57.76657433523998009 ) ) ;
#23625=CARTESIAN_POINT ( 'NONE',  ( -114.7760651468638571, 22.09554796279716626, -1.204233200294609896 ) ) ;
#23626=FACE_OUTER_BOUND ( 'NONE', #24648, .T. ) ;
#23627=CARTESIAN_POINT ( 'NONE',  ( -162.0762913951020892, -1.198031840315659124, -57.76657433523998009 ) ) ;
#23628=CARTESIAN_POINT ( 'NONE',  ( -192.9588430854690273, -10.23066800231931239, -66.79921049724377724 ) ) ;
#23629=CARTESIAN_POINT ( 'NONE',  ( 91.82158438592158234, -40.45024623143936537, -16.11829626348475131 ) ) ;
#23630=CARTESIAN_POINT ( 'NONE',  ( -56.48582580120559271, 21.81201906317798489, -21.81201906317746619 ) ) ;
#23631=CARTESIAN_POINT ( 'NONE',  ( -208.1127848780265026, -10.60833733269551971, 10.60833733269537049 ) ) ;
#23632=CARTESIAN_POINT ( 'NONE',  ( 136.1360204305621266, 35.03383547441298873, 0.000000000000000000 ) ) ;
#23633=CARTESIAN_POINT ( 'NONE',  ( 136.1360204305621551, -39.99999999999987921, -35.03383547441310242 ) ) ;
#23635=CARTESIAN_POINT ( 'NONE',  ( 146.6084372240433709, -34.62501878078303008, 40.00000000000002132 ) ) ;
#23638=CARTESIAN_POINT ( 'NONE',  ( 163.1118516004056573, 37.29075403953160617, -19.27778845539222985 ) ) ;
#23639=AXIS2_PLACEMENT_3D ( 'NONE', #15876, #4070, #24005 ) ;
#23640=CARTESIAN_POINT ( 'NONE',  ( 22.63898026999810043, 42.29338810984155828, 17.51849495380543331 ) ) ;
#23641=CARTESIAN_POINT ( 'NONE',  ( 23.05038679986142469, 17.85133178553910582, 43.09692730307104824 ) ) ;
#23642=CARTESIAN_POINT ( 'NONE',  ( -7.297127544327485893, -45.86058602274801643, -13.59739983758753645 ) ) ;
#23643=VERTEX_POINT ( 'NONE', #7948 ) ;
#23644=CARTESIAN_POINT ( 'NONE',  ( -114.4364955367328207, -20.29001642038830155, 8.064892380842811903 ) ) ;
#23646=CARTESIAN_POINT ( 'NONE',  ( 44.65795722950328894, -15.21593185908468726, 36.73450905844209302 ) ) ;
#23647=CARTESIAN_POINT ( 'NONE',  ( 90.71511022963046855, 9.285713564076607085, -21.07400258596608822 ) ) ;
#23649=CARTESIAN_POINT ( 'NONE',  ( -103.9474983245028881, -19.92928099173742496, -8.577167319634591891 ) ) ;
#23650=CARTESIAN_POINT ( 'NONE',  ( 146.6084372240433709, 40.00000000000003553, 5.374981219217116468 ) ) ;
#23654=CARTESIAN_POINT ( 'NONE',  ( -86.96347745069645896, 21.75974354311648895, 40.00000000000002132 ) ) ;
#23655=CARTESIAN_POINT ( 'NONE',  ( 90.68848816889322961, -9.291443202883320041, -21.08311784352002505 ) ) ;
#23657=CARTESIAN_POINT ( 'NONE',  ( 192.4448373802101173, -19.99999999996057554, 40.00000000000002132 ) ) ;
#23658=CARTESIAN_POINT ( 'NONE',  ( 57.59792236341147031, 2.435789363418170872, -40.00000000000002132 ) ) ;
#23659=CARTESIAN_POINT ( 'NONE',  ( -91.56559293963834989, -22.67402823373193499, 0.000000000000000000 ) ) ;
#23660=CARTESIAN_POINT ( 'NONE',  ( -280.0000000000000568, 39.99999999999976552, 20.00000000000043343 ) ) ;
#23661=CARTESIAN_POINT ( 'NONE',  ( 199.9999999999999432, 2.486775779033024914E-13, -19.99999999999992539 ) ) ;
#23665=CARTESIAN_POINT ( 'NONE',  ( 1.925538622547987355, 48.64880301058932588, -14.07631154916797733 ) ) ;
#23666=CARTESIAN_POINT ( 'NONE',  ( 14.38125909742182884, -55.17850393971007605, 40.00000000000002132 ) ) ;
#23668=CARTESIAN_POINT ( 'NONE',  ( -188.6889827002243578, 47.12918603174835397, -13.84869468768081369 ) ) ;
#23672=CARTESIAN_POINT ( 'NONE',  ( -89.92902785008668332, 8.734793929541243784, -20.17328762787294139 ) ) ;
#23673=CARTESIAN_POINT ( 'NONE',  ( 135.5356265174576720, 12.51227922893905387, -30.20731421070341582 ) ) ;
#23675=CARTESIAN_POINT ( 'NONE',  ( -99.29480781227204034, 8.165122821357641669, -20.80016781325159414 ) ) ;
#23676=VERTEX_POINT ( 'NONE', #17660 ) ;
#23679=CARTESIAN_POINT ( 'NONE',  ( -208.1127848780264742, 67.17687982760683951, 10.60833733268317403 ) ) ;
#23681=CARTESIAN_POINT ( 'NONE',  ( 163.1118516004056573, 1.251511021549353291E-13, -27.26290988616872824 ) ) ;
#23682=CARTESIAN_POINT ( 'NONE',  ( -199.9999999999999716, -45.81998439131056244, 19.51623549979313665 ) ) ;
#23685=CARTESIAN_POINT ( 'NONE',  ( 146.6084372240433993, -3.357462877844280890E-13, 34.62501878078305850 ) ) ;
#23686=CARTESIAN_POINT ( 'NONE',  ( 146.6084372240433993, 8.568076647504290689E-14, -5.374981219216972583 ) ) ;
#23688=CARTESIAN_POINT ( 'NONE',  ( -110.0685463886661068, -10.00056106068391948, 17.53216629777173452 ) ) ;
#23689=CARTESIAN_POINT ( 'NONE',  ( -30.26275506840324070, -1.198031551616032919, 1.198031551616014712 ) ) ;
#23690=CARTESIAN_POINT ( 'NONE',  ( -199.9999999999999432, 14.17215463606722636, -49.28189405767596298 ) ) ;
#23691=CARTESIAN_POINT ( 'NONE',  ( -197.4154352061136137, 14.14666496778293592, 49.11380478893853052 ) ) ;
#23692=CARTESIAN_POINT ( 'NONE',  ( 110.0479209278586694, 22.74092928740047626, 9.419601331808811651 ) ) ;
#23694=CARTESIAN_POINT ( 'NONE',  ( 192.4448373802100889, 14.14213562375893574, -14.14213562375874922 ) ) ;
#23695=CARTESIAN_POINT ( 'NONE',  ( 130.8568914410475088, -39.99999999999988631, -34.05028731879802706 ) ) ;
#23696=CARTESIAN_POINT ( 'NONE',  ( 14.38125909742181285, -17.55144818341476309, 39.01709431150910490 ) ) ;
#23697=CARTESIAN_POINT ( 'NONE',  ( -105.3755690713226585, -41.18208027870611687, 15.38646221621750954 ) ) ;
#23699=CARTESIAN_POINT ( 'NONE',  ( -77.70103689343427789, 11.20642775818909520, 18.98727594172718725 ) ) ;
#23700=ORIENTED_EDGE ( 'NONE', *, *, #2591, .F. ) ;
#23701=CARTESIAN_POINT ( 'NONE',  ( 192.4448373802101173, 42.42640687116487896, 14.14213562375934075 ) ) ;
#23703=B_SPLINE_CURVE_WITH_KNOTS ( 'NONE', 3,
 ( #5493, #9613, #26127, #19593, #17848, #25998 ),
 .UNSPECIFIED., .F., .F.,
 ( 4, 2, 4 ),
 ( -0.0001050551439130371028, 0.04006379722394161347, 0.08023264959179625400 ),
 .UNSPECIFIED. ) ;
#23706=CARTESIAN_POINT ( 'NONE',  ( -238.4067589809705794, -3.369206980223063916E-14, -0.9644942799825824142 ) ) ;
#23708=CARTESIAN_POINT ( 'NONE',  ( 21.16156876808018694, -43.48822901267196528, 23.80729322913559187 ) ) ;
#23711=CARTESIAN_POINT ( 'NONE',  ( -100.7734535825088500, 16.03295912088713848, -16.03295912088698927 ) ) ;
#23712=CARTESIAN_POINT ( 'NONE',  ( 170.2234770963711128, -2.511315425431857630E-14, 15.44714144992816074 ) ) ;
#23714=DIRECTION ( 'NONE',  ( 0.01051738792039888168, -0.3656191332797650295, -0.9307051272723736446 ) ) ;
#23716=CARTESIAN_POINT ( 'NONE',  ( 4.995406935893305089, -40.00000000000021316, 55.24977328853194791 ) ) ;
#23718=CARTESIAN_POINT ( 'NONE',  ( 151.7948205124836534, 40.00000000000017053, -33.23291073765538783 ) ) ;
#23720=CARTESIAN_POINT ( 'NONE',  ( -86.96347745069644475, -15.38646221621807442, 15.38646221621768184 ) ) ;
#23721=CARTESIAN_POINT ( 'NONE',  ( -91.56559293963834989, 16.03295912088740849, -40.53558337403661938 ) ) ;
#23722=CARTESIAN_POINT ( 'NONE',  ( -87.04503123322947999, -18.12276621389172959, 11.46092073712200232 ) ) ;
#23723=CARTESIAN_POINT ( 'NONE',  ( 163.1118516004056573, -2.556006622855449647E-13, 27.26290988616872824 ) ) ;
#23725=CARTESIAN_POINT ( 'NONE',  ( -105.3755690713226869, 21.75974354311648540, -0.000000000000000000 ) ) ;
#23726=CARTESIAN_POINT ( 'NONE',  ( 200.0000000000000000, -19.99999999999988631, -40.00000000000002132 ) ) ;
#23727=CARTESIAN_POINT ( 'NONE',  ( 4.995406935893293543, -10.78321810389005364, 10.78321810388994173 ) ) ;
#23728=CARTESIAN_POINT ( 'NONE',  ( -56.48582580120559271, 9.153146818113576444, -0.000000000000000000 ) ) ;
#23729=CARTESIAN_POINT ( 'NONE',  ( -105.4053751741942335, 19.27722189457469781, 9.295450928565532678 ) ) ;
#23730=CARTESIAN_POINT ( 'NONE',  ( -259.2033419157646676, -1.473088368616265084E-13, 9.517827891722632216 ) ) ;
#23731=CARTESIAN_POINT ( 'NONE',  ( -100.7734535825088500, 40.53558337403677569, -16.03295912088699993 ) ) ;
#23732=CARTESIAN_POINT ( 'NONE',  ( 91.82158438592158234, 22.79471317813472453, -40.00000000000002132 ) ) ;
#23735=CARTESIAN_POINT ( 'NONE',  ( 23.38399212876576527, -46.80460545930662875, 13.80022400692479501 ) ) ;
#23736=CARTESIAN_POINT ( 'NONE',  ( 110.0479209278586836, 9.419601331808605593, 22.74092928740057218 ) ) ;
#23737=CARTESIAN_POINT ( 'NONE',  ( -162.0762913951021176, 29.48230308784768638, -27.08623940707612121 ) ) ;
#23738=CARTESIAN_POINT ( 'NONE',  ( -56.48582580120557850, -40.00000000000014211, 30.84685318188629921 ) ) ;
#23739=CARTESIAN_POINT ( 'NONE',  ( 130.8568914410475088, 4.207082182989012153, 52.36146031193425188 ) ) ;
#23740=CARTESIAN_POINT ( 'NONE',  ( -100.7734535825088500, -22.67402823373193499, -40.00000000000002132 ) ) ;
#23743=CARTESIAN_POINT ( 'NONE',  ( 169.9999999999999716, -19.80854622259151654, 15.47746304364889447 ) ) ;
#23744=CARTESIAN_POINT ( 'NONE',  ( -30.26275506840325136, 29.48230279907760121, 27.08623969584625613 ) ) ;
#23745=CARTESIAN_POINT ( 'NONE',  ( -91.56559293963834989, 16.03295912088740849, -40.53558337403661938 ) ) ;
#23746=CARTESIAN_POINT ( 'NONE',  ( 170.2234770963711128, 17.36149277827004411, -17.36149277826983095 ) ) ;
#23748=CARTESIAN_POINT ( 'NONE',  ( 192.4448373802101173, 42.42640687122089815, -14.14213562370272470 ) ) ;
#23749=CARTESIAN_POINT ( 'NONE',  ( 91.82158438592159655, 12.16597498400091304, -44.40256751092321963 ) ) ;
#23750=CARTESIAN_POINT ( 'NONE',  ( -280.0000000000000568, -42.42640687119276066, -14.14213562373147148 ) ) ;
#23751=CARTESIAN_POINT ( 'NONE',  ( 14.38125909742180752, 10.73282306404735387, -10.73282306404708919 ) ) ;
#23753=CARTESIAN_POINT ( 'NONE',  ( -114.6379872168154890, -5.502324066487487286, -21.35005244387444989 ) ) ;
#23756=CARTESIAN_POINT ( 'NONE',  ( -208.1127848780264742, -40.00000000000025580, 55.00245453014408525 ) ) ;
#23757=CARTESIAN_POINT ( 'NONE',  ( 4.995406935893301537, -10.78321810390187530, 67.35176059882529387 ) ) ;
#23759=CARTESIAN_POINT ( 'NONE',  ( -198.0356074513804572, 55.37879056873070027, 2.449293598294708485E-15 ) ) ;
#23760=VERTEX_POINT ( 'NONE', #2375 ) ;
#23761=CARTESIAN_POINT ( 'NONE',  ( -238.4067589809705794, 0.6820004457912757223, 0.6820004457913219076 ) ) ;
#23762=ADVANCED_FACE ( 'NONE', ( #24864 ), #16443, .T. ) ;
#23763=CARTESIAN_POINT ( 'NONE',  ( -48.88328292457690338, 29.77915576935907183, 12.33493019568957649 ) ) ;
#23764=CARTESIAN_POINT ( 'NONE',  ( -77.90255099906769942, -8.064892378657791738, -20.29001641120690635 ) ) ;
#23765=CARTESIAN_POINT ( 'NONE',  ( 14.38125909742180752, 15.17850393972634038, 0.000000000000000000 ) ) ;
#23766=EDGE_CURVE ( 'NONE', #23081, #17509, #18452, .T. ) ;
#23767=EDGE_CURVE ( 'NONE', #25051, #10094, #19704, .T. ) ;
#23768=ORIENTED_EDGE ( 'NONE', *, *, #7837, .T. ) ;
#23769=CARTESIAN_POINT ( 'NONE',  ( -192.9370391625363936, -48.35015248261021270, 14.03127550871790419 ) ) ;
#23771=CARTESIAN_POINT ( 'NONE',  ( 23.39921416754910055, -13.79910252519578862, 46.79910576274385647 ) ) ;
#23773=CARTESIAN_POINT ( 'NONE',  ( 11.59303701476897253, 18.58252782964011374, -44.86219070953460175 ) ) ;
#23775=CARTESIAN_POINT ( 'NONE',  ( -94.58366989427298677, -20.58370269626831117, -9.000605044545542555 ) ) ;
#23776=CARTESIAN_POINT ( 'NONE',  ( -192.9588430854689989, -8.596193650988133061E-14, 14.46834944099969533 ) ) ;
#23777=CARTESIAN_POINT ( 'NONE',  ( 192.4448373802100889, 1.051811698935164031E-13, -20.00000000003942091 ) ) ;
#23779=CARTESIAN_POINT ( 'NONE',  ( -162.0762913951021176, -1.694272876828353702, 40.00000000000002132 ) ) ;
#23781=CARTESIAN_POINT ( 'NONE',  ( -183.6285492668827999, 17.34367427885824142, -41.87133366543424273 ) ) ;
#23783=CARTESIAN_POINT ( 'NONE',  ( -259.2033419157646676, -6.730120644403663199, 6.730120644403451813 ) ) ;
#23784=CARTESIAN_POINT ( 'NONE',  ( -91.56559293963834989, -17.32597176626812185, -40.00000000000002132 ) ) ;
#23785=CARTESIAN_POINT ( 'NONE',  ( 200.0000000000000000, -20.00000000000006750, 40.00000000000002132 ) ) ;
#23786=CARTESIAN_POINT ( 'NONE',  ( 0.2972598230770103767, -39.99999999999945288, -54.33493731733979359 ) ) ;
#23787=CARTESIAN_POINT ( 'NONE',  ( -192.9588430854689989, 1.161019517985663313E-13, -14.46834944099969533 ) ) ;
#23791=CARTESIAN_POINT ( 'NONE',  ( -208.1127848780265026, 10.60833733269537049, 10.60833733269544510 ) ) ;
#23793=CARTESIAN_POINT ( 'NONE',  ( -89.91498783732308198, -8.733585467820335069, 20.17141720494836221 ) ) ;
#23795=ORIENTED_EDGE ( 'NONE', *, *, #26073, .F. ) ;
#23796=ORIENTED_EDGE ( 'NONE', *, *, #5649, .T. ) ;
#23797=CARTESIAN_POINT ( 'NONE',  ( -238.4067589809705794, -0.6820004457913680929, 0.6820004457913170226 ) ) ;
#23798=CARTESIAN_POINT ( 'NONE',  ( 147.2817042152898068, 12.35516179550147520, -29.82799917201316475 ) ) ;
#23800=CARTESIAN_POINT ( 'NONE',  ( 200.0000000000000000, 19.99999999999996447, -40.00000000000002132 ) ) ;
#23801=FACE_OUTER_BOUND ( 'NONE', #2167, .T. ) ;
#23805=CARTESIAN_POINT ( 'NONE',  ( 19.06497207195980792, 66.60410523465817789, 10.03556273973446800 ) ) ;
#23806=FACE_OUTER_BOUND ( 'NONE', #3229, .T. ) ;
#23807=CARTESIAN_POINT ( 'NONE',  ( -213.1075012329537230, -8.703598725189323045E-14, 13.71589010951911902 ) ) ;
#23808=CARTESIAN_POINT ( 'NONE',  ( 14.33519811653600939, -14.14278418308700758, 49.08818492847921533 ) ) ;
#23809=DIRECTION ( 'NONE',  ( 0.000000000000000000, 1.000000000000000000, 0.000000000000000000 ) ) ;
#23811=CARTESIAN_POINT ( 'NONE',  ( -100.7734535825088358, -2.560096224687585342E-13, 22.67402823373191723 ) ) ;
#23812=CARTESIAN_POINT ( 'NONE',  ( -213.1075012329537230, 1.045191102001431893E-13, -13.71589010951911902 ) ) ;
#23813=CARTESIAN_POINT ( 'NONE',  ( -105.3239292022655320, -10.85048923515416952, 18.46172643730481511 ) ) ;
#23814=CARTESIAN_POINT ( 'NONE',  ( -259.2033419157646676, -21.55415060305824326, -35.01439189186556433 ) ) ;
#23815=CARTESIAN_POINT ( 'NONE',  ( 199.9999999999999432, 1.065690307512836407E-13, -20.00000000000010303 ) ) ;
#23816=CARTESIAN_POINT ( 'NONE',  ( 130.8568914410475088, -32.49135343045460900, -24.07718906446924478 ) ) ;
#23817=CARTESIAN_POINT ( 'NONE',  ( -93.02511667906883019, 8.169918093965335970, 20.82219708225692401 ) ) ;
#23819=CARTESIAN_POINT ( 'NONE',  ( 57.59792236341146321, 40.00000000000000711, 2.435789363418579434 ) ) ;
#23820=CARTESIAN_POINT ( 'NONE',  ( 151.7948205124836250, 1.439163438361279259E-13, -33.23291073765553705 ) ) ;
#23821=CARTESIAN_POINT ( 'NONE',  ( 170.2234770963711128, -17.36149277826995885, 39.20704971665388427 ) ) ;
#23822=CARTESIAN_POINT ( 'NONE',  ( 136.1360204305621266, -3.511608612531119000, 53.05693388239312469 ) ) ;
#23823=CARTESIAN_POINT ( 'NONE',  ( -194.4222169614342590, -14.07715596671444658, -48.65437996132243370 ) ) ;
#23824=CARTESIAN_POINT ( 'NONE',  ( -259.2033419157646676, 6.730120644403521979, -6.730120644403498886 ) ) ;
#23825=ORIENTED_EDGE ( 'NONE', *, *, #18835, .F. ) ;
#23826=CARTESIAN_POINT ( 'NONE',  ( -280.0000000000000568, -14.14213562373049449, -42.42640687119305198 ) ) ;
#23828=CARTESIAN_POINT ( 'NONE',  ( -65.65510974524495680, 9.107311025939294424, -24.89665924127712060 ) ) ;
#23829=CARTESIAN_POINT ( 'NONE',  ( -213.1075012329537230, -18.58567234101102272, -37.98287015391260013 ) ) ;
#23830=CARTESIAN_POINT ( 'NONE',  ( -82.24465949240999407, 2.525178489058720110, 20.03613703210050545 ) ) ;
#23838=EDGE_LOOP ( 'NONE', ( #13428, #25343 ) ) ;
#23840=CARTESIAN_POINT ( 'NONE',  ( -259.2033419157646676, -9.517827891722680178, -40.00000000000002132 ) ) ;
#23841=CARTESIAN_POINT ( 'NONE',  ( -192.9370379452204816, -44.11033005023536191, -24.26711011077032154 ) ) ;
#23842=CARTESIAN_POINT ( 'NONE',  ( -100.7734535825088500, 40.00000000000008527, -22.67402823373177512 ) ) ;
#23844=B_SPLINE_CURVE_WITH_KNOTS ( 'NONE', 3,
 ( #8703, #14950, #6434, #22946, #18951, #10972, #17079, #20551, #8567, #23085, #16681, #2319, #10706, #10427, #596, #14552, #10835, #19082, #24812, #327, #18816, #12961, #24678, #8429, #16548, #22682, #12551, #20819, #16814, #22815, #20683, #14813, #10563, #25213 ),
 .UNSPECIFIED., .F., .F.,
 ( 4, 2, 2, 2, 2, 2, 2, 2, 2, 2, 2, 2, 2, 2, 2, 2, 4 ),
 ( -5.298243351211008199E-05, 0.01887868273877531602, 0.02834451532491905068, 0.03071097347145496786, 0.03307743161799088505, 0.03544388976452680223, 0.03781034791106271942, 0.04254326420413454685, 0.04727618049720638121, 0.04964263864374229146, 0.05200909679027820171, 0.05674201308334994587, 0.05910847122988582142, 0.06029170030315371409, 0.06147492937642162064, 0.06620784566949321215, 0.07567367825563638128 ),
 .UNSPECIFIED. ) ;
#23846=CARTESIAN_POINT ( 'NONE',  ( -91.56559293963836410, 39.99999999999976552, 22.67402823373234000 ) ) ;
#23850=CARTESIAN_POINT ( 'NONE',  ( -4.439300432586500200, -23.37136716947730619, -42.88738538954447677 ) ) ;
#23851=CARTESIAN_POINT ( 'NONE',  ( -30.26275506840325136, 27.08623969584614244, -29.48230279907770779 ) ) ;
#23853=CARTESIAN_POINT ( 'NONE',  ( -213.1075012329537230, 1.045191102001431893E-13, -13.71589010951911902 ) ) ;
#23854=CARTESIAN_POINT ( 'NONE',  ( -105.4288953903223671, -20.05883966465301782, -7.317865678945969954 ) ) ;
#23855=CARTESIAN_POINT ( 'NONE',  ( -30.26275506840324070, -1.694272468446265112, 0.000000000000000000 ) ) ;
#23856=CARTESIAN_POINT ( 'NONE',  ( 4.995406935893307754, -55.24977328854835434, -2.449293598294708485E-15 ) ) ;
#23858=CARTESIAN_POINT ( 'NONE',  ( -208.1127848780265026, -10.60833733269551971, 10.60833733269537049 ) ) ;
#23859=CARTESIAN_POINT ( 'NONE',  ( 146.6084372240433709, 34.62501878078307982, -40.00000000000002132 ) ) ;
#23860=FACE_OUTER_BOUND ( 'NONE', #10227, .T. ) ;
#23861=CARTESIAN_POINT ( 'NONE',  ( 151.7948205124836250, -3.202120068677277203E-13, 33.23291073765553705 ) ) ;
#23862=CARTESIAN_POINT ( 'NONE',  ( 130.8568914410475372, 4.207082182992862407, 4.207082182992856190 ) ) ;
#23864=CARTESIAN_POINT ( 'NONE',  ( 184.8905102610680444, 19.07866798485562043, 2.449293598294708485E-15 ) ) ;
#23865=ORIENTED_EDGE ( 'NONE', *, *, #18576, .T. ) ;
#23867=CARTESIAN_POINT ( 'NONE',  ( 22.98934664983286780, -43.11412319250639058, 17.85845455616057720 ) ) ;
#23869=DIRECTION ( 'NONE',  ( 0.000000000000000000, 1.000000000000000000, 0.000000000000000000 ) ) ;
#23870=CARTESIAN_POINT ( 'NONE',  ( 91.82158438592158234, 16.11829626348434630, -40.45024623143955012 ) ) ;
#23871=CARTESIAN_POINT ( 'NONE',  ( 146.6084372240433993, 5.715592784339989804E-15, 5.374981219216972583 ) ) ;
#23872=CARTESIAN_POINT ( 'NONE',  ( 136.1360204305621551, 3.511608612530062512, 53.05693388239318864 ) ) ;
#23873=CARTESIAN_POINT ( 'NONE',  ( 91.82158438592158234, -1.633484621919921769E-13, 17.20528682183300262 ) ) ;
#23874=CARTESIAN_POINT ( 'NONE',  ( -162.0762913951020892, 1.694272876828294194, 0.000000000000000000 ) ) ;
#23875=CARTESIAN_POINT ( 'NONE',  ( -114.4364955367323660, -8.064892380834915997, 20.29001642039123610 ) ) ;
#23877=CARTESIAN_POINT ( 'NONE',  ( -77.78761611107495355, 6.817130479269885690, -20.88739660331173198 ) ) ;
#23878=CARTESIAN_POINT ( 'NONE',  ( -238.4067589809705794, 0.6820004457912851592, -0.6820004457913123597 ) ) ;
#23879=CARTESIAN_POINT ( 'NONE',  ( 170.2234770963711128, 17.36149277827028925, -39.20704971665377059 ) ) ;
#23880=CARTESIAN_POINT ( 'NONE',  ( -110.0745364228914838, 19.60339732655324951, -4.981072281427304738 ) ) ;
#23881=CARTESIAN_POINT ( 'NONE',  ( -77.70933353447252045, 18.93828009115779665, -11.19441472886040145 ) ) ;
#23882=CARTESIAN_POINT ( 'NONE',  ( 170.2234770963711128, 45.64576402573196390, -10.92277846919159856 ) ) ;
#23883=CARTESIAN_POINT ( 'NONE',  ( 4.995406935893305977, -39.06748935135157552, -39.06748935135225764 ) ) ;
#23884=CARTESIAN_POINT ( 'NONE',  ( -238.4067589809705794, 0.6820004458491113475, -57.25054294077229144 ) ) ;
#23885=CARTESIAN_POINT ( 'NONE',  ( 163.1118516004056573, -19.27778845539181063, -37.29075403953176959 ) ) ;
#23887=CARTESIAN_POINT ( 'NONE',  ( 165.3321726438082351, 26.53500608755495094, 0.000000000000000000 ) ) ;
#23890=CARTESIAN_POINT ( 'NONE',  ( 136.1360204305621551, -40.00000000000001421, 4.966164525586921563 ) ) ;
#23891=CARTESIAN_POINT ( 'NONE',  ( 170.2234770963711128, 17.36149277826973503, 39.20704971665401217 ) ) ;
#23892=CARTESIAN_POINT ( 'NONE',  ( -86.96347745069644475, 15.38646221621772092, 15.38646221621800336 ) ) ;
#23893=CARTESIAN_POINT ( 'NONE',  ( -91.56559293963834989, -22.67402823373193499, 40.00000000000002132 ) ) ;
#23894=ORIENTED_EDGE ( 'NONE', *, *, #26226, .F. ) ;
#23895=CARTESIAN_POINT ( 'NONE',  ( -135.8532207217289738, 50.09629031063965243, -6.472252184284084109 ) ) ;
#23897=CARTESIAN_POINT ( 'NONE',  ( 22.89778847644965154, 17.86913359794376532, 43.13990468001245659 ) ) ;
#23898=CARTESIAN_POINT ( 'NONE',  ( 98.29820294267359770, -19.33391160836604783, -5.160908283052728862 ) ) ;
#23899=ORIENTED_EDGE ( 'NONE', *, *, #8523, .F. ) ;
#23902=CARTESIAN_POINT ( 'NONE',  ( -0.6848998193088060571, -24.09453515733104112, 43.87669161504448567 ) ) ;
#23904=CARTESIAN_POINT ( 'NONE',  ( 23.41418334855269023, 13.79799959793996678, -46.79369727367426179 ) ) ;
#23906=CARTESIAN_POINT ( 'NONE',  ( -77.70103891335998014, -5.501929570351923537, 21.35016180889197557 ) ) ;
#23909=CARTESIAN_POINT ( 'NONE',  ( -56.48582580120559271, 21.81201906317798489, -21.81201906317746619 ) ) ;
#23910=CARTESIAN_POINT ( 'NONE',  ( 192.4448373802100889, -19.99999999996057198, -2.449293598294708485E-15 ) ) ;
#23911=CARTESIAN_POINT ( 'NONE',  ( 44.82887508586490100, -12.17256213127418185, -38.96139886160057131 ) ) ;
#23914=CARTESIAN_POINT ( 'NONE',  ( -208.1127848780265026, 10.60833733269551615, -10.60833733269529766 ) ) ;
#23915=CARTESIAN_POINT ( 'NONE',  ( -162.0762913951021176, -1.694272876828353702, -40.00000000000002132 ) ) ;
#23916=CARTESIAN_POINT ( 'NONE',  ( -198.0356074513804572, 55.37879056871320671, 40.00000000000002132 ) ) ;
#23917=CARTESIAN_POINT ( 'NONE',  ( 0.2972598230770030492, 5.716321584140269555E-13, -54.33493731733936016 ) ) ;
#23920=CARTESIAN_POINT ( 'NONE',  ( -4.039451493210501454, 43.00522595894040734, -23.44932283416630270 ) ) ;
#23921=CARTESIAN_POINT ( 'NONE',  ( -135.8532207217289738, -6.472252184284190690, -6.472252184284188914 ) ) ;
#23923=CARTESIAN_POINT ( 'NONE',  ( -89.91646883264553480, -8.407637968170137199, 20.29783361038910883 ) ) ;
#23926=ORIENTED_EDGE ( 'NONE', *, *, #9954, .T. ) ;
#23927=CARTESIAN_POINT ( 'NONE',  ( -198.0356074513804572, -67.44298959250878056, 10.87444709758448447 ) ) ;
#23928=CARTESIAN_POINT ( 'NONE',  ( 23.48902902575167673, -46.76665409567426224, -13.79248457097946101 ) ) ;
#23929=ORIENTED_EDGE ( 'NONE', *, *, #43, .T. ) ;
#23930=CARTESIAN_POINT ( 'NONE',  ( 19.06497207195980792, 14.19242893257840699, -40.00000000000002132 ) ) ;
#23931=CARTESIAN_POINT ( 'NONE',  ( -86.86578273022429642, -19.68494377654087657, 8.153770686795153821 ) ) ;
#23934=CARTESIAN_POINT ( 'NONE',  ( -105.2109914857827420, 21.45686921896511734, -1.364328617316883818 ) ) ;
#23935=CARTESIAN_POINT ( 'NONE',  ( -213.1075012329537230, 37.98287015391228749, 37.98287015391245802 ) ) ;
#23936=CARTESIAN_POINT ( 'NONE',  ( -105.2276019182101550, -2.726932708308365427, -21.34775691551994115 ) ) ;
#23938=CARTESIAN_POINT ( 'NONE',  ( 199.9999999999999432, 1.065690307512836407E-13, -20.00000000000010303 ) ) ;
#23939=CARTESIAN_POINT ( 'NONE',  ( 91.82158438592158234, -17.20528682183298486, 40.00000000000002132 ) ) ;
#23941=SPHERICAL_SURFACE ( 'NONE', #8987, 15.00000000000000000 ) ;
#23944=CARTESIAN_POINT ( 'NONE',  ( 200.0000000000000000, -39.99999999999977973, -20.00000000000034817 ) ) ;
#23945=CARTESIAN_POINT ( 'NONE',  ( -105.3901353553839044, -9.627478968556738792, 19.08722479150669571 ) ) ;
#23946=CARTESIAN_POINT ( 'NONE',  ( -56.48582580120558561, -50.09629031063963112, -6.472252184284449150 ) ) ;
#23948=CARTESIAN_POINT ( 'NONE',  ( -91.56559293963836410, 22.67402823373190301, -40.00000000000002132 ) ) ;
#23950=CARTESIAN_POINT ( 'NONE',  ( 192.4448373802101173, -14.14213562370283128, -42.42640687122081999 ) ) ;
#23954=CARTESIAN_POINT ( 'NONE',  ( 91.82158438592158234, -1.633484621919921769E-13, 17.20528682183300262 ) ) ;
#23955=CARTESIAN_POINT ( 'NONE',  ( -198.0356074513804572, -40.00000000000011369, 15.37879056873056527 ) ) ;
#23956=CARTESIAN_POINT ( 'NONE',  ( 151.7948205124836250, 4.785054706301690608, 4.785054706301682614 ) ) ;
#23957=CARTESIAN_POINT ( 'NONE',  ( 91.82158438592156813, -16.11829626348459144, 40.45024623143943643 ) ) ;
#23958=CARTESIAN_POINT ( 'NONE',  ( -188.8948648269078490, -17.93710299892572380, -43.30399732969062399 ) ) ;
#23959=CARTESIAN_POINT ( 'NONE',  ( -238.4067589809705794, -28.96627169325313389, -27.60227080167074831 ) ) ;
#23960=VERTEX_POINT ( 'NONE', #1292 ) ;
#23961=CARTESIAN_POINT ( 'NONE',  ( 91.82158438592158234, -12.16597498397778843, 12.16597498397750954 ) ) ;
#23962=CARTESIAN_POINT ( 'NONE',  ( -280.0000000000000000, 14.14213562373098299, -14.14213562373088706 ) ) ;
#23963=CARTESIAN_POINT ( 'NONE',  ( -280.0000000000000568, 19.99999999999996092, -40.00000000000002132 ) ) ;
#23965=CARTESIAN_POINT ( 'NONE',  ( 136.1360204305621551, -53.05693388239309627, -3.511608612531332163 ) ) ;
#23966=DIRECTION ( 'NONE',  ( 0.3301743741142292299, 0.000000000000000000, -0.9439199556521077339 ) ) ;
#23969=CARTESIAN_POINT ( 'NONE',  ( 22.68416413276403176, -23.49220544186193038, 43.06288726621021823 ) ) ;
#23970=CARTESIAN_POINT ( 'NONE',  ( -5.152948516938606005, 13.74948675458142766, 46.60473671797301165 ) ) ;
#23974=CARTESIAN_POINT ( 'NONE',  ( -238.4067589809705794, 0.9644942799825385604, -40.00000000000002132 ) ) ;
#23975=CARTESIAN_POINT ( 'NONE',  ( -213.1075012329537230, -9.698598906450557777, 9.698598906450415669 ) ) ;
#23976=CARTESIAN_POINT ( 'NONE',  ( 4.995406935893283773, 39.99999999999997158, 15.24977328854846803 ) ) ;
#23977=CARTESIAN_POINT ( 'NONE',  ( -93.01741312767285308, -20.82169463880986626, -8.169811846216443740 ) ) ;
#23979=CARTESIAN_POINT ( 'NONE',  ( -100.7734535825088358, -2.560096224687585342E-13, 22.67402823373191723 ) ) ;
#23982=CARTESIAN_POINT ( 'NONE',  ( -199.9999999999999432, 43.68705981750494516, 18.09577267661451927 ) ) ;
#23983=CARTESIAN_POINT ( 'NONE',  ( 9.028290303189734800, -18.59346688788116353, -44.88859993223265832 ) ) ;
#23984=CARTESIAN_POINT ( 'NONE',  ( 14.38125909742183062, -67.30136555895943218, -10.73282306403629605 ) ) ;
#23985=CARTESIAN_POINT ( 'NONE',  ( -87.13361725327075646, 15.19799821270843765, 15.19799821270837015 ) ) ;
#23986=CARTESIAN_POINT ( 'NONE',  ( 192.4448373802101173, -14.14213562370283128, -42.42640687122081999 ) ) ;
#23987=CARTESIAN_POINT ( 'NONE',  ( -135.8532207217289738, -1.208299557080134822E-13, 9.153146818113572891 ) ) ;
#23988=CARTESIAN_POINT ( 'NONE',  ( 200.0000000000000000, 7.347880794884121511E-14, 0.000000000000000000 ) ) ;
#23990=CARTESIAN_POINT ( 'NONE',  ( 4.995406935893309530, -55.24977328856464709, 40.00000000000002132 ) ) ;
#23991=CARTESIAN_POINT ( 'NONE',  ( 200.0000000000000000, 14.14213562373083022, 42.42640687119289566 ) ) ;
#23992=CARTESIAN_POINT ( 'NONE',  ( -280.0000000000000000, -20.00000000000006750, -2.449293598294708485E-15 ) ) ;
#23993=CARTESIAN_POINT ( 'NONE',  ( 98.29820294273055481, 14.14213562373424971, 14.14213562373465294 ) ) ;
#23994=CARTESIAN_POINT ( 'NONE',  ( -114.5544872014192208, 20.90328437005500817, -6.783945353999890848 ) ) ;
#23995=CARTESIAN_POINT ( 'NONE',  ( 91.82158438592158234, 16.11829626348434630, -40.45024623143955012 ) ) ;
#23996=CARTESIAN_POINT ( 'NONE',  ( -91.56559293963834989, -22.67402823373193499, 0.000000000000000000 ) ) ;
#23998=CARTESIAN_POINT ( 'NONE',  ( 23.37583784646145091, -46.80752016581931940, 13.80085822091005099 ) ) ;
#23999=CARTESIAN_POINT ( 'NONE',  ( -114.4364955367323091, -20.29001642039124675, -8.064892380834873364 ) ) ;
#24000=CARTESIAN_POINT ( 'NONE',  ( 200.0000000000000000, 14.14213562373100608, -42.42640687119291698 ) ) ;
#24002=CARTESIAN_POINT ( 'NONE',  ( 163.1118516004056573, -40.00000000000003553, 12.73709011382460687 ) ) ;
#24004=CARTESIAN_POINT ( 'NONE',  ( -238.4067589809705794, 0.6820004457912851592, -0.6820004457913123597 ) ) ;
#24005=DIRECTION ( 'NONE',  ( 0.000000000000000000, 0.3656393565653410227, -0.9307566067079424688 ) ) ;
#24006=CARTESIAN_POINT ( 'NONE',  ( 19.06497207195980792, 14.19242893257840876, 0.000000000000000000 ) ) ;
#24010=CARTESIAN_POINT ( 'NONE',  ( 130.8568914410475088, 32.49135343045448820, 24.07718906446946860 ) ) ;
#24011=CARTESIAN_POINT ( 'NONE',  ( 0.2972598230770153171, -66.70487387989849992, -10.13633138497533004 ) ) ;
#24014=DIRECTION ( 'NONE',  ( -1.000000000000000000, -1.836970198721024264E-16, 0.000000000000000000 ) ) ;
#24015=CARTESIAN_POINT ( 'NONE',  ( -82.25988539629349816, 17.04081484591361217, -10.82485991171699879 ) ) ;
#24016=CARTESIAN_POINT ( 'NONE',  ( -91.56559293963834989, 16.03295912088740849, -40.53558337403661938 ) ) ;
#24017=CARTESIAN_POINT ( 'NONE',  ( 184.8905102610680444, -13.49065550809791603, -13.49065550809818781 ) ) ;
#24019=CARTESIAN_POINT ( 'NONE',  ( -208.1127848780265026, 10.60833733269551615, -10.60833733269529766 ) ) ;
#24020=CARTESIAN_POINT ( 'NONE',  ( -135.8532207217289738, 6.472252184284186249, -6.472252184284142729 ) ) ;
#24023=CARTESIAN_POINT ( 'NONE',  ( 14.38125909742181818, -40.00000000000007816, 15.17850393972619649 ) ) ;
#24024=CARTESIAN_POINT ( 'NONE',  ( 199.9999999999999432, -14.14213562373093680, 14.14213562373082311 ) ) ;
#24028=CARTESIAN_POINT ( 'NONE',  ( 163.1118516004056573, 12.73709011382477918, 40.00000000000002132 ) ) ;
#24030=CARTESIAN_POINT ( 'NONE',  ( 14.32711916788068329, -24.71075626504557121, -44.71189734681527739 ) ) ;
#24031=CARTESIAN_POINT ( 'NONE',  ( 24.02412737066820370, 41.95328616380271569, 17.37762011516664629 ) ) ;
#24033=CARTESIAN_POINT ( 'NONE',  ( -105.3755690713226727, -21.75974354311652093, 0.000000000000000000 ) ) ;
#24035=ORIENTED_EDGE ( 'NONE', *, *, #11656, .F. ) ;
#24041=CARTESIAN_POINT ( 'NONE',  ( 16.38602454705575795, -14.09104119325942328, 48.74566733940696395 ) ) ;
#24042=CARTESIAN_POINT ( 'NONE',  ( 22.92196489051228880, 13.82589419143594611, -46.97629733300941268 ) ) ;
#24045=CARTESIAN_POINT ( 'NONE',  ( -188.2995950289363805, 23.44932284466059969, -43.00522595870931752 ) ) ;
#24046=CARTESIAN_POINT ( 'NONE',  ( -183.1091233173814317, -22.43565125815695538, 41.47045062403629601 ) ) ;
#24047=( BOUNDED_SURFACE ( )  B_SPLINE_SURFACE ( 3, 2, ( 
 ( #10404, #6409, #26126 ),
 ( #14526, #15988, #24116 ),
 ( #10010, #26269, #8005 ),
 ( #16122, #4568, #6540 ),
 ( #12664, #436, #25054 ),
 ( #14788, #21051, #23058 ),
 ( #16785, #571, #12524 ),
 ( #24921, #15052, #20791 ),
 ( #9069, #22918, #10677 ),
 ( #8943, #2429, #19181 ),
 ( #17050, #8540, #4697 ),
 ( #12800, #16920, #10810 ),
 ( #8676, #17176, #2835 ),
 ( #20926, #13067, #4960 ),
 ( #2705, #16657, #25185 ),
 ( #6673, #6934, #18920 ) ),
 .UNSPECIFIED., .F., .F., .F. ) 
 B_SPLINE_SURFACE_WITH_KNOTS ( ( 4, 2, 2, 2, 2, 2, 2, 4 ),
 ( 3, 3 ),
 ( 0.04143342415521648198, 0.04844520227998382056, 0.05195109134236748638, 0.05545698040475115220, 0.06246875852951849079, 0.06422170306071033063, 0.06597464759190216355, 0.06948053665428582937 ),
 ( 0.000000000000000000, 1.000000000000000000 ),
 .UNSPECIFIED. ) 
 GEOMETRIC_REPRESENTATION_ITEM ( )  RATIONAL_B_SPLINE_SURFACE ( (
 ( 1.000000000000000000, 0.9541700777564650071, 1.000000000000000000),
 ( 1.000000000000000000, 0.9520170179154711088, 1.000000000000000000),
 ( 1.000000000000000000, 0.9503264940275176764, 1.000000000000000000),
 ( 1.000000000000000000, 0.9485966650353455654, 1.000000000000000000),
 ( 1.000000000000000000, 0.9481601953995637544, 1.000000000000000000),
 ( 1.000000000000000000, 0.9475786562863925955, 1.000000000000000000),
 ( 1.000000000000000000, 0.9474333041674911637, 1.000000000000000000),
 ( 1.000000000000000000, 0.9474385324093995697, 1.000000000000000000),
 ( 1.000000000000000000, 0.9480205960576686408, 1.000000000000000000),
 ( 1.000000000000000000, 0.9494433550397629595, 1.000000000000000000),
 ( 1.000000000000000000, 0.9497628485356935935, 1.000000000000000000),
 ( 1.000000000000000000, 0.9504717112739308194, 1.000000000000000000),
 ( 1.000000000000000000, 0.9508623530679600755, 1.000000000000000000),
 ( 1.000000000000000000, 0.9521262215768991899, 1.000000000000000000),
 ( 1.000000000000000000, 0.9530922057183041085, 1.000000000000000000),
 ( 1.000000000000000000, 0.9541700777564281477, 1.000000000000000000) ) ) 
 REPRESENTATION_ITEM ( '' )  SURFACE ( )  );
#24048=CARTESIAN_POINT ( 'NONE',  ( 57.59792236341147031, 54.84617931850878136, 1.722363176415705910 ) ) ;
#24049=CARTESIAN_POINT ( 'NONE',  ( 146.6084372240433709, 34.62501878078307982, 40.00000000000002132 ) ) ;
#24050=CARTESIAN_POINT ( 'NONE',  ( -173.7925586254464747, 12.78856870749536512, -41.93433064659100751 ) ) ;
#24051=CARTESIAN_POINT ( 'NONE',  ( 151.7948205124836534, 4.785054706297857230, 51.78348778862544322 ) ) ;
#24053=VECTOR ( 'NONE', #22996, 1000.000000000000000 ) ;
#24054=CARTESIAN_POINT ( 'NONE',  ( -56.48582580120558561, -30.84685318188645553, -40.00000000000002132 ) ) ;
#24055=CARTESIAN_POINT ( 'NONE',  ( -162.0762913951021176, 1.694272876828294194, 40.00000000000002132 ) ) ;
#24056=CARTESIAN_POINT ( 'NONE',  ( -238.4067589809705794, 3.877349844572403567E-13, -40.96449427998260973 ) ) ;
#24057=CARTESIAN_POINT ( 'NONE',  ( 98.29850319158911987, -8.262390927704235111, 18.22532005579163794 ) ) ;
#24058=CARTESIAN_POINT ( 'NONE',  ( -280.0000000000000568, 42.42640687119294540, -14.14213562373059041 ) ) ;
#24059=ORIENTED_EDGE ( 'NONE', *, *, #7756, .T. ) ;
#24060=CARTESIAN_POINT ( 'NONE',  ( -77.90255099906772784, 20.04994828523968664, -8.644468104261312291 ) ) ;
#24061=CARTESIAN_POINT ( 'NONE',  ( 0.2972598230769983307, -14.33493731733933352, 0.000000000000000000 ) ) ;
#24062=CARTESIAN_POINT ( 'NONE',  ( -100.0968563617495590, -8.893120081474123140, 20.41799937592168490 ) ) ;
#24066=CARTESIAN_POINT ( 'NONE',  ( 151.7948205124835681, -4.785054706298153882, -51.78348778862540058 ) ) ;
#24067=CARTESIAN_POINT ( 'NONE',  ( 23.84827734669235966, -42.71123329578353633, -23.24317830786350214 ) ) ;
#24069=CARTESIAN_POINT ( 'NONE',  ( 0.2972598230769930017, 14.33493731733933352, -40.00000000000002132 ) ) ;
#24070=CARTESIAN_POINT ( 'NONE',  ( -89.91498783733561595, -20.17141720492066170, 8.733585467896798349 ) ) ;
#24071=ORIENTED_EDGE ( 'NONE', *, *, #388, .T. ) ;
#24073=CARTESIAN_POINT ( 'NONE',  ( -105.2501940903818252, 21.20184772653823657, -3.401136913335300438 ) ) ;
#24074=CARTESIAN_POINT ( 'NONE',  ( 146.6084372240433709, 3.800685668858776900, -52.76785682606518435 ) ) ;
#24075=CARTESIAN_POINT ( 'NONE',  ( -187.7699188115095694, -42.84915433765046089, -23.34606611631119222 ) ) ;
#24076=AXIS2_PLACEMENT_3D ( 'NONE', #22002, #4047, #8016 ) ;
#24078=CARTESIAN_POINT ( 'NONE',  ( -56.48582580120557850, -40.00000000000014211, 30.84685318188629921 ) ) ;
#24079=CARTESIAN_POINT ( 'NONE',  ( 19.06497207195980792, 14.19242893257840699, 40.00000000000002132 ) ) ;
#24081=CARTESIAN_POINT ( 'NONE',  ( -93.12335834970889437, -2.546043227727554326E-13, 22.67402823373191723 ) ) ;
#24082=CARTESIAN_POINT ( 'NONE',  ( 4.995406935893297984, -40.00000000000007816, 15.24977328854818914 ) ) ;
#24083=CARTESIAN_POINT ( 'NONE',  ( -135.8532207217289738, -40.00000000000014211, 9.153146818113153671 ) ) ;
#24085=CARTESIAN_POINT ( 'NONE',  ( 184.8905102610680444, -13.49065550809810965, 13.49065550809799596 ) ) ;
#24086=CARTESIAN_POINT ( 'NONE',  ( 151.7948205124835681, 33.23291073765556547, -40.00000000000002132 ) ) ;
#24087=CARTESIAN_POINT ( 'NONE',  ( 146.6084372240433709, -3.800685668858344801, -52.76785682606520567 ) ) ;
#24090=CARTESIAN_POINT ( 'NONE',  ( 160.7895100360998981, 20.14405787076340459, 20.14405787076372434 ) ) ;
#24091=CARTESIAN_POINT ( 'NONE',  ( 192.4448373802101173, -39.99999999999991473, -20.00000000003956302 ) ) ;
#24092=CARTESIAN_POINT ( 'NONE',  ( -162.0762913951020892, 57.76657433537918251, 1.198031840455469066 ) ) ;
#24093=CARTESIAN_POINT ( 'NONE',  ( -114.7569578620488215, 13.65702197131982132, 17.44219256208173974 ) ) ;
#24094=CARTESIAN_POINT ( 'NONE',  ( -188.6890294954785361, -23.53287096355055752, -43.11788624870519726 ) ) ;
#24095=CARTESIAN_POINT ( 'NONE',  ( -91.56559293963836410, 16.03295912088714203, -16.03295912088699282 ) ) ;
#24097=CARTESIAN_POINT ( 'NONE',  ( -238.4067589809705794, -27.60227080167029001, -28.96627169325357798 ) ) ;
#24099=CARTESIAN_POINT ( 'NONE',  ( 14.38125909742181285, -10.73282306404727393, 10.73282306404716380 ) ) ;
#24101=CIRCLE ( 'NONE', #18519, 15.00000000000000000 ) ;
#24103=CARTESIAN_POINT ( 'NONE',  ( 170.0000000000000000, -30.00000000000001066, 3.673940397442064700E-15 ) ) ;
#24104=CARTESIAN_POINT ( 'NONE',  ( 19.06497207195981858, 10.03556273973516078, -66.60410523465806421 ) ) ;
#24105=CARTESIAN_POINT ( 'NONE',  ( -199.0730705748672449, -18.57195860672538501, -44.83667434817598973 ) ) ;
#24111=CARTESIAN_POINT ( 'NONE',  ( -3.993758944537615818, 13.83056263162083610, 47.00698038896962316 ) ) ;
#24116=CARTESIAN_POINT ( 'NONE',  ( -114.5514240062852878, 6.817200167027167801, 20.88736325032624919 ) ) ;
#24120=CARTESIAN_POINT ( 'NONE',  ( 21.16156876808017273, 43.48822901267212160, -23.80729322913541424 ) ) ;
#24121=DIRECTION ( 'NONE',  ( 0.9352143323240664774, -0.3271292298997905967, 0.1355013636862025250 ) ) ;
#24122=CARTESIAN_POINT ( 'NONE',  ( -109.1264249741456211, -33.12752917268984731, 13.72187187124577434 ) ) ;
#24124=CARTESIAN_POINT ( 'NONE',  ( -28.75704569508430808, -18.59466133783069708, 35.61514925947740551 ) ) ;
#24127=CARTESIAN_POINT ( 'NONE',  ( 1.925538622545307943, -14.07631154917879890, -48.64880301057759482 ) ) ;
#24128=CARTESIAN_POINT ( 'NONE',  ( -238.4067589809705794, -28.96627169325303797, -28.96627169325349627 ) ) ;
#24129=CARTESIAN_POINT ( 'NONE',  ( -200.0000000000000568, 14.52307781036561352, 48.92947633520088857 ) ) ;
#24130=CARTESIAN_POINT ( 'NONE',  ( 200.0000000000000000, -14.14213562373062949, -42.42640687119301646 ) ) ;
#24131=CARTESIAN_POINT ( 'NONE',  ( 184.8905102610680444, -1.851754852062639767E-13, 20.92133201514444352 ) ) ;
#24133=CARTESIAN_POINT ( 'NONE',  ( 91.82158438592159655, -22.79471317813468545, -2.449293598294708485E-15 ) ) ;
#24135=CARTESIAN_POINT ( 'NONE',  ( 19.06497207195982924, -54.19242893257843008, -40.00000000000002132 ) ) ;
#24136=CARTESIAN_POINT ( 'NONE',  ( -110.0473846051921214, 8.595625304770370789, 18.26116446882227251 ) ) ;
#24137=CARTESIAN_POINT ( 'NONE',  ( 91.82158438592156813, 39.99999999999986500, 17.20528682183341473 ) ) ;
#24138=CARTESIAN_POINT ( 'NONE',  ( -86.96347745069644475, -15.38646221621786125, -15.38646221621789856 ) ) ;
#24139=CARTESIAN_POINT ( 'NONE',  ( 136.1360204305621551, -35.03383547441293899, -40.00000000000002132 ) ) ;
#24141=CARTESIAN_POINT ( 'NONE',  ( 23.49666234703823520, -46.76389514419459204, 13.79192166426267363 ) ) ;
#24143=CARTESIAN_POINT ( 'NONE',  ( 146.6084372240433709, 3.800685668858776900, -52.76785682606518435 ) ) ;
#24144=CARTESIAN_POINT ( 'NONE',  ( 170.2234770963711128, -40.00000000000004263, 15.44714144992801685 ) ) ;
#24145=CARTESIAN_POINT ( 'NONE',  ( 91.82158438592158234, 16.11829626348378142, 40.45024623143977749 ) ) ;
#24146=CARTESIAN_POINT ( 'NONE',  ( -198.0356074513804572, 15.37879056873067007, 0.000000000000000000 ) ) ;
#24147=CARTESIAN_POINT ( 'NONE',  ( 184.8905102610680444, -20.92133201514440799, -40.00000000000002132 ) ) ;
#24148=CARTESIAN_POINT ( 'NONE',  ( -126.6834156230571011, -24.04426801068274244, -11.16464796290152428 ) ) ;
#24151=CARTESIAN_POINT ( 'NONE',  ( -56.48582580120559271, 21.81201906317798489, -21.81201906317746619 ) ) ;
#24152=CARTESIAN_POINT ( 'NONE',  ( 14.38125909742183062, -67.30136555895943218, -10.73282306403629605 ) ) ;
#24154=CARTESIAN_POINT ( 'NONE',  ( -77.90255099906775627, 20.04994828523981099, -8.644468104260917940 ) ) ;
#24155=CARTESIAN_POINT ( 'NONE',  ( 184.8905102610680444, -13.49065550809791603, -13.49065550809818781 ) ) ;
#24157=CARTESIAN_POINT ( 'NONE',  ( -280.0000000000000568, -42.42640687119276066, -14.14213562373147148 ) ) ;
#24158=CARTESIAN_POINT ( 'NONE',  ( 4.995406935893293543, -10.78321810389005364, 10.78321810388994173 ) ) ;
#24160=AXIS2_PLACEMENT_3D ( 'NONE', #22301, #22437, #203 ) ;
#24162=CARTESIAN_POINT ( 'NONE',  ( 57.59792236341147031, 1.908507979671054758E-14, -2.435789363418160658 ) ) ;
#24163=( BOUNDED_SURFACE ( )  B_SPLINE_SURFACE ( 3, 3, ( 
 ( #26131, #26274, #16400, #12811, #12404, #14403, #8685, #22665, #20933, #6547, #14795, #21059, #4707, #4574, #2572, #712, #10817, #24660, #2712, #16532, #14657, #23065, #6285, #24529, #20529, #444, #22533, #4837, #8816, #4314 ),
 ( #8547, #578, #2300, #16794, #12531, #10409, #16927, #18930, #6417, #18526, #24930, #25061, #6813, #16663, #6680, #14929, #308, #20664, #10686, #22797, #12943, #2845, #10953, #14534, #24795, #8410, #4437, #19059, #8275, #2434 ),
 ( #10546, #18657, #12671, #20800, #18797, #22926, #17183, #17314, #13199, #25446, #973, #17438, #15562, #19436, #9077, #21566, #13446, #21192, #9202, #25193, #3339, #2964, #7198, #13319, #11196, #11440, #23562, #6941, #21321, #21439 ),
 ( #25697, #7321, #15191, #1223, #4968, #15313, #5094, #13077, #23439, #3094, #19189, #21694, #15059, #19310, #841, #11320, #25319, #7077, #5215, #1093, #3214, #23319, #25575, #23686, #9327, #15435, #19562, #1354, #11075, #5337 ),
 ( #11569, #23189, #9453, #17559, #7448, #5465, #13568, #3470, #8951, #17060, #3594, #1476, #24222, #26098, #9582, #2010, #13963, #1, #13700, #8113, #15817, #24723, #3872, #17818, #5594, #9979, #17687, #19956, #22721, #23944 ),
 ( #1739, #9848, #17951, #7706, #7834, #19688, #15957, #19824, #24083, #11836, #5857, #22098, #6479, #11973, #18215, #25966, #25830, #26239, #20098, #14592, #11703, #4007, #10115, #1876, #16229, #5722, #4498, #7574, #12106, #18088 ),
 ( #1610, #7974, #15687, #23812, #21825, #9714, #16092, #13826, #21959, #20231, #3733, #5996, #14102, #22231, #4897, #20731, #13006, #16861, #6606, #21254, #7001, #20857, #16722, #21127, #3027, #23253, #12872, #11011, #15122, #1031 ) ),
 .UNSPECIFIED., .T., .F., .F. ) 
 B_SPLINE_SURFACE_WITH_KNOTS ( ( 4, 3, 4 ),
 ( 4, 2, 2, 2, 2, 2, 2, 2, 2, 2, 2, 2, 2, 2, 4 ),
 ( 0.000000000000000000, 0.5000000000000000000, 1.000000000000000000 ),
 ( 0.000000000000000000, 0.1357259735107005372, 0.1651108541090157700, 0.1944957347073310028, 0.3598804999793158710, 0.3867117631979620773, 0.4135430264166082281, 0.5789277916885930964, 0.6062785021374117456, 0.6336292125862302838, 0.8508620842112317728, 0.8814014469398914198, 0.9119408096685510667, 0.9559704048342755334, 1.000000000000000000 ),
 .UNSPECIFIED. ) 
 GEOMETRIC_REPRESENTATION_ITEM ( )  RATIONAL_B_SPLINE_SURFACE ( (
 ( 1.000000000000000000, 1.000000000000000000, 1.000000000000000000, 1.000000000000000000, 1.000000000000000000, 1.000000000000000000, 1.000000000000000000, 1.000000000000000000, 1.000000000000000000, 1.000000000000000000, 1.000000000000000000, 1.000000000000000000, 1.000000000000000000, 1.000000000000000000, 1.000000000000000000, 1.000000000000000000, 1.000000000000000000, 1.000000000000000000, 1.000000000000000000, 1.000000000000000000, 1.000000000000000000, 1.000000000000000000, 1.000000000000000000, 1.000000000000000000, 1.000000000000000000, 1.000000000000000000, 1.000000000000000000, 1.000000000000000000, 1.000000000000000000, 1.000000000000000000),
 ( 0.3333333333333333703, 0.3333333333333333703, 0.3333333333333333703, 0.3333333333333333703, 0.3333333333333333703, 0.3333333333333333703, 0.3333333333333333703, 0.3333333333333333703, 0.3333333333333333703, 0.3333333333333333703, 0.3333333333333333703, 0.3333333333333333703, 0.3333333333333333703, 0.3333333333333333703, 0.3333333333333333703, 0.3333333333333333703, 0.3333333333333333703, 0.3333333333333333703, 0.3333333333333333703, 0.3333333333333333703, 0.3333333333333333703, 0.3333333333333333703, 0.3333333333333333703, 0.3333333333333333703, 0.3333333333333333703, 0.3333333333333333703, 0.3333333333333333703, 0.3333333333333333703, 0.3333333333333333703, 0.3333333333333333703),
 ( 0.3333333333333333703, 0.3333333333333333703, 0.3333333333333333703, 0.3333333333333333703, 0.3333333333333333703, 0.3333333333333333703, 0.3333333333333333703, 0.3333333333333333703, 0.3333333333333333703, 0.3333333333333333703, 0.3333333333333333703, 0.3333333333333333703, 0.3333333333333333703, 0.3333333333333333703, 0.3333333333333333703, 0.3333333333333333703, 0.3333333333333333703, 0.3333333333333333703, 0.3333333333333333703, 0.3333333333333333703, 0.3333333333333333703, 0.3333333333333333703, 0.3333333333333333703, 0.3333333333333333703, 0.3333333333333333703, 0.3333333333333333703, 0.3333333333333333703, 0.3333333333333333703, 0.3333333333333333703, 0.3333333333333333703),
 ( 1.000000000000000000, 1.000000000000000000, 1.000000000000000000, 1.000000000000000000, 1.000000000000000000, 1.000000000000000000, 1.000000000000000000, 1.000000000000000000, 1.000000000000000000, 1.000000000000000000, 1.000000000000000000, 1.000000000000000000, 1.000000000000000000, 1.000000000000000000, 1.000000000000000000, 1.000000000000000000, 1.000000000000000000, 1.000000000000000000, 1.000000000000000000, 1.000000000000000000, 1.000000000000000000, 1.000000000000000000, 1.000000000000000000, 1.000000000000000000, 1.000000000000000000, 1.000000000000000000, 1.000000000000000000, 1.000000000000000000, 1.000000000000000000, 1.000000000000000000),
 ( 0.3333333333333333703, 0.3333333333333333703, 0.3333333333333333703, 0.3333333333333333703, 0.3333333333333333703, 0.3333333333333333703, 0.3333333333333333703, 0.3333333333333333703, 0.3333333333333333703, 0.3333333333333333703, 0.3333333333333333703, 0.3333333333333333703, 0.3333333333333333703, 0.3333333333333333703, 0.3333333333333333703, 0.3333333333333333703, 0.3333333333333333703, 0.3333333333333333703, 0.3333333333333333703, 0.3333333333333333703, 0.3333333333333333703, 0.3333333333333333703, 0.3333333333333333703, 0.3333333333333333703, 0.3333333333333333703, 0.3333333333333333703, 0.3333333333333333703, 0.3333333333333333703, 0.3333333333333333703, 0.3333333333333333703),
 ( 0.3333333333333333703, 0.3333333333333333703, 0.3333333333333333703, 0.3333333333333333703, 0.3333333333333333703, 0.3333333333333333703, 0.3333333333333333703, 0.3333333333333333703, 0.3333333333333333703, 0.3333333333333333703, 0.3333333333333333703, 0.3333333333333333703, 0.3333333333333333703, 0.3333333333333333703, 0.3333333333333333703, 0.3333333333333333703, 0.3333333333333333703, 0.3333333333333333703, 0.3333333333333333703, 0.3333333333333333703, 0.3333333333333333703, 0.3333333333333333703, 0.3333333333333333703, 0.3333333333333333703, 0.3333333333333333703, 0.3333333333333333703, 0.3333333333333333703, 0.3333333333333333703, 0.3333333333333333703, 0.3333333333333333703),
 ( 1.000000000000000000, 1.000000000000000000, 1.000000000000000000, 1.000000000000000000, 1.000000000000000000, 1.000000000000000000, 1.000000000000000000, 1.000000000000000000, 1.000000000000000000, 1.000000000000000000, 1.000000000000000000, 1.000000000000000000, 1.000000000000000000, 1.000000000000000000, 1.000000000000000000, 1.000000000000000000, 1.000000000000000000, 1.000000000000000000, 1.000000000000000000, 1.000000000000000000, 1.000000000000000000, 1.000000000000000000, 1.000000000000000000, 1.000000000000000000, 1.000000000000000000, 1.000000000000000000, 1.000000000000000000, 1.000000000000000000, 1.000000000000000000, 1.000000000000000000) ) ) 
 REPRESENTATION_ITEM ( '' )  SURFACE ( )  );
#24164=CARTESIAN_POINT ( 'NONE',  ( -192.9588430854689989, -10.23066800230742501, -10.23066800230756712 ) ) ;
#24165=CARTESIAN_POINT ( 'NONE',  ( -4.082462733455239245, 42.99255347688239937, -23.44093842354132917 ) ) ;
#24166=CARTESIAN_POINT ( 'NONE',  ( -91.56559293963834989, 17.32597176626809343, 2.449293598294708485E-15 ) ) ;
#24168=CARTESIAN_POINT ( 'NONE',  ( -86.96347745069644475, -15.38646221621786125, -15.38646221621789856 ) ) ;
#24169=CARTESIAN_POINT ( 'NONE',  ( 6.875206813650288851, 43.66894609317728992, 18.08826972633240970 ) ) ;
#24170=CARTESIAN_POINT ( 'NONE',  ( -86.86493150571111244, 7.943527260496201947, -19.77569912839169319 ) ) ;
#24171=FACE_OUTER_BOUND ( 'NONE', #5107, .T. ) ;
#24173=CARTESIAN_POINT ( 'NONE',  ( -193.3669111531511646, -44.23532963564880305, 18.32287347113157949 ) ) ;
#24175=ADVANCED_FACE ( 'NONE', ( #17129 ), #16591, .T. ) ;
#24176=CARTESIAN_POINT ( 'NONE',  ( 20.38198589868259347, -18.12553405622861646, 43.75891014376981047 ) ) ;
#24177=B_SPLINE_CURVE_WITH_KNOTS ( 'NONE', 3,
 ( #19118, #10607, #367, #6477, #8470, #18719 ),
 .UNSPECIFIED., .F., .F.,
 ( 4, 2, 4 ),
 ( 3.460613336329060854E-15, 0.03937794852164089310, 0.07875589704327831675 ),
 .UNSPECIFIED. ) ;
#24178=CARTESIAN_POINT ( 'NONE',  ( 23.30336656375570215, 13.80490921643141355, -46.83484695576438384 ) ) ;
#24182=CARTESIAN_POINT ( 'NONE',  ( -144.1957134278176227, -12.48102206790046864, 30.13185274883752740 ) ) ;
#24183=CARTESIAN_POINT ( 'NONE',  ( -135.8532207217289738, 21.81201906317798134, -21.81201906317747685 ) ) ;
#24184=CARTESIAN_POINT ( 'NONE',  ( -192.9588430854689989, -14.46834944099973086, 0.000000000000000000 ) ) ;
#24185=CARTESIAN_POINT ( 'NONE',  ( -188.8753834511962566, 17.93496043754537439, -43.29882472894595935 ) ) ;
#24186=FACE_OUTER_BOUND ( 'NONE', #16653, .T. ) ;
#24187=CARTESIAN_POINT ( 'NONE',  ( -91.56559293963836410, 22.67402823373189946, -0.000000000000000000 ) ) ;
#24188=CARTESIAN_POINT ( 'NONE',  ( 199.9999999999999432, 20.00000000000013856, 0.000000000000000000 ) ) ;
#24189=CARTESIAN_POINT ( 'NONE',  ( 14.38125909742180752, 15.17850393972634038, 0.000000000000000000 ) ) ;
#24190=B_SPLINE_CURVE_WITH_KNOTS ( 'NONE', 3,
 ( #18882, #661, #18749, #16884, #21011, #10641, #25148, #4395, #16746, #797, #24879, #21149, #17011, #397 ),
 .UNSPECIFIED., .F., .F.,
 ( 4, 2, 2, 2, 2, 2, 4 ),
 ( 0.0003132551814622137128, 0.004485169056170316450, 0.006571125993524368387, 0.008657082930878422927, 0.01282899680558652854, 0.01491495374294058394, 0.01700091068029464109 ),
 .UNSPECIFIED. ) ;
#24191=CARTESIAN_POINT ( 'NONE',  ( -213.1075012329537230, -39.99999999999948841, -53.71589010950208376 ) ) ;
#24192=CARTESIAN_POINT ( 'NONE',  ( -213.1075012329537230, 66.26714140136188291, 9.698598906438215650 ) ) ;
#24195=CARTESIAN_POINT ( 'NONE',  ( 57.59792236341147031, 1.722363176415040886, 1.722363176415060426 ) ) ;
#24196=B_SPLINE_CURVE_WITH_KNOTS ( 'NONE', 3,
 ( #6528, #16909, #20642, #2284, #2549, #22907, #4685, #8797 ),
 .UNSPECIFIED., .F., .F.,
 ( 4, 2, 2, 4 ),
 ( 0.0002291277468225442668, 0.002289782534629433795, 0.004350437322436322835, 0.008471746898050105251 ),
 .UNSPECIFIED. ) ;
#24197=EDGE_CURVE ( 'NONE', #25714, #2784, #9963, .T. ) ;
#24198=ORIENTED_EDGE ( 'NONE', *, *, #18927, .T. ) ;
#24199=CARTESIAN_POINT ( 'NONE',  ( 146.6084372240433993, -24.48358557860319706, -24.48358557860330720 ) ) ;
#24200=CARTESIAN_POINT ( 'NONE',  ( -100.0968563617643099, -8.149320301498496733, 20.72609133247458146 ) ) ;
#24203=CARTESIAN_POINT ( 'NONE',  ( -100.7734535825088500, -40.53558337403669753, -16.03295912088728770 ) ) ;
#24204=CARTESIAN_POINT ( 'NONE',  ( 22.92196489051404029, -42.99364193793746836, -23.44087486047875402 ) ) ;
#24206=CARTESIAN_POINT ( 'NONE',  ( -280.0000000000000000, -20.00000000000006750, 0.000000000000000000 ) ) ;
#24207=CARTESIAN_POINT ( 'NONE',  ( -86.86493150571010347, -19.77569912839160082, 7.943527260495840459 ) ) ;
#24213=CARTESIAN_POINT ( 'NONE',  ( 163.1118516004056573, -19.27778845538761132, -19.27778845538770724 ) ) ;
#24214=CARTESIAN_POINT ( 'NONE',  ( -166.3490736459090442, -39.29841219601716062, -12.23457872942467972 ) ) ;
#24215=( BOUNDED_SURFACE ( )  B_SPLINE_SURFACE ( 3, 2, ( 
 ( #24915, #16778, #8669 ),
 ( #565, #10532, #6800 ),
 ( #17044, #4690, #8802 ),
 ( #8397, #6666, #12930 ),
 ( #2423, #25179, #20648 ),
 ( #18645, #430, #290 ),
 ( #8534, #12518, #16519 ),
 ( #24646, #12793, #16651 ),
 ( #4956, #20919, #24781 ),
 ( #16914, #6403, #6533 ),
 ( #21046, #14644, #22650 ),
 ( #22783, #2829, #10938 ) ),
 .UNSPECIFIED., .F., .F., .F. ) 
 B_SPLINE_SURFACE_WITH_KNOTS ( ( 4, 2, 2, 2, 2, 4 ),
 ( 3, 3 ),
 ( 0.006022589392326821271, 0.01254516766564470545, 0.01580645680230364711, 0.01906774593896258876, 0.02559032421228047555, 0.03211290248559835886 ),
 ( 0.000000000000000000, 1.000000000000000000 ),
 .UNSPECIFIED. ) 
 GEOMETRIC_REPRESENTATION_ITEM ( )  RATIONAL_B_SPLINE_SURFACE ( (
 ( 1.000000000000000000, 0.9998834880171258988, 1.000000000000000000),
 ( 1.000000000000000000, 0.9998139205011338237, 1.000000000000000000),
 ( 1.000000000000000000, 0.9997315632445886724, 1.000000000000000000),
 ( 1.000000000000000000, 0.9996405464946352959, 1.000000000000000000),
 ( 1.000000000000000000, 0.9996155081776924023, 1.000000000000000000),
 ( 1.000000000000000000, 0.9995814087511104562, 1.000000000000000000),
 ( 1.000000000000000000, 0.9995724100939918921, 1.000000000000000000),
 ( 1.000000000000000000, 0.9995726760936894939, 1.000000000000000000),
 ( 1.000000000000000000, 0.9996103361816741639, 1.000000000000000000),
 ( 1.000000000000000000, 0.9997312749796802844, 1.000000000000000000),
 ( 1.000000000000000000, 0.9998135910914284219, 1.000000000000000000),
 ( 1.000000000000000000, 0.9998834880173383954, 1.000000000000000000) ) ) 
 REPRESENTATION_ITEM ( '' )  SURFACE ( )  );
#24216=CARTESIAN_POINT ( 'NONE',  ( -135.8532207217289738, -40.00000000000001421, -9.153146818113709671 ) ) ;
#24217=CARTESIAN_POINT ( 'NONE',  ( -105.3755690713226585, -21.75974354311652448, 40.00000000000002132 ) ) ;
#24220=CARTESIAN_POINT ( 'NONE',  ( -198.0356074513804572, -40.00000000000011369, 15.37879056873056527 ) ) ;
#24221=CARTESIAN_POINT ( 'NONE',  ( -86.96347745069643054, -40.00000000000009948, 18.24025645688337960 ) ) ;
#24222=CARTESIAN_POINT ( 'NONE',  ( -86.96347745069643054, -39.99999999999985079, -18.24025645688394448 ) ) ;
#24223=CARTESIAN_POINT ( 'NONE',  ( 136.1360204305621551, 40.00000000000017053, -35.03383547441281820 ) ) ;
#24225=CARTESIAN_POINT ( 'NONE',  ( -56.48582580120558561, -21.81201906317785699, 21.81201906317761896 ) ) ;
#24226=CARTESIAN_POINT ( 'NONE',  ( 14.38125909742181285, -15.17850393972633505, 0.000000000000000000 ) ) ;
#24227=CARTESIAN_POINT ( 'NONE',  ( 4.995406935893310418, -67.35176059880237176, 10.78321810387813429 ) ) ;
#24228=CARTESIAN_POINT ( 'NONE',  ( -100.0753760173604121, -8.894334231739641439, 20.41987330121789768 ) ) ;
#24231=CARTESIAN_POINT ( 'NONE',  ( -105.3755690713226585, 39.99999999999977263, 21.75974354311691883 ) ) ;
#24232=CARTESIAN_POINT ( 'NONE',  ( -135.8532207217289738, -40.00000000000001421, -9.153146818113709671 ) ) ;
#24233=CARTESIAN_POINT ( 'NONE',  ( 192.4448373802100889, 14.14213562370310662, 14.14213562370312438 ) ) ;
#24234=CARTESIAN_POINT ( 'NONE',  ( 184.8905102610680444, -13.49065550809840630, 43.07788698682565354 ) ) ;
#24235=CARTESIAN_POINT ( 'NONE',  ( -188.8842637254080046, -17.93596642850386758, -43.30125340596359251 ) ) ;
#24236=CARTESIAN_POINT ( 'NONE',  ( -100.7734535825088500, 16.03295912088713848, -16.03295912088698927 ) ) ;
#24238=CARTESIAN_POINT ( 'NONE',  ( 19.06497207195980792, -18.24870850772710540, -38.31983398719647482 ) ) ;
#24240=CARTESIAN_POINT ( 'NONE',  ( -280.0000000000000000, 19.99999999999996092, -0.000000000000000000 ) ) ;
#24241=CARTESIAN_POINT ( 'NONE',  ( -87.01524264494790373, 18.58252313551766832, 10.72938103944079380 ) ) ;
#24242=CARTESIAN_POINT ( 'NONE',  ( -238.4067589809705794, -27.60227080167029001, -28.96627169325357798 ) ) ;
#24243=DIRECTION ( 'NONE',  ( 0.7071067811865479058, -0.7071067811865472397, 8.659560562354931626E-17 ) ) ;
#24244=ORIENTED_EDGE ( 'NONE', *, *, #970, .T. ) ;
#24247=CARTESIAN_POINT ( 'NONE',  ( -4.558244102845256940, 23.34817229226072754, 42.85231560262773343 ) ) ;
#24250=CARTESIAN_POINT ( 'NONE',  ( 199.9999999999999432, -20.00000000000006750, 0.000000000000000000 ) ) ;
#24252=CARTESIAN_POINT ( 'NONE',  ( -105.2054292637484849, -1.359563962808593374, -21.49321519467867247 ) ) ;
#24255=CARTESIAN_POINT ( 'NONE',  ( -89.91646883263047130, -8.407637968043596643, -20.29783361037425493 ) ) ;
#24256=CARTESIAN_POINT ( 'NONE',  ( -192.9588430854690273, 40.00000000000014211, -14.46834944099927966 ) ) ;
#24257=CARTESIAN_POINT ( 'NONE',  ( 98.29850319134099834, 7.044854746987213368, -18.72964005463162351 ) ) ;
#24259=CARTESIAN_POINT ( 'NONE',  ( -65.65555754753385997, -11.16466304451101621, 24.04429191298356017 ) ) ;
#24262=CARTESIAN_POINT ( 'NONE',  ( -2.004660104927048714, -18.09067139730387197, -43.67474423982621801 ) ) ;
#24264=CARTESIAN_POINT ( 'NONE',  ( 91.82158438592159655, -44.40256751092341858, 12.16597498400012434 ) ) ;
#24265=CARTESIAN_POINT ( 'NONE',  ( -114.7826396787321812, -14.66025428929974517, -16.63820106242354058 ) ) ;
#24266=CARTESIAN_POINT ( 'NONE',  ( -238.4067589809705794, -57.25054294065807881, 0.6820004457338858517 ) ) ;
#24267=CARTESIAN_POINT ( 'NONE',  ( 192.4448373802100889, -1.741373372144848397E-13, 20.00000000003942091 ) ) ;
#24269=CARTESIAN_POINT ( 'NONE',  ( -238.4067589809705794, 27.60227080167080160, -28.96627169325299533 ) ) ;
#24270=CARTESIAN_POINT ( 'NONE',  ( 146.6084372240433993, -5.374981219216945938, -2.449293598294708485E-15 ) ) ;
#24271=EDGE_CURVE ( 'NONE', #7299, #12394, #22036, .T. ) ;
#24272=CARTESIAN_POINT ( 'NONE',  ( -213.1075012329537230, 9.698598906450543566, -9.698598906450348167 ) ) ;
#24273=AXIS2_PLACEMENT_3D ( 'NONE', #9377, #19488, #11244 ) ;
#24275=CARTESIAN_POINT ( 'NONE',  ( 91.82158438592159655, -22.79471317813468545, -40.00000000000002132 ) ) ;
#24277=CARTESIAN_POINT ( 'NONE',  ( -110.0853217340286250, 16.68198050937877497, 11.37485173728495269 ) ) ;
#24278=CARTESIAN_POINT ( 'NONE',  ( 19.06497207195979726, 40.00000000000017053, -14.19242893257798599 ) ) ;
#24279=CARTESIAN_POINT ( 'NONE',  ( -198.0356074513804572, 39.15871834505912119, -17.40982414986464377 ) ) ;
#24280=CARTESIAN_POINT ( 'NONE',  ( -280.0000000000000000, -20.00000000000006750, 0.000000000000000000 ) ) ;
#24283=CARTESIAN_POINT ( 'NONE',  ( 170.2234770963711128, -24.55285855007183926, 0.000000000000000000 ) ) ;
#24284=CARTESIAN_POINT ( 'NONE',  ( 155.1206158682454941, 11.51471166709214877, 27.79897307351034996 ) ) ;
#24285=CARTESIAN_POINT ( 'NONE',  ( -86.96347745069644475, -8.210974027862429531E-14, 18.24025645688352881 ) ) ;
#24287=CARTESIAN_POINT ( 'NONE',  ( 91.82158438592158234, -12.16597498397778843, 12.16597498397750954 ) ) ;
#24290=CARTESIAN_POINT ( 'NONE',  ( 136.1360204305621266, -35.03383547441293899, 0.000000000000000000 ) ) ;
#24292=DIRECTION ( 'NONE',  ( 0.000000000000000000, -0.3656393565208022056, -0.9307566067254390285 ) ) ;
#24296=CARTESIAN_POINT ( 'NONE',  ( 151.7948205124836250, 4.785054706301759886, -4.785054706301612448 ) ) ;
#24297=CARTESIAN_POINT ( 'NONE',  ( 163.1118516004056573, -9.006482792069506971, -9.006482792069697041 ) ) ;
#24299=CARTESIAN_POINT ( 'NONE',  ( -100.7734535825088358, -2.560096224687585342E-13, 22.67402823373191723 ) ) ;
#24300=CARTESIAN_POINT ( 'NONE',  ( 4.995406935893312195, -67.35176059882525124, -10.78321810390210445 ) ) ;
#24301=CARTESIAN_POINT ( 'NONE',  ( -192.9588430854689989, 10.23066800230756712, -10.23066800230735396 ) ) ;
#24302=CARTESIAN_POINT ( 'NONE',  ( 130.8568914410475088, -24.07718906446864793, -32.49135343045505664 ) ) ;
#24304=CARTESIAN_POINT ( 'NONE',  ( -259.2033419157646676, -49.83842185052031937, -6.730120644403796426 ) ) ;
#24307=CARTESIAN_POINT ( 'NONE',  ( 170.2234770963711128, 40.00000000000000000, 15.44714144992830462 ) ) ;
#24310=CARTESIAN_POINT ( 'NONE',  ( 21.80824205440350383, 47.36272483143649481, -13.88338701302033051 ) ) ;
#24311=CARTESIAN_POINT ( 'NONE',  ( -198.0356074513804572, 55.37879056874818673, -40.00000000000002132 ) ) ;
#24312=ORIENTED_EDGE ( 'NONE', *, *, #19871, .T. ) ;
#24313=CARTESIAN_POINT ( 'NONE',  ( -208.1127848780265026, 15.00245453012665564, 0.000000000000000000 ) ) ;
#24314=CARTESIAN_POINT ( 'NONE',  ( -5.304449574935675038, -42.80137191221822235, 17.72890873421427571 ) ) ;
#24315=APPLICATION_CONTEXT ( 'automotive_design' ) ;
#24316=CARTESIAN_POINT ( 'NONE',  ( 130.8568914410475372, -34.05028731879786363, 0.000000000000000000 ) ) ;
#24317=ORIENTED_EDGE ( 'NONE', *, *, #17520, .F. ) ;
#24318=CARTESIAN_POINT ( 'NONE',  ( -190.5535326093807953, -43.70552662394274535, 18.10342187830013927 ) ) ;
#24320=CARTESIAN_POINT ( 'NONE',  ( 17.91733029160310409, -24.32486282486970097, 44.18858371746046743 ) ) ;
#24321=CARTESIAN_POINT ( 'NONE',  ( 20.91285618074528330, 13.92631245145418895, -47.65039156502910345 ) ) ;
#24326=CARTESIAN_POINT ( 'NONE',  ( 91.82158438592158234, 7.693928927950222250E-14, -17.20528682183300262 ) ) ;
#24327=CARTESIAN_POINT ( 'NONE',  ( -259.2033419157646676, 21.55415060305860209, -21.55415060305812602 ) ) ;
#24328=CARTESIAN_POINT ( 'NONE',  ( 146.6084372240433993, 34.62501878078308692, 0.000000000000000000 ) ) ;
#24329=CARTESIAN_POINT ( 'NONE',  ( -189.2667921706156449, 17.97629039507469173, -43.39860407294614220 ) ) ;
#24330=CARTESIAN_POINT ( 'NONE',  ( -105.3755690713226727, -15.38646221621807619, 15.38646221621768362 ) ) ;
#24331=CARTESIAN_POINT ( 'NONE',  ( -280.0000000000000000, -14.14213562373118549, 14.14213562373078936 ) ) ;
#24332=CARTESIAN_POINT ( 'NONE',  ( 136.1360204305621266, -4.966164525587039691, -2.449293598294708485E-15 ) ) ;
#24333=CARTESIAN_POINT ( 'NONE',  ( -192.9588430854689989, 54.46834944099968823, 2.449293598294708485E-15 ) ) ;
#24334=CARTESIAN_POINT ( 'NONE',  ( -280.0000000000000000, 1.605030083646939673E-13, -20.00000000000001421 ) ) ;
#24335=CARTESIAN_POINT ( 'NONE',  ( 0.2972598230769959993, 38.42060263243659080, 38.42060263243672580 ) ) ;
#24337=CARTESIAN_POINT ( 'NONE',  ( 184.8905102610680444, 14.79361573936375507, 14.79361573936398067 ) ) ;
#24339=CARTESIAN_POINT ( 'NONE',  ( -105.3755690713226727, -15.38646221621786481, -15.38646221621789856 ) ) ;
#24340=CARTESIAN_POINT ( 'NONE',  ( -99.31267923333066960, 8.544756979486514581, 20.62886818712721393 ) ) ;
#24343=CARTESIAN_POINT ( 'NONE',  ( -208.1127848780264742, -67.17687982763172272, 10.60833733270744617 ) ) ;
#24344=CARTESIAN_POINT ( 'NONE',  ( 67.78092418438932043, -29.26022923833890133, -12.11998378862976011 ) ) ;
#24346=CARTESIAN_POINT ( 'NONE',  ( -198.0356074513804572, 15.37879056873067007, 0.000000000000000000 ) ) ;
#24348=ORIENTED_EDGE ( 'NONE', *, *, #12164, .T. ) ;
#24351=CARTESIAN_POINT ( 'NONE',  ( -192.9588430854689989, 10.23066800230742679, 10.23066800230749607 ) ) ;
#24352=CARTESIAN_POINT ( 'NONE',  ( -188.3120606736146669, -46.99497558484360127, -13.82878088495401236 ) ) ;
#24353=CARTESIAN_POINT ( 'NONE',  ( -238.4067589809705794, -40.00000000000021316, 40.96449427990166470 ) ) ;
#24354=CARTESIAN_POINT ( 'NONE',  ( -100.7734535825088358, -22.67402823373193499, 0.000000000000000000 ) ) ;
#24357=CARTESIAN_POINT ( 'NONE',  ( -105.3755690713226585, -39.99999999999996447, -21.75974354311664527 ) ) ;
#24358=CARTESIAN_POINT ( 'NONE',  ( 170.2234770963711128, -40.00000000000004263, 15.44714144992801685 ) ) ;
#24359=CARTESIAN_POINT ( 'NONE',  ( -259.2033419157646676, 40.00000000000000711, -9.517827891722491884 ) ) ;
#24360=CARTESIAN_POINT ( 'NONE',  ( -213.1075012329537230, -13.71589010951915810, -40.00000000000002132 ) ) ;
#24361=CARTESIAN_POINT ( 'NONE',  ( -105.3755690713226585, -41.18208027870589660, -15.38646221621809040 ) ) ;
#24362=CARTESIAN_POINT ( 'NONE',  ( -198.0356074513804572, -15.37879056873074290, 0.000000000000000000 ) ) ;
#24363=CARTESIAN_POINT ( 'NONE',  ( -192.9588430854690273, -38.51493924976932703, -18.05360324515463688 ) ) ;
#24365=EDGE_CURVE ( 'NONE', #4560, #22478, #14444, .T. ) ;
#24367=CARTESIAN_POINT ( 'NONE',  ( 19.06497207195981147, 1.521599808664285085E-13, -14.19242893257840521 ) ) ;
#24368=CARTESIAN_POINT ( 'NONE',  ( -105.3755690713226585, -40.00000000000010658, 18.24025645688337249 ) ) ;
#24369=CARTESIAN_POINT ( 'NONE',  ( 4.995406935893287326, 67.35176059882533650, 10.78321810390163549 ) ) ;
#24370=CARTESIAN_POINT ( 'NONE',  ( 151.7948205124835681, -4.785054706298876859, 51.78348778862533663 ) ) ;
#24371=CARTESIAN_POINT ( 'NONE',  ( -188.2507053403081727, -23.43979243030855741, -42.99082124349035183 ) ) ;
#24372=CARTESIAN_POINT ( 'NONE',  ( 151.7948205124836250, -3.202120068677277203E-13, 33.23291073765553705 ) ) ;
#24374=CARTESIAN_POINT ( 'NONE',  ( -162.0762913951020892, 1.198031840385732849, -1.198031840385733515 ) ) ;
#24376=CARTESIAN_POINT ( 'NONE',  ( 163.1118516004056573, 27.26290988616875310, 0.000000000000000000 ) ) ;
#24377=CARTESIAN_POINT ( 'NONE',  ( 57.59792236341147031, -1.722363176414363206, -54.84617931850881689 ) ) ;
#24378=LINE ( 'NONE', #17971, #4102 ) ;
#24381=CARTESIAN_POINT ( 'NONE',  ( -105.3841681040951102, -19.11869201644174154, 9.644852623833179095 ) ) ;
#24382=CARTESIAN_POINT ( 'NONE',  ( -5.787027468459356783, 17.67457596681839860, 42.67020100828666074 ) ) ;
#24385=CARTESIAN_POINT ( 'NONE',  ( 91.82158438592158234, -17.20528682183298486, 0.000000000000000000 ) ) ;
#24387=CARTESIAN_POINT ( 'NONE',  ( -114.5516833806003660, -6.814384331921130133, -20.88871136328873845 ) ) ;
#24389=CARTESIAN_POINT ( 'NONE',  ( -102.4309680866877699, -8.087567261546894315, -20.43798635343767245 ) ) ;
#24390=CARTESIAN_POINT ( 'NONE',  ( -86.96347745069645896, 39.99999999999977973, 21.75974354311691883 ) ) ;
#24392=DIRECTION ( 'NONE',  ( -4.625929269271485322E-15, -0.9166903767141219017, 0.3995982397855640800 ) ) ;
#24397=CARTESIAN_POINT ( 'NONE',  ( 15.76057515058496605, -18.44716516376509929, -44.53539632572822171 ) ) ;
#24398=CARTESIAN_POINT ( 'NONE',  ( -213.1075012329537230, -66.26714140136188291, -9.698598906438677503 ) ) ;
#24399=CARTESIAN_POINT ( 'NONE',  ( -93.02511667906868809, 20.50052124204824011, -8.946512270084841845 ) ) ;
#24400=CARTESIAN_POINT ( 'NONE',  ( 57.59792236341147031, -26.56190807104670171, -30.00663442387710234 ) ) ;
#24401=DIRECTION ( 'NONE',  ( 0.01051738792036172217, 0.9307051272717591361, -0.3656191332813304995 ) ) ;
#24402=CARTESIAN_POINT ( 'NONE',  ( 19.06497207195981147, -10.03556273973425483, -10.03556273973443247 ) ) ;
#24403=CARTESIAN_POINT ( 'NONE',  ( -135.8532207217289454, -30.84685318188649106, 40.00000000000002132 ) ) ;
#24404=DIRECTION ( 'NONE',  ( -1.836970198721030181E-16, 1.000000000000000000, 0.000000000000000000 ) ) ;
#24405=CARTESIAN_POINT ( 'NONE',  ( -238.4067589809705794, -40.96449428006345528, 40.00000000000002132 ) ) ;
#24406=CARTESIAN_POINT ( 'NONE',  ( -105.3881900741214395, 9.658524497639083606, 19.07360370665400495 ) ) ;
#24407=CARTESIAN_POINT ( 'NONE',  ( -192.9588430854689989, 5.375290060580374156E-13, -54.46834944099972375 ) ) ;
#24408=CARTESIAN_POINT ( 'NONE',  ( 170.2234770963711128, -17.36149277826985937, -17.36149277826995174 ) ) ;
#24409=CARTESIAN_POINT ( 'NONE',  ( 200.0000000000000000, 19.99999999999996447, -40.00000000000002132 ) ) ;
#24413=CARTESIAN_POINT ( 'NONE',  ( -86.96347745069644475, -21.75974354311652093, 40.00000000000002132 ) ) ;
#24414=CARTESIAN_POINT ( 'NONE',  ( -105.4741150117379789, -19.60045294982730724, -8.366608964594114184 ) ) ;
#24415=CARTESIAN_POINT ( 'NONE',  ( 199.9999999999999432, -3.553951640073651008E-14, 19.99999999999992539 ) ) ;
#24416=CARTESIAN_POINT ( 'NONE',  ( -198.0356074513804572, 39.15871834505956173, -39.15871834505865223 ) ) ;
#24419=CARTESIAN_POINT ( 'NONE',  ( -87.12803293485021072, 1.366105440193874143, -21.45672515674945657 ) ) ;
#24422=CARTESIAN_POINT ( 'NONE',  ( 200.0000000000000000, 42.42640687119267540, 14.14213562373153543 ) ) ;
#24423=CARTESIAN_POINT ( 'NONE',  ( 136.1360204305621266, -3.511608612530630058, -3.511608612530719764 ) ) ;
#24425=CARTESIAN_POINT ( 'NONE',  ( -198.0356074513804572, 40.00000000000014921, -15.37879056873028816 ) ) ;
#24426=CARTESIAN_POINT ( 'NONE',  ( 19.06497207195982924, -66.60410523465809263, -10.03556273973493163 ) ) ;
#24428=CARTESIAN_POINT ( 'NONE',  ( -162.0762913951021176, -27.08623940707624911, 29.48230308784761888 ) ) ;
#24429=CARTESIAN_POINT ( 'NONE',  ( -162.0762913951020892, -57.76657433524000851, 1.198031840315820329 ) ) ;
#24432=CARTESIAN_POINT ( 'NONE',  ( -162.0762913951020892, 39.99999999999985079, 41.69427287692695216 ) ) ;
#24434=CARTESIAN_POINT ( 'NONE',  ( 22.90311673803743986, 46.98314248934284620, -13.82691048574049475 ) ) ;
#24435=CARTESIAN_POINT ( 'NONE',  ( 151.7948205124836534, 6.767089262349062828, -40.00000000000002132 ) ) ;
#24436=ORIENTED_EDGE ( 'NONE', *, *, #25095, .T. ) ;
#24437=CARTESIAN_POINT ( 'NONE',  ( -91.56559293963834989, -22.67402823373193499, 0.000000000000000000 ) ) ;
#24439=CARTESIAN_POINT ( 'NONE',  ( -4.915070467874388171, -46.68718905935042329, 13.76630780994306846 ) ) ;
#24440=CARTESIAN_POINT ( 'NONE',  ( -259.2033419157646676, 30.48217210827734647, 40.00000000000002132 ) ) ;
#24441=VERTEX_POINT ( 'NONE', #20113 ) ;
#24442=CARTESIAN_POINT ( 'NONE',  ( -109.1264249741463459, 33.12752917270373132, -13.72187187121062557 ) ) ;
#24444=CARTESIAN_POINT ( 'NONE',  ( -3.786831587087837736, -13.84155926340451970, 47.08106124085753663 ) ) ;
#24446=EDGE_CURVE ( 'NONE', #6051, #61, #20824, .T. ) ;
#24448=CARTESIAN_POINT ( 'NONE',  ( -0.1993645192496782403, 18.24262160100998997, -44.04158448241128099 ) ) ;
#24451=B_SPLINE_CURVE_WITH_KNOTS ( 'NONE', 3,
 ( #25736, #13355, #9243, #13606, #17597, #17350 ),
 .UNSPECIFIED., .F., .F.,
 ( 4, 2, 4 ),
 ( -6.000000000996541667E-08, 0.04016968416332604430, 0.08033942832665208478 ),
 .UNSPECIFIED. ) ;
#24453=CARTESIAN_POINT ( 'NONE',  ( -86.86493150571111244, 8.366608963953098055, -19.60045294882791467 ) ) ;
#24454=CARTESIAN_POINT ( 'NONE',  ( -238.4067589809705794, 0.6820004458491113475, -57.25054294077229144 ) ) ;
#24455=CARTESIAN_POINT ( 'NONE',  ( 192.4448373802100889, 20.00000000003945644, 0.000000000000000000 ) ) ;
#24457=CARTESIAN_POINT ( 'NONE',  ( -188.3611024622299510, 13.83140737835798895, -47.01268868735313333 ) ) ;
#24458=CARTESIAN_POINT ( 'NONE',  ( 151.7948205124836250, -23.49921654116371883, 23.49921654116317526 ) ) ;
#24459=CARTESIAN_POINT ( 'NONE',  ( -105.3755690713226585, 41.18208027870575449, 15.38646221621837107 ) ) ;
#24460=CARTESIAN_POINT ( 'NONE',  ( -135.8532207217289454, -30.84685318188649106, 40.00000000000002132 ) ) ;
#24461=CARTESIAN_POINT ( 'NONE',  ( -135.8532207217289738, 30.84685318188643777, -40.00000000000002132 ) ) ;
#24462=CARTESIAN_POINT ( 'NONE',  ( -238.4067589809705794, -40.00000000000005684, -0.9644942799830014124 ) ) ;
#24463=CARTESIAN_POINT ( 'NONE',  ( 170.2234770963711128, -17.36149277826995885, 39.20704971665388427 ) ) ;
#24464=CARTESIAN_POINT ( 'NONE',  ( 98.29820294267328507, -5.160908283042997091, 19.33391160836888290 ) ) ;
#24465=CARTESIAN_POINT ( 'NONE',  ( -280.0000000000000568, 14.14213562373127431, -42.42640687119274645 ) ) ;
#24467=CARTESIAN_POINT ( 'NONE',  ( 170.2234770963711128, -17.36149277826985937, -17.36149277826995174 ) ) ;
#24470=B_SPLINE_CURVE_WITH_KNOTS ( 'NONE', 3,
 ( #3847, #7811, #1325, #15927, #1454, #25552, #9555, #17663 ),
 .UNSPECIFIED., .F., .F.,
 ( 4, 2, 2, 4 ),
 ( 0.0002291277466117084692, 0.002289782534329003541, 0.004350437322046298017, 0.008471746897480886968 ),
 .UNSPECIFIED. ) ;
#24471=CARTESIAN_POINT ( 'NONE',  ( -94.58360650945733994, 8.190527749687760206, 20.91945674502158070 ) ) ;
#24475=CARTESIAN_POINT ( 'NONE',  ( -192.9588430854690273, -38.51493924976932703, -18.05360324515463688 ) ) ;
#24476=CARTESIAN_POINT ( 'NONE',  ( 16.38602454699764976, -44.43226271089463353, -24.50452114743870169 ) ) ;
#24478=CARTESIAN_POINT ( 'NONE',  ( -89.92902785008656963, -20.44110050034138126, 8.088236460649854465 ) ) ;
#24479=DIRECTION ( 'NONE',  ( 0.000000000000000000, -0.3995982397418283427, -0.9166903767331869846 ) ) ;
#24483=CARTESIAN_POINT ( 'NONE',  ( -397.9898987322331436, -3.637015436189069562E-14, 0.000000000000000000 ) ) ;
#24484=CARTESIAN_POINT ( 'NONE',  ( 4.995406935893289102, 10.78321810388998081, 10.78321810389001811 ) ) ;
#24485=CARTESIAN_POINT ( 'NONE',  ( -151.7004448984925773, -32.50164219295758983, -13.46262099560747139 ) ) ;
#24486=CARTESIAN_POINT ( 'NONE',  ( 136.1360204305621551, -40.00000000000001421, 4.966164525586921563 ) ) ;
#24487=CARTESIAN_POINT ( 'NONE',  ( 199.9999999999999432, -20.00000000000006750, 0.000000000000000000 ) ) ;
#24491=CARTESIAN_POINT ( 'NONE',  ( -208.1127848780264742, -40.00000000000025580, 55.00245453014408525 ) ) ;
#24492=CARTESIAN_POINT ( 'NONE',  ( -198.0356074513804572, -40.00000000000025580, 55.37879056871310013 ) ) ;
#24493=CARTESIAN_POINT ( 'NONE',  ( 170.2234770963711128, 40.00000000000000000, 15.44714144992830462 ) ) ;
#24494=CARTESIAN_POINT ( 'NONE',  ( 0.2972598230769983307, -14.33493731733933352, -40.00000000000002132 ) ) ;
#24495=CARTESIAN_POINT ( 'NONE',  ( 14.38125909742183062, -67.30136555898262429, 10.73282306405838682 ) ) ;
#24496=CARTESIAN_POINT ( 'NONE',  ( -86.96347745069645896, 21.75974354311648895, -40.00000000000002132 ) ) ;
#24497=CARTESIAN_POINT ( 'NONE',  ( 184.8905102610680444, 14.79361573936366092, 41.77492675556006674 ) ) ;
#24498=CARTESIAN_POINT ( 'NONE',  ( -238.4067589809705794, -3.369206980223063916E-14, -0.9644942799825824142 ) ) ;
#24500=CARTESIAN_POINT ( 'NONE',  ( 4.995406935893298872, 5.820775922023080204E-13, -55.24977328854835434 ) ) ;
#24501=CARTESIAN_POINT ( 'NONE',  ( 91.82158438592159655, -40.00000000000008527, 22.79471317813456110 ) ) ;
#24502=CARTESIAN_POINT ( 'NONE',  ( -162.0762913951021176, 29.48230308784768638, -27.08623940707612121 ) ) ;
#24506=CARTESIAN_POINT ( 'NONE',  ( 146.6084372240433709, -3.800685668858344801, -52.76785682606520567 ) ) ;
#24508=CARTESIAN_POINT ( 'NONE',  ( -280.0000000000000568, -42.42640687119276066, -14.14213562373147148 ) ) ;
#24510=CARTESIAN_POINT ( 'NONE',  ( 19.06497207195982924, -54.19242893257843008, -2.449293598294708485E-15 ) ) ;
#24511=CARTESIAN_POINT ( 'NONE',  ( 23.37394308801977871, 23.33966569535068203, 42.85717664514594816 ) ) ;
#24512=CARTESIAN_POINT ( 'NONE',  ( -91.56559293963834989, -16.03295912088728414, 16.03295912088688269 ) ) ;
#24513=( NAMED_UNIT ( * ) PLANE_ANGLE_UNIT ( ) SI_UNIT ( $, .RADIAN. ) );
#24514=EDGE_LOOP ( 'NONE', ( #14130, #14356, #5083, #22210, #652, #2426, #25718, #18075, #23825, #13618, #23302, #19173, #19328, #15047, #13848 ) ) ;
#24517=CARTESIAN_POINT ( 'NONE',  ( -53.37769371738607305, -13.65853730965327806, -27.95780717557944328 ) ) ;
#24518=CARTESIAN_POINT ( 'NONE',  ( 22.82148508083373883, 17.87803012130506275, 43.16138278737005862 ) ) ;
#24521=ORIENTED_EDGE ( 'NONE', *, *, #24699, .F. ) ;
#24522=CARTESIAN_POINT ( 'NONE',  ( -135.8532207217289738, -9.153146818113595984, 0.000000000000000000 ) ) ;
#24524=CARTESIAN_POINT ( 'NONE',  ( -190.1760717700867360, -43.55712811731331158, 23.85870456434319209 ) ) ;
#24527=CARTESIAN_POINT ( 'NONE',  ( 5.009866156928143077, 44.71726210619370079, -24.71463403307565088 ) ) ;
#24528=CARTESIAN_POINT ( 'NONE',  ( 163.1118516004056573, 39.99999999999976552, 27.26290988616914746 ) ) ;
#24529=CARTESIAN_POINT ( 'NONE',  ( 146.6084372240433993, -3.357462877844280890E-13, 34.62501878078305850 ) ) ;
#24533=CARTESIAN_POINT ( 'NONE',  ( -188.9524464570897635, 13.86227157644379915, 47.22058047019342553 ) ) ;
#24534=CARTESIAN_POINT ( 'NONE',  ( 23.38399212876534250, -13.80022400692441842, -46.80460545930682059 ) ) ;
#24535=CARTESIAN_POINT ( 'NONE',  ( 130.8568914410475372, -4.207082182992785135, -4.207082182992884611 ) ) ;
#24537=CARTESIAN_POINT ( 'NONE',  ( -30.26275506840324070, -29.48230279907780016, -27.08623969584605362 ) ) ;
#24539=CARTESIAN_POINT ( 'NONE',  ( 146.6084372240433993, 24.48358557860307272, 24.48358557860347418 ) ) ;
#24540=CARTESIAN_POINT ( 'NONE',  ( 91.82158438592156813, 17.20528682183302038, 40.00000000000002132 ) ) ;
#24541=CARTESIAN_POINT ( 'NONE',  ( 192.4448373802100889, 14.14213562375893574, -14.14213562375874922 ) ) ;
#24543=CARTESIAN_POINT ( 'NONE',  ( -86.96347745069643054, -18.24025645688353947, 40.00000000000002132 ) ) ;
#24544=CARTESIAN_POINT ( 'NONE',  ( -110.1022965999516003, 13.49625447730847938, 15.07957642757643413 ) ) ;
#24545=CARTESIAN_POINT ( 'NONE',  ( -30.26275506840324425, 40.00000000000044764, -41.69427246844585255 ) ) ;
#24546=CARTESIAN_POINT ( 'NONE',  ( 192.4448373802100889, -14.14213562375876698, -14.14213562375885047 ) ) ;
#24547=EDGE_CURVE ( 'NONE', #19647, #22653, #13031, .T. ) ;
#24548=CARTESIAN_POINT ( 'NONE',  ( -192.9588430854690273, 14.46834944099966336, -40.00000000000002132 ) ) ;
#24549=ORIENTED_EDGE ( 'NONE', *, *, #16629, .T. ) ;
#24551=CARTESIAN_POINT ( 'NONE',  ( -77.90255099906767100, -8.064892378658175431, 20.29001641120675004 ) ) ;
#24552=CARTESIAN_POINT ( 'NONE',  ( -105.4741150117390021, -7.943527260764932763, -19.77569912954469800 ) ) ;
#24553=CARTESIAN_POINT ( 'NONE',  ( 151.7948205124836534, 33.06932595376333239, 23.49921654116065284 ) ) ;
#24554=CARTESIAN_POINT ( 'NONE',  ( -114.5444905533601343, -20.85462941671032766, -6.798574478272650268 ) ) ;
#24559=CARTESIAN_POINT ( 'NONE',  ( -105.3755690713226585, 41.18208027870575449, 15.38646221621837107 ) ) ;
#24560=CARTESIAN_POINT ( 'NONE',  ( -100.7734535825088500, -12.25131212657524316, 44.31723036834888774 ) ) ;
#24562=CARTESIAN_POINT ( 'NONE',  ( 163.1118516004056573, 39.99999999999976552, 27.26290988616914746 ) ) ;
#24563=CARTESIAN_POINT ( 'NONE',  ( -56.48582580120559982, -21.81201906317804173, 34.75652343174591152 ) ) ;
#24565=CARTESIAN_POINT ( 'NONE',  ( -105.3755690713226727, -15.38646221621786481, -15.38646221621789856 ) ) ;
#24566=CARTESIAN_POINT ( 'NONE',  ( 184.8905102610680444, 14.79361573936396113, -14.79361573936377461 ) ) ;
#24569=CARTESIAN_POINT ( 'NONE',  ( 136.1360204305621266, 5.219216885335291329E-15, 4.966164525587064560 ) ) ;
#24571=CARTESIAN_POINT ( 'NONE',  ( 23.42154907652877327, 46.79103593565408659, -13.79745687233748441 ) ) ;
#24572=CARTESIAN_POINT ( 'NONE',  ( 170.2234770963711128, 15.44714144992819094, 2.449293598294708485E-15 ) ) ;
#24573=FACE_OUTER_BOUND ( 'NONE', #20580, .T. ) ;
#24574=CARTESIAN_POINT ( 'NONE',  ( 0.2972598230769938343, 10.13633138497472252, 10.13633138497475628 ) ) ;
#24575=CARTESIAN_POINT ( 'NONE',  ( -3.439026802539349781, -43.30533194338908487, 17.93765581402033149 ) ) ;
#24576=CARTESIAN_POINT ( 'NONE',  ( 4.995406935893288214, 55.24977328854835434, 2.449293598294708485E-15 ) ) ;
#24578=DIRECTION ( 'NONE',  ( 1.000000000000000000, 0.000000000000000000, 0.000000000000000000 ) ) ;
#24579=CARTESIAN_POINT ( 'NONE',  ( -192.9588430854689989, 10.23066800230742679, 10.23066800230749607 ) ) ;
#24581=CARTESIAN_POINT ( 'NONE',  ( -3.336279363872681536, 17.94861674415367148, -43.33179396957144291 ) ) ;
#24583=CARTESIAN_POINT ( 'NONE',  ( -4.039451493210481026, -46.99046209229796034, -13.82811171175467102 ) ) ;
#24584=CARTESIAN_POINT ( 'NONE',  ( 144.9504669809063557, -30.13886470195709322, 12.48392651407819187 ) ) ;
#24585=CARTESIAN_POINT ( 'NONE',  ( -190.0144721488334767, -13.91469502169458394, 47.57279682960911771 ) ) ;
#24588=CARTESIAN_POINT ( 'NONE',  ( 4.995406935893294431, -17.50105314357144337, -39.06748935135212264 ) ) ;
#24589=CARTESIAN_POINT ( 'NONE',  ( 184.8905102610680444, 20.92133201514447549, 0.000000000000000000 ) ) ;
#24590=CARTESIAN_POINT ( 'NONE',  ( -188.8948648269078774, 17.93710299892656934, -43.30399732969019055 ) ) ;
#24591=CARTESIAN_POINT ( 'NONE',  ( -198.0356074513804572, 39.15871834505887250, 17.40982414986519089 ) ) ;
#24592=CARTESIAN_POINT ( 'NONE',  ( 146.6084372240433993, -24.48358557860353457, 24.48358557860296258 ) ) ;
#24593=CARTESIAN_POINT ( 'NONE',  ( 0.2972598230770129857, -54.33493731733938148, 40.00000000000002132 ) ) ;
#24594=CARTESIAN_POINT ( 'NONE',  ( -162.0762913951021176, 41.69427287672986182, 40.00000000000002132 ) ) ;
#24596=CARTESIAN_POINT ( 'NONE',  ( 200.0000000000000000, -40.00000000000019185, 19.99999999999968381 ) ) ;
#24597=CARTESIAN_POINT ( 'NONE',  ( -100.7734535825088358, 12.25131212657480440, 12.25131212657487012 ) ) ;
#24598=CARTESIAN_POINT ( 'NONE',  ( -93.01741312764252712, 20.50009083229532436, -8.946232117619326019 ) ) ;
#24599=CARTESIAN_POINT ( 'NONE',  ( -280.0000000000000000, -14.14213562373088706, -14.14213562373108424 ) ) ;
#24601=CARTESIAN_POINT ( 'NONE',  ( -114.4364955367323660, -8.064892380834915997, 20.29001642039123610 ) ) ;
#24602=EDGE_CURVE ( 'NONE', #9554, #15971, #5515, .T. ) ;
#24604=CARTESIAN_POINT ( 'NONE',  ( 146.6084372240433709, -52.76785682606516303, 3.800685668858563737 ) ) ;
#24605=CARTESIAN_POINT ( 'NONE',  ( -100.0968563617859530, 8.149320301543554024, 20.72609133245155988 ) ) ;
#24606=CARTESIAN_POINT ( 'NONE',  ( -56.48582580120558561, -21.81201906317785699, 21.81201906317761896 ) ) ;
#24607=CARTESIAN_POINT ( 'NONE',  ( 17.91733029160166168, -44.18858371746068769, -24.32486282486966545 ) ) ;
#24608=ORIENTED_EDGE ( 'NONE', *, *, #20698, .T. ) ;
#24609=CARTESIAN_POINT ( 'NONE',  ( -188.2995950289365226, 23.44932284465886241, 43.00522595870971543 ) ) ;
#24610=CARTESIAN_POINT ( 'NONE',  ( -77.70093066171460805, -11.20685550411562303, -18.98763857597440818 ) ) ;
#24615=CARTESIAN_POINT ( 'NONE',  ( -86.96347745069644475, -15.38646221621786125, -15.38646221621789856 ) ) ;
#24616=CARTESIAN_POINT ( 'NONE',  ( -189.2667921706087952, -43.39860407294495559, -17.97629039507308590 ) ) ;
#24617=CARTESIAN_POINT ( 'NONE',  ( 130.8568914410475088, -39.99999999999988631, -34.05028731879802706 ) ) ;
#24618=CARTESIAN_POINT ( 'NONE',  ( 136.1360204305621266, 4.966164525587089429, 2.449293598294708485E-15 ) ) ;
#24621=CARTESIAN_POINT ( 'NONE',  ( -192.9588430854690273, -40.00000000000011369, 14.46834944099955855 ) ) ;
#24622=CARTESIAN_POINT ( 'NONE',  ( -30.26275506840325136, 40.00000000000001421, 1.694272468446399227 ) ) ;
#24624=CARTESIAN_POINT ( 'NONE',  ( 151.7948205124836250, 33.23291073765556547, 0.000000000000000000 ) ) ;
#24625=CARTESIAN_POINT ( 'NONE',  ( 170.2234770963711128, -15.44714144992812699, -40.00000000000002132 ) ) ;
#24626=CARTESIAN_POINT ( 'NONE',  ( 91.82158438592159655, -16.11829626346147393, 16.11829626346132116 ) ) ;
#24627=CARTESIAN_POINT ( 'NONE',  ( -192.9588430854689989, 1.161019517985663313E-13, -14.46834944099969533 ) ) ;
#24629=CARTESIAN_POINT ( 'NONE',  ( -213.1075012329537230, 5.259461644596141978E-13, -53.71589010951915100 ) ) ;
#24630=CARTESIAN_POINT ( 'NONE',  ( 19.06497207195982924, -40.00000000000021316, 54.19242893257830218 ) ) ;
#24631=CARTESIAN_POINT ( 'NONE',  ( 184.8905102610680444, -14.79361573936379415, -14.79361573936387941 ) ) ;
#24633=CARTESIAN_POINT ( 'NONE',  ( -114.7823189589623780, -14.64951506473200737, 16.64646944814565543 ) ) ;
#24634=CARTESIAN_POINT ( 'NONE',  ( 163.1118516004056573, -9.006482792073960297, -47.56205970284963769 ) ) ;
#24637=CARTESIAN_POINT ( 'NONE',  ( -4.580761711668102087, 42.99740816077407857, -17.81010960708308843 ) ) ;
#24639=CARTESIAN_POINT ( 'NONE',  ( 57.59792236341148453, -37.56421063658185489, -2.449293598294708485E-15 ) ) ;
#24641=CARTESIAN_POINT ( 'NONE',  ( -86.94949953272045207, -6.679047987426590893, -20.30809431151271127 ) ) ;
#24642=CARTESIAN_POINT ( 'NONE',  ( -238.4067589809705794, 0.9644942799825386714, 0.000000000000000000 ) ) ;
#24644=ORIENTED_EDGE ( 'NONE', *, *, #7803, .T. ) ;
#24645=CARTESIAN_POINT ( 'NONE',  ( -97.72675010090222258, 8.987772175319644674, -20.56394680065910308 ) ) ;
#24646=CARTESIAN_POINT ( 'NONE',  ( -94.58360650936646152, 8.190527749686246750, -20.91945674502226282 ) ) ;
#24647=CARTESIAN_POINT ( 'NONE',  ( 21.80824205439611774, 23.67346680102962608, 43.30754100652750083 ) ) ;
#24648=EDGE_LOOP ( 'NONE', ( #2732, #4552, #16149, #729, #24644 ) ) ;
#24651=CARTESIAN_POINT ( 'NONE',  ( -213.1075012329537230, 13.71589010951907994, 0.000000000000000000 ) ) ;
#24653=CARTESIAN_POINT ( 'NONE',  ( -105.2272259197136322, -2.713789710689835655, -21.35019349091949792 ) ) ;
#24654=DIRECTION ( 'NONE',  ( -5.494191223143503443E-14, 0.7071067811865585639, -0.7071067811865364705 ) ) ;
#24655=CARTESIAN_POINT ( 'NONE',  ( -192.9588430854690273, 38.51493924976939098, -18.05360324515436687 ) ) ;
#24656=CARTESIAN_POINT ( 'NONE',  ( -199.9999999999999147, -22.35311919176581696, 45.06067021511796611 ) ) ;
#24657=CARTESIAN_POINT ( 'NONE',  ( 14.32711916788066553, 44.71189734681538397, -24.71075626504571687 ) ) ;
#24659=CARTESIAN_POINT ( 'NONE',  ( -105.3755690713226727, 1.741486606973311632E-13, -18.24025645688352881 ) ) ;
#24660=CARTESIAN_POINT ( 'NONE',  ( 14.38125909742181108, 1.616281842095393922E-13, -15.17850393972633682 ) ) ;
#24664=CARTESIAN_POINT ( 'NONE',  ( -188.2870673237720496, 23.44688076656433751, 43.00153493964062790 ) ) ;
#24665=CARTESIAN_POINT ( 'NONE',  ( 184.8905102610680444, -13.49065550809840630, 43.07788698682565354 ) ) ;
#24666=B_SPLINE_CURVE_WITH_KNOTS ( 'NONE', 3,
 ( #16558, #335, #10045, #20558, #18150, #8303 ),
 .UNSPECIFIED., .F., .F.,
 ( 4, 2, 4 ),
 ( -6.000000014155440701E-08, 0.03937727993095193474, 0.07875461986190401831 ),
 .UNSPECIFIED. ) ;
#24668=CARTESIAN_POINT ( 'NONE',  ( 91.82158438592156813, 40.45024623143950038, 16.11829626348447420 ) ) ;
#24670=CARTESIAN_POINT ( 'NONE',  ( 4.995406935893300648, -10.78321810387790514, -67.35176059880241439 ) ) ;
#24672=CARTESIAN_POINT ( 'NONE',  ( -192.9588430854689989, -14.46834944099973086, 0.000000000000000000 ) ) ;
#24673=CARTESIAN_POINT ( 'NONE',  ( 165.3321726438350368, 18.76308274332837911, -18.76308274332814818 ) ) ;
#24674=CARTESIAN_POINT ( 'NONE',  ( -162.0762913951020892, -1.694272876828353702, 0.000000000000000000 ) ) ;
#24676=CARTESIAN_POINT ( 'NONE',  ( 4.995406935893291767, 40.00000000000059686, -55.24977328853165659 ) ) ;
#24678=CARTESIAN_POINT ( 'NONE',  ( 151.0853911467766011, -12.04115959308015960, 29.06993079631205390 ) ) ;
#24681=CARTESIAN_POINT ( 'NONE',  ( -100.7734535825088358, -22.67402823373193499, 0.000000000000000000 ) ) ;
#24682=CARTESIAN_POINT ( 'NONE',  ( 159.7744820660628591, 10.75261058663732960, 25.95909830917690186 ) ) ;
#24683=CARTESIAN_POINT ( 'NONE',  ( 14.38125909742180397, 67.30136555898270956, -10.73282306405792319 ) ) ;
#24684=CARTESIAN_POINT ( 'NONE',  ( 98.29820294267337033, 18.47759065023124236, -7.653668647303903505 ) ) ;
#24686=CARTESIAN_POINT ( 'NONE',  ( -199.9999999999999716, -49.28189405767602693, 14.17215463606940595 ) ) ;
#24687=CARTESIAN_POINT ( 'NONE',  ( 200.0000000000000000, -59.99999999999992184, 0.000000000000000000 ) ) ;
#24692=CARTESIAN_POINT ( 'NONE',  ( -259.2033419157646676, -35.01439189186523748, -21.55415060305881170 ) ) ;
#24693=CARTESIAN_POINT ( 'NONE',  ( 184.8905102610680444, -13.49065550809840630, 43.07788698682565354 ) ) ;
#24694=CARTESIAN_POINT ( 'NONE',  ( -114.4627503397241384, 20.42543059692667029, 7.807380225631771253 ) ) ;
#24695=CARTESIAN_POINT ( 'NONE',  ( -105.3755690713226585, 39.99999999999977263, 21.75974354311691883 ) ) ;
#24696=CARTESIAN_POINT ( 'NONE',  ( 19.06497207195981858, -38.31983398719641087, 18.24870850772724040 ) ) ;
#24697=CARTESIAN_POINT ( 'NONE',  ( 5.009865950673426660, 14.14399394884953409, 49.09576456953139001 ) ) ;
#24698=FACE_OUTER_BOUND ( 'NONE', #23539, .T. ) ;
#24699=EDGE_CURVE ( 'NONE', #8490, #13725, #14858, .T. ) ;
#24700=CARTESIAN_POINT ( 'NONE',  ( 57.59792236341147031, -26.56190807104670171, -30.00663442387710234 ) ) ;
#24704=CARTESIAN_POINT ( 'NONE',  ( 192.4448373802101173, -40.00000000000005684, 19.99999999996046185 ) ) ;
#24706=CARTESIAN_POINT ( 'NONE',  ( 20.69615274308407393, 43.59383154590945963, -23.88537831999326855 ) ) ;
#24707=CARTESIAN_POINT ( 'NONE',  ( 14.38125909742180752, 55.17850393971008316, -40.00000000000002132 ) ) ;
#24708=CARTESIAN_POINT ( 'NONE',  ( -91.56559293963834989, -16.03295912088706388, -16.03295912088710651 ) ) ;
#24709=CARTESIAN_POINT ( 'NONE',  ( 184.8905102610680444, -20.92133201514440799, 0.000000000000000000 ) ) ;
#24710=CARTESIAN_POINT ( 'NONE',  ( -77.90022806218901508, -20.16431395584850250, 8.352332316461128059 ) ) ;
#24711=AXIS2_PLACEMENT_3D ( 'NONE', #7267, #5411, #13512 ) ;
#24712=CARTESIAN_POINT ( 'NONE',  ( 14.38125909742180752, 55.17850393974265444, 40.00000000000002132 ) ) ;
#24714=CARTESIAN_POINT ( 'NONE',  ( 23.30631261066140780, 23.35506702543256097, -42.87793822514780828 ) ) ;
#24716=CARTESIAN_POINT ( 'NONE',  ( -208.1127848780264742, -17.67593391476659548, 38.89260858015730804 ) ) ;
#24717=CARTESIAN_POINT ( 'NONE',  ( -16.37606550806344785, -16.46709356867778595, 39.75508062653803876 ) ) ;
#24718=CARTESIAN_POINT ( 'NONE',  ( 11.71430589688568169, 14.17293196763019303, -49.28686712666840464 ) ) ;
#24721=DIRECTION ( 'NONE',  ( 0.01051738792036946944, 0.9166396752533303438, -0.3995761383050819293 ) ) ;
#24722=CARTESIAN_POINT ( 'NONE',  ( -197.4153392276050170, -14.14666332908280211, 49.11379398046769040 ) ) ;
#24723=CARTESIAN_POINT ( 'NONE',  ( 130.8568914410475088, -39.99999999999992895, -5.949712681207114606 ) ) ;
#24724=CARTESIAN_POINT ( 'NONE',  ( -91.56559293963834989, -16.03295912088728414, 16.03295912088688269 ) ) ;
#24725=CARTESIAN_POINT ( 'NONE',  ( -90.07798792367796636, -22.27377874500496802, 0.000000000000000000 ) ) ;
#24727=CARTESIAN_POINT ( 'NONE',  ( -188.2871287166139496, 23.44689273421231945, -43.00155302796424905 ) ) ;
#24728=CARTESIAN_POINT ( 'NONE',  ( 170.2234770963711128, 39.20704971665372796, 17.36149277827039583 ) ) ;
#24729=CARTESIAN_POINT ( 'NONE',  ( 136.1360204305621551, 3.511608612530062512, 53.05693388239318864 ) ) ;
#24730=CARTESIAN_POINT ( 'NONE',  ( 14.38125909742182884, -55.17850393974264733, -40.00000000000002132 ) ) ;
#24731=CARTESIAN_POINT ( 'NONE',  ( -208.1127848780265026, 55.00245453012668406, 2.449293598294708485E-15 ) ) ;
#24732=CARTESIAN_POINT ( 'NONE',  ( 192.4448373802101173, -39.99999999999977973, -19.99999999996102673 ) ) ;
#24733=CARTESIAN_POINT ( 'NONE',  ( 200.0000000000000000, -14.14213562373106114, 42.42640687119278908 ) ) ;
#24735=CARTESIAN_POINT ( 'NONE',  ( 14.38125909742182529, -39.01709431150879936, -39.01709431150948859 ) ) ;
#24736=CARTESIAN_POINT ( 'NONE',  ( 199.9999999999999432, 14.14213562373113398, -14.14213562373094923 ) ) ;
#24737=ORIENTED_EDGE ( 'NONE', *, *, #15341, .T. ) ;
#24738=CARTESIAN_POINT ( 'NONE',  ( -213.1075012329537230, -18.58567234101155208, 37.98287015391234434 ) ) ;
#24741=CARTESIAN_POINT ( 'NONE',  ( 170.2234770963711128, 17.36149277826973503, 39.20704971665401217 ) ) ;
#24742=CARTESIAN_POINT ( 'NONE',  ( 17.49521241101099633, -44.30201726250688665, -18.35049639065449867 ) ) ;
#24743=VERTEX_POINT ( 'NONE', #4417 ) ;
#24744=CARTESIAN_POINT ( 'NONE',  ( -99.29480781227000818, -20.80016781325181441, 8.165122821357652327 ) ) ;
#24749=CARTESIAN_POINT ( 'NONE',  ( -1.828631717510329713, 13.94691770814087661, -47.79123445024869454 ) ) ;
#24750=CARTESIAN_POINT ( 'NONE',  ( -190.5535808405085163, -43.70553721440995076, -18.10342626500903052 ) ) ;
#24751=CARTESIAN_POINT ( 'NONE',  ( -105.3755690713226727, -8.549198663894545631E-14, 18.24025645688352881 ) ) ;
#24752=CARTESIAN_POINT ( 'NONE',  ( 151.7948205124836250, 6.767089262349059275, 2.449293598294708485E-15 ) ) ;
#24756=CARTESIAN_POINT ( 'NONE',  ( 19.06497207195981858, -1.881589693694111225E-13, 54.19242893257843008 ) ) ;
#24757=CARTESIAN_POINT ( 'NONE',  ( -259.2033419157646676, 40.00000000000000711, -9.517827891722491884 ) ) ;
#24758=CARTESIAN_POINT ( 'NONE',  ( -90.07798792367799479, 15.74993999324186156, -15.74993999324171234 ) ) ;
#24759=CARTESIAN_POINT ( 'NONE',  ( -192.9588430854690273, -14.46834944099973264, -40.00000000000002132 ) ) ;
#24760=CARTESIAN_POINT ( 'NONE',  ( -280.0000000000000000, -20.00000000000006750, -2.449293598294708485E-15 ) ) ;
#24761=CARTESIAN_POINT ( 'NONE',  ( 57.59792236341148453, 1.722363176414758668, 54.84617931850880268 ) ) ;
#24762=CARTESIAN_POINT ( 'NONE',  ( 118.9130007099546305, -10.68958087202327789, -25.80693111732292166 ) ) ;
#24763=CARTESIAN_POINT ( 'NONE',  ( -110.0904723790853410, 16.34339323355447959, -11.87257855583790800 ) ) ;
#24764=CARTESIAN_POINT ( 'NONE',  ( 146.6084372240433709, 39.99999999999968026, 34.62501878078347772 ) ) ;
#24765=CARTESIAN_POINT ( 'NONE',  ( 14.38125909742182529, -40.00000000000021316, 55.17850393974251944 ) ) ;
#24767=CARTESIAN_POINT ( 'NONE',  ( -175.9235640283763757, -42.70623598288129585, -12.95568063866271480 ) ) ;
#24768=CARTESIAN_POINT ( 'NONE',  ( -114.5523123854248695, -19.58652998792717881, 9.959192389756644559 ) ) ;
#24769=CARTESIAN_POINT ( 'NONE',  ( 4.995406935893297984, -39.06748935135182421, -17.50105314357212549 ) ) ;
#24772=CARTESIAN_POINT ( 'NONE',  ( 127.8236149080042878, 28.75948073575762720, -11.91256696755847067 ) ) ;
#24773=CARTESIAN_POINT ( 'NONE',  ( -135.8532207217289454, -30.84685318188648750, -40.00000000000002132 ) ) ;
#24775=CARTESIAN_POINT ( 'NONE',  ( 169.9999999999674571, -17.64300463372919836, -17.64300463252165585 ) ) ;
#24776=CARTESIAN_POINT ( 'NONE',  ( -198.0356074513804572, 10.87444709759730088, -10.87444709759707173 ) ) ;
#24778=ORIENTED_EDGE ( 'NONE', *, *, #19245, .T. ) ;
#24781=CARTESIAN_POINT ( 'NONE',  ( -93.01741312759801872, 8.946232117438750464, -20.50009083235881135 ) ) ;
#24782=CARTESIAN_POINT ( 'NONE',  ( 22.75856136761766635, 17.88529938203902958, 43.17893233522205065 ) ) ;
#24786=CARTESIAN_POINT ( 'NONE',  ( -105.3755690713226585, -15.38646221621796251, 41.18208027870593924 ) ) ;
#24788=CARTESIAN_POINT ( 'NONE',  ( -105.2054292635175869, -15.19799821370180126, -15.19799821370278892 ) ) ;
#24789=CARTESIAN_POINT ( 'NONE',  ( -105.4894168351564048, 19.67999904371083275, 8.151722511394638104 ) ) ;
#24790=CARTESIAN_POINT ( 'NONE',  ( -199.9999999999999147, -16.85576820966601019, 47.13392792189009839 ) ) ;
#24791=EDGE_CURVE ( 'NONE', #23081, #3931, #119, .T. ) ;
#24794=CARTESIAN_POINT ( 'NONE',  ( 14.38125909742180930, 40.00000000000060396, -55.17850393974224232 ) ) ;
#24795=CARTESIAN_POINT ( 'NONE',  ( 151.7948205124836534, 39.99999999999970157, 33.23291073765595627 ) ) ;
#24797=DIRECTION ( 'NONE',  ( 0.000000000000000000, 1.000000000000000000, 0.000000000000000000 ) ) ;
#24799=CARTESIAN_POINT ( 'NONE',  ( -189.5227390968106818, 18.00253259953367291, 43.46195835885502845 ) ) ;
#24800=CARTESIAN_POINT ( 'NONE',  ( -135.8532207217289738, -21.81201906317806305, 34.75652343174590442 ) ) ;
#24801=DIRECTION ( 'NONE',  ( 1.000000000000000000, 1.836970198721025990E-16, 0.000000000000000000 ) ) ;
#24802=CARTESIAN_POINT ( 'NONE',  ( 4.995406935893301537, -10.78321810390187530, 67.35176059882529387 ) ) ;
#24804=CARTESIAN_POINT ( 'NONE',  ( -135.8532207217289738, 34.75652343174625258, -21.81201906317744132 ) ) ;
#24806=CARTESIAN_POINT ( 'NONE',  ( -105.3755690713226869, 21.75974354311648540, -0.000000000000000000 ) ) ;
#24807=CARTESIAN_POINT ( 'NONE',  ( 91.82158438592158234, -12.16597498397778843, 12.16597498397750954 ) ) ;
#24808=CARTESIAN_POINT ( 'NONE',  ( 136.1360204305621266, 35.03383547441298163, 40.00000000000002132 ) ) ;
#24810=CARTESIAN_POINT ( 'NONE',  ( 57.59792236341147742, 4.064940816252731242E-13, -37.56421063658186199 ) ) ;
#24812=CARTESIAN_POINT ( 'NONE',  ( 144.9504669809063273, -12.48392651407863596, 30.13886470195687295 ) ) ;
#24815=CARTESIAN_POINT ( 'NONE',  ( -91.56559293963834989, 17.32597176626808988, 40.00000000000002132 ) ) ;
#24817=CARTESIAN_POINT ( 'NONE',  ( 146.6084372240433709, 32.08495691632030145, 24.48358557860365181 ) ) ;
#24818=B_SPLINE_CURVE_WITH_KNOTS ( 'NONE', 3,
 ( #23201, #19576, #21706, #15070, #21205, #5479, #19701, #9341, #11208, #19323, #9465, #2977, #17449, #11085, #13579, #25588 ),
 .UNSPECIFIED., .F., .F.,
 ( 4, 2, 2, 2, 2, 2, 2, 4 ),
 ( -5.998499569545109335E-08, 0.003520343011582055190, 0.007040746008159805801, 0.01408155200131531309, 0.01760195499789306978, 0.02112235799447082299, 0.02464276099104858314, 0.02816316398762633982 ),
 .UNSPECIFIED. ) ;
#24819=CARTESIAN_POINT ( 'NONE',  ( -114.6375327213568340, -21.34761811098216455, 5.510795915293953406 ) ) ;
#24820=CARTESIAN_POINT ( 'NONE',  ( -163.5815439473242634, 12.03526835478819557, -38.33196286486828797 ) ) ;
#24825=CARTESIAN_POINT ( 'NONE',  ( -56.48582580120559982, -6.472252184283581400, -50.09629031063973059 ) ) ;
#24826=CARTESIAN_POINT ( 'NONE',  ( -100.7734535825088500, 16.03295912088691821, 16.03295912088721309 ) ) ;
#24827=CARTESIAN_POINT ( 'NONE',  ( 170.0000000000000000, 3.122849337825751958E-14, 0.000000000000000000 ) ) ;
#24828=CARTESIAN_POINT ( 'NONE',  ( -100.7734535825088500, 39.99999999999976552, 22.67402823373233645 ) ) ;
#24829=CARTESIAN_POINT ( 'NONE',  ( 151.7948205124836250, 23.49921654116328540, 23.49921654116366554 ) ) ;
#24830=CARTESIAN_POINT ( 'NONE',  ( 20.59573805978978456, 13.93986955483944534, 47.74081960064682306 ) ) ;
#24831=CARTESIAN_POINT ( 'NONE',  ( -208.1127848780265026, 10.60833733269537049, 10.60833733269544510 ) ) ;
#24832=CARTESIAN_POINT ( 'NONE',  ( -208.1127848780264742, -38.89260858015758515, 38.89260858015713751 ) ) ;
#24835=CARTESIAN_POINT ( 'NONE',  ( -30.26275506840323359, -1.535832457777009877E-13, 41.69427246844629309 ) ) ;
#24837=CARTESIAN_POINT ( 'NONE',  ( 22.86726691379442045, 43.14849715852157885, -17.87269271907634760 ) ) ;
#24838=CARTESIAN_POINT ( 'NONE',  ( 4.995406935893288214, 15.24977328854832770, -40.00000000000002132 ) ) ;
#24839=CARTESIAN_POINT ( 'NONE',  ( -238.4067589809705794, -27.60227080167069147, 28.96627169325319429 ) ) ;
#24840=CARTESIAN_POINT ( 'NONE',  ( 0.2972598230769930017, 54.33493731733936016, 40.00000000000002132 ) ) ;
#24841=CARTESIAN_POINT ( 'NONE',  ( -17.28139728210402382, -42.38047544432864555, 12.88180358343662846 ) ) ;
#24842=CARTESIAN_POINT ( 'NONE',  ( 163.1118516004056573, -27.26290988616869626, 40.00000000000002132 ) ) ;
#24843=ORIENTED_EDGE ( 'NONE', *, *, #15245, .F. ) ;
#24844=CARTESIAN_POINT ( 'NONE',  ( 23.23639021239541691, 23.37084785298121403, -42.89921396172169921 ) ) ;
#24845=CARTESIAN_POINT ( 'NONE',  ( 151.7948205124836250, -23.49921654116339553, -23.49921654116350211 ) ) ;
#24846=CARTESIAN_POINT ( 'NONE',  ( -4.151555265633219527, -23.42746911247767017, 42.97219445042060926 ) ) ;
#24848=CARTESIAN_POINT ( 'NONE',  ( -3.786831587087909679, 13.84155926340511478, -47.08106124085716004 ) ) ;
#24850=CARTESIAN_POINT ( 'NONE',  ( -208.1127848780264742, 38.89260858015707356, 17.67593391476696141 ) ) ;
#24851=CARTESIAN_POINT ( 'NONE',  ( -77.78745312850900007, -20.88824371468822250, 6.815361097891073250 ) ) ;
#24853=CARTESIAN_POINT ( 'NONE',  ( -192.6563370915827420, -18.27409561807003868, 44.11756948122302191 ) ) ;
#24854=CARTESIAN_POINT ( 'NONE',  ( -238.4067589809705794, -0.6820004457913585449, -0.6820004457913265705 ) ) ;
#24855=CARTESIAN_POINT ( 'NONE',  ( 136.1360204305621551, -53.05693388239309627, -3.511608612531332163 ) ) ;
#24856=CARTESIAN_POINT ( 'NONE',  ( -259.2033419157646676, 35.01439189186559275, -21.55415060305807984 ) ) ;
#24857=CARTESIAN_POINT ( 'NONE',  ( 130.8568914410475372, 24.07718906447210472, 24.07718906447249907 ) ) ;
#24858=CARTESIAN_POINT ( 'NONE',  ( 184.8905102610680444, 13.49065550809826952, -13.49065550809790359 ) ) ;
#24859=CARTESIAN_POINT ( 'NONE',  ( 151.7948205124836534, 4.785054706297857230, 51.78348778862544322 ) ) ;
#24860=CARTESIAN_POINT ( 'NONE',  ( 4.995406935893307754, -55.24977328854835434, -2.449293598294708485E-15 ) ) ;
#24861=CARTESIAN_POINT ( 'NONE',  ( -259.2033419157646676, 30.48217210827734647, 2.449293598294708485E-15 ) ) ;
#24862=CARTESIAN_POINT ( 'NONE',  ( 4.995406935893297984, -39.99999999999986500, -15.24977328854874870 ) ) ;
#24863=CARTESIAN_POINT ( 'NONE',  ( -238.4067589809705794, 0.6820004457912757223, 0.6820004457913219076 ) ) ;
#24864=FACE_OUTER_BOUND ( 'NONE', #21711, .T. ) ;
#24866=CARTESIAN_POINT ( 'NONE',  ( 200.0000000000000000, 14.14213562373142352, -42.42640687119268961 ) ) ;
#24867=CARTESIAN_POINT ( 'NONE',  ( -100.7734535825088500, 16.03295912088713848, -16.03295912088698927 ) ) ;
#24868=ORIENTED_EDGE ( 'NONE', *, *, #20621, .T. ) ;
#24869=CARTESIAN_POINT ( 'NONE',  ( -135.8532207217289738, 21.81201906317767936, 21.81201906317778239 ) ) ;
#24872=CARTESIAN_POINT ( 'NONE',  ( -162.0762913951020892, -29.48230308784785692, 29.48230308784751230 ) ) ;
#24873=CARTESIAN_POINT ( 'NONE',  ( -4.022465846214346996, -43.01021959554127250, -23.45302613997624874 ) ) ;
#24875=CARTESIAN_POINT ( 'NONE',  ( -4.039451493210481026, -46.99046209229796034, -13.82811171175467102 ) ) ;
#24876=DIRECTION ( 'NONE',  ( -0.01051738777842141370, -0.9166396752737698828, 0.3995761382619288926 ) ) ;
#24877=VERTEX_POINT ( 'NONE', #4550 ) ;
#24879=CARTESIAN_POINT ( 'NONE',  ( -114.6318783467508240, -21.31802243455910784, -5.473070270850431740 ) ) ;
#24880=CARTESIAN_POINT ( 'NONE',  ( -280.0000000000000000, 19.99999999999996092, 2.449293598294708485E-15 ) ) ;
#24885=CARTESIAN_POINT ( 'NONE',  ( -91.56559293963836410, -12.25131212657524138, 44.31723036834888774 ) ) ;
#24886=CARTESIAN_POINT ( 'NONE',  ( -162.0762913951020892, 39.99999999999985079, 41.69427287692695216 ) ) ;
#24887=CARTESIAN_POINT ( 'NONE',  ( -208.1127848780264742, 39.99999999999979394, 55.00245453010936103 ) ) ;
#24888=CARTESIAN_POINT ( 'NONE',  ( -86.86493150571116928, -8.366608963953867217, -19.60045294882765887 ) ) ;
#24889=CARTESIAN_POINT ( 'NONE',  ( -86.96347745069645896, 21.75974354311648895, -40.00000000000002132 ) ) ;
#24891=CARTESIAN_POINT ( 'NONE',  ( 184.8905102610680444, -19.07866798485553872, -40.00000000000002132 ) ) ;
#24892=CARTESIAN_POINT ( 'NONE',  ( -238.4067589809705794, 27.60227080167040370, 28.96627169325338613 ) ) ;
#24893=CARTESIAN_POINT ( 'NONE',  ( 121.8740240556053180, -11.10671848392261829, -26.81399039734618839 ) ) ;
#24894=CARTESIAN_POINT ( 'NONE',  ( -110.0791661673351172, 10.82529631555651761, -17.04053483147850301 ) ) ;
#24895=CARTESIAN_POINT ( 'NONE',  ( 14.38125909742181818, 5.830552384690105017E-13, -55.17850393972636880 ) ) ;
#24896=CARTESIAN_POINT ( 'NONE',  ( -86.96347745069645896, 39.99999999999994316, 18.24025645688366737 ) ) ;
#24898=CARTESIAN_POINT ( 'NONE',  ( -114.4364955367323091, -20.29001642039124675, -8.064892380834873364 ) ) ;
#24899=CARTESIAN_POINT ( 'NONE',  ( -114.5450021253288782, -9.945938879692020507, 19.55077795857343403 ) ) ;
#24900=CARTESIAN_POINT ( 'NONE',  ( 0.2972598230770100991, -38.42060263243686791, 38.42060263243645579 ) ) ;
#24902=CARTESIAN_POINT ( 'NONE',  ( -30.26275506840324070, -1.198031551616016266, -1.198031551616031587 ) ) ;
#24904=CARTESIAN_POINT ( 'NONE',  ( 144.9504669809064694, 30.13886470195707545, -12.48392651407830911 ) ) ;
#24905=CARTESIAN_POINT ( 'NONE',  ( 151.7948205124835681, 33.23291073765556547, -40.00000000000002132 ) ) ;
#24907=CARTESIAN_POINT ( 'NONE',  ( 192.4448373802100889, -14.14213562375896061, 14.14213562375865330 ) ) ;
#24911=VERTEX_POINT ( 'NONE', #10520 ) ;
#24915=CARTESIAN_POINT ( 'NONE',  ( -105.4741150117382205, 7.943527260749760899, -19.77569912955142684 ) ) ;
#24916=CARTESIAN_POINT ( 'NONE',  ( 22.57783252599927337, 17.90541116499370844, 43.22748647440086955 ) ) ;
#24919=CARTESIAN_POINT ( 'NONE',  ( -259.2033419157646676, -6.730120644403667640, 49.83842185052029805 ) ) ;
#24921=CARTESIAN_POINT ( 'NONE',  ( -105.2055636155232889, -1.377569041481722545, 21.49233843348530115 ) ) ;
#24922=CARTESIAN_POINT ( 'NONE',  ( -198.0356074513804572, -17.40982414986482141, 39.15871834505909987 ) ) ;
#24924=CARTESIAN_POINT ( 'NONE',  ( -91.56559293963834989, -16.03295912088706388, -16.03295912088710651 ) ) ;
#24925=CARTESIAN_POINT ( 'NONE',  ( -213.1075012329537230, 39.99999999999979394, 53.71589010950180665 ) ) ;
#24929=CARTESIAN_POINT ( 'NONE',  ( 4.995406935893291767, 40.00000000000059686, -55.24977328853165659 ) ) ;
#24930=CARTESIAN_POINT ( 'NONE',  ( -100.7734535825088500, 39.99999999999976552, 22.67402823373233645 ) ) ;
#24931=CARTESIAN_POINT ( 'NONE',  ( 170.0000000000000853, 9.369682556672316309, -22.62041470344884075 ) ) ;
#24935=CARTESIAN_POINT ( 'NONE',  ( -185.5190358316759500, 17.55874045217352020, 42.39054933781988410 ) ) ;
#24936=CARTESIAN_POINT ( 'NONE',  ( 57.59792236341147031, -26.56190807104712448, 30.00663442387673285 ) ) ;
#24937=EDGE_CURVE ( 'NONE', #9554, #151, #19480, .T. ) ;
#24938=( BOUNDED_SURFACE ( )  B_SPLINE_SURFACE ( 3, 3, ( 
 ( #14012, #18402, #2055, #47, #5768, #10162, #16411, #26141, #9761, #1919, #3779, #13877, #8160, #16273, #4053, #10024, #12154, #26283, #24402, #8022, #7885, #6168, #22415, #24539, #4191, #6295, #14413, #22543, #22010, #11883 ),
 ( #20003, #16138, #24269, #1789, #9893, #17996, #6042, #22279, #24804, #10962, #4447, #10555, #22806, #25071, #4583, #22936, #18536, #8419, #16540, #4846, #19069, #6556, #17069, #4323, #10826, #8694, #20539, #16805, #10419, #4716 ),
 ( #850, #14940, #20943, #12680, #24942, #14544, #12952, #12542, #6690, #12413, #23075, #21070, #318, #2854, #25203, #2310, #24670, #8960, #6950, #12821, #18941, #2443, #16673, #2581, #18667, #721, #6426, #15068, #454, #14670 ),
 ( #2721, #8826, #22674, #20810, #20674, #10696, #6822, #8558, #18807, #587, #14804, #16936, #1234, #7460, #9463, #23199, #13329, #11083, #19321, #9086, #3350, #11579, #21704, #25707, #19699, #4979, #17447, #5477, #13086, #15324 ),
 ( #19446, #1105, #1365, #5350, #1487, #13457, #15573, #17698, #11450, #23697, #21203, #981, #17192, #9593, #13577, #3102, #21451, #19199, #25458, #25842, #17570, #7209, #21331, #3482, #7332, #9339, #21576, #11206, #7586, #23329 ),
 ( #2975, #25330, #17324, #7087, #15201, #19574, #25586, #5104, #15445, #13209, #23573, #3226, #11330, #9213, #23451, #5225, #7847, #1885, #25976, #16241, #23957, #9990, #23822, #13, #24370, #14241, #10259, #24234, #9859, #21836 ),
 ( #5605, #22381, #7984, #22243, #9727, #15698, #13837, #13711, #22108, #5732, #1620, #6133, #21971, #15968, #18100, #3605, #8124, #4157, #12252, #18369, #6007, #17961, #11715, #19834, #17829, #26249, #20374, #16102, #3884, #26108 ) ),
 .UNSPECIFIED., .T., .F., .F. ) 
 B_SPLINE_SURFACE_WITH_KNOTS ( ( 4, 3, 4 ),
 ( 4, 2, 2, 2, 2, 2, 2, 2, 2, 2, 2, 2, 2, 2, 4 ),
 ( 0.000000000000000000, 0.5000000000000000000, 1.000000000000000000 ),
 ( 0.000000000000000000, 0.1357259735107005372, 0.1651108541090157700, 0.1944957347073310028, 0.3598804999793158710, 0.3867117631979620773, 0.4135430264166082281, 0.5789277916885930964, 0.6062785021374117456, 0.6336292125862302838, 0.8508620842112317728, 0.8814014469398914198, 0.9119408096685510667, 0.9559704048342755334, 1.000000000000000000 ),
 .UNSPECIFIED. ) 
 GEOMETRIC_REPRESENTATION_ITEM ( )  RATIONAL_B_SPLINE_SURFACE ( (
 ( 1.000000000000000000, 1.000000000000000000, 1.000000000000000000, 1.000000000000000000, 1.000000000000000000, 1.000000000000000000, 1.000000000000000000, 1.000000000000000000, 1.000000000000000000, 1.000000000000000000, 1.000000000000000000, 1.000000000000000000, 1.000000000000000000, 1.000000000000000000, 1.000000000000000000, 1.000000000000000000, 1.000000000000000000, 1.000000000000000000, 1.000000000000000000, 1.000000000000000000, 1.000000000000000000, 1.000000000000000000, 1.000000000000000000, 1.000000000000000000, 1.000000000000000000, 1.000000000000000000, 1.000000000000000000, 1.000000000000000000, 1.000000000000000000, 1.000000000000000000),
 ( 0.3333333333333333703, 0.3333333333333333703, 0.3333333333333333703, 0.3333333333333333703, 0.3333333333333333703, 0.3333333333333333703, 0.3333333333333333703, 0.3333333333333333703, 0.3333333333333333703, 0.3333333333333333703, 0.3333333333333333703, 0.3333333333333333703, 0.3333333333333333703, 0.3333333333333333703, 0.3333333333333333703, 0.3333333333333333703, 0.3333333333333333703, 0.3333333333333333703, 0.3333333333333333703, 0.3333333333333333703, 0.3333333333333333703, 0.3333333333333333703, 0.3333333333333333703, 0.3333333333333333703, 0.3333333333333333703, 0.3333333333333333703, 0.3333333333333333703, 0.3333333333333333703, 0.3333333333333333703, 0.3333333333333333703),
 ( 0.3333333333333333703, 0.3333333333333333703, 0.3333333333333333703, 0.3333333333333333703, 0.3333333333333333703, 0.3333333333333333703, 0.3333333333333333703, 0.3333333333333333703, 0.3333333333333333703, 0.3333333333333333703, 0.3333333333333333703, 0.3333333333333333703, 0.3333333333333333703, 0.3333333333333333703, 0.3333333333333333703, 0.3333333333333333703, 0.3333333333333333703, 0.3333333333333333703, 0.3333333333333333703, 0.3333333333333333703, 0.3333333333333333703, 0.3333333333333333703, 0.3333333333333333703, 0.3333333333333333703, 0.3333333333333333703, 0.3333333333333333703, 0.3333333333333333703, 0.3333333333333333703, 0.3333333333333333703, 0.3333333333333333703),
 ( 1.000000000000000000, 1.000000000000000000, 1.000000000000000000, 1.000000000000000000, 1.000000000000000000, 1.000000000000000000, 1.000000000000000000, 1.000000000000000000, 1.000000000000000000, 1.000000000000000000, 1.000000000000000000, 1.000000000000000000, 1.000000000000000000, 1.000000000000000000, 1.000000000000000000, 1.000000000000000000, 1.000000000000000000, 1.000000000000000000, 1.000000000000000000, 1.000000000000000000, 1.000000000000000000, 1.000000000000000000, 1.000000000000000000, 1.000000000000000000, 1.000000000000000000, 1.000000000000000000, 1.000000000000000000, 1.000000000000000000, 1.000000000000000000, 1.000000000000000000),
 ( 0.3333333333333333703, 0.3333333333333333703, 0.3333333333333333703, 0.3333333333333333703, 0.3333333333333333703, 0.3333333333333333703, 0.3333333333333333703, 0.3333333333333333703, 0.3333333333333333703, 0.3333333333333333703, 0.3333333333333333703, 0.3333333333333333703, 0.3333333333333333703, 0.3333333333333333703, 0.3333333333333333703, 0.3333333333333333703, 0.3333333333333333703, 0.3333333333333333703, 0.3333333333333333703, 0.3333333333333333703, 0.3333333333333333703, 0.3333333333333333703, 0.3333333333333333703, 0.3333333333333333703, 0.3333333333333333703, 0.3333333333333333703, 0.3333333333333333703, 0.3333333333333333703, 0.3333333333333333703, 0.3333333333333333703),
 ( 0.3333333333333333703, 0.3333333333333333703, 0.3333333333333333703, 0.3333333333333333703, 0.3333333333333333703, 0.3333333333333333703, 0.3333333333333333703, 0.3333333333333333703, 0.3333333333333333703, 0.3333333333333333703, 0.3333333333333333703, 0.3333333333333333703, 0.3333333333333333703, 0.3333333333333333703, 0.3333333333333333703, 0.3333333333333333703, 0.3333333333333333703, 0.3333333333333333703, 0.3333333333333333703, 0.3333333333333333703, 0.3333333333333333703, 0.3333333333333333703, 0.3333333333333333703, 0.3333333333333333703, 0.3333333333333333703, 0.3333333333333333703, 0.3333333333333333703, 0.3333333333333333703, 0.3333333333333333703, 0.3333333333333333703),
 ( 1.000000000000000000, 1.000000000000000000, 1.000000000000000000, 1.000000000000000000, 1.000000000000000000, 1.000000000000000000, 1.000000000000000000, 1.000000000000000000, 1.000000000000000000, 1.000000000000000000, 1.000000000000000000, 1.000000000000000000, 1.000000000000000000, 1.000000000000000000, 1.000000000000000000, 1.000000000000000000, 1.000000000000000000, 1.000000000000000000, 1.000000000000000000, 1.000000000000000000, 1.000000000000000000, 1.000000000000000000, 1.000000000000000000, 1.000000000000000000, 1.000000000000000000, 1.000000000000000000, 1.000000000000000000, 1.000000000000000000, 1.000000000000000000, 1.000000000000000000) ) ) 
 REPRESENTATION_ITEM ( '' )  SURFACE ( )  );
#24940=CARTESIAN_POINT ( 'NONE',  ( 91.82158438592159655, 12.16597498400028776, 44.40256751092339016 ) ) ;
#24942=CARTESIAN_POINT ( 'NONE',  ( -208.1127848780264742, -10.60833733270725787, -67.17687982763172272 ) ) ;
#24944=CARTESIAN_POINT ( 'NONE',  ( 151.7948205124836250, 33.23291073765556547, 0.000000000000000000 ) ) ;
#24946=CARTESIAN_POINT ( 'NONE',  ( -30.26275506840325136, 29.48230279907760121, 27.08623969584625613 ) ) ;
#24947=CARTESIAN_POINT ( 'NONE',  ( -208.1127848780264742, -15.00245453012673202, 40.00000000000002132 ) ) ;
#24950=CARTESIAN_POINT ( 'NONE',  ( -213.1075012329537230, -39.99999999999991473, -13.71589010951953647 ) ) ;
#24957=CARTESIAN_POINT ( 'NONE',  ( 151.7948205124836534, 6.767089262349056611, 40.00000000000002132 ) ) ;
#24959=CARTESIAN_POINT ( 'NONE',  ( -110.0960685945383091, -20.07406508573906834, -2.528047301430426330 ) ) ;
#24961=CARTESIAN_POINT ( 'NONE',  ( -163.5815439473248603, -12.03526835478804635, 38.33196286486853666 ) ) ;
#24962=CARTESIAN_POINT ( 'NONE',  ( -135.8532207217289738, 7.002209520526292428E-15, -9.153146818113572891 ) ) ;
#24964=CARTESIAN_POINT ( 'NONE',  ( -105.2276019244895053, 2.726957955475640016, -21.34775676748449769 ) ) ;
#24965=CARTESIAN_POINT ( 'NONE',  ( -192.9588430854690273, -18.05360324515400094, -38.51493924976961836 ) ) ;
#24966=CARTESIAN_POINT ( 'NONE',  ( -259.2033419157646676, 6.730120644403426944, 6.730120644403592145 ) ) ;
#24967=CARTESIAN_POINT ( 'NONE',  ( -110.1017833366170748, -14.28014421838191694, -14.28014421838201287 ) ) ;
#24968=CARTESIAN_POINT ( 'NONE',  ( 130.8568914410475088, 39.99999999999969447, 34.05028731879830417 ) ) ;
#24969=CARTESIAN_POINT ( 'NONE',  ( 151.7948205124835681, -4.785054706298876859, 51.78348778862533663 ) ) ;
#24970=CARTESIAN_POINT ( 'NONE',  ( -4.039451493210489019, 13.82811171175440812, 46.99046209229809534 ) ) ;
#24971=CARTESIAN_POINT ( 'NONE',  ( -259.2033419157646676, -6.730120644403570829, -6.730120644403545960 ) ) ;
#24972=CARTESIAN_POINT ( 'NONE',  ( 130.8568914410475372, -4.207082182992846420, 4.207082182992822439 ) ) ;
#24975=CARTESIAN_POINT ( 'NONE',  ( -91.56559293963834989, 6.234561990864368500E-14, -22.67402823373191723 ) ) ;
#24976=CARTESIAN_POINT ( 'NONE',  ( 37.15749683989781005, 38.58455518501556014, -20.52531616266200132 ) ) ;
#24977=CARTESIAN_POINT ( 'NONE',  ( -162.0762913951020892, 1.694272876828294194, 0.000000000000000000 ) ) ;
#24978=CARTESIAN_POINT ( 'NONE',  ( 200.0000000000000000, -42.42640687119293119, 14.14213562373082134 ) ) ;
#24979=CARTESIAN_POINT ( 'NONE',  ( 130.8568914410475088, -34.05028731879786363, 40.00000000000002132 ) ) ;
#24981=CARTESIAN_POINT ( 'NONE',  ( 3.774039766349060354, -44.61221010186880420, 18.47898247163330154 ) ) ;
#24982=CARTESIAN_POINT ( 'NONE',  ( 151.7948205124836534, 6.767089262349056611, 40.00000000000002132 ) ) ;
#24983=ORIENTED_EDGE ( 'NONE', *, *, #43, .F. ) ;
#24984=CARTESIAN_POINT ( 'NONE',  ( 0.4311942631275938465, 24.25071831022430402, -44.08816696360397458 ) ) ;
#24985=CARTESIAN_POINT ( 'NONE',  ( -259.2033419157646676, -6.730120644403570829, -6.730120644403545960 ) ) ;
#24986=CARTESIAN_POINT ( 'NONE',  ( -4.121597284766226998, -13.82232031191914245, 46.96202426942505070 ) ) ;
#24987=CARTESIAN_POINT ( 'NONE',  ( 6.371015797563456928, 18.55864253217522020, -44.80452650039788409 ) ) ;
#24989=CARTESIAN_POINT ( 'NONE',  ( 19.06497207195979726, 38.31983398719604139, 18.24870850772803976 ) ) ;
#24990=CARTESIAN_POINT ( 'NONE',  ( -87.10437264497180365, -21.30276644672514053, 2.718829733159835005 ) ) ;
#24991=CARTESIAN_POINT ( 'NONE',  ( -109.1264249741455785, -13.72187187124632501, -33.12752917268957731 ) ) ;
#24992=CARTESIAN_POINT ( 'NONE',  ( -188.8753834511958019, -17.93496043754513991, 43.29882472894604462 ) ) ;
#24993=CARTESIAN_POINT ( 'NONE',  ( -208.1127848780265026, -10.60833733269537227, -10.60833733269551793 ) ) ;
#24994=CARTESIAN_POINT ( 'NONE',  ( 146.6084372240433709, 24.48358557860311180, 32.08495691632071356 ) ) ;
#24995=CARTESIAN_POINT ( 'NONE',  ( -86.96347745069644475, -15.38646221621807442, 15.38646221621768184 ) ) ;
#24996=CARTESIAN_POINT ( 'NONE',  ( -280.0000000000000568, 42.42640687119294540, -14.14213562373059041 ) ) ;
#24997=CARTESIAN_POINT ( 'NONE',  ( -30.26275506840324070, -1.198031551616016266, -1.198031551616031587 ) ) ;
#24998=CARTESIAN_POINT ( 'NONE',  ( -280.0000000000000000, 14.14213562373108246, -14.14213562373078581 ) ) ;
#24999=CARTESIAN_POINT ( 'NONE',  ( -91.56559293963834989, -16.03295912088728414, 16.03295912088688269 ) ) ;
#25000=CARTESIAN_POINT ( 'NONE',  ( 170.2234770963711128, -15.44714144992813409, 40.00000000000002132 ) ) ;
#25001=CARTESIAN_POINT ( 'NONE',  ( -198.0356074513804572, 15.37879056873066830, -40.00000000000002132 ) ) ;
#25002=CARTESIAN_POINT ( 'NONE',  ( 136.1360204305621551, 3.511608612530801032, -53.05693388239316022 ) ) ;
#25003=CARTESIAN_POINT ( 'NONE',  ( -103.9663809734080786, 19.92521373365561033, -8.574562932722885833 ) ) ;
#25004=CARTESIAN_POINT ( 'NONE',  ( -259.2033419157646676, 6.730120644403918995, -49.83842185052024831 ) ) ;
#25006=ORIENTED_EDGE ( 'NONE', *, *, #8079, .T. ) ;
#25007=CARTESIAN_POINT ( 'NONE',  ( -162.0762913951021176, 1.198031840315997298, 57.76657433523996588 ) ) ;
#25008=CARTESIAN_POINT ( 'NONE',  ( -82.30220482034329166, -18.51665893431366072, -7.992411108784819085 ) ) ;
#25009=CARTESIAN_POINT ( 'NONE',  ( 170.2234770963711128, -10.92277846919202666, 10.92277846919193962 ) ) ;
#25010=CARTESIAN_POINT ( 'NONE',  ( -3.434479974377945499, -43.30650750418227091, -17.93814274724467239 ) ) ;
#25012=CARTESIAN_POINT ( 'NONE',  ( -105.4741150117398263, -19.77569912953930498, 7.943527260776862775 ) ) ;
#25013=CARTESIAN_POINT ( 'NONE',  ( -114.5516609237780585, -9.951797154676993884, -19.58913668464228053 ) ) ;
#25016=CARTESIAN_POINT ( 'NONE',  ( -259.2033419157646676, 30.48217210827734647, 2.449293598294708485E-15 ) ) ;
#25019=EDGE_CURVE ( 'NONE', #2784, #19812, #17271, .T. ) ;
#25020=CARTESIAN_POINT ( 'NONE',  ( -192.9588430854690273, -38.51493924976957572, 18.05360324515410397 ) ) ;
#25021=CARTESIAN_POINT ( 'NONE',  ( -30.26275506840323359, -1.535832457777009877E-13, 41.69427246844629309 ) ) ;
#25022=CARTESIAN_POINT ( 'NONE',  ( -91.56559293963836410, 40.00000000000008527, -22.67402823373177867 ) ) ;
#25023=CARTESIAN_POINT ( 'NONE',  ( -188.2995950289364089, -23.44932284465861727, -43.00522595870986464 ) ) ;
#25024=CARTESIAN_POINT ( 'NONE',  ( -198.0356074513804288, -55.37879056873077133, -2.449293598294708485E-15 ) ) ;
#25025=CARTESIAN_POINT ( 'NONE',  ( 22.90311673803731196, -13.82691048573729908, -46.98314248934561732 ) ) ;
#25026=CARTESIAN_POINT ( 'NONE',  ( -135.8532207217289738, 6.472252184284186249, -6.472252184284142729 ) ) ;
#25027=CARTESIAN_POINT ( 'NONE',  ( 163.1118516004056573, -12.73709011382472234, -2.449293598294708485E-15 ) ) ;
#25028=CARTESIAN_POINT ( 'NONE',  ( 130.8568914410475372, -4.207082182992846420, 4.207082182992822439 ) ) ;
#25029=CARTESIAN_POINT ( 'NONE',  ( -135.8532207217289738, -1.208299557080134822E-13, 9.153146818113572891 ) ) ;
#25030=CARTESIAN_POINT ( 'NONE',  ( -105.3239292022353055, 10.85048923520651520, -18.46172643728406726 ) ) ;
#25031=CARTESIAN_POINT ( 'NONE',  ( 184.8905102610680444, 40.00000000000025580, -19.07866798485515503 ) ) ;
#25032=CARTESIAN_POINT ( 'NONE',  ( 146.6084372240433993, -24.48358557860319706, -24.48358557860330720 ) ) ;
#25034=CARTESIAN_POINT ( 'NONE',  ( -88.39148973765161088, -8.577159256668537068, -19.92926839984431098 ) ) ;
#25035=CARTESIAN_POINT ( 'NONE',  ( -213.1075012329536946, -37.98287015391263566, 37.98287015391218802 ) ) ;
#25037=CARTESIAN_POINT ( 'NONE',  ( 151.7948205124836250, 23.49921654116328540, 23.49921654116366554 ) ) ;
#25038=CARTESIAN_POINT ( 'NONE',  ( -188.5332406156470313, 23.50029615585822640, -43.07394490459756042 ) ) ;
#25040=CARTESIAN_POINT ( 'NONE',  ( -105.3755690713226727, -18.24025645688354302, -2.449293598294708485E-15 ) ) ;
#25043=CARTESIAN_POINT ( 'NONE',  ( -114.6318783467488203, 11.20407312249095533, -18.94416332741571196 ) ) ;
#25046=( BOUNDED_SURFACE ( )  B_SPLINE_SURFACE ( 3, 2, ( 
 ( #15391, #25008, #13395 ),
 ( #17387, #19512, #788 ),
 ( #17004, #25526, #23516 ),
 ( #25141, #5288, #1297 ),
 ( #2917, #6892, #16876 ),
 ( #17134, #14873, #23140 ) ),
 .UNSPECIFIED., .F., .F., .F. ) 
 B_SPLINE_SURFACE_WITH_KNOTS ( ( 4, 2, 4 ),
 ( 3, 3 ),
 ( 0.04143185595419456024, 0.04845767571923142308, 0.05548349548426828592 ),
 ( 0.000000000000000000, 1.000000000000000000 ),
 .UNSPECIFIED. ) 
 GEOMETRIC_REPRESENTATION_ITEM ( )  RATIONAL_B_SPLINE_SURFACE ( (
 ( 1.000000000000000000, 0.9541700779530466470, 1.000000000000000000),
 ( 1.000000000000000000, 0.9520118410151657828, 1.000000000000000000),
 ( 1.000000000000000000, 0.9503153331900817680, 1.000000000000000000),
 ( 1.000000000000000000, 0.9480088290653094774, 1.000000000000000000),
 ( 1.000000000000000000, 0.9474362546590832102, 1.000000000000000000),
 ( 1.000000000000000000, 0.9474350314971536902, 1.000000000000000000) ) ) 
 REPRESENTATION_ITEM ( '' )  SURFACE ( )  );
#25049=DIRECTION ( 'NONE',  ( 0.000000000000000000, 1.000000000000000000, 0.000000000000000000 ) ) ;
#25051=VERTEX_POINT ( 'NONE', #10924 ) ;
#25052=CARTESIAN_POINT ( 'NONE',  ( -86.96347745069644475, -43.67073346367983788, 12.89780903124397149 ) ) ;
#25054=CARTESIAN_POINT ( 'NONE',  ( -114.7465989397623645, 2.774003790519791846, 21.93543632637892671 ) ) ;
#25055=CARTESIAN_POINT ( 'NONE',  ( 4.995406935893294431, -17.50105314357198694, 39.06748935135188816 ) ) ;
#25056=CARTESIAN_POINT ( 'NONE',  ( -105.4000354196369784, 20.24155804474649401, 6.858112701554157198 ) ) ;
#25057=CARTESIAN_POINT ( 'NONE',  ( 200.0000000000000000, 40.00000000000012790, -19.99999999999996092 ) ) ;
#25059=DIRECTION ( 'NONE',  ( -0.2259624730577678986, 0.9741360073262960162, 0.000000000000000000 ) ) ;
#25060=CARTESIAN_POINT ( 'NONE',  ( -100.7734535825088500, -40.00000000000027711, 22.67402823373149801 ) ) ;
#25061=CARTESIAN_POINT ( 'NONE',  ( -91.56559293963836410, 39.99999999999976552, 22.67402823373234000 ) ) ;
#25062=CARTESIAN_POINT ( 'NONE',  ( -87.08360718067700645, 17.46847230663351525, 12.46771266860896255 ) ) ;
#25066=CARTESIAN_POINT ( 'NONE',  ( -188.3065677117174914, 23.45084385698005391, 43.00727648871502140 ) ) ;
#25067=CARTESIAN_POINT ( 'NONE',  ( 170.2234770963711128, -10.92277846919235529, 45.64576402573175073 ) ) ;
#25068=CARTESIAN_POINT ( 'NONE',  ( -190.1935165880708496, -47.62328200654635424, 13.92226094463972963 ) ) ;
#25069=CARTESIAN_POINT ( 'NONE',  ( -198.0356074513804572, 17.40982414986446969, 39.15871834505921356 ) ) ;
#25070=CARTESIAN_POINT ( 'NONE',  ( -82.29192131168281321, -18.26745044309027222, 8.580784324611526515 ) ) ;
#25071=CARTESIAN_POINT ( 'NONE',  ( -56.48582580120559982, 34.75652343174628101, -21.81201906317743067 ) ) ;
#25072=CARTESIAN_POINT ( 'NONE',  ( 200.0000000000000000, 60.00000000000007105, 7.347880794884118356E-15 ) ) ;
#25073=CARTESIAN_POINT ( 'NONE',  ( 151.7948205124835681, 33.23291073765556547, 40.00000000000002132 ) ) ;
#25074=CARTESIAN_POINT ( 'NONE',  ( 19.06497207195980792, 10.03556273973447155, -10.03556273973422286 ) ) ;
#25075=CARTESIAN_POINT ( 'NONE',  ( 192.4448373802101173, -19.99999999996057554, 40.00000000000002132 ) ) ;
#25076=CARTESIAN_POINT ( 'NONE',  ( -86.86493150571116928, 19.77569912839177846, -7.943527260495974573 ) ) ;
#25077=ORIENTED_EDGE ( 'NONE', *, *, #14186, .T. ) ;
#25078=CARTESIAN_POINT ( 'NONE',  ( 200.0000000000000000, -39.99999999999977973, -20.00000000000034817 ) ) ;
#25084=CARTESIAN_POINT ( 'NONE',  ( -100.7734535825088358, 17.32597176626809343, 2.449293598294708485E-15 ) ) ;
#25088=CARTESIAN_POINT ( 'NONE',  ( -105.3178975793522199, -20.76461410733032409, 5.416379678195457181 ) ) ;
#25089=EDGE_CURVE ( 'NONE', #23960, #9969, #21199, .T. ) ;
#25090=B_SPLINE_CURVE_WITH_KNOTS ( 'NONE', 3,
 ( #4689, #6532, #12792, #8936, #20918, #24645, #13185, #19673, #9562, #23672, #21306, #19808 ),
 .UNSPECIFIED., .F., .F.,
 ( 4, 2, 2, 2, 2, 4 ),
 ( 1.457502235237144910E-15, 0.004698945756008141884, 0.007048418634011504626, 0.009397891512014868234, 0.01409683726802163535, 0.01879578302402840420 ),
 .UNSPECIFIED. ) ;
#25091=CARTESIAN_POINT ( 'NONE',  ( 160.7895100360861136, -20.14405787076863064, -20.14405787076872656 ) ) ;
#25092=( BOUNDED_CURVE ( )  B_SPLINE_CURVE ( 3, ( #1938, #16158, #5787, #20028 ),
 .UNSPECIFIED., .F., .F. ) 
 B_SPLINE_CURVE_WITH_KNOTS ( ( 4, 4 ),
 ( 0.004183487405659287901, 0.01388163287021764933 ),
 .UNSPECIFIED. ) 
 CURVE ( )  GEOMETRIC_REPRESENTATION_ITEM ( )  RATIONAL_B_SPLINE_CURVE ( ( 0.6809743333591588010, 0.7608653435686177913, 0.8672072324488981909, 1.000000000000000000 ) ) 
 REPRESENTATION_ITEM ( '' )  );
#25093=CARTESIAN_POINT ( 'NONE',  ( 151.7948205124836250, 1.439163438361279259E-13, -33.23291073765553705 ) ) ;
#25095=EDGE_CURVE ( 'NONE', #12893, #7090, #18253, .T. ) ;
#25097=CARTESIAN_POINT ( 'NONE',  ( -213.1075012329537230, 9.698598906438871126, -66.26714140136179765 ) ) ;
#25098=CARTESIAN_POINT ( 'NONE',  ( -238.4067589809705794, -0.6820004457913585449, -0.6820004457913265705 ) ) ;
#25099=DIRECTION ( 'NONE',  ( 0.000000000000000000, 1.000000000000000000, 0.000000000000000000 ) ) ;
#25100=CARTESIAN_POINT ( 'NONE',  ( 200.0000000000000000, -39.99999999999977973, -20.00000000000034817 ) ) ;
#25102=CARTESIAN_POINT ( 'NONE',  ( -259.2033419157646676, 9.517827891722584255, -0.000000000000000000 ) ) ;
#25103=CARTESIAN_POINT ( 'NONE',  ( -208.1127848780264742, -10.60833733268345469, 67.17687982760682530 ) ) ;
#25106=CARTESIAN_POINT ( 'NONE',  ( -198.0356074513804572, -9.007331120208026888E-14, 15.37879056873070560 ) ) ;
#25108=CARTESIAN_POINT ( 'NONE',  ( 19.06497207195981858, 10.03556273973424062, 66.60410523465820631 ) ) ;
#25109=CARTESIAN_POINT ( 'NONE',  ( 91.82158438592158234, -17.20528682183298486, 40.00000000000002132 ) ) ;
#25110=B_SPLINE_CURVE_WITH_KNOTS ( 'NONE', 3,
 ( #18664, #18936, #23072, #718, #4713, #16670, #22803, #11081, #9083, #8554, #12949, #6687 ),
 .UNSPECIFIED., .F., .F.,
 ( 4, 2, 2, 2, 2, 4 ),
 ( 1.326269557315125156E-15, 0.004680202113614923519, 0.009360404227228521709, 0.01170050528403532124, 0.01404060634084211903, 0.01872080845445575625 ),
 .UNSPECIFIED. ) ;
#25112=CARTESIAN_POINT ( 'NONE',  ( 12.77879914705803444, -44.80239647190084185, 18.55776024549615855 ) ) ;
#25113=CARTESIAN_POINT ( 'NONE',  ( -135.8532207217289738, -9.153146818113595984, -40.00000000000002132 ) ) ;
#25114=CARTESIAN_POINT ( 'NONE',  ( -87.02146317964799493, -10.86006974119950463, 18.50839211081909852 ) ) ;
#25115=CARTESIAN_POINT ( 'NONE',  ( -238.4067589809705794, 0.6820004457912757223, 0.6820004457913219076 ) ) ;
#25116=CARTESIAN_POINT ( 'NONE',  ( -77.90022806219006668, -8.352332316461408723, 20.16431395584796249 ) ) ;
#25117=CARTESIAN_POINT ( 'NONE',  ( -82.24426486890021692, 20.04463774090378791, 2.459032291083046662 ) ) ;
#25118=CARTESIAN_POINT ( 'NONE',  ( -62.62756078652115121, 10.52198127423075213, -25.40230989557676367 ) ) ;
#25120=CARTESIAN_POINT ( 'NONE',  ( -56.48582580120559271, -6.472252184284276844, 6.472252184284108978 ) ) ;
#25122=CARTESIAN_POINT ( 'NONE',  ( -77.55640685876514340, -22.13135000837104727, -2.449293598294710063E-15 ) ) ;
#25123=CARTESIAN_POINT ( 'NONE',  ( -188.8532066752250671, -17.93248812771289380, 43.29285604501835394 ) ) ;
#25124=CARTESIAN_POINT ( 'NONE',  ( -208.1127848780264742, 17.67593391476678377, -38.89260858015718014 ) ) ;
#25125=CARTESIAN_POINT ( 'NONE',  ( -100.7734535825088500, 16.03295912088713848, -16.03295912088698927 ) ) ;
#25126=CARTESIAN_POINT ( 'NONE',  ( 14.38125909742181285, -17.55144818341421598, -39.01709431150935359 ) ) ;
#25127=CARTESIAN_POINT ( 'NONE',  ( 200.0000000000000000, 7.347880794884121511E-14, 0.000000000000000000 ) ) ;
#25128=CARTESIAN_POINT ( 'NONE',  ( -100.7734535825088500, 44.31723036834907958, -12.25131212657445801 ) ) ;
#25129=CARTESIAN_POINT ( 'NONE',  ( -86.96347745069644475, 12.89780903124419353, -12.89780903124389333 ) ) ;
#25130=CARTESIAN_POINT ( 'NONE',  ( 170.2234770963711128, 10.92277846919216522, -10.92277846919186501 ) ) ;
#25131=CARTESIAN_POINT ( 'NONE',  ( -105.3755690713226585, 21.75974354311648185, 40.00000000000002132 ) ) ;
#25132=CARTESIAN_POINT ( 'NONE',  ( 192.4448373802101173, -20.00000000003938538, -40.00000000000002132 ) ) ;
#25133=CARTESIAN_POINT ( 'NONE',  ( 184.8905102610680444, 13.49065550809817715, -43.07788698682574591 ) ) ;
#25135=CARTESIAN_POINT ( 'NONE',  ( 192.4448373802101173, -42.42640687116510634, 14.14213562375845257 ) ) ;
#25137=CARTESIAN_POINT ( 'NONE',  ( -114.4364955367337444, 20.04994829327354822, -8.644468109217221752 ) ) ;
#25139=CARTESIAN_POINT ( 'NONE',  ( -208.1127848780264742, 10.60833733270764867, 67.17687982763166588 ) ) ;
#25140=AXIS2_PLACEMENT_3D ( 'NONE', #2047, #8277, #26133 ) ;
#25141=CARTESIAN_POINT ( 'NONE',  ( -77.58456235491127018, -17.49514130593958328, -13.58502979129033328 ) ) ;
#25142=CARTESIAN_POINT ( 'NONE',  ( -162.0762913951020607, -1.198031840455708430, 57.76657433537920383 ) ) ;
#25143=CARTESIAN_POINT ( 'NONE',  ( -5.859158571312020669, -46.35984297724550629, -13.69949429424737275 ) ) ;
#25146=CARTESIAN_POINT ( 'NONE',  ( -114.7544835083390780, -13.58506800096324163, -17.49509852148034383 ) ) ;
#25148=CARTESIAN_POINT ( 'NONE',  ( -114.7827960788993096, -22.13220202243095969, 0.6714470530277172333 ) ) ;
#25149=CARTESIAN_POINT ( 'NONE',  ( -135.8532207217289738, 30.84685318188643066, 2.449293598294708485E-15 ) ) ;
#25152=CARTESIAN_POINT ( 'NONE',  ( -280.0000000000000000, 14.14213562373078581, 14.14213562373108424 ) ) ;
#25153=CARTESIAN_POINT ( 'NONE',  ( 19.06497207195982924, -40.00000000000021316, 54.19242893257830218 ) ) ;
#25154=CARTESIAN_POINT ( 'NONE',  ( 4.995406935893292655, 39.99999999999982947, 55.24977328856478209 ) ) ;
#25156=CARTESIAN_POINT ( 'NONE',  ( -91.56559293963834989, -17.32597176626812185, -40.00000000000002132 ) ) ;
#25157=CARTESIAN_POINT ( 'NONE',  ( 22.82148508083543348, -17.87803012130470748, -43.16138278736961098 ) ) ;
#25158=CARTESIAN_POINT ( 'NONE',  ( 130.8568914410475372, 24.07718906447243867, -24.07718906447216156 ) ) ;
#25159=CARTESIAN_POINT ( 'NONE',  ( 192.4448373802101173, -19.99999999996056843, -40.00000000000002132 ) ) ;
#25160=CARTESIAN_POINT ( 'NONE',  ( 57.59792236341147031, 1.722363176415065089, -1.722363176415036445 ) ) ;
#25161=CARTESIAN_POINT ( 'NONE',  ( 91.82158438592158234, -1.633484621919921769E-13, 17.20528682183300262 ) ) ;
#25162=CARTESIAN_POINT ( 'NONE',  ( -175.9234121931127390, -21.03678983223290189, 39.35887396220598333 ) ) ;
#25163=CARTESIAN_POINT ( 'NONE',  ( -56.48582580120557850, -39.99999999999970868, -30.84685318188687120 ) ) ;
#25164=CARTESIAN_POINT ( 'NONE',  ( -91.56559293963834989, -16.03295912088706388, -16.03295912088710651 ) ) ;
#25165=CARTESIAN_POINT ( 'NONE',  ( -53.37769371738423985, -27.95780717557995843, 13.65853730965386248 ) ) ;
#25167=CARTESIAN_POINT ( 'NONE',  ( 163.1118516004056573, -9.006482792069636645, 9.006482792069567367 ) ) ;
#25169=CARTESIAN_POINT ( 'NONE',  ( -87.01701082927731079, 18.46482525711258660, -10.86389608310530619 ) ) ;
#25170=CARTESIAN_POINT ( 'NONE',  ( -6.342283169554576716, 46.19215417243025712, -13.66521761903544174 ) ) ;
#25172=CARTESIAN_POINT ( 'NONE',  ( -162.0762913951020607, -41.69427287692683848, 40.00000000000002132 ) ) ;
#25174=CARTESIAN_POINT ( 'NONE',  ( -188.6013476421509552, 47.09841799633670689, -13.84412643133189391 ) ) ;
#25177=AXIS2_PLACEMENT_3D ( 'NONE', #21799, #3572, #7682 ) ;
#25179=CARTESIAN_POINT ( 'NONE',  ( -99.31267923331542136, 8.544756979562974308, -20.62886818714414616 ) ) ;
#25180=ORIENTED_EDGE ( 'NONE', *, *, #11242, .F. ) ;
#25183=CARTESIAN_POINT ( 'NONE',  ( 91.82158438592158234, -12.16597498397761967, -12.16597498397768007 ) ) ;
#25185=CARTESIAN_POINT ( 'NONE',  ( -114.4940140762809619, -7.440456728164089206, 20.58897208711081106 ) ) ;
#25186=CARTESIAN_POINT ( 'NONE',  ( -238.4067589809705794, 0.6820004457340470561, 57.25054294065803617 ) ) ;
#25188=CARTESIAN_POINT ( 'NONE',  ( -259.2033419157646676, 40.00000000000000711, -9.517827891722491884 ) ) ;
#25191=EDGE_CURVE ( 'NONE', #25529, #12893, #3596, .T. ) ;
#25192=CARTESIAN_POINT ( 'NONE',  ( 192.4448373802101173, -40.00000000000019185, 20.00000000003900524 ) ) ;
#25193=CARTESIAN_POINT ( 'NONE',  ( 57.59792236341147031, 40.00000000000042633, -37.56421063658144277 ) ) ;
#25194=CARTESIAN_POINT ( 'NONE',  ( -77.55640685875366103, 16.16066924852440678, 15.13778608694647332 ) ) ;
#25198=CARTESIAN_POINT ( 'NONE',  ( -199.9999999999999716, -44.86878812508714276, 24.82633483071253622 ) ) ;
#25199=CARTESIAN_POINT ( 'NONE',  ( -280.0000000000000568, -14.14213562373137556, 42.42640687119276066 ) ) ;
#25201=CARTESIAN_POINT ( 'NONE',  ( -105.3755690713226727, 15.38646221621793231, -15.38646221621779020 ) ) ;
#25202=CARTESIAN_POINT ( 'NONE',  ( -87.13368444202060914, -14.72469439729719554, 15.67192210925610496 ) ) ;
#25203=CARTESIAN_POINT ( 'NONE',  ( -30.26275506840323359, -1.198031551615522439, -57.76657404653986561 ) ) ;
#25207=CARTESIAN_POINT ( 'NONE',  ( -30.26275506840325136, 57.76657404653985139, -1.198031551615314161 ) ) ;
#25208=CARTESIAN_POINT ( 'NONE',  ( -56.48582580120559271, 9.153146818113576444, -0.000000000000000000 ) ) ;
#25211=CARTESIAN_POINT ( 'NONE',  ( -86.96347745069643054, -39.99999999999985079, -18.24025645688394448 ) ) ;
#25213=CARTESIAN_POINT ( 'NONE',  ( 170.0000000000000853, -9.369682556672300322, 22.62041470344878746 ) ) ;
#25216=ORIENTED_EDGE ( 'NONE', *, *, #379, .T. ) ;
#25217=CARTESIAN_POINT ( 'NONE',  ( -56.48582580120559271, 30.84685318188643066, 2.449293598294708485E-15 ) ) ;
#25218=CARTESIAN_POINT ( 'NONE',  ( -114.4364955367323660, -8.064892380834915997, 20.29001642039123610 ) ) ;
#25219=CARTESIAN_POINT ( 'NONE',  ( 199.9999999999999432, 1.065690307512836407E-13, -20.00000000000010303 ) ) ;
#25222=CARTESIAN_POINT ( 'NONE',  ( 57.59792236341147031, -1.722363176414363206, -54.84617931850881689 ) ) ;
#25223=CARTESIAN_POINT ( 'NONE',  ( 19.06497207195981147, -10.03556273973425483, -10.03556273973443247 ) ) ;
#25225=CARTESIAN_POINT ( 'NONE',  ( 130.8568914410475372, 8.880724697947696879E-14, -5.949712681206690945 ) ) ;
#25226=CARTESIAN_POINT ( 'NONE',  ( 136.1360204305621266, 24.77266263493104148, 24.77266263493145004 ) ) ;
#25227=CARTESIAN_POINT ( 'NONE',  ( -56.48582580120559271, 9.153146818113576444, -0.000000000000000000 ) ) ;
#25228=CARTESIAN_POINT ( 'NONE',  ( 91.82158438592159655, -44.40256751092324095, -12.16597498400075139 ) ) ;
#25230=EDGE_CURVE ( 'NONE', #11453, #12520, #13448, .T. ) ;
#25232=CARTESIAN_POINT ( 'NONE',  ( -238.4067589809705794, -4.716212492215116094E-14, 0.9644942799825824142 ) ) ;
#25233=CARTESIAN_POINT ( 'NONE',  ( 200.0000000000000000, -20.00000000000006750, -40.00000000000002132 ) ) ;
#25234=CARTESIAN_POINT ( 'NONE',  ( -280.0000000000000568, -14.14213562373108601, 42.42640687119285303 ) ) ;
#25235=CARTESIAN_POINT ( 'NONE',  ( 91.82158438592158234, 22.79471317813471742, 40.00000000000002132 ) ) ;
#25237=CARTESIAN_POINT ( 'NONE',  ( 11.38508063387934754, -44.88728980639579902, 24.83994849158430540 ) ) ;
#25238=CARTESIAN_POINT ( 'NONE',  ( 91.82158438592158234, -17.20528682183298486, -40.00000000000002132 ) ) ;
#25240=( BOUNDED_SURFACE ( )  B_SPLINE_SURFACE ( 3, 2, ( 
 ( #21657, #19526, #17525 ),
 ( #23407, #19275, #13286 ),
 ( #15277, #5299, #13409 ),
 ( #3307, #3430, #25663 ),
 ( #11531, #9677, #21787 ),
 ( #1573, #3559, #25927 ) ),
 .UNSPECIFIED., .F., .F., .F. ) 
 B_SPLINE_SURFACE_WITH_KNOTS ( ( 4, 2, 4 ),
 ( 3, 3 ),
 ( 0.04143178499028438849, 0.04845752250266459338, 0.05548326001504480520 ),
 ( 0.000000000000000000, 1.000000000000000000 ),
 .UNSPECIFIED. ) 
 GEOMETRIC_REPRESENTATION_ITEM ( )  RATIONAL_B_SPLINE_SURFACE ( (
 ( 1.000000000000000000, 0.9541700779530452037, 1.000000000000000000),
 ( 1.000000000000000000, 0.9520119333866750022, 1.000000000000000000),
 ( 1.000000000000000000, 0.9503150296563032118, 1.000000000000000000),
 ( 1.000000000000000000, 0.9480088385138416562, 1.000000000000000000),
 ( 1.000000000000000000, 0.9474362539901676206, 1.000000000000000000),
 ( 1.000000000000000000, 0.9474350314971542453, 1.000000000000000000) ) ) 
 REPRESENTATION_ITEM ( '' )  SURFACE ( )  );
#25241=CARTESIAN_POINT ( 'NONE',  ( 130.8568914410475372, 4.207082182992862407, 4.207082182992856190 ) ) ;
#25242=CARTESIAN_POINT ( 'NONE',  ( 91.82158438592159655, -39.99999999999994316, -17.20528682183314118 ) ) ;
#25243=CARTESIAN_POINT ( 'NONE',  ( -77.90255099906774205, 20.29001641120652621, -8.064892378658626626 ) ) ;
#25244=CARTESIAN_POINT ( 'NONE',  ( 12.01676479903291650, -14.17570730777163668, -49.30523874212537550 ) ) ;
#25246=CARTESIAN_POINT ( 'NONE',  ( -198.0356074513804572, 67.44298959250878056, -10.87444709758402261 ) ) ;
#25247=FACE_OUTER_BOUND ( 'NONE', #10564, .T. ) ;
#25249=CARTESIAN_POINT ( 'NONE',  ( -259.2033419157646676, 6.730120644403521979, -6.730120644403498886 ) ) ;
#25250=CARTESIAN_POINT ( 'NONE',  ( 163.1118516004056573, 19.27778845538753316, 19.27778845538783870 ) ) ;
#25252=CARTESIAN_POINT ( 'NONE',  ( 184.8905102610680444, 43.07788698682572459, 13.49065550809829439 ) ) ;
#25254=CARTESIAN_POINT ( 'NONE',  ( -114.4364955367328349, 20.29001642038852538, -8.064892380842216824 ) ) ;
#25255=CARTESIAN_POINT ( 'NONE',  ( -200.4318156386386534, 24.83634777281940487, -44.88237417767393111 ) ) ;
#25256=CARTESIAN_POINT ( 'NONE',  ( -259.2033419157646676, 49.83842185052017015, 6.730120644404137487 ) ) ;
#25257=CARTESIAN_POINT ( 'NONE',  ( -91.56559293963834989, -16.03295912088659492, -40.53558337403696044 ) ) ;
#25258=CARTESIAN_POINT ( 'NONE',  ( -56.48582580120559982, -9.153146818113595984, -40.00000000000002132 ) ) ;
#25259=CARTESIAN_POINT ( 'NONE',  ( -86.96347745069644475, 12.89780903124410472, -43.67073346367977393 ) ) ;
#25260=ADVANCED_FACE ( 'NONE', ( #23860 ), #22746, .T. ) ;
#25261=CARTESIAN_POINT ( 'NONE',  ( -280.0000000000000000, 1.839446121267387017E-14, -20.00000000000001421 ) ) ;
#25262=CARTESIAN_POINT ( 'NONE',  ( -208.1127848780264742, -67.17687982760682530, -10.60833733268364298 ) ) ;
#25264=CARTESIAN_POINT ( 'NONE',  ( -83.21262154144228873, -33.12752917117752105, 13.72187187063023650 ) ) ;
#25266=CARTESIAN_POINT ( 'NONE',  ( -100.7734535825088358, 12.25131212657480440, 12.25131212657487012 ) ) ;
#25267=CARTESIAN_POINT ( 'NONE',  ( -16.41532015104117193, 42.70629200743962173, -12.95569205199923957 ) ) ;
#25268=CARTESIAN_POINT ( 'NONE',  ( -56.48582580120559982, 34.75652343174597547, 21.81201906317791384 ) ) ;
#25269=CARTESIAN_POINT ( 'NONE',  ( -4.081455915266338330, -43.13234798823421556, -17.86600351372032591 ) ) ;
#25271=EDGE_CURVE ( 'NONE', #25810, #20782, #13130, .T. ) ;
#25272=ORIENTED_EDGE ( 'NONE', *, *, #17665, .T. ) ;
#25273=CARTESIAN_POINT ( 'NONE',  ( -187.7698581930904140, -42.84913646251419550, 23.34605429454595082 ) ) ;
#25275=CARTESIAN_POINT ( 'NONE',  ( 90.71511022971527893, -8.335579104983011689, 21.46756116496406364 ) ) ;
#25276=CARTESIAN_POINT ( 'NONE',  ( -213.1075012329537230, 13.71589010951907817, -40.00000000000002132 ) ) ;
#25277=CARTESIAN_POINT ( 'NONE',  ( 67.90397382968500040, 14.12691053360184412, -28.69135535065072773 ) ) ;
#25279=CARTESIAN_POINT ( 'NONE',  ( -105.3755690713226585, -12.89780903124444578, 43.67073346367968156 ) ) ;
#25280=CARTESIAN_POINT ( 'NONE',  ( 4.995406935893298872, -1.944352046434030652E-13, 55.24977328854835434 ) ) ;
#25282=CARTESIAN_POINT ( 'NONE',  ( -199.9999999999999147, -19.98641303047005024, -45.65206365911544140 ) ) ;
#25283=CARTESIAN_POINT ( 'NONE',  ( -30.26275506840323004, -41.69427246844627888, -40.00000000000002132 ) ) ;
#25284=CARTESIAN_POINT ( 'NONE',  ( 21.60666276257293461, -18.00814241471057642, -43.47550165074667916 ) ) ;
#25286=CARTESIAN_POINT ( 'NONE',  ( -213.1075012329537230, -13.71589010951915810, 40.00000000000002132 ) ) ;
#25287=CARTESIAN_POINT ( 'NONE',  ( 146.6084372240433709, 52.76785682606519146, 3.800685668858932775 ) ) ;
#25288=CARTESIAN_POINT ( 'NONE',  ( -56.48582580120559982, 40.00000000000034106, -30.84685318188602210 ) ) ;
#25289=CARTESIAN_POINT ( 'NONE',  ( -110.0822598093739657, 11.09289860106540893, -16.86905266168659523 ) ) ;
#25290=CARTESIAN_POINT ( 'NONE',  ( 91.82158438592159655, -40.00000000000017764, 17.20528682183258340 ) ) ;
#25294=CARTESIAN_POINT ( 'NONE',  ( 136.1360204305621266, 53.05693388239316022, 3.511608612530967566 ) ) ;
#25297=CARTESIAN_POINT ( 'NONE',  ( 6.615221834188973027, 49.23097633541777185, -14.16446777330068763 ) ) ;
#25298=CARTESIAN_POINT ( 'NONE',  ( 158.3379117892987438, 26.51167085133959134, -10.98149362779631666 ) ) ;
#25299=CARTESIAN_POINT ( 'NONE',  ( 184.8905102610680444, -19.07866798485555293, -2.449293598294708485E-15 ) ) ;
#25300=CARTESIAN_POINT ( 'NONE',  ( -188.3610564113212149, 47.01267209787937418, -13.83140491817310824 ) ) ;
#25304=CARTESIAN_POINT ( 'NONE',  ( -192.9588430854689989, -10.23066800230756890, 10.23066800230742501 ) ) ;
#25305=CARTESIAN_POINT ( 'NONE',  ( 146.5090579137181805, 12.40347562390462066, -29.94463907179407514 ) ) ;
#25306=CARTESIAN_POINT ( 'NONE',  ( 130.8568914410475372, 1.429239637432775288E-13, -34.05028731879788495 ) ) ;
#25307=ORIENTED_EDGE ( 'NONE', *, *, #21220, .T. ) ;
#25311=CARTESIAN_POINT ( 'NONE',  ( -83.21262154144248768, 33.12752917118412199, -13.72187187061503444 ) ) ;
#25312=CARTESIAN_POINT ( 'NONE',  ( 57.59792236341147031, -30.00663442387700641, 26.56190807104681895 ) ) ;
#25313=CARTESIAN_POINT ( 'NONE',  ( 170.2234770963711128, -17.36149277826985937, -17.36149277826995174 ) ) ;
#25314=CARTESIAN_POINT ( 'NONE',  ( 130.8568914410475088, 40.00000000000015632, -34.05028731879774284 ) ) ;
#25315=CYLINDRICAL_SURFACE ( 'NONE', #20256, 30.00000000000003908 ) ;
#25317=CARTESIAN_POINT ( 'NONE',  ( -192.9588430854690273, -39.99999999999948841, -54.46834944098263520 ) ) ;
#25319=CARTESIAN_POINT ( 'NONE',  ( 4.995406935893298872, 5.820775922023080204E-13, -55.24977328854835434 ) ) ;
#25320=CARTESIAN_POINT ( 'NONE',  ( -77.59736708337840128, 17.53068837882001674, 13.45304834675272332 ) ) ;
#25321=CARTESIAN_POINT ( 'NONE',  ( -213.1075012329537230, -66.26714140138676612, 9.698598906462487790 ) ) ;
#25322=DIRECTION ( 'NONE',  ( 0.000000000000000000, -0.9166903767334039221, -0.3995982397413309073 ) ) ;
#25323=CARTESIAN_POINT ( 'NONE',  ( -200.4317933031571499, 24.83634732651995236, 44.88237357214655532 ) ) ;
#25325=CARTESIAN_POINT ( 'NONE',  ( -109.1264249741459480, -33.12752917269222763, 13.72187187123999053 ) ) ;
#25326=CARTESIAN_POINT ( 'NONE',  ( 91.82158438592158234, 12.16597498397773869, -12.16597498397759303 ) ) ;
#25327=CARTESIAN_POINT ( 'NONE',  ( -82.23866184892956710, -13.36787606754601399, 15.15017645652793199 ) ) ;
#25330=CARTESIAN_POINT ( 'NONE',  ( -259.2033419157646676, -21.55415060305872998, 35.01439189186525880 ) ) ;
#25332=CARTESIAN_POINT ( 'NONE',  ( -87.13361725327075646, 15.19799821270843765, 15.19799821270837015 ) ) ;
#25334=CARTESIAN_POINT ( 'NONE',  ( 199.9999999999999432, -14.14213562373115884, 14.14213562373085153 ) ) ;
#25339=CARTESIAN_POINT ( 'NONE',  ( -135.8532207217289738, 3.005970985514575011E-13, -30.84685318188645553 ) ) ;
#25341=CARTESIAN_POINT ( 'NONE',  ( -199.9999999999999432, -4.865628651907146107, -55.16984130227028515 ) ) ;
#25343=ORIENTED_EDGE ( 'NONE', *, *, #1264, .T. ) ;
#25344=ORIENTED_EDGE ( 'NONE', *, *, #12400, .T. ) ;
#25345=CARTESIAN_POINT ( 'NONE',  ( -213.1075012329537230, 53.71589010950162191, -40.00000000000002132 ) ) ;
#25346=EDGE_CURVE ( 'NONE', #24441, #17844, #16571, .T. ) ;
#25347=CARTESIAN_POINT ( 'NONE',  ( -103.9663809734175999, -20.15238534381313684, -8.026122150562576607 ) ) ;
#25348=CARTESIAN_POINT ( 'NONE',  ( -77.70077460412316839, -11.21025402036352325, 18.98542998413487837 ) ) ;
#25349=CARTESIAN_POINT ( 'NONE',  ( 192.4448373802100889, 1.051811698935164031E-13, -20.00000000003942091 ) ) ;
#25354=CARTESIAN_POINT ( 'NONE',  ( -40.07203023092074545, -16.33025453607757882, -32.10811084135991678 ) ) ;
#25355=CARTESIAN_POINT ( 'NONE',  ( -135.8532207217289738, 34.75652343174625258, -21.81201906317744132 ) ) ;
#25356=CARTESIAN_POINT ( 'NONE',  ( -99.31680025536471135, 20.62455315994730398, 8.542969636735133321 ) ) ;
#25357=CARTESIAN_POINT ( 'NONE',  ( -259.2033419157646676, -39.99999999999975131, -30.48217210827782608 ) ) ;
#25358=CARTESIAN_POINT ( 'NONE',  ( 163.1118516004056573, -9.006482792074626431, 47.56205970284951690 ) ) ;
#25359=CARTESIAN_POINT ( 'NONE',  ( -198.0356074513804572, -15.37879056873074290, -40.00000000000002132 ) ) ;
#25361=CARTESIAN_POINT ( 'NONE',  ( 14.38125909742181996, -10.73282306403606157, 67.30136555895948902 ) ) ;
#25362=CARTESIAN_POINT ( 'NONE',  ( 130.8568914410475088, 34.05028731879790627, -40.00000000000002132 ) ) ;
#25364=CARTESIAN_POINT ( 'NONE',  ( 184.8905102610680444, 39.99999999999999289, 19.07866798485573057 ) ) ;
#25366=CARTESIAN_POINT ( 'NONE',  ( 136.1360204305621551, -35.03383547441293899, -40.00000000000002132 ) ) ;
#25367=CARTESIAN_POINT ( 'NONE',  ( 163.1118516004056573, -47.56205970284957374, 9.006482792074162802 ) ) ;
#25368=CARTESIAN_POINT ( 'NONE',  ( -238.4067589809705794, 40.96449428006337001, -40.00000000000002132 ) ) ;
#25369=VERTEX_POINT ( 'NONE', #1111 ) ;
#25371=CARTESIAN_POINT ( 'NONE',  ( -1.087763065864006062, -47.95583523903733436, 13.97201973055748603 ) ) ;
#25372=CARTESIAN_POINT ( 'NONE',  ( 192.4448373802100889, 19.99999999996064304, 2.449293598294708485E-15 ) ) ;
#25375=CARTESIAN_POINT ( 'NONE',  ( 0.2972598230770011618, 10.13633138497462305, 66.70487387989858519 ) ) ;
#25376=CARTESIAN_POINT ( 'NONE',  ( -238.4067589809705794, -40.00000000000007105, 0.9644942799824426372 ) ) ;
#25377=CARTESIAN_POINT ( 'NONE',  ( -87.05902966484931937, 21.00921308708589308, -4.297868118821011940 ) ) ;
#25378=CARTESIAN_POINT ( 'NONE',  ( -5.859158571311539276, 13.69949429424878851, -46.35984297724471048 ) ) ;
#25381=CARTESIAN_POINT ( 'NONE',  ( -87.10570614283763291, 2.723277571087649118, -21.31140251566250399 ) ) ;
#25382=CARTESIAN_POINT ( 'NONE',  ( 151.7948205124836250, -23.49921654116371883, 23.49921654116317526 ) ) ;
#25383=CARTESIAN_POINT ( 'NONE',  ( -162.0762913951021176, 27.08623940707639477, -29.48230308784743059 ) ) ;
#25384=CARTESIAN_POINT ( 'NONE',  ( -91.56559293963836410, 44.31723036834890905, 12.25131212657507795 ) ) ;
#25386=CARTESIAN_POINT ( 'NONE',  ( -135.8532207217289738, 6.472252184284096543, 6.472252184284234211 ) ) ;
#25387=CARTESIAN_POINT ( 'NONE',  ( -100.7734535825088500, 16.03295912088691821, 16.03295912088721309 ) ) ;
#25388=CARTESIAN_POINT ( 'NONE',  ( -30.26275506840324070, -27.08623969584554558, -29.48230279907826912 ) ) ;
#25389=CARTESIAN_POINT ( 'NONE',  ( -86.96347745069644475, 41.18208027870576871, 15.38646221621837107 ) ) ;
#25390=CARTESIAN_POINT ( 'NONE',  ( 151.7948205124836534, 6.767089262349062828, -40.00000000000002132 ) ) ;
#25391=CARTESIAN_POINT ( 'NONE',  ( -30.26275506840324070, 1.198031551616013601, 1.198031551616023371 ) ) ;
#25393=CARTESIAN_POINT ( 'NONE',  ( -135.8532207217289738, 7.002209520526292428E-15, -9.153146818113572891 ) ) ;
#25394=CARTESIAN_POINT ( 'NONE',  ( 136.1360204305621551, -31.79587985999279454, 24.77266263493094911 ) ) ;
#25395=CARTESIAN_POINT ( 'NONE',  ( -129.2920181227953549, 25.26067667711114950, -10.46331487475240074 ) ) ;
#25396=EDGE_LOOP ( 'NONE', ( #23548, #17335, #5572, #3846, #19178, #12553 ) ) ;
#25397=CARTESIAN_POINT ( 'NONE',  ( 192.4448373802100889, 14.14213562370310662, 14.14213562370312438 ) ) ;
#25398=CARTESIAN_POINT ( 'NONE',  ( -53.37769371643639715, 29.42719939405414920, -10.11111068829008275 ) ) ;
#25399=CARTESIAN_POINT ( 'NONE',  ( 23.42154907652747298, 23.32998349128558147, 42.84253412640366321 ) ) ;
#25400=CARTESIAN_POINT ( 'NONE',  ( -70.30307074924525068, -23.14841682968063452, -8.711708293734362840 ) ) ;
#25401=ORIENTED_EDGE ( 'NONE', *, *, #9331, .T. ) ;
#25402=CARTESIAN_POINT ( 'NONE',  ( -121.8425418806976381, -22.74408238789939674, 9.420907390773301415 ) ) ;
#25404=CARTESIAN_POINT ( 'NONE',  ( 23.35928221536216398, -13.80178577956153063, 46.81377789283308033 ) ) ;
#25408=CARTESIAN_POINT ( 'NONE',  ( -162.0762913951021176, -29.48230308784793152, 27.08623940707591515 ) ) ;
#25409=CARTESIAN_POINT ( 'NONE',  ( -105.3755690713226585, 40.00000000000007816, -21.75974354311636461 ) ) ;
#25410=CARTESIAN_POINT ( 'NONE',  ( -162.0762913951020892, -3.568845385355699554E-14, 1.694272876828323948 ) ) ;
#25412=CARTESIAN_POINT ( 'NONE',  ( -162.0762913951020607, -41.69427287682838568, -2.449293598294708485E-15 ) ) ;
#25413=CARTESIAN_POINT ( 'NONE',  ( 20.69615274309022723, -13.93598092274699773, -47.71500688528268341 ) ) ;
#25415=EDGE_CURVE ( 'NONE', #10231, #22478, #10925, .T. ) ;
#25416=CARTESIAN_POINT ( 'NONE',  ( -259.2033419157646676, 9.517827891722584255, -0.000000000000000000 ) ) ;
#25418=CARTESIAN_POINT ( 'NONE',  ( 163.1118516004056573, 47.56205970284957374, 9.006482792074494981 ) ) ;
#25419=CARTESIAN_POINT ( 'NONE',  ( 14.38125909742180930, 40.00000000000060396, -55.17850393974224232 ) ) ;
#25420=CARTESIAN_POINT ( 'NONE',  ( -105.4293522940765229, 9.002736003387274977, -19.36070119847539672 ) ) ;
#25421=CARTESIAN_POINT ( 'NONE',  ( 19.06497207195981858, -39.99999999999987210, -14.19242893257882621 ) ) ;
#25422=CARTESIAN_POINT ( 'NONE',  ( 118.9119131903919993, -25.80655941808602094, -10.68942690915843841 ) ) ;
#25424=CARTESIAN_POINT ( 'NONE',  ( -208.1127848780264742, -10.60833733268345469, 67.17687982760682530 ) ) ;
#25427=CARTESIAN_POINT ( 'NONE',  ( 12.96694272564693406, 49.19577900140143356, -14.15914421027473047 ) ) ;
#25428=CARTESIAN_POINT ( 'NONE',  ( 151.7948205124835681, 33.23291073765556547, 40.00000000000002132 ) ) ;
#25430=CARTESIAN_POINT ( 'NONE',  ( -189.1815713358188304, 43.37724571962049680, -17.96744347545783427 ) ) ;
#25433=ORIENTED_EDGE ( 'NONE', *, *, #13609, .F. ) ;
#25434=CARTESIAN_POINT ( 'NONE',  ( 19.06497207195981147, -10.03556273973439517, 10.03556273973429214 ) ) ;
#25436=CARTESIAN_POINT ( 'NONE',  ( -88.39148973765155404, 8.027153355909614874, -20.15708830332384949 ) ) ;
#25440=CARTESIAN_POINT ( 'NONE',  ( -280.0000000000000568, -14.14213562373108601, 42.42640687119285303 ) ) ;
#25441=CARTESIAN_POINT ( 'NONE',  ( 136.1360204305621266, 1.473277640373554421E-13, -35.03383547441296741 ) ) ;
#25443=DIRECTION ( 'NONE',  ( 1.000000000000000000, 1.836970198721030181E-16, -0.000000000000000000 ) ) ;
#25445=CARTESIAN_POINT ( 'NONE',  ( 192.4448373802100889, 2.472897170449861688E-13, -19.99999999996060751 ) ) ;
#25446=CARTESIAN_POINT ( 'NONE',  ( -105.3755690713226585, 40.00000000000019185, -18.24025645688310249 ) ) ;
#25447=CARTESIAN_POINT ( 'NONE',  ( -105.3846709045749890, -19.12138504414901519, 9.637707283831149496 ) ) ;
#25448=CARTESIAN_POINT ( 'NONE',  ( -192.9588430854690273, -38.51493924976932703, -18.05360324515463688 ) ) ;
#25449=FACE_OUTER_BOUND ( 'NONE', #10635, .T. ) ;
#25451=CARTESIAN_POINT ( 'NONE',  ( -163.5815475691942140, 35.61501186087246396, -18.59457173339175284 ) ) ;
#25453=AXIS2_PLACEMENT_3D ( 'NONE', #15886, #24014, #7515 ) ;
#25454=CARTESIAN_POINT ( 'NONE',  ( -77.55625318716889183, 15.17516088037486277, -16.12447834766239296 ) ) ;
#25456=CARTESIAN_POINT ( 'NONE',  ( -87.02115643449447191, -10.85297647556013345, 18.51269039639111824 ) ) ;
#25457=CARTESIAN_POINT ( 'NONE',  ( -100.7734535825088358, 12.25131212657480440, 12.25131212657487012 ) ) ;
#25458=CARTESIAN_POINT ( 'NONE',  ( 19.06497207195982924, -66.60410523465809263, -10.03556273973493163 ) ) ;
#25459=CARTESIAN_POINT ( 'NONE',  ( -114.4364955367313428, -8.644468109216784768, -20.04994829327278438 ) ) ;
#25462=CARTESIAN_POINT ( 'NONE',  ( -238.4067589809705794, 0.6820004458491113475, -57.25054294077229144 ) ) ;
#25463=CARTESIAN_POINT ( 'NONE',  ( 170.0000000000428315, 17.64300463311351308, -17.64300463311329992 ) ) ;
#25465=VERTEX_POINT ( 'NONE', #17453 ) ;
#25466=CARTESIAN_POINT ( 'NONE',  ( 192.4448373802101173, -40.00000000000019185, 20.00000000003900524 ) ) ;
#25467=CARTESIAN_POINT ( 'NONE',  ( -1.815588850254800546, -23.89016120430182966, 43.60036197523994161 ) ) ;
#25468=CARTESIAN_POINT ( 'NONE',  ( 1.564253033640336188, -44.28527310957331053, 24.39614062124470450 ) ) ;
#25471=CARTESIAN_POINT ( 'NONE',  ( -197.6433718613163251, -44.74793361790577961, -18.53520099270188837 ) ) ;
#25472=CARTESIAN_POINT ( 'NONE',  ( 91.82158438592156813, 40.00000000000009948, -17.20528682183286051 ) ) ;
#25473=CARTESIAN_POINT ( 'NONE',  ( -99.31364972217929221, -20.48028939131244996, -8.933506367407366255 ) ) ;
#25475=( BOUNDED_SURFACE ( )  B_SPLINE_SURFACE ( 3, 2, ( 
 ( #23434, #7315, #5210 ),
 ( #11434, #13314, #21434 ),
 ( #3207, #10107, #26091 ),
 ( #7827, #16223, #10239 ),
 ( #11967, #24485, #18208 ),
 ( #22489, #18479, #24214 ),
 ( #12357, #26232, #4269 ),
 ( #3864, #22091, #15946 ),
 ( #14224, #6369, #9581 ),
 ( #17945, #130, #22362 ),
 ( #24075, #20091, #12099 ),
 ( #14488, #8102, #9973 ),
 ( #20223, #6247, #11830 ),
 ( #14095, #3727, #18080 ),
 ( #20487, #1870, #7966 ),
 ( #12231, #2131, #260 ),
 ( #16085, #8234, #24352 ),
 ( #6116, #4139, #4000 ),
 ( #5986, #2261, #20356 ),
 ( #22224, #18350, #9841 ),
 ( #1999, #13957, #16352 ),
 ( #14360, #10368, #8368 ),
 ( #16491, #24616, #19948 ),
 ( #1732, #5851, #10502 ),
 ( #399, #20615, #6504 ),
 ( #12490, #24750, #2391 ),
 ( #18615, #8503, #22621 ),
 ( #4396, #16616, #9611 ),
 ( #23841, #25720, #3362 ),
 ( #17716, #7602, #9746 ),
 ( #17338, #7733, #1505 ),
 ( #19717, #25471, #7473 ),
 ( #25601, #7347, #15845 ),
 ( #15587, #15459, #11344 ) ),
 .UNSPECIFIED., .F., .F., .F. ) 
 B_SPLINE_SURFACE_WITH_KNOTS ( ( 4, 2, 2, 2, 2, 2, 2, 2, 2, 2, 2, 2, 2, 2, 2, 2, 4 ),
 ( 3, 3 ),
 ( 0.005135431517081588682, 0.02907016617530113270, 0.05300490083352067672, 0.07693963549174021033, 0.08292331915629509720, 0.08441924007243381545, 0.08446598760106314996, 0.08448936136537782415, 0.08451273512969248447, 0.08460623018695115349, 0.08479322030146849154, 0.08516720053050318151, 0.08591516098857254757, 0.08890700282084998407, 0.09189884465312742057, 0.09489068648540487094, 0.1008743701499597578 ),
 ( 0.000000000000000000, 1.000000000000000000 ),
 .UNSPECIFIED. ) 
 GEOMETRIC_REPRESENTATION_ITEM ( )  RATIONAL_B_SPLINE_SURFACE ( (
 ( 1.000000000000000000, 0.9997813423552077694, 1.000000000000000000),
 ( 1.000000000000000000, 0.9991063894446133853, 1.000000000000000000),
 ( 1.000000000000000000, 0.9968824679666075106, 1.000000000000000000),
 ( 1.000000000000000000, 0.9891556708435274015, 1.000000000000000000),
 ( 1.000000000000000000, 0.9836552227702378692, 1.000000000000000000),
 ( 1.000000000000000000, 0.9690804699600285010, 1.000000000000000000),
 ( 1.000000000000000000, 0.9600093828087571390, 1.000000000000000000),
 ( 1.000000000000000000, 0.9461484455229860480, 1.000000000000000000),
 ( 1.000000000000000000, 0.9432496483672391241, 1.000000000000000000),
 ( 1.000000000000000000, 0.9394619383806329660, 1.000000000000000000),
 ( 1.000000000000000000, 0.9386961831921698529, 1.000000000000000000),
 ( 1.000000000000000000, 0.9378979462694481128, 1.000000000000000000),
 ( 1.000000000000000000, 0.9378737491732476173, 1.000000000000000000),
 ( 1.000000000000000000, 0.9378374413774223095, 1.000000000000000000),
 ( 1.000000000000000000, 0.9378252326299115760, 1.000000000000000000),
 ( 1.000000000000000000, 0.9378013115143154499, 1.000000000000000000),
 ( 1.000000000000000000, 0.9377893564346068134, 1.000000000000000000),
 ( 1.000000000000000000, 0.9377296084626393080, 1.000000000000000000),
 ( 1.000000000000000000, 0.9376818978498918655, 1.000000000000000000),
 ( 1.000000000000000000, 0.9375390306864356260, 1.000000000000000000),
 ( 1.000000000000000000, 0.9374441388112084717, 1.000000000000000000),
 ( 1.000000000000000000, 0.9371605328928015455, 1.000000000000000000),
 ( 1.000000000000000000, 0.9369728885716435141, 1.000000000000000000),
 ( 1.000000000000000000, 0.9364143219790276307, 1.000000000000000000),
 ( 1.000000000000000000, 0.9360477663173705221, 1.000000000000000000),
 ( 1.000000000000000000, 0.9342452504720827333, 1.000000000000000000),
 ( 1.000000000000000000, 0.9329001521055318991, 1.000000000000000000),
 ( 1.000000000000000000, 0.9304320728630436355, 1.000000000000000000),
 ( 1.000000000000000000, 0.9293115496648971519, 1.000000000000000000),
 ( 1.000000000000000000, 0.9273349178231704570, 1.000000000000000000),
 ( 1.000000000000000000, 0.9264755994062942035, 1.000000000000000000),
 ( 1.000000000000000000, 0.9243018539387418686, 1.000000000000000000),
 ( 1.000000000000000000, 0.9233922906947681364, 1.000000000000000000),
 ( 1.000000000000000000, 0.9230540990195943429, 1.000000000000000000) ) ) 
 REPRESENTATION_ITEM ( '' )  SURFACE ( )  );
#25479=CARTESIAN_POINT ( 'NONE',  ( 130.8568914410475088, -39.99999999999988631, -34.05028731879802706 ) ) ;
#25481=CARTESIAN_POINT ( 'NONE',  ( -82.30220482034332008, 7.992411108785294260, 18.51665893431345111 ) ) ;
#25482=CARTESIAN_POINT ( 'NONE',  ( -8.720657192082322595, -13.49580954685952072, -45.36528685024973129 ) ) ;
#25483=CARTESIAN_POINT ( 'NONE',  ( 0.2972598230770048811, -10.13633138497415942, -66.70487387989865624 ) ) ;
#25485=CARTESIAN_POINT ( 'NONE',  ( -135.8532207217289738, 3.005970985514575011E-13, -30.84685318188645553 ) ) ;
#25487=CARTESIAN_POINT ( 'NONE',  ( -238.4067589809705794, -0.9644942799826263791, -40.00000000000002132 ) ) ;
#25488=CARTESIAN_POINT ( 'NONE',  ( 163.1118516004056573, 19.27778845539212327, 37.29075403953164169 ) ) ;
#25489=CARTESIAN_POINT ( 'NONE',  ( 184.8905102610680444, 20.92133201514447194, -40.00000000000002132 ) ) ;
#25490=CARTESIAN_POINT ( 'NONE',  ( -2.652172544013597033, -43.38951316025622162, -23.73409167602006420 ) ) ;
#25491=CARTESIAN_POINT ( 'NONE',  ( 192.4448373802101173, 40.00000000000012790, -20.00000000003928236 ) ) ;
#25492=CARTESIAN_POINT ( 'NONE',  ( -198.0356074513804572, 1.247057299367198800E-13, -15.37879056873070560 ) ) ;
#25493=CARTESIAN_POINT ( 'NONE',  ( -192.9588430854690273, 66.79921049721887982, 10.23066800229522677 ) ) ;
#25494=CARTESIAN_POINT ( 'NONE',  ( 136.1360204305621266, 4.966164525587089429, 2.449293598294708485E-15 ) ) ;
#25495=ORIENTED_EDGE ( 'NONE', *, *, #20796, .T. ) ;
#25497=CARTESIAN_POINT ( 'NONE',  ( 22.57783252600012247, -43.22748647439753711, 17.90541116499475649 ) ) ;
#25500=CARTESIAN_POINT ( 'NONE',  ( -198.0356074513804572, 10.87444709758468875, 67.44298959250869530 ) ) ;
#25501=CARTESIAN_POINT ( 'NONE',  ( 19.06497207195981147, -4.605042221739098431E-14, 14.19242893257840521 ) ) ;
#25504=CARTESIAN_POINT ( 'NONE',  ( 22.82385994800818452, -13.83113328680564358, -47.01156385802205762 ) ) ;
#25507=ADVANCED_FACE ( 'NONE', ( #17199 ), #2570, .T. ) ;
#25508=CARTESIAN_POINT ( 'NONE',  ( -82.26674357280019478, -5.016125564933051173, -19.55222226025773935 ) ) ;
#25509=CARTESIAN_POINT ( 'NONE',  ( 151.7948205124836250, -33.23291073765550863, 0.000000000000000000 ) ) ;
#25510=CARTESIAN_POINT ( 'NONE',  ( 4.995406935893287326, 17.50105314357225694, -39.06748935135176026 ) ) ;
#25511=AXIS2_PLACEMENT_3D ( 'NONE', #6431, #4721, #12957 ) ;
#25513=CARTESIAN_POINT ( 'NONE',  ( 184.8905102610680444, 14.79361573936366092, 41.77492675556006674 ) ) ;
#25515=CARTESIAN_POINT ( 'NONE',  ( -30.26275506840322649, -29.48230279907769358, -29.48230279907820162 ) ) ;
#25516=CARTESIAN_POINT ( 'NONE',  ( 200.0000000000000000, 14.14213562373142352, -42.42640687119268961 ) ) ;
#25517=CARTESIAN_POINT ( 'NONE',  ( -213.1075012329537230, 9.698598906450543566, -9.698598906450348167 ) ) ;
#25518=CARTESIAN_POINT ( 'NONE',  ( 146.6084372240433993, 3.800685668858732935, -3.800685668858610367 ) ) ;
#25519=CARTESIAN_POINT ( 'NONE',  ( -91.56559293963834989, -22.67402823373193499, 0.000000000000000000 ) ) ;
#25522=CARTESIAN_POINT ( 'NONE',  ( 136.1360204305621266, -3.511608612531119000, 53.05693388239312469 ) ) ;
#25523=CARTESIAN_POINT ( 'NONE',  ( -188.8842190493874966, 43.30124183641388669, -17.93596163623950446 ) ) ;
#25525=CARTESIAN_POINT ( 'NONE',  ( 192.4448373802101173, 42.42640687116508502, -14.14213562375874567 ) ) ;
#25526=CARTESIAN_POINT ( 'NONE',  ( -82.26522933719705577, -17.41047943211789217, -10.29035321569880246 ) ) ;
#25527=CARTESIAN_POINT ( 'NONE',  ( 37.15749683964845218, 20.52531616279084759, 38.58455518508856841 ) ) ;
#25529=VERTEX_POINT ( 'NONE', #5111 ) ;
#25530=CARTESIAN_POINT ( 'NONE',  ( -188.8531444083262159, -43.29283928523321379, 17.93248118558238602 ) ) ;
#25533=CARTESIAN_POINT ( 'NONE',  ( 22.81400246987424651, -17.87890238636459728, 43.16348862150608312 ) ) ;
#25534=CARTESIAN_POINT ( 'NONE',  ( -114.4098922876147384, 20.15198150140922451, 8.347224046571190215 ) ) ;
#25537=CARTESIAN_POINT ( 'NONE',  ( -198.0356074513804572, 39.99999999999992895, 15.37879056873084771 ) ) ;
#25539=CARTESIAN_POINT ( 'NONE',  ( -200.0000000000000000, -17.28402242884604334, -46.84854965773187274 ) ) ;
#25540=CARTESIAN_POINT ( 'NONE',  ( -100.7734535825088500, -17.32597176626812185, -40.00000000000002132 ) ) ;
#25543=CARTESIAN_POINT ( 'NONE',  ( 0.2972598230770129857, -54.33493731733938148, 40.00000000000002132 ) ) ;
#25544=CARTESIAN_POINT ( 'NONE',  ( -208.1127848780265026, -15.00245453012673202, 0.000000000000000000 ) ) ;
#25547=CARTESIAN_POINT ( 'NONE',  ( -259.2033419157646676, 40.00000000000029843, -30.48217210827696988 ) ) ;
#25549=CARTESIAN_POINT ( 'NONE',  ( -280.0000000000000568, -40.00000000000028422, 19.99999999999959499 ) ) ;
#25552=CARTESIAN_POINT ( 'NONE',  ( -87.11162894489403641, 21.34897934681861287, -2.713946817477653095 ) ) ;
#25553=CARTESIAN_POINT ( 'NONE',  ( -4.027137536849644484, 46.99492183298354320, -13.82877337592798384 ) ) ;
#25554=CARTESIAN_POINT ( 'NONE',  ( -91.56559293963836410, 22.67402823373190301, 40.00000000000002132 ) ) ;
#25555=EDGE_CURVE ( 'NONE', #7172, #6927, #11843, .T. ) ;
#25556=CARTESIAN_POINT ( 'NONE',  ( -188.4701769959647777, 47.05181236278308177, -13.83721050406937358 ) ) ;
#25558=ORIENTED_EDGE ( 'NONE', *, *, #6062, .F. ) ;
#25561=CARTESIAN_POINT ( 'NONE',  ( 14.38125909742181285, -10.73282306404727393, 10.73282306404716380 ) ) ;
#25562=CARTESIAN_POINT ( 'NONE',  ( 130.8888609958233928, 12.21841679119731516, -29.49786752803534284 ) ) ;
#25563=CARTESIAN_POINT ( 'NONE',  ( -105.4741150117382062, 7.943527260750565588, -19.77569912955109288 ) ) ;
#25564=ORIENTED_EDGE ( 'NONE', *, *, #2485, .F. ) ;
#25567=DIRECTION ( 'NONE',  ( 0.01051738792034601078, 0.9307051272717529189, 0.3656191332813465977 ) ) ;
#25568=CARTESIAN_POINT ( 'NONE',  ( -238.4067589809705794, 57.25054294077225592, 0.6820004458485544596 ) ) ;
#25570=CARTESIAN_POINT ( 'NONE',  ( -192.9588430854689989, -8.596193650988133061E-14, 14.46834944099969533 ) ) ;
#25572=DIRECTION ( 'NONE',  ( 0.000000000000000000, 1.000000000000000000, 0.000000000000000000 ) ) ;
#25573=CARTESIAN_POINT ( 'NONE',  ( -4.039451493210497901, 23.44932283416708074, -43.00522595893983890 ) ) ;
#25574=CARTESIAN_POINT ( 'NONE',  ( -213.1075012329537230, -39.99999999999991473, -13.71589010951953647 ) ) ;
#25575=CARTESIAN_POINT ( 'NONE',  ( 136.1360204305621266, 7.947488714877270288E-14, -4.966164525587064560 ) ) ;
#25576=CARTESIAN_POINT ( 'NONE',  ( -82.30777374956703341, 18.64665802842208819, 7.678022728832912591 ) ) ;
#25577=CARTESIAN_POINT ( 'NONE',  ( -100.7734535825088500, -12.25131212657462498, -44.31723036834905827 ) ) ;
#25578=CARTESIAN_POINT ( 'NONE',  ( 146.6084372240433993, 1.478241399363601114E-13, -34.62501878078305850 ) ) ;
#25579=CARTESIAN_POINT ( 'NONE',  ( -162.0762913951020892, -1.198031840385783919, 1.198031840385741731 ) ) ;
#25580=CARTESIAN_POINT ( 'NONE',  ( 154.0339099654742370, 28.18615453125279657, 11.67508747798898661 ) ) ;
#25582=CARTESIAN_POINT ( 'NONE',  ( 184.8905102610680444, 43.07788698682572459, 13.49065550809829439 ) ) ;
#25583=CARTESIAN_POINT ( 'NONE',  ( -86.95438060917874168, -9.637778285156878511, 19.12135828302521290 ) ) ;
#25584=CARTESIAN_POINT ( 'NONE',  ( -238.4067589809705794, 0.6820004457340470561, 57.25054294065803617 ) ) ;
#25586=CARTESIAN_POINT ( 'NONE',  ( -192.9588430854690273, -38.51493924976957572, 18.05360324515410397 ) ) ;
#25588=CARTESIAN_POINT ( 'NONE',  ( -4.039451493210496125, 23.44932283416649454, 43.00522595894017286 ) ) ;
#25589=ORIENTED_EDGE ( 'NONE', *, *, #3142, .F. ) ;
#25590=CARTESIAN_POINT ( 'NONE',  ( -105.3755690713226727, 12.89780903124418998, -12.89780903124389155 ) ) ;
#25592=EDGE_CURVE ( 'NONE', #17844, #15971, #6365, .T. ) ;
#25594=EDGE_LOOP ( 'NONE', ( #8262, #18813, #6400, #21804 ) ) ;
#25595=CARTESIAN_POINT ( 'NONE',  ( -198.0356074513804572, 1.247057299367198800E-13, -15.37879056873070560 ) ) ;
#25597=EDGE_CURVE ( 'NONE', #12394, #11522, #15645, .T. ) ;
#25598=CARTESIAN_POINT ( 'NONE',  ( -16.41594856527310142, 21.03672846649599748, 39.35878123536664219 ) ) ;
#25601=CARTESIAN_POINT ( 'NONE',  ( -198.9233928135190581, -44.84148042516751786, -24.80620717268675790 ) ) ;
#25602=CARTESIAN_POINT ( 'NONE',  ( 57.59792236341147031, 39.99999999999990763, 37.56421063658199699 ) ) ;
#25603=EDGE_CURVE ( 'NONE', #23960, #8098, #4892, .T. ) ;
#25605=CARTESIAN_POINT ( 'NONE',  ( -94.58360650938176661, -20.58386743652064510, -9.000712009641768319 ) ) ;
#25608=CARTESIAN_POINT ( 'NONE',  ( -100.7734535825088358, -8.145438380286941744E-14, 17.32597176626811120 ) ) ;
#25611=CARTESIAN_POINT ( 'NONE',  ( -162.0762913951020892, 1.198031840385732849, -1.198031840385733515 ) ) ;
#25612=CARTESIAN_POINT ( 'NONE',  ( 19.06497207195980792, 18.24870850772790831, -38.31983398719609824 ) ) ;
#25613=CARTESIAN_POINT ( 'NONE',  ( -86.91014751117384662, -19.35827336066798665, 9.009177718430992243 ) ) ;
#25614=CARTESIAN_POINT ( 'NONE',  ( 192.4448373802100889, 2.472897170449861688E-13, -19.99999999996060751 ) ) ;
#25615=CARTESIAN_POINT ( 'NONE',  ( 170.0000000000000284, -22.62041470344884431, 9.369682556672202622 ) ) ;
#25616=CARTESIAN_POINT ( 'NONE',  ( -192.9588430854690273, -14.46834944099973264, 40.00000000000002132 ) ) ;
#25617=CARTESIAN_POINT ( 'NONE',  ( 192.4448373802101173, -19.99999999996056843, -40.00000000000002132 ) ) ;
#25618=CARTESIAN_POINT ( 'NONE',  ( -91.56559293963836410, 16.03295912088714203, -16.03295912088699282 ) ) ;
#25619=CARTESIAN_POINT ( 'NONE',  ( -100.7734535825088500, 22.67402823373189946, -40.00000000000002132 ) ) ;
#25620=CARTESIAN_POINT ( 'NONE',  ( 1.564570055219380640, -44.28524390194900207, -24.39611894128482916 ) ) ;
#25623=CARTESIAN_POINT ( 'NONE',  ( 0.2972598230769959993, 38.42060263243659080, 38.42060263243672580 ) ) ;
#25624=CARTESIAN_POINT ( 'NONE',  ( 4.995406935893289102, 55.24977328856464709, -40.00000000000002132 ) ) ;
#25626=( BOUNDED_SURFACE ( )  B_SPLINE_SURFACE ( 3, 2, ( 
 ( #5226, #9214, #25459 ),
 ( #21577, #3351, #21332 ),
 ( #11084, #9594, #17571 ),
 ( #15325, #11451, #5478 ),
 ( #3483, #11207, #3227 ),
 ( #17699, #9087, #11580 ),
 ( #13087, #1235, #19700 ),
 ( #1488, #25843, #7587 ),
 ( #4980, #9340, #982 ),
 ( #19322, #1106, #7210 ),
 ( #23452, #25977, #18101 ),
 ( #6134, #19970, #24371 ),
 ( #21837, #7985, #2024 ),
 ( #12119, #21972, #13712 ),
 ( #5733, #24235, #12253 ),
 ( #22109, #23958, #5869 ),
 ( #6008, #14117, #17830 ),
 ( #1751, #10260, #13838 ),
 ( #14242, #13975, #18370 ),
 ( #26109, #20244, #4158 ),
 ( #9991, #20375, #11986 ),
 ( #3744, #10126, #3885 ),
 ( #26250, #20109, #24094 ),
 ( #17962, #22382, #16103 ),
 ( #11849, #18227, #3606 ),
 ( #14, #2150, #7848 ),
 ( #22244, #1886, #9860 ),
 ( #15969, #4019, #8125 ),
 ( #16242, #149, #8253 ),
 ( #23823, #5606, #19835 ),
 ( #11716, #1621, #7718 ),
 ( #9728, #15828, #26117 ),
 ( #4297, #24105, #20117 ),
 ( #7856, #3752, #22390 ) ),
 .UNSPECIFIED., .F., .F., .T. ) 
 B_SPLINE_SURFACE_WITH_KNOTS ( ( 4, 2, 2, 2, 2, 2, 2, 2, 2, 2, 2, 2, 2, 2, 2, 2, 4 ),
 ( 3, 3 ),
 ( 0.005135431517081092551, 0.02907016617530085861, 0.05300490083352062815, 0.07693963549174039074, 0.08292331915629533312, 0.08441924007243406525, 0.08446598760106339976, 0.08448936136537807395, 0.08451273512969273427, 0.08460623018695140329, 0.08479322030146874134, 0.08516720053050343131, 0.08591516098857279737, 0.08890700282085027550, 0.09189884465312775363, 0.09489068648540521789, 0.1008743701499601603 ),
 ( 0.000000000000000000, 1.000000000000000000 ),
 .UNSPECIFIED. ) 
 GEOMETRIC_REPRESENTATION_ITEM ( )  RATIONAL_B_SPLINE_SURFACE ( (
 ( 1.000000000000000000, 0.9997813423552077694, 1.000000000000000000),
 ( 1.000000000000000000, 0.9991063894442805404, 1.000000000000000000),
 ( 1.000000000000000000, 0.9968824679670508226, 1.000000000000000000),
 ( 1.000000000000000000, 0.9891556708430847555, 1.000000000000000000),
 ( 1.000000000000000000, 0.9836552227706814033, 1.000000000000000000),
 ( 1.000000000000000000, 0.9690804699595860772, 1.000000000000000000),
 ( 1.000000000000000000, 0.9600093828096437631, 1.000000000000000000),
 ( 1.000000000000000000, 0.9461484455227653356, 1.000000000000000000),
 ( 1.000000000000000000, 0.9432496483672401233, 1.000000000000000000),
 ( 1.000000000000000000, 0.9394619383806339652, 1.000000000000000000),
 ( 1.000000000000000000, 0.9386961831920875854, 1.000000000000000000),
 ( 1.000000000000000000, 0.9378979462694514435, 1.000000000000000000),
 ( 1.000000000000000000, 0.9378737491732502818, 1.000000000000000000),
 ( 1.000000000000000000, 0.9378374413774224205, 1.000000000000000000),
 ( 1.000000000000000000, 0.9378252326299112429, 1.000000000000000000),
 ( 1.000000000000000000, 0.9378013115143177814, 1.000000000000000000),
 ( 1.000000000000000000, 0.9377893564346067024, 1.000000000000000000),
 ( 1.000000000000000000, 0.9377296084626435269, 1.000000000000000000),
 ( 1.000000000000000000, 0.9376818978498911994, 1.000000000000000000),
 ( 1.000000000000000000, 0.9375390306864400669, 1.000000000000000000),
 ( 1.000000000000000000, 0.9374441388111988127, 1.000000000000000000),
 ( 1.000000000000000000, 0.9371605328928230838, 1.000000000000000000),
 ( 1.000000000000000000, 0.9369728885716236411, 1.000000000000000000),
 ( 1.000000000000000000, 0.9364143219790700412, 1.000000000000000000),
 ( 1.000000000000000000, 0.9360477663173711882, 1.000000000000000000),
 ( 1.000000000000000000, 0.9342452504720832884, 1.000000000000000000),
 ( 1.000000000000000000, 0.9329001521054770540, 1.000000000000000000),
 ( 1.000000000000000000, 0.9304320728630998127, 1.000000000000000000),
 ( 1.000000000000000000, 0.9293115496652294416, 1.000000000000000000),
 ( 1.000000000000000000, 0.9273349178228399436, 1.000000000000000000),
 ( 1.000000000000000000, 0.9264755994061858457, 1.000000000000000000),
 ( 1.000000000000000000, 0.9243018539389626920, 1.000000000000000000),
 ( 1.000000000000000000, 0.9233922906946046005, 1.000000000000000000),
 ( 1.000000000000000000, 0.9230540990195957862, 1.000000000000000000) ) ) 
 REPRESENTATION_ITEM ( '' )  SURFACE ( )  );
#25627=CARTESIAN_POINT ( 'NONE',  ( 23.36462152323065311, -46.81175967489662071, 13.80148662728995568 ) ) ;
#25629=CARTESIAN_POINT ( 'NONE',  ( -91.56559293963834989, 12.25131212657480440, 12.25131212657486834 ) ) ;
#25631=CARTESIAN_POINT ( 'NONE',  ( -87.01809839470989516, 20.74596926290789156, -5.316578559416913485 ) ) ;
#25632=CARTESIAN_POINT ( 'NONE',  ( -16.87994666115289988, 12.91133298909479166, -42.52193590819778279 ) ) ;
#25635=CARTESIAN_POINT ( 'NONE',  ( -86.99952317291963766, -5.713267018748582338, -20.62702873475882370 ) ) ;
#25636=CARTESIAN_POINT ( 'NONE',  ( -91.56559293963834989, -16.03295912088728414, 16.03295912088688269 ) ) ;
#25637=CARTESIAN_POINT ( 'NONE',  ( 146.6084372240433709, 24.48358557860356655, -32.08495691632035118 ) ) ;
#25638=CARTESIAN_POINT ( 'NONE',  ( -105.2105218841390126, 21.45999192170251035, -1.182031380070910798 ) ) ;
#25640=CARTESIAN_POINT ( 'NONE',  ( 57.59792236341148453, 1.722363176415528940, -54.84617931850878136 ) ) ;
#25641=CARTESIAN_POINT ( 'NONE',  ( -135.8532207217289738, -21.81201906317757633, -21.81201906317793515 ) ) ;
#25642=CARTESIAN_POINT ( 'NONE',  ( 57.59792236341147031, -30.00663442387662627, -26.56190807104723461 ) ) ;
#25643=CARTESIAN_POINT ( 'NONE',  ( 0.2972598230769907257, 66.70487387989869887, -10.13633138497392494 ) ) ;
#25644=CARTESIAN_POINT ( 'NONE',  ( -105.3220005116046849, -10.86457728905244124, 18.46446237100853338 ) ) ;
#25646=CARTESIAN_POINT ( 'NONE',  ( 0.2972598230770030492, -40.00000000000007816, 14.33493731733919496 ) ) ;
#25647=CARTESIAN_POINT ( 'NONE',  ( -259.2033419157646676, -49.83842185052040463, 6.730120644403092101 ) ) ;
#25648=CARTESIAN_POINT ( 'NONE',  ( 136.1360204305621551, 4.966164525587085876, 40.00000000000002132 ) ) ;
#25650=CARTESIAN_POINT ( 'NONE',  ( 151.7948205124836534, 4.785054706298574878, -51.78348778862537927 ) ) ;
#25651=CARTESIAN_POINT ( 'NONE',  ( -2.717871546781097880, 42.53710973099089188, 17.61944775472897717 ) ) ;
#25653=CARTESIAN_POINT ( 'NONE',  ( -5.859158571313241026, -42.46836465824206641, -23.09435402966316175 ) ) ;
#25654=ORIENTED_EDGE ( 'NONE', *, *, #7013, .T. ) ;
#25655=CARTESIAN_POINT ( 'NONE',  ( -105.2113312088911385, 16.16375985776740620, 14.17769269060415738 ) ) ;
#25656=B_SPLINE_CURVE_WITH_KNOTS ( 'NONE', 3,
 ( #11769, #16559, #24419, #18557, #12431, #12174, #22826, #10440 ),
 .UNSPECIFIED., .F., .F.,
 ( 4, 2, 2, 4 ),
 ( 0.008471746897510642679, 0.01052245438202778841, 0.01257316186654493587, 0.01667457683557922732 ),
 .UNSPECIFIED. ) ;
#25658=CARTESIAN_POINT ( 'NONE',  ( 90.71511022962279469, -9.285713562939564625, 21.07400258644036484 ) ) ;
#25662=CARTESIAN_POINT ( 'NONE',  ( -30.26275506840325136, 40.00000000000001421, 1.694272468446399227 ) ) ;
#25663=CARTESIAN_POINT ( 'NONE',  ( -77.58456292359235817, -2.764817855541193747, 21.97699700613614837 ) ) ;
#25665=CARTESIAN_POINT ( 'NONE',  ( 170.2234770963711128, -15.44714144992812876, -2.449293598294708485E-15 ) ) ;
#25666=CARTESIAN_POINT ( 'NONE',  ( -114.4364955367313996, 8.064892380834940866, -20.29001642039080622 ) ) ;
#25668=CARTESIAN_POINT ( 'NONE',  ( 200.0000000000000000, -19.99999999999989342, 40.00000000000002132 ) ) ;
#25669=CARTESIAN_POINT ( 'NONE',  ( -56.48582580120559982, 34.75652343174597547, 21.81201906317791384 ) ) ;
#25670=CARTESIAN_POINT ( 'NONE',  ( -213.1075012329537230, 13.71589010951907817, 40.00000000000002132 ) ) ;
#25671=CARTESIAN_POINT ( 'NONE',  ( 192.4448373802101173, 39.99999999999985079, 20.00000000003984013 ) ) ;
#25672=CARTESIAN_POINT ( 'NONE',  ( -135.8532207217289738, -39.99999999999972289, -30.84685318188688541 ) ) ;
#25674=VERTEX_POINT ( 'NONE', #8131 ) ;
#25676=CARTESIAN_POINT ( 'NONE',  ( 8.209392600928651973, 49.31072049265984703, -14.17653494425351290 ) ) ;
#25677=CARTESIAN_POINT ( 'NONE',  ( 4.995406935893309530, -55.24977328856464709, 40.00000000000002132 ) ) ;
#25679=CARTESIAN_POINT ( 'NONE',  ( -188.9266304146017887, 43.31220791188989239, -17.94050393342734040 ) ) ;
#25683=CARTESIAN_POINT ( 'NONE',  ( -88.39148973765254880, -19.92926839984449217, 8.577159256668625886 ) ) ;
#25684=CARTESIAN_POINT ( 'NONE',  ( 141.7948666911895259, 12.58737617328916158, -30.38861427224623668 ) ) ;
#25685=ORIENTED_EDGE ( 'NONE', *, *, #26060, .F. ) ;
#25686=CARTESIAN_POINT ( 'NONE',  ( -162.0762913951021176, 57.76657433523994456, -1.198031840315424867 ) ) ;
#25690=CARTESIAN_POINT ( 'NONE',  ( 163.1118516004056573, 37.29075403953160617, -19.27778845539222985 ) ) ;
#25692=CARTESIAN_POINT ( 'NONE',  ( 0.2972598230769957217, -4.999556039334937811E-14, 14.33493731733933352 ) ) ;
#25693=CARTESIAN_POINT ( 'NONE',  ( -105.2054292635175869, -15.19799821370180126, -15.19799821370278892 ) ) ;
#25695=CARTESIAN_POINT ( 'NONE',  ( -16.41582555379474684, 21.03675245593366583, -39.35881747758678983 ) ) ;
#25696=CARTESIAN_POINT ( 'NONE',  ( 98.29820294270304259, -18.47759065022024672, 7.653668647299475047 ) ) ;
#25697=CARTESIAN_POINT ( 'NONE',  ( -280.0000000000000000, 1.605030083646939673E-13, -20.00000000000001421 ) ) ;
#25698=CARTESIAN_POINT ( 'NONE',  ( -110.0368417077422691, -7.992411109419241377, 18.51665893311217559 ) ) ;
#25699=CARTESIAN_POINT ( 'NONE',  ( 163.1118516004056573, 19.27778845538780317, -19.27778845538757224 ) ) ;
#25701=CARTESIAN_POINT ( 'NONE',  ( -199.9999999999998863, -44.86878812508856385, -24.82633483071075986 ) ) ;
#25702=CARTESIAN_POINT ( 'NONE',  ( 169.9999999999999432, 22.62041470344884075, 9.369682556672378482 ) ) ;
#25704=CARTESIAN_POINT ( 'NONE',  ( 192.4448373802101173, 42.42640687122070631, 14.14213562370331623 ) ) ;
#25705=CARTESIAN_POINT ( 'NONE',  ( -238.4067589809705794, -40.00000000000007105, 0.9644942799824426372 ) ) ;
#25706=CARTESIAN_POINT ( 'NONE',  ( -56.48582580120559982, -6.472252184284282173, 50.09629031063965243 ) ) ;
#25707=CARTESIAN_POINT ( 'NONE',  ( 146.6084372240433993, -3.800685668858596156, -3.800685668858692967 ) ) ;
#25710=ORIENTED_EDGE ( 'NONE', *, *, #8923, .F. ) ;
#25711=CARTESIAN_POINT ( 'NONE',  ( 91.82158438592158234, -12.16597498399995203, -44.40256751092347542 ) ) ;
#25714=VERTEX_POINT ( 'NONE', #26256 ) ;
#25715=CARTESIAN_POINT ( 'NONE',  ( 0.2972598230769957217, 1.502051041545559470E-13, -14.33493731733933352 ) ) ;
#25717=CARTESIAN_POINT ( 'NONE',  ( -47.65341557557733410, 10.55973086684486262, 31.50022537349512319 ) ) ;
#25718=ORIENTED_EDGE ( 'NONE', *, *, #8336, .F. ) ;
#25720=CARTESIAN_POINT ( 'NONE',  ( -193.3669098796383139, -44.23532903079497203, -18.32287322058288126 ) ) ;
#25721=CARTESIAN_POINT ( 'NONE',  ( -238.4067589809705794, 39.99999999999983658, 40.96449428006354765 ) ) ;
#25724=EDGE_CURVE ( 'NONE', #17668, #17072, #3750, .T. ) ;
#25726=CARTESIAN_POINT ( 'NONE',  ( -56.48582580120557850, -40.00000000000014211, 30.84685318188629921 ) ) ;
#25730=CARTESIAN_POINT ( 'NONE',  ( 136.1360204305621551, 40.00000000000002842, 4.966164525587208445 ) ) ;
#25731=CARTESIAN_POINT ( 'NONE',  ( -83.21262154144253032, -13.72187187061455127, -33.12752917118434937 ) ) ;
#25732=CARTESIAN_POINT ( 'NONE',  ( -47.65341557555752416, -10.55973086695903618, -31.50022537343778595 ) ) ;
#25733=CARTESIAN_POINT ( 'NONE',  ( -208.1127848780264742, -10.60833733270725787, -67.17687982763172272 ) ) ;
#25734=CARTESIAN_POINT ( 'NONE',  ( 170.0000000000427178, -17.64300463311358769, 17.64300463311318268 ) ) ;
#25735=CARTESIAN_POINT ( 'NONE',  ( 146.6084372240433709, -40.00000000000036238, 34.62501878078263218 ) ) ;
#25736=CARTESIAN_POINT ( 'NONE',  ( 23.37394308801976450, 13.80096434448266685, 46.80823611210199431 ) ) ;
#25737=CARTESIAN_POINT ( 'NONE',  ( 136.1360204305621551, -4.966164525587043244, 40.00000000000002132 ) ) ;
#25738=CARTESIAN_POINT ( 'NONE',  ( 0.2972598230770129857, -54.33493731733936016, -40.00000000000002132 ) ) ;
#25739=EDGE_CURVE ( 'NONE', #6802, #19642, #11467, .T. ) ;
#25741=CARTESIAN_POINT ( 'NONE',  ( -56.48582580120559271, 6.472252184284211118, -6.472252184284153387 ) ) ;
#25743=CARTESIAN_POINT ( 'NONE',  ( 14.38125909742181285, -15.17850393972633505, 0.000000000000000000 ) ) ;
#25744=CARTESIAN_POINT ( 'NONE',  ( 22.89172254855148481, -43.00256445985474585, -23.44749030158409298 ) ) ;
#25748=CARTESIAN_POINT ( 'NONE',  ( 151.7948205124836250, 4.785054706301690608, 4.785054706301682614 ) ) ;
#25749=CARTESIAN_POINT ( 'NONE',  ( -208.1127848780264742, 55.00245453010919050, -40.00000000000002132 ) ) ;
#25751=CARTESIAN_POINT ( 'NONE',  ( 23.05038679986302341, -43.09692730307091324, 17.85133178553853739 ) ) ;
#25753=B_SPLINE_CURVE_WITH_KNOTS ( 'NONE', 3,
 ( #8778, #2803, #934, #6378, #24758, #17019 ),
 .UNSPECIFIED., .F., .F.,
 ( 4, 2, 4 ),
 ( 0.3689590070116580689, 0.3867117631979620773, 0.4044645193949217288 ),
 .UNSPECIFIED. ) ;
#25755=CARTESIAN_POINT ( 'NONE',  ( -280.0000000000000568, 42.42640687119285303, -14.14213562373088351 ) ) ;
#25756=CARTESIAN_POINT ( 'NONE',  ( 0.2972598230770030492, -40.00000000000007816, 14.33493731733919496 ) ) ;
#25757=CARTESIAN_POINT ( 'NONE',  ( 170.2234770963711128, -17.36149277827010096, 17.36149277826970660 ) ) ;
#25759=CARTESIAN_POINT ( 'NONE',  ( -238.4067589809705794, 0.9644942799825385604, -40.00000000000002132 ) ) ;
#25762=CARTESIAN_POINT ( 'NONE',  ( -86.94888381182468606, -6.689462128214199055, -20.30418897962128000 ) ) ;
#25763=CARTESIAN_POINT ( 'NONE',  ( -86.96347745069644475, 12.89780903124349898, 43.67073346367994446 ) ) ;
#25764=CARTESIAN_POINT ( 'NONE',  ( -30.26275506840325136, 27.08623969584614244, -29.48230279907770779 ) ) ;
#25765=CARTESIAN_POINT ( 'NONE',  ( 163.1118516004056573, 19.27778845538780317, -19.27778845538757224 ) ) ;
#25766=CARTESIAN_POINT ( 'NONE',  ( -83.21262154144248768, 33.12752917118453411, -13.72187187061400415 ) ) ;
#25767=CARTESIAN_POINT ( 'NONE',  ( 14.38125909742181996, -10.73282306405815234, -67.30136555898266693 ) ) ;
#25768=CARTESIAN_POINT ( 'NONE',  ( -30.26275506840323359, -1.198031551615522439, -57.76657404653986561 ) ) ;
#25769=CARTESIAN_POINT ( 'NONE',  ( 130.8568914410475088, -24.07718906446864793, -32.49135343045505664 ) ) ;
#25770=CARTESIAN_POINT ( 'NONE',  ( 0.2972598230769990524, -18.14793986248671231, -38.42060263243687501 ) ) ;
#25773=CARTESIAN_POINT ( 'NONE',  ( -198.0356074513804572, -40.00000000000011369, 15.37879056873056527 ) ) ;
#25775=CARTESIAN_POINT ( 'NONE',  ( 14.38125909742180752, 55.17850393974265444, 40.00000000000002132 ) ) ;
#25776=ORIENTED_EDGE ( 'NONE', *, *, #6452, .T. ) ;
#25777=AXIS2_PLACEMENT_3D ( 'NONE', #13257, #21380, #3152 ) ;
#25778=CARTESIAN_POINT ( 'NONE',  ( 200.0000000000000000, 42.42640687119288856, -14.14213562373094746 ) ) ;
#25779=CARTESIAN_POINT ( 'NONE',  ( -41.56387280713217791, 32.03616492527998361, 13.26981399847223564 ) ) ;
#25780=CARTESIAN_POINT ( 'NONE',  ( 98.29820294267331349, 7.653668647304012751, 18.47759065023121039 ) ) ;
#25781=CARTESIAN_POINT ( 'NONE',  ( -105.2940237833723813, -4.710801307188510201, 20.91877113669150745 ) ) ;
#25782=ORIENTED_EDGE ( 'NONE', *, *, #348, .T. ) ;
#25783=CARTESIAN_POINT ( 'NONE',  ( -188.9524464570969258, -47.22058047019496740, 13.86227157644530017 ) ) ;
#25785=CARTESIAN_POINT ( 'NONE',  ( 60.07376046262002944, -13.17995839195482333, 31.81923430127606167 ) ) ;
#25786=CARTESIAN_POINT ( 'NONE',  ( 23.10188454848723083, 23.40120037233813477, -42.94013537404166669 ) ) ;
#25790=CARTESIAN_POINT ( 'NONE',  ( 151.7948205124836534, 40.00000000000002842, 6.767089262349174739 ) ) ;
#25793=CARTESIAN_POINT ( 'NONE',  ( 23.23834162557336924, 46.85950693575997406, -13.80856396595088320 ) ) ;
#25794=CARTESIAN_POINT ( 'NONE',  ( -213.1075012329537230, -13.71589010951915810, 40.00000000000002132 ) ) ;
#25795=CARTESIAN_POINT ( 'NONE',  ( 98.29820294267329928, -7.653668647303861761, -18.47759065023126013 ) ) ;
#25798=CARTESIAN_POINT ( 'NONE',  ( -213.1075012329537230, -53.71589010953668719, -40.00000000000002132 ) ) ;
#25799=CARTESIAN_POINT ( 'NONE',  ( -56.48582580120559271, -9.153146818113595984, 0.000000000000000000 ) ) ;
#25800=CARTESIAN_POINT ( 'NONE',  ( 170.2234770963711128, 40.00000000000021316, -15.44714144992773797 ) ) ;
#25802=CARTESIAN_POINT ( 'NONE',  ( -30.26275506840324070, -1.198031551616016266, -1.198031551616031587 ) ) ;
#25805=CARTESIAN_POINT ( 'NONE',  ( 98.29820294267338454, 8.858778887860573548, -17.94316440882722929 ) ) ;
#25806=CARTESIAN_POINT ( 'NONE',  ( 192.4448373802101173, 20.00000000003945644, 40.00000000000002132 ) ) ;
#25810=VERTEX_POINT ( 'NONE', #9734 ) ;
#25813=CARTESIAN_POINT ( 'NONE',  ( -100.0753760173624869, -20.41987330121788702, 8.894334231739227548 ) ) ;
#25814=CARTESIAN_POINT ( 'NONE',  ( 158.3379117892984880, 10.98149362779651206, -26.51167085133954160 ) ) ;
#25816=CARTESIAN_POINT ( 'NONE',  ( 0.2972598230769930017, 54.33493731733938148, -40.00000000000002132 ) ) ;
#25817=CARTESIAN_POINT ( 'NONE',  ( -99.31364972221751941, -20.79869444138732959, 8.164808577175515225 ) ) ;
#25818=ORIENTED_EDGE ( 'NONE', *, *, #58, .F. ) ;
#25822=CARTESIAN_POINT ( 'NONE',  ( 91.82158438592158234, 44.40256751092336884, -12.16597498400043342 ) ) ;
#25823=DIRECTION ( 'NONE',  ( 0.000000000000000000, 1.000000000000000000, 0.000000000000000000 ) ) ;
#25824=CARTESIAN_POINT ( 'NONE',  ( 14.38125909742181108, -5.035366881890652543E-14, 15.17850393972633682 ) ) ;
#25825=CARTESIAN_POINT ( 'NONE',  ( -1.828631717523949929, -13.94691770808705478, 47.79123445029436823 ) ) ;
#25826=CARTESIAN_POINT ( 'NONE',  ( -87.13361725327072804, 8.813415818526478339E-15, 21.49321519333429009 ) ) ;
#25828=CARTESIAN_POINT ( 'NONE',  ( 98.29820294267867098, 15.96737102139294606, 12.31690022607448221 ) ) ;
#25829=CARTESIAN_POINT ( 'NONE',  ( -99.21568817060986589, -16.03295912088728770, 16.03295912088687913 ) ) ;
#25830=CARTESIAN_POINT ( 'NONE',  ( 4.995406935893297984, -39.99999999999986500, -15.24977328854874870 ) ) ;
#25831=CARTESIAN_POINT ( 'NONE',  ( -114.6097568999262393, -10.88341597697256269, 19.09891331899296318 ) ) ;
#25832=CARTESIAN_POINT ( 'NONE',  ( 192.4448373802101173, -14.14213562370283128, -42.42640687122081999 ) ) ;
#25833=CARTESIAN_POINT ( 'NONE',  ( 136.1360204305621551, 40.00000000000017053, -35.03383547441281820 ) ) ;
#25835=CARTESIAN_POINT ( 'NONE',  ( -208.1127848780264742, -38.89260858015728672, -17.67593391476669851 ) ) ;
#25836=CARTESIAN_POINT ( 'NONE',  ( 140.2235668266256425, 30.42137084504298628, 12.60094438999839994 ) ) ;
#25839=FACE_OUTER_BOUND ( 'NONE', #26260, .T. ) ;
#25840=CARTESIAN_POINT ( 'NONE',  ( -135.8532207217289738, 7.002209520526292428E-15, -9.153146818113572891 ) ) ;
#25841=CARTESIAN_POINT ( 'NONE',  ( -259.2033419157646676, -6.730120644403667640, 49.83842185052029805 ) ) ;
#25842=CARTESIAN_POINT ( 'NONE',  ( 57.59792236341148453, -54.84617931850879557, 1.722363176414566155 ) ) ;
#25843=CARTESIAN_POINT ( 'NONE',  ( -183.6285492669668997, -17.34367427887346480, -41.87133366542966684 ) ) ;
#25844=CARTESIAN_POINT ( 'NONE',  ( 91.82158438592158234, 12.16597498397773869, -12.16597498397759303 ) ) ;
#25846=CARTESIAN_POINT ( 'NONE',  ( 91.82158438592158234, 16.11829626346161604, -16.11829626346121103 ) ) ;
#25848=CARTESIAN_POINT ( 'NONE',  ( -53.37717264285771535, 10.11115224722917993, -29.42738956023907093 ) ) ;
#25849=CARTESIAN_POINT ( 'NONE',  ( 199.9999999999999432, 14.14213562373110911, -14.14213562373072364 ) ) ;
#25850=CARTESIAN_POINT ( 'NONE',  ( -77.90255099907052738, 8.064892378688682584, 20.29001641119209154 ) ) ;
#25854=CARTESIAN_POINT ( 'NONE',  ( 8.517493242716003721, -44.90626920808415434, 24.85395068094661397 ) ) ;
#25857=CARTESIAN_POINT ( 'NONE',  ( -56.48582580120559982, 30.84685318188643777, -40.00000000000002132 ) ) ;
#25858=FACE_OUTER_BOUND ( 'NONE', #11095, .T. ) ;
#25859=CARTESIAN_POINT ( 'NONE',  ( -162.0762913951021176, 39.99999999999998579, 1.694272876828463614 ) ) ;
#25860=CARTESIAN_POINT ( 'NONE',  ( 190.0000000000001137, -30.00000000000000711, 3.673940397442064700E-15 ) ) ;
#25861=CARTESIAN_POINT ( 'NONE',  ( -208.1127848780265026, 1.189126717069624012E-13, -15.00245453012669472 ) ) ;
#25862=CARTESIAN_POINT ( 'NONE',  ( 130.8568914410475372, 8.154165912415230659E-16, 5.949712681206690945 ) ) ;
#25864=CARTESIAN_POINT ( 'NONE',  ( -208.1127848780264742, 39.99999999999992895, 15.00245453012683683 ) ) ;
#25865=CARTESIAN_POINT ( 'NONE',  ( -121.3893627896829770, 22.57752009493451339, 9.351915028061926094 ) ) ;
#25866=CARTESIAN_POINT ( 'NONE',  ( -135.8532207217289738, -6.472252184284280396, 6.472252184284099208 ) ) ;
#25867=CARTESIAN_POINT ( 'NONE',  ( 151.7948205124836250, 23.49921654116328540, 23.49921654116366554 ) ) ;
#25869=CARTESIAN_POINT ( 'NONE',  ( 14.38125909742181818, -39.99999999999986500, -15.17850393972675604 ) ) ;
#25871=CARTESIAN_POINT ( 'NONE',  ( 19.06497207195982924, -54.19242893257843008, 40.00000000000002132 ) ) ;
#25872=CARTESIAN_POINT ( 'NONE',  ( -105.3755690713226585, -18.24025645688353947, -40.00000000000002132 ) ) ;
#25873=CARTESIAN_POINT ( 'NONE',  ( 170.2234770963711128, 45.64576402573181468, 10.92277846919223627 ) ) ;
#25874=CARTESIAN_POINT ( 'NONE',  ( -86.96347745069645896, 21.75974354311648895, -0.000000000000000000 ) ) ;
#25875=CARTESIAN_POINT ( 'NONE',  ( -105.2054292635175443, 0.6800022380124111088, 21.49321519473986442 ) ) ;
#25876=CARTESIAN_POINT ( 'NONE',  ( 14.38125909742181108, 1.616281842095393922E-13, -15.17850393972633682 ) ) ;
#25877=CARTESIAN_POINT ( 'NONE',  ( -280.0000000000000568, 42.42640687119285303, -14.14213562373088351 ) ) ;
#25878=CARTESIAN_POINT ( 'NONE',  ( -213.1075012329537230, 53.71589010951910836, 2.449293598294708485E-15 ) ) ;
#25880=ORIENTED_EDGE ( 'NONE', *, *, #14642, .F. ) ;
#25881=EDGE_CURVE ( 'NONE', #151, #23459, #4237, .T. ) ;
#25882=CARTESIAN_POINT ( 'NONE',  ( 44.46627453565378119, -36.79413088022850786, 15.24062802607578249 ) ) ;
#25883=DIRECTION ( 'NONE',  ( 1.000000000000000000, 0.000000000000000000, 0.000000000000000000 ) ) ;
#25884=CARTESIAN_POINT ( 'NONE',  ( 170.2234770963711128, 39.20704971665398375, -17.36149277826984871 ) ) ;
#25885=CARTESIAN_POINT ( 'NONE',  ( 130.8568914410475372, 8.154165912415230659E-16, 5.949712681206690945 ) ) ;
#25886=CARTESIAN_POINT ( 'NONE',  ( 4.995406935893289102, 10.78321810389013002, -10.78321810388986712 ) ) ;
#25887=EDGE_CURVE ( 'NONE', #22617, #13720, #17220, .T. ) ;
#25888=CARTESIAN_POINT ( 'NONE',  ( 0.2972598230769930572, 14.33493731733933352, 0.000000000000000000 ) ) ;
#25889=CARTESIAN_POINT ( 'NONE',  ( 200.0000000000000000, -20.00000000000006750, -40.00000000000002132 ) ) ;
#25891=CARTESIAN_POINT ( 'NONE',  ( -175.9234121947850440, -39.35887396291793294, -21.03678982257773455 ) ) ;
#25893=CARTESIAN_POINT ( 'NONE',  ( 170.0000000000427178, -17.64300463311358769, 17.64300463311318268 ) ) ;
#25894=CARTESIAN_POINT ( 'NONE',  ( -280.0000000000000000, -14.14213562373118549, 14.14213562373078936 ) ) ;
#25895=CARTESIAN_POINT ( 'NONE',  ( -56.48582580120558561, -21.81201906317755146, -21.81201906317792449 ) ) ;
#25896=CARTESIAN_POINT ( 'NONE',  ( -190.1760961840481627, -13.92889018258695799, 47.67020129369084458 ) ) ;
#25897=CARTESIAN_POINT ( 'NONE',  ( -77.55632011646486035, 15.16702236932743375, -16.13210123263645812 ) ) ;
#25898=CARTESIAN_POINT ( 'NONE',  ( 151.7948205124836534, 23.49921654116056047, -33.06932595376338213 ) ) ;
#25899=CARTESIAN_POINT ( 'NONE',  ( -86.96347745069644475, -12.89780903124395195, -12.89780903124416511 ) ) ;
#25900=CARTESIAN_POINT ( 'NONE',  ( 130.8568914410475088, -52.36146031193413108, -4.207082182990267150 ) ) ;
#25901=CARTESIAN_POINT ( 'NONE',  ( -105.3755690713226585, -43.67073346367964604, -12.89780903124457545 ) ) ;
#25906=CARTESIAN_POINT ( 'NONE',  ( 151.7948205124836250, 1.439163438361279259E-13, -33.23291073765553705 ) ) ;
#25907=CARTESIAN_POINT ( 'NONE',  ( -192.9588430854690273, -10.23066800229550388, 66.79921049721887982 ) ) ;
#25908=CARTESIAN_POINT ( 'NONE',  ( -162.0762913951020892, -1.198031840385767266, -1.198031840385758384 ) ) ;
#25909=CARTESIAN_POINT ( 'NONE',  ( -162.0762913951021176, 41.69427287672986182, 40.00000000000002132 ) ) ;
#25911=CARTESIAN_POINT ( 'NONE',  ( 192.4448373802101173, 14.14213562370320076, -42.42640687122072762 ) ) ;
#25912=EDGE_CURVE ( 'NONE', #25369, #19288, #21875, .T. ) ;
#25914=CARTESIAN_POINT ( 'NONE',  ( 23.46661716382972429, 23.32081713244427590, 42.82867125331105740 ) ) ;
#25915=CARTESIAN_POINT ( 'NONE',  ( -56.48582580120559982, -9.153146818113595984, 40.00000000000002132 ) ) ;
#25917=CARTESIAN_POINT ( 'NONE',  ( -188.3120147333417549, -46.99495896211615786, 13.82877842034796068 ) ) ;
#25919=CARTESIAN_POINT ( 'NONE',  ( -3.921555385250262482, -13.83441994316381241, 47.03297225793202330 ) ) ;
#25921=EDGE_CURVE ( 'NONE', #15233, #6802, #2995, .T. ) ;
#25923=CARTESIAN_POINT ( 'NONE',  ( 23.48902902575293794, 13.79248457098146119, -46.76665409567217324 ) ) ;
#25925=CARTESIAN_POINT ( 'NONE',  ( 110.0479209278586410, -22.74092928740055086, 9.419601331808566513 ) ) ;
#25927=CARTESIAN_POINT ( 'NONE',  ( -77.55640685876515761, -9.396736996787120630E-14, 22.13135000837099398 ) ) ;
#25928=( BOUNDED_SURFACE ( )  B_SPLINE_SURFACE ( 3, 3, ( 
 ( #15986, #13994, #16390, #22125, #16120, #164, #14131, #14395, #18516, #21991, #22260, #297, #8401, #1769, #3760, #19985, #9875, #12003, #10808, #14648, #25183, #10942, #16655, #832, #20789, #18918, #22787, #12662, #8941, #8538 ),
 ( #700, #4828, #14915, #2703, #21049, #4566, #22655, #12933, #2560, #6932, #16918, #6538, #25052, #4429, #20653, #8806, #2427, #4695, #6803, #10675, #18788, #15050, #569, #22916, #8674, #16783, #2833, #19050, #6407, #12797 ),
 ( #17047, #24919, #14524, #20924, #12522, #10537, #18649, #23056, #434, #24786, #14786, #6671, #12471, #10221, #1848, #109, #20469, #20598, #6489, #18328, #8216, #18060, #239, #22472, #2374, #4251, #24463, #8083, #16202, #24733 ),
 ( #20335, #16334, #14471, #14601, #3982, #8351, #6228, #14076, #4380, #12079, #24597, #14341, #10486, #22604, #18600, #24335, #378, #8483, #11947, #12341, #16600, #2244, #9951, #10351, #18461, #3843, #20072, #16472, #6352, #26211 ),
 ( #7947, #20201, #16065, #24192, #1980, #22340, #5965, #22207, #10086, #6099, #14206, #18190, #26341, #4116, #12213, #2112, #14735, #9139, #23001, #10756, #2911, #9024, #2508, #19259, #10892, #17128, #8621, #4778, #19129, #21263 ),
 ( #19004, #12882, #648, #17255, #11019, #22867, #20998, #2780, #10619, #18867, #16732, #516, #25259, #4644, #8754, #7010, #14867, #15131, #4905, #22731, #781, #8887, #25002, #18733, #16998, #7143, #11144, #25133, #13016, #20866 ),
 ( #23261, #12610, #24863, #6618, #4509, #2650, #1039, #6884, #5037, #911, #23133, #13144, #3035, #21136, #25391, #16870, #20739, #12746, #6755, #14998, #3540, #5282, #11640, #13268, #11264, #13641, #19383, #1421, #21767, #17505 ) ),
 .UNSPECIFIED., .T., .F., .F. ) 
 B_SPLINE_SURFACE_WITH_KNOTS ( ( 4, 3, 4 ),
 ( 4, 2, 2, 2, 2, 2, 2, 2, 2, 2, 2, 2, 2, 2, 4 ),
 ( 0.000000000000000000, 0.5000000000000000000, 1.000000000000000000 ),
 ( 0.000000000000000000, 0.1357259735107005372, 0.1651108541090157700, 0.1944957347073310028, 0.3598804999793158710, 0.3867117631979620773, 0.4135430264166082281, 0.5789277916885930964, 0.6062785021374117456, 0.6336292125862302838, 0.8508620842112317728, 0.8814014469398914198, 0.9119408096685510667, 0.9559704048342755334, 1.000000000000000000 ),
 .UNSPECIFIED. ) 
 GEOMETRIC_REPRESENTATION_ITEM ( )  RATIONAL_B_SPLINE_SURFACE ( (
 ( 1.000000000000000000, 1.000000000000000000, 1.000000000000000000, 1.000000000000000000, 1.000000000000000000, 1.000000000000000000, 1.000000000000000000, 1.000000000000000000, 1.000000000000000000, 1.000000000000000000, 1.000000000000000000, 1.000000000000000000, 1.000000000000000000, 1.000000000000000000, 1.000000000000000000, 1.000000000000000000, 1.000000000000000000, 1.000000000000000000, 1.000000000000000000, 1.000000000000000000, 1.000000000000000000, 1.000000000000000000, 1.000000000000000000, 1.000000000000000000, 1.000000000000000000, 1.000000000000000000, 1.000000000000000000, 1.000000000000000000, 1.000000000000000000, 1.000000000000000000),
 ( 0.3333333333333333703, 0.3333333333333333703, 0.3333333333333333703, 0.3333333333333333703, 0.3333333333333333703, 0.3333333333333333703, 0.3333333333333333703, 0.3333333333333333703, 0.3333333333333333703, 0.3333333333333333703, 0.3333333333333333703, 0.3333333333333333703, 0.3333333333333333703, 0.3333333333333333703, 0.3333333333333333703, 0.3333333333333333703, 0.3333333333333333703, 0.3333333333333333703, 0.3333333333333333703, 0.3333333333333333703, 0.3333333333333333703, 0.3333333333333333703, 0.3333333333333333703, 0.3333333333333333703, 0.3333333333333333703, 0.3333333333333333703, 0.3333333333333333703, 0.3333333333333333703, 0.3333333333333333703, 0.3333333333333333703),
 ( 0.3333333333333333703, 0.3333333333333333703, 0.3333333333333333703, 0.3333333333333333703, 0.3333333333333333703, 0.3333333333333333703, 0.3333333333333333703, 0.3333333333333333703, 0.3333333333333333703, 0.3333333333333333703, 0.3333333333333333703, 0.3333333333333333703, 0.3333333333333333703, 0.3333333333333333703, 0.3333333333333333703, 0.3333333333333333703, 0.3333333333333333703, 0.3333333333333333703, 0.3333333333333333703, 0.3333333333333333703, 0.3333333333333333703, 0.3333333333333333703, 0.3333333333333333703, 0.3333333333333333703, 0.3333333333333333703, 0.3333333333333333703, 0.3333333333333333703, 0.3333333333333333703, 0.3333333333333333703, 0.3333333333333333703),
 ( 1.000000000000000000, 1.000000000000000000, 1.000000000000000000, 1.000000000000000000, 1.000000000000000000, 1.000000000000000000, 1.000000000000000000, 1.000000000000000000, 1.000000000000000000, 1.000000000000000000, 1.000000000000000000, 1.000000000000000000, 1.000000000000000000, 1.000000000000000000, 1.000000000000000000, 1.000000000000000000, 1.000000000000000000, 1.000000000000000000, 1.000000000000000000, 1.000000000000000000, 1.000000000000000000, 1.000000000000000000, 1.000000000000000000, 1.000000000000000000, 1.000000000000000000, 1.000000000000000000, 1.000000000000000000, 1.000000000000000000, 1.000000000000000000, 1.000000000000000000),
 ( 0.3333333333333333703, 0.3333333333333333703, 0.3333333333333333703, 0.3333333333333333703, 0.3333333333333333703, 0.3333333333333333703, 0.3333333333333333703, 0.3333333333333333703, 0.3333333333333333703, 0.3333333333333333703, 0.3333333333333333703, 0.3333333333333333703, 0.3333333333333333703, 0.3333333333333333703, 0.3333333333333333703, 0.3333333333333333703, 0.3333333333333333703, 0.3333333333333333703, 0.3333333333333333703, 0.3333333333333333703, 0.3333333333333333703, 0.3333333333333333703, 0.3333333333333333703, 0.3333333333333333703, 0.3333333333333333703, 0.3333333333333333703, 0.3333333333333333703, 0.3333333333333333703, 0.3333333333333333703, 0.3333333333333333703),
 ( 0.3333333333333333703, 0.3333333333333333703, 0.3333333333333333703, 0.3333333333333333703, 0.3333333333333333703, 0.3333333333333333703, 0.3333333333333333703, 0.3333333333333333703, 0.3333333333333333703, 0.3333333333333333703, 0.3333333333333333703, 0.3333333333333333703, 0.3333333333333333703, 0.3333333333333333703, 0.3333333333333333703, 0.3333333333333333703, 0.3333333333333333703, 0.3333333333333333703, 0.3333333333333333703, 0.3333333333333333703, 0.3333333333333333703, 0.3333333333333333703, 0.3333333333333333703, 0.3333333333333333703, 0.3333333333333333703, 0.3333333333333333703, 0.3333333333333333703, 0.3333333333333333703, 0.3333333333333333703, 0.3333333333333333703),
 ( 1.000000000000000000, 1.000000000000000000, 1.000000000000000000, 1.000000000000000000, 1.000000000000000000, 1.000000000000000000, 1.000000000000000000, 1.000000000000000000, 1.000000000000000000, 1.000000000000000000, 1.000000000000000000, 1.000000000000000000, 1.000000000000000000, 1.000000000000000000, 1.000000000000000000, 1.000000000000000000, 1.000000000000000000, 1.000000000000000000, 1.000000000000000000, 1.000000000000000000, 1.000000000000000000, 1.000000000000000000, 1.000000000000000000, 1.000000000000000000, 1.000000000000000000, 1.000000000000000000, 1.000000000000000000, 1.000000000000000000, 1.000000000000000000, 1.000000000000000000) ) ) 
 REPRESENTATION_ITEM ( '' )  SURFACE ( )  );
#25929=CARTESIAN_POINT ( 'NONE',  ( 184.8905102610680444, 41.77492675555983936, 14.79361573936436081 ) ) ;
#25930=CARTESIAN_POINT ( 'NONE',  ( 170.2234770963711128, -15.44714144992813409, 40.00000000000002132 ) ) ;
#25931=CARTESIAN_POINT ( 'NONE',  ( 60.14720761606899657, -10.94158980359358324, -33.22245024492937659 ) ) ;
#25934=CARTESIAN_POINT ( 'NONE',  ( -259.2033419157646676, 9.517827891722582478, -40.00000000000002132 ) ) ;
#25935=CARTESIAN_POINT ( 'NONE',  ( 170.2234770963711128, -24.55285855007184281, 40.00000000000002132 ) ) ;
#25936=CARTESIAN_POINT ( 'NONE',  ( -100.7734535825088500, -39.99999999999986500, -17.32597176626853397 ) ) ;
#25937=CARTESIAN_POINT ( 'NONE',  ( 184.8905102610680444, -1.851754852062639767E-13, 20.92133201514444352 ) ) ;
#25938=CARTESIAN_POINT ( 'NONE',  ( 4.995406935893287326, 17.50105314357225694, -39.06748935135176026 ) ) ;
#25941=CARTESIAN_POINT ( 'NONE',  ( -198.0356074513804572, -15.37879056873074290, 0.000000000000000000 ) ) ;
#25944=CARTESIAN_POINT ( 'NONE',  ( -188.7701069479164460, 47.15820909662599547, -13.85300054332491371 ) ) ;
#25947=EDGE_LOOP ( 'NONE', ( #5947, #10837, #24244, #6833 ) ) ;
#25948=CARTESIAN_POINT ( 'NONE',  ( 19.06497207195982924, -66.60410523465823474, 10.03556273973400081 ) ) ;
#25949=CARTESIAN_POINT ( 'NONE',  ( 23.10188454848715978, -42.94013537404167380, -23.40120037234288475 ) ) ;
#25950=ORIENTED_EDGE ( 'NONE', *, *, #1426, .F. ) ;
#25951=CARTESIAN_POINT ( 'NONE',  ( -162.0762913951020892, 41.69427287692678163, -40.00000000000002132 ) ) ;
#25955=CARTESIAN_POINT ( 'NONE',  ( -175.9234121941017293, 21.03678982652580487, -39.35887396262683069 ) ) ;
#25956=CARTESIAN_POINT ( 'NONE',  ( 14.38125909742181108, 39.01709431150907648, 39.01709431150921858 ) ) ;
#25958=CARTESIAN_POINT ( 'NONE',  ( 163.1118516004056573, 1.251511021549353291E-13, -27.26290988616872824 ) ) ;
#25959=CARTESIAN_POINT ( 'NONE',  ( 0.2972598230769930572, 14.33493731733933352, 0.000000000000000000 ) ) ;
#25962=B_SPLINE_CURVE_WITH_KNOTS ( 'NONE', 3,
 ( #25218, #22825, #23347, #24961, #15217, #16954 ),
 .UNSPECIFIED., .F., .F.,
 ( 4, 2, 4 ),
 ( 1.440969542111313559E-17, 0.03937685683732346925, 0.07875371367464692463 ),
 .UNSPECIFIED. ) ;
#25965=CARTESIAN_POINT ( 'NONE',  ( 199.9999999999999432, -1.727494763561684666E-13, 20.00000000000010303 ) ) ;
#25966=CARTESIAN_POINT ( 'NONE',  ( 0.2972598230770030492, -39.99999999999987210, -14.33493731733975451 ) ) ;
#25967=CARTESIAN_POINT ( 'NONE',  ( -114.7538884075548964, -13.57382480623414445, 17.50182194317655160 ) ) ;
#25968=CARTESIAN_POINT ( 'NONE',  ( 170.2234770963711128, -39.20704971665379190, -17.36149277827012938 ) ) ;
#25969=CARTESIAN_POINT ( 'NONE',  ( -213.1075012329537230, -13.71589010951915810, 0.000000000000000000 ) ) ;
#25970=CARTESIAN_POINT ( 'NONE',  ( 91.82158438592159655, -44.40256751092324095, -12.16597498400075139 ) ) ;
#25972=DIRECTION ( 'NONE',  ( -0.01051738777839801575, 0.9307051272556606802, -0.3656191333263937304 ) ) ;
#25973=CARTESIAN_POINT ( 'NONE',  ( 165.3321726438165626, 18.76308274333374371, 18.76308274333403503 ) ) ;
#25974=CARTESIAN_POINT ( 'NONE',  ( 146.6084372240433993, 1.478241399363601114E-13, -34.62501878078305850 ) ) ;
#25975=CARTESIAN_POINT ( 'NONE',  ( -259.2033419157646676, 21.55415060305830366, 21.55415060305842800 ) ) ;
#25976=CARTESIAN_POINT ( 'NONE',  ( 19.06497207195981858, -38.31983398719641087, 18.24870850772724040 ) ) ;
#25977=CARTESIAN_POINT ( 'NONE',  ( -188.3509229510629552, -17.87648076835369437, -43.15764231844840282 ) ) ;
#25978=CARTESIAN_POINT ( 'NONE',  ( -30.26275506840324070, -29.48230279907780016, -27.08623969584605362 ) ) ;
#25980=CARTESIAN_POINT ( 'NONE',  ( -105.3755690713226585, -15.38646221621738164, -41.18208027870615240 ) ) ;
#25981=CARTESIAN_POINT ( 'NONE',  ( -135.8532207217289738, 6.472252184284186249, -6.472252184284142729 ) ) ;
#25984=CARTESIAN_POINT ( 'NONE',  ( -91.56559293963834989, -44.31723036834885932, -12.25131212657538171 ) ) ;
#25985=( LENGTH_UNIT ( ) NAMED_UNIT ( * ) SI_UNIT ( .MILLI., .METRE. ) );
#25986=CARTESIAN_POINT ( 'NONE',  ( -82.24889283716245814, 3.157952835618418330, 19.94440861093309181 ) ) ;
#25990=CARTESIAN_POINT ( 'NONE',  ( -105.2054292635176296, -15.67883240738871287, 14.71716402001586665 ) ) ;
#25991=CARTESIAN_POINT ( 'NONE',  ( -3.494657986429658969, 17.93150516116838844, 43.29048295385586442 ) ) ;
#25995=CARTESIAN_POINT ( 'NONE',  ( 163.1118516004056573, 12.73709011382478806, -40.00000000000002132 ) ) ;
#25996=CARTESIAN_POINT ( 'NONE',  ( 184.8905102610680444, 14.79361573936396113, -14.79361573936377461 ) ) ;
#25997=CARTESIAN_POINT ( 'NONE',  ( 0.2972598230769956662, 39.99999999999983658, 54.33493731733950938 ) ) ;
#25998=CARTESIAN_POINT ( 'NONE',  ( 23.37394308801977161, 13.80096434448334186, -46.80823611210181667 ) ) ;
#25999=EDGE_CURVE ( 'NONE', #13223, #5232, #14677, .T. ) ;
#26001=CARTESIAN_POINT ( 'NONE',  ( -162.0762913951020892, -1.202636532414034422E-14, -1.694272876828323948 ) ) ;
#26002=CARTESIAN_POINT ( 'NONE',  ( 98.29820294267527458, 2.689882573189819553E-13, -20.00000000000500222 ) ) ;
#26005=CARTESIAN_POINT ( 'NONE',  ( -129.2303492455655771, 11.67678589714761017, 24.84170067272852833 ) ) ;
#26006=CARTESIAN_POINT ( 'NONE',  ( -4.027137536849729749, -23.45200847982304992, -43.00884733904526058 ) ) ;
#26007=CARTESIAN_POINT ( 'NONE',  ( -105.3755690713226585, -41.18208027870611687, 15.38646221621750954 ) ) ;
#26008=CARTESIAN_POINT ( 'NONE',  ( 130.8568914410475372, -24.07718906447255947, 24.07718906447199458 ) ) ;
#26009=CARTESIAN_POINT ( 'NONE',  ( -105.3755690713226585, -41.18208027870589660, -15.38646221621809040 ) ) ;
#26010=CARTESIAN_POINT ( 'NONE',  ( 19.06497207195981858, -39.99999999999987210, -14.19242893257882621 ) ) ;
#26013=CARTESIAN_POINT ( 'NONE',  ( 199.9999999999999432, -19.99999999999988987, -2.449293598294708485E-15 ) ) ;
#26014=CARTESIAN_POINT ( 'NONE',  ( 151.7948205124836534, 23.49921654116009506, 33.06932595376371609 ) ) ;
#26015=CARTESIAN_POINT ( 'NONE',  ( 57.59792236341148453, -37.56421063658185489, 40.00000000000002132 ) ) ;
#26016=CARTESIAN_POINT ( 'NONE',  ( -105.2334157265395618, 2.725992507770012452, 21.31091308246880089 ) ) ;
#26017=CARTESIAN_POINT ( 'NONE',  ( -238.4067589809705794, 39.99999999999999289, -0.9644942799821634161 ) ) ;
#26018=CARTESIAN_POINT ( 'NONE',  ( -238.4067589809705794, 28.96627169325315165, 28.96627169325329731 ) ) ;
#26019=CARTESIAN_POINT ( 'NONE',  ( 57.59792236341147031, -2.435789363418150000, -40.00000000000002132 ) ) ;
#26020=ORIENTED_EDGE ( 'NONE', *, *, #10770, .F. ) ;
#26021=CARTESIAN_POINT ( 'NONE',  ( 67.67011021022788952, -29.29769665550713498, 12.13550330104319208 ) ) ;
#26023=CARTESIAN_POINT ( 'NONE',  ( -28.75791583366072146, -12.03523584680483083, 38.33181286256369447 ) ) ;
#26024=CARTESIAN_POINT ( 'NONE',  ( 192.4448373802101173, 14.14213562370320076, -42.42640687122072762 ) ) ;
#26025=CARTESIAN_POINT ( 'NONE',  ( -162.0762913951021176, -40.00000000000019895, 41.69427287672974813 ) ) ;
#26026=CARTESIAN_POINT ( 'NONE',  ( 199.9999999999999432, -14.14213562373115884, 14.14213562373085153 ) ) ;
#26027=CARTESIAN_POINT ( 'NONE',  ( 14.38125909742180752, 15.17850393972634038, 0.000000000000000000 ) ) ;
#26028=CARTESIAN_POINT ( 'NONE',  ( 163.1118516004056573, -27.26290988616869626, -40.00000000000002132 ) ) ;
#26032=CARTESIAN_POINT ( 'NONE',  ( -135.8532207217289738, 21.81201906317798134, -21.81201906317747685 ) ) ;
#26033=CARTESIAN_POINT ( 'NONE',  ( 14.38125909742181996, -10.73282306405815234, -67.30136555898266693 ) ) ;
#26034=CARTESIAN_POINT ( 'NONE',  ( -196.0240701931629417, -14.12332411430281631, 48.96019555158520831 ) ) ;
#26036=CARTESIAN_POINT ( 'NONE',  ( -105.3755690713226727, -12.89780903124395550, -12.89780903124416511 ) ) ;
#26037=CARTESIAN_POINT ( 'NONE',  ( 19.06497207195982568, -38.31983398719592770, -38.31983398719660272 ) ) ;
#26039=CARTESIAN_POINT ( 'NONE',  ( 163.1118516004056573, -47.56205970284945295, -9.006482792074823607 ) ) ;
#26040=CARTESIAN_POINT ( 'NONE',  ( -105.4288953903231629, -9.009229104196512239, 19.35825399501247546 ) ) ;
#26043=CARTESIAN_POINT ( 'NONE',  ( 146.6084372240433709, -39.99999999999987921, -34.62501878078319351 ) ) ;
#26044=CARTESIAN_POINT ( 'NONE',  ( 136.1360204305621551, 24.77266263493108411, 31.79587985999273769 ) ) ;
#26046=CARTESIAN_POINT ( 'NONE',  ( -30.26275506840324425, 41.69427246844627177, 40.00000000000002132 ) ) ;
#26048=CARTESIAN_POINT ( 'NONE',  ( -105.3755690713226585, 12.89780903124410472, -43.67073346367977393 ) ) ;
#26049=CARTESIAN_POINT ( 'NONE',  ( 96.51883974015090928, 19.13300947096759685, 7.925152011866398283 ) ) ;
#26051=CARTESIAN_POINT ( 'NONE',  ( 98.29820294267403824, -19.87244099730552094, -2.605266741664709507 ) ) ;
#26053=CARTESIAN_POINT ( 'NONE',  ( -197.4154352059224493, -49.11380478891992141, 14.14666496776951377 ) ) ;
#26055=CARTESIAN_POINT ( 'NONE',  ( 17.49521241104683966, -18.35049639064382276, 44.30201726249271843 ) ) ;
#26056=CARTESIAN_POINT ( 'NONE',  ( 23.39921416754926753, 23.33452606844902988, -42.84940400815654726 ) ) ;
#26059=FACE_OUTER_BOUND ( 'NONE', #11463, .T. ) ;
#26060=EDGE_CURVE ( 'NONE', #4428, #21267, #8647, .T. ) ;
#26061=CARTESIAN_POINT ( 'NONE',  ( -105.3755690713226585, -15.38646221621738164, -41.18208027870615240 ) ) ;
#26062=CARTESIAN_POINT ( 'NONE',  ( -280.0000000000000568, 19.99999999999996092, 40.00000000000002132 ) ) ;
#26063=CARTESIAN_POINT ( 'NONE',  ( 44.46627453556679654, -15.24062802624899504, -36.79413088011303046 ) ) ;
#26064=CARTESIAN_POINT ( 'NONE',  ( -259.2033419157646676, -9.517827891722680178, 0.000000000000000000 ) ) ;
#26066=CARTESIAN_POINT ( 'NONE',  ( 91.82158438592158234, 17.20528682183301683, 0.000000000000000000 ) ) ;
#26067=CARTESIAN_POINT ( 'NONE',  ( -100.7734535825088500, 22.67402823373189591, -0.000000000000000000 ) ) ;
#26068=CARTESIAN_POINT ( 'NONE',  ( 192.4448373802101173, -20.00000000003938538, 40.00000000000002132 ) ) ;
#26069=CARTESIAN_POINT ( 'NONE',  ( -56.48582580120558561, 3.151766524733697544E-13, -30.84685318188644132 ) ) ;
#26071=CARTESIAN_POINT ( 'NONE',  ( -56.48582580120559271, 6.472252184284121412, 6.472252184284244869 ) ) ;
#26073=EDGE_CURVE ( 'NONE', #7090, #16387, #24196, .T. ) ;
#26074=VERTEX_POINT ( 'NONE', #15666 ) ;
#26075=CARTESIAN_POINT ( 'NONE',  ( -65.65550967526021964, -24.89650881518424796, 9.107276986624334825 ) ) ;
#26076=CARTESIAN_POINT ( 'NONE',  ( 163.1118516004056573, 27.26290988616876021, 40.00000000000002132 ) ) ;
#26077=CARTESIAN_POINT ( 'NONE',  ( -77.90255099906863734, -20.04994828524331396, -8.644468104250957907 ) ) ;
#26079=ORIENTED_EDGE ( 'NONE', *, *, #25887, .T. ) ;
#26082=CARTESIAN_POINT ( 'NONE',  ( -56.48582580120558561, -50.09629031063963112, -6.472252184284449150 ) ) ;
#26083=CARTESIAN_POINT ( 'NONE',  ( 23.72853009152626669, -42.74808902029896984, -23.26754081577798416 ) ) ;
#26084=ORIENTED_EDGE ( 'NONE', *, *, #13844, .T. ) ;
#26085=CARTESIAN_POINT ( 'NONE',  ( -238.4067589809705794, 0.9644942799825385604, -40.00000000000002132 ) ) ;
#26086=CARTESIAN_POINT ( 'NONE',  ( -97.73806390046078718, -20.71810467719840076, 8.581719943915564031 ) ) ;
#26090=CARTESIAN_POINT ( 'NONE',  ( -208.1127848780264742, 38.89260858015732936, -17.67593391476642140 ) ) ;
#26091=CARTESIAN_POINT ( 'NONE',  ( -129.2303573022218472, -25.82247248374897453, -9.309001178860381032 ) ) ;
#26092=( BOUNDED_SURFACE ( )  B_SPLINE_SURFACE ( 3, 2, ( 
 ( #13281, #3176, #1054 ),
 ( #23647, #9289, #21528 ),
 ( #15018, #15146, #23148 ),
 ( #25277, #19144, #928 ),
 ( #17272, #9038, #9414 ),
 ( #7027, #23276, #9159 ),
 ( #3303, #17521, #7157 ),
 ( #11281, #15910, #15648 ),
 ( #13923, #11658, #3970 ),
 ( #7935, #6086, #3692 ),
 ( #19918, #12067, #8069 ),
 ( #22193, #7664, #10074 ),
 ( #11798, #19782, #25923 ),
 ( #26198, #18179, #23904 ),
 ( #26056, #1568, #13659 ),
 ( #18045, #1836, #7794 ),
 ( #1702, #9937, #5820 ),
 ( #14062, #16053, #14193 ),
 ( #1969, #4100, #24178 ),
 ( #25786, #21782, #3555 ),
 ( #26328, #15775, #24042 ),
 ( #22325, #20185, #16188 ),
 ( #17913, #9673, #22058 ),
 ( #5680, #12201, #24321 ),
 ( #17777, #20322, #5550 ),
 ( #13785, #3831, #5953 ),
 ( #21920, #9536, #9809 ),
 ( #11932, #20059, #17645 ),
 ( #7536, #23773, #24718 ),
 ( #2359, #8467, #16321 ),
 ( #14459, #16856, #4627 ),
 ( #4492, #8203, #6214 ),
 ( #12594, #24987, #22715 ),
 ( #4367, #4762, #16586 ),
 ( #10338, #14326, #18852 ),
 ( #10472, #24448, #12730 ),
 ( #95, #22458, #6738 ),
 ( #20724, #8607, #223 ),
 ( #364, #16459, #24848 ),
 ( #14850, #24581, #16716 ),
 ( #12328, #2632, #18447 ),
 ( #8337, #22590, #22986 ),
 ( #12866, #18313, #6473 ),
 ( #6337, #4238, #8738 ),
 ( #6600, #20456, #2099 ),
 ( #2230, #14587, #12457 ),
 ( #632, #20584, #18587 ),
 ( #20852, #10208, #2492 ),
 ( #10603, #18715, #500 ),
 ( #14720, #22852, #10741 ),
 ( #766, #11371, #25378 ),
 ( #7253, #8872, #17490 ),
 ( #15372, #6870, #23373 ),
 ( #19492, #9383, #25632 ),
 ( #19114, #21502, #23495 ),
 ( #23118, #11004, #14984 ),
 ( #3273, #9007, #18988 ),
 ( #13000, #25118, #9260 ),
 ( #13254, #19243, #21377 ),
 ( #3147, #17240, #17114 ) ),
 .UNSPECIFIED., .F., .F., .F. ) 
 B_SPLINE_SURFACE_WITH_KNOTS ( ( 4, 2, 2, 2, 2, 2, 2, 2, 2, 2, 2, 2, 2, 2, 2, 2, 2, 2, 2, 2, 2, 2, 2, 2, 2, 2, 2, 2, 2, 4 ),
 ( 3, 3 ),
 ( -6.934549977324636831E-05, 0.02465257023823466329, 0.04937448597624257557, 0.07409640171425048438, 0.08027688064875246332, 0.08066316058215883267, 0.08085630054886201734, 0.08090458554053781004, 0.08095287053221361662, 0.08104944051556520201, 0.08182200038237795459, 0.08336712011600344585, 0.08645735958325444226, 0.09263783851775642120, 0.09881831745225840014, 0.1019085569195093965, 0.1049987963867603791, 0.1111792753212623441, 0.1173597542557643231, 0.1177460341891707063, 0.1179391741558738910, 0.1179874591475496837, 0.1180357441392254902, 0.1181323141225770756, 0.1189048739893898143, 0.1204499937230153195, 0.1235402331902663020, 0.1482621489282742178, 0.1729840646662821335, 0.1977059804042900493 ),
 ( 0.000000000000000000, 1.000000000000000000 ),
 .UNSPECIFIED. ) 
 GEOMETRIC_REPRESENTATION_ITEM ( )  RATIONAL_B_SPLINE_SURFACE ( (
 ( 1.000000000000000000, 1.000000000000000000, 1.000000000000000000),
 ( 1.000000000000000000, 0.9999975583951711267, 1.000000000000000000),
 ( 1.000000000000000000, 0.9982436956960244467, 1.000000000000000000),
 ( 1.000000000000000000, 0.9910288481552836926, 1.000000000000000000),
 ( 1.000000000000000000, 0.9855714588515669394, 1.000000000000000000),
 ( 1.000000000000000000, 0.9705958323316277170, 1.000000000000000000),
 ( 1.000000000000000000, 0.9610788543728805422, 1.000000000000000000),
 ( 1.000000000000000000, 0.9462867046313790942, 1.000000000000000000),
 ( 1.000000000000000000, 0.9431828180754202595, 1.000000000000000000),
 ( 1.000000000000000000, 0.9397240291170393389, 1.000000000000000000),
 ( 1.000000000000000000, 0.9395199791395948408, 1.000000000000000000),
 ( 1.000000000000000000, 0.9392130141387217135, 1.000000000000000000),
 ( 1.000000000000000000, 0.9391105441325077186, 1.000000000000000000),
 ( 1.000000000000000000, 0.9389822709566318926, 1.000000000000000000),
 ( 1.000000000000000000, 0.9389566070380594986, 1.000000000000000000),
 ( 1.000000000000000000, 0.9389052606279759683, 1.000000000000000000),
 ( 1.000000000000000000, 0.9388799835492042112, 1.000000000000000000),
 ( 1.000000000000000000, 0.9388039637710107188, 1.000000000000000000),
 ( 1.000000000000000000, 0.9387533729070498545, 1.000000000000000000),
 ( 1.000000000000000000, 0.9382988607466662412, 1.000000000000000000),
 ( 1.000000000000000000, 0.9379005790853373048, 1.000000000000000000),
 ( 1.000000000000000000, 0.9367237203701870296, 1.000000000000000000),
 ( 1.000000000000000000, 0.9359625442025352182, 1.000000000000000000),
 ( 1.000000000000000000, 0.9337619511410462092, 1.000000000000000000),
 ( 1.000000000000000000, 0.9324064515426850885, 1.000000000000000000),
 ( 1.000000000000000000, 0.9287106072119778455, 1.000000000000000000),
 ( 1.000000000000000000, 0.9267422912949104807, 1.000000000000000000),
 ( 1.000000000000000000, 0.9239539123017169731, 1.000000000000000000),
 ( 1.000000000000000000, 0.9231338493907679243, 1.000000000000000000),
 ( 1.000000000000000000, 0.9228496048507219829, 1.000000000000000000),
 ( 1.000000000000000000, 0.9229135694614544194, 1.000000000000000000),
 ( 1.000000000000000000, 0.9233494155302709450, 1.000000000000000000),
 ( 1.000000000000000000, 0.9237209353787055877, 1.000000000000000000),
 ( 1.000000000000000000, 0.9252744993866384160, 1.000000000000000000),
 ( 1.000000000000000000, 0.9268968421606754715, 1.000000000000000000),
 ( 1.000000000000000000, 0.9311673748451266830, 1.000000000000000000),
 ( 1.000000000000000000, 0.9338157035271601458, 1.000000000000000000),
 ( 1.000000000000000000, 0.9370733336298897598, 1.000000000000000000),
 ( 1.000000000000000000, 0.9372665829346482624, 1.000000000000000000),
 ( 1.000000000000000000, 0.9375588533504889410, 1.000000000000000000),
 ( 1.000000000000000000, 0.9376566762263730537, 1.000000000000000000),
 ( 1.000000000000000000, 0.9377794499114625593, 1.000000000000000000),
 ( 1.000000000000000000, 0.9378038842964711019, 1.000000000000000000),
 ( 1.000000000000000000, 0.9378536652368905102, 1.000000000000000000),
 ( 1.000000000000000000, 0.9378785472098797316, 1.000000000000000000),
 ( 1.000000000000000000, 0.9379531676447510069, 1.000000000000000000),
 ( 1.000000000000000000, 0.9380028806225376714, 1.000000000000000000),
 ( 1.000000000000000000, 0.9384499917948705416, 1.000000000000000000),
 ( 1.000000000000000000, 0.9388452506063379444, 1.000000000000000000),
 ( 1.000000000000000000, 0.9400245377241723821, 1.000000000000000000),
 ( 1.000000000000000000, 0.9408020798629984638, 1.000000000000000000),
 ( 1.000000000000000000, 0.9431089717073131151, 1.000000000000000000),
 ( 1.000000000000000000, 0.9446123105951671484, 1.000000000000000000),
 ( 1.000000000000000000, 0.9578370004747042143, 1.000000000000000000),
 ( 1.000000000000000000, 0.9674308273343070752, 1.000000000000000000),
 ( 1.000000000000000000, 0.9828254127557658482, 1.000000000000000000),
 ( 1.000000000000000000, 0.9886239107116221447, 1.000000000000000000),
 ( 1.000000000000000000, 0.9967564037645806341, 1.000000000000000000),
 ( 1.000000000000000000, 0.9990872413561198151, 1.000000000000000000),
 ( 1.000000000000000000, 0.9997813423572990965, 1.000000000000000000) ) ) 
 REPRESENTATION_ITEM ( '' )  SURFACE ( )  );
#26093=CARTESIAN_POINT ( 'NONE',  ( 91.82158438592159655, -39.99999999999994316, -17.20528682183314118 ) ) ;
#26094=CARTESIAN_POINT ( 'NONE',  ( -135.8532207217289738, 30.84685318188643421, 40.00000000000002132 ) ) ;
#26097=CARTESIAN_POINT ( 'NONE',  ( -86.96347745069643054, -39.99999999999995737, -21.75974354311664527 ) ) ;
#26098=CARTESIAN_POINT ( 'NONE',  ( -56.48582580120557850, -39.99999999999970868, -30.84685318188687120 ) ) ;
#26099=CARTESIAN_POINT ( 'NONE',  ( 170.0000000000000000, 1.183443619805854272E-13, -24.95097643317000546 ) ) ;
#26100=CARTESIAN_POINT ( 'NONE',  ( -162.0762913951020607, -1.198031840455708430, 57.76657433537920383 ) ) ;
#26101=CARTESIAN_POINT ( 'NONE',  ( -135.8532207217289738, 9.153146818113546246, -0.000000000000000000 ) ) ;
#26102=CARTESIAN_POINT ( 'NONE',  ( -238.4067589809705794, -28.96627169325343942, 28.96627169325309126 ) ) ;
#26104=CARTESIAN_POINT ( 'NONE',  ( 12.01676479903286676, -49.30523874212533286, 14.17570730777206833 ) ) ;
#26105=CARTESIAN_POINT ( 'NONE',  ( 98.29820294273055481, 14.14213562373424971, 14.14213562373465294 ) ) ;
#26106=CARTESIAN_POINT ( 'NONE',  ( 163.1118516004056573, 1.251511021549353291E-13, -27.26290988616872824 ) ) ;
#26107=CARTESIAN_POINT ( 'NONE',  ( -100.7734535825088500, 12.25131212657490209, -44.31723036834897300 ) ) ;
#26108=CARTESIAN_POINT ( 'NONE',  ( 199.9999999999999432, 14.14213562373093680, 14.14213562373114641 ) ) ;
#26109=CARTESIAN_POINT ( 'NONE',  ( -188.4265466358192214, -13.83489705870103137, -47.03621809928373665 ) ) ;
#26111=EDGE_LOOP ( 'NONE', ( #17305, #21850, #8532, #9901 ) ) ;
#26112=CARTESIAN_POINT ( 'NONE',  ( 57.59792236341147031, -30.00663442387662627, -26.56190807104723461 ) ) ;
#26113=CARTESIAN_POINT ( 'NONE',  ( 136.1360204305621266, 53.05693388239316022, 3.511608612530967566 ) ) ;
#26114=CARTESIAN_POINT ( 'NONE',  ( -198.0356074513804572, -15.37879056873074290, 0.000000000000000000 ) ) ;
#26116=CARTESIAN_POINT ( 'NONE',  ( -86.96347745069644475, -43.67073346367964604, -12.89780903124457545 ) ) ;
#26117=CARTESIAN_POINT ( 'NONE',  ( -197.4153392274985492, -24.72549520219616781, -44.73189834453274472 ) ) ;
#26118=ORIENTED_EDGE ( 'NONE', *, *, #21119, .T. ) ;
#26121=CARTESIAN_POINT ( 'NONE',  ( -4.082462733456094561, 13.82507958736525921, 46.97557262069152273 ) ) ;
#26123=ORIENTED_EDGE ( 'NONE', *, *, #22018, .F. ) ;
#26124=CARTESIAN_POINT ( 'NONE',  ( -105.3755690713226727, -21.75974354311652093, 0.000000000000000000 ) ) ;
#26126=CARTESIAN_POINT ( 'NONE',  ( -114.4364955367317549, 8.064892380853404319, 20.29001642038314657 ) ) ;
#26127=CARTESIAN_POINT ( 'NONE',  ( 73.43468571101038833, 9.843145813772503416, -28.18272067128102520 ) ) ;
#26130=CARTESIAN_POINT ( 'NONE',  ( -198.0356074513804572, 1.247057299367198800E-13, -15.37879056873070560 ) ) ;
#26131=CARTESIAN_POINT ( 'NONE',  ( -280.0000000000000000, -2.609240458947769655E-13, 20.00000000000001421 ) ) ;
#26133=DIRECTION ( 'NONE',  ( 1.000000000000000000, 0.000000000000000000, 0.000000000000000000 ) ) ;
#26135=CARTESIAN_POINT ( 'NONE',  ( -151.4802849341772628, 16.17241510384845782, 31.86309571750582137 ) ) ;
#26136=CARTESIAN_POINT ( 'NONE',  ( 8.209392600897984948, -14.17653494425323224, -49.31072049265799961 ) ) ;
#26137=CARTESIAN_POINT ( 'NONE',  ( 163.1118516004056573, -9.006482792069506971, -9.006482792069697041 ) ) ;
#26138=CARTESIAN_POINT ( 'NONE',  ( -110.1017833366333463, 1.261429655903683500, -20.19517362625915524 ) ) ;
#26139=CARTESIAN_POINT ( 'NONE',  ( 91.82158438592159655, -44.40256751092324095, -12.16597498400075139 ) ) ;
#26140=CARTESIAN_POINT ( 'NONE',  ( 136.1360204305621266, -3.419521671106983309E-13, 35.03383547441296741 ) ) ;
#26141=CARTESIAN_POINT ( 'NONE',  ( -162.0762913951020892, -1.198031840385767266, -1.198031840385758384 ) ) ;
#26142=CARTESIAN_POINT ( 'NONE',  ( 19.06497207195982924, -54.19242893257843008, 40.00000000000002132 ) ) ;
#26143=CARTESIAN_POINT ( 'NONE',  ( 107.5473083967384298, 16.96446921415044784, -16.96446921415024889 ) ) ;
#26144=B_SPLINE_CURVE_WITH_KNOTS ( 'NONE', 3,
 ( #20121, #24381, #2035, #21986, #1899, #10004, #25990, #19981 ),
 .UNSPECIFIED., .F., .F.,
 ( 4, 2, 2, 4 ),
 ( 0.0002282271114689535154, 0.004312393619941001614, 0.006354476874177026301, 0.008396560128413051854 ),
 .UNSPECIFIED. ) ;
#26145=CARTESIAN_POINT ( 'NONE',  ( 4.995406935893307754, -55.24977328854835434, -2.449293598294708485E-15 ) ) ;
#26146=CARTESIAN_POINT ( 'NONE',  ( -114.7469097549961674, 17.41872337029852602, 13.60512637059788155 ) ) ;
#26147=EDGE_CURVE ( 'NONE', #10974, #16948, #2631, .T. ) ;
#26148=CARTESIAN_POINT ( 'NONE',  ( 14.38125909742180930, 40.00000000000060396, -55.17850393974224232 ) ) ;
#26149=CARTESIAN_POINT ( 'NONE',  ( -192.9588430854689989, 10.23066800230742679, 10.23066800230749607 ) ) ;
#26150=CARTESIAN_POINT ( 'NONE',  ( 163.1118516004056573, 12.73709011382478806, -40.00000000000002132 ) ) ;
#26152=CARTESIAN_POINT ( 'NONE',  ( 23.40652632868000538, -46.79646383233843920, 13.79856377312506055 ) ) ;
#26154=CARTESIAN_POINT ( 'NONE',  ( 141.7948666911896112, 12.58737617328871572, 30.38861427224642853 ) ) ;
#26155=CARTESIAN_POINT ( 'NONE',  ( 0.2972598230769886718, 38.42060263243669027, -18.14793986248710667 ) ) ;
#26157=CARTESIAN_POINT ( 'NONE',  ( 19.06497207195982924, -40.00000000000021316, 54.19242893257830218 ) ) ;
#26158=AXIS2_PLACEMENT_3D ( 'NONE', #15252, #13261, #17498 ) ;
#26159=CARTESIAN_POINT ( 'NONE',  ( -280.0000000000000568, 14.14213562373038968, 42.42640687119305198 ) ) ;
#26160=CARTESIAN_POINT ( 'NONE',  ( -86.96347745069644475, -21.75974354311651737, 0.000000000000000000 ) ) ;
#26162=CARTESIAN_POINT ( 'NONE',  ( -56.48582580120559271, -9.153146818113595984, 0.000000000000000000 ) ) ;
#26167=CARTESIAN_POINT ( 'NONE',  ( 146.6084372240433709, 32.08495691632030145, 24.48358557860365181 ) ) ;
#26168=CARTESIAN_POINT ( 'NONE',  ( -135.8532207217289738, -50.09629031063973770, 6.472252184283735943 ) ) ;
#26169=CARTESIAN_POINT ( 'NONE',  ( 146.6084372240433993, 24.48358557860341733, -24.48358557860313311 ) ) ;
#26170=CARTESIAN_POINT ( 'NONE',  ( -82.27051431265631720, 17.53273480389332306, -9.999544339261095871 ) ) ;
#26171=CARTESIAN_POINT ( 'NONE',  ( 136.1360204305621266, -3.511608612531119000, 53.05693388239312469 ) ) ;
#26172=CARTESIAN_POINT ( 'NONE',  ( 170.2234770963711128, -10.92277846919187034, -10.92277846919209594 ) ) ;
#26174=CARTESIAN_POINT ( 'NONE',  ( -56.48582580120559271, -6.472252184284276844, 6.472252184284108978 ) ) ;
#26175=CARTESIAN_POINT ( 'NONE',  ( -105.4741150117390021, -8.366608964578313490, 19.60045294983322961 ) ) ;
#26179=CARTESIAN_POINT ( 'NONE',  ( -280.0000000000000568, -40.00000000000000000, -20.00000000000015277 ) ) ;
#26180=CARTESIAN_POINT ( 'NONE',  ( 170.2234770963711128, 45.64576402573181468, 10.92277846919223627 ) ) ;
#26181=CIRCLE ( 'NONE', #15519, 14.99999999999999645 ) ;
#26184=CARTESIAN_POINT ( 'NONE',  ( -4.201409602818355182, 42.95750343186458764, -23.41774994521173170 ) ) ;
#26185=CARTESIAN_POINT ( 'NONE',  ( -100.7734535825088500, -22.67402823373193499, 40.00000000000002132 ) ) ;
#26187=CARTESIAN_POINT ( 'NONE',  ( -1.821043593238323544, -23.89737153267490655, -43.61003463695192295 ) ) ;
#26188=CARTESIAN_POINT ( 'NONE',  ( 47.87955150251453063, 35.38323854600922402, 14.65621728643953148 ) ) ;
#26191=CARTESIAN_POINT ( 'NONE',  ( -280.0000000000000000, -20.00000000000006750, 0.000000000000000000 ) ) ;
#26194=CARTESIAN_POINT ( 'NONE',  ( -188.6013476421507278, -47.09841799633881010, 13.84412643132970189 ) ) ;
#26197=CARTESIAN_POINT ( 'NONE',  ( 13.08024833506956064, -18.54957993049078979, 44.78264744452992829 ) ) ;
#26198=CARTESIAN_POINT ( 'NONE',  ( 23.41418334855310945, 23.33148157649319288, -42.84479974151748394 ) ) ;
#26200=CIRCLE ( 'NONE', #20242, 14.99999999999999645 ) ;
#26201=CARTESIAN_POINT ( 'NONE',  ( 130.8888609958233928, -29.49786752803548495, 12.21841679119701851 ) ) ;
#26202=CARTESIAN_POINT ( 'NONE',  ( 57.59792236341147031, 1.908507979671054758E-14, -2.435789363418160658 ) ) ;
#26203=CARTESIAN_POINT ( 'NONE',  ( -86.96347745069644475, 41.18208027870576871, 15.38646221621837107 ) ) ;
#26205=CARTESIAN_POINT ( 'NONE',  ( -189.1288815661392562, 23.62384257861526038, -43.24061771115778186 ) ) ;
#26206=CARTESIAN_POINT ( 'NONE',  ( 184.8905102610680444, 13.49065550809757497, 43.07788698682593065 ) ) ;
#26208=CARTESIAN_POINT ( 'NONE',  ( 170.2234770963711128, 24.55285855007190676, -40.00000000000002132 ) ) ;
#26209=CARTESIAN_POINT ( 'NONE',  ( 4.995406935893288214, 15.24977328854832770, 0.000000000000000000 ) ) ;
#26210=CARTESIAN_POINT ( 'NONE',  ( -192.9588430854690273, -39.99999999999948841, -54.46834944098263520 ) ) ;
#26211=CARTESIAN_POINT ( 'NONE',  ( 199.9999999999999432, 14.14213562373090838, 14.14213562373092437 ) ) ;
#26212=CARTESIAN_POINT ( 'NONE',  ( -105.3755690713226727, -2.472783935621397949E-13, 21.75974354311649961 ) ) ;
#26213=CARTESIAN_POINT ( 'NONE',  ( 130.8568914410475372, 24.07718906447210472, 24.07718906447249907 ) ) ;
#26215=CARTESIAN_POINT ( 'NONE',  ( 0.2972598230769990524, -18.14793986248724522, 38.42060263243662632 ) ) ;
#26216=CARTESIAN_POINT ( 'NONE',  ( -192.9588430854689989, -14.46834944099973086, 0.000000000000000000 ) ) ;
#26220=ORIENTED_EDGE ( 'NONE', *, *, #16965, .F. ) ;
#26221=CARTESIAN_POINT ( 'NONE',  ( 199.9999999999999432, 14.14213562373113398, -14.14213562373094923 ) ) ;
#26222=CARTESIAN_POINT ( 'NONE',  ( 22.76838195347375304, -43.17632592580142870, -17.88421977190818168 ) ) ;
#26224=CARTESIAN_POINT ( 'NONE',  ( 146.6084372240433709, 5.374981219217002781, -40.00000000000002132 ) ) ;
#26226=EDGE_CURVE ( 'NONE', #11892, #17137, #19070, .T. ) ;
#26227=ORIENTED_EDGE ( 'NONE', *, *, #20292, .F. ) ;
#26230=CARTESIAN_POINT ( 'NONE',  ( 192.4448373802101173, 14.14213562370320076, -42.42640687122072762 ) ) ;
#26232=CARTESIAN_POINT ( 'NONE',  ( -174.2682069750611902, -39.26787081113005939, -16.26528465560755876 ) ) ;
#26233=CARTESIAN_POINT ( 'NONE',  ( -213.1075012329537230, -40.00000000000025580, 53.71589010953650956 ) ) ;
#26234=CARTESIAN_POINT ( 'NONE',  ( 163.1118516004056573, -27.26290988616869626, 40.00000000000002132 ) ) ;
#26237=EDGE_CURVE ( 'NONE', #11587, #961, #18153, .T. ) ;
#26238=CARTESIAN_POINT ( 'NONE',  ( -213.1075012329537230, -40.00000000000011369, 13.71589010951897691 ) ) ;
#26239=CARTESIAN_POINT ( 'NONE',  ( 14.38125909742181818, -39.99999999999986500, -15.17850393972675604 ) ) ;
#26240=CARTESIAN_POINT ( 'NONE',  ( -105.3394646353678041, -10.54672847193054075, 18.62482576794085887 ) ) ;
#26241=CARTESIAN_POINT ( 'NONE',  ( -198.0356074513804288, -39.15871834505936278, 39.15871834505892224 ) ) ;
#26242=CARTESIAN_POINT ( 'NONE',  ( -208.1127848780264742, -15.00245453012673202, -40.00000000000002132 ) ) ;
#26243=CARTESIAN_POINT ( 'NONE',  ( 136.1360204305621551, -31.79587985999244282, -24.77266263493140386 ) ) ;
#26244=CARTESIAN_POINT ( 'NONE',  ( -105.4741150117390021, -8.366608964578313490, 19.60045294983322961 ) ) ;
#26246=CARTESIAN_POINT ( 'NONE',  ( 107.5473083967699068, 16.96446921415981635, 16.96446921416008990 ) ) ;
#26247=CARTESIAN_POINT ( 'NONE',  ( -238.4067589809705794, -4.716212492215116094E-14, 0.9644942799825824142 ) ) ;
#26248=CARTESIAN_POINT ( 'NONE',  ( 14.38125909742180220, 39.01709431150916885, -17.55144818341463164 ) ) ;
#26249=CARTESIAN_POINT ( 'NONE',  ( 163.1118516004056573, 19.27778845538753316, 19.27778845538783870 ) ) ;
#26250=CARTESIAN_POINT ( 'NONE',  ( -188.6890294954627620, -13.84869711777154855, -47.12920239600004635 ) ) ;
#26251=CARTESIAN_POINT ( 'NONE',  ( 165.3321726438082351, -2.475684083387132530E-13, 26.53500608755492252 ) ) ;
#26253=CARTESIAN_POINT ( 'NONE',  ( 170.2234770963711128, -17.36149277826940462, -39.20704971665412586 ) ) ;
#26254=CARTESIAN_POINT ( 'NONE',  ( 98.29820294267493352, -20.00000000000511235, 5.223721743777709619E-12 ) ) ;
#26255=CARTESIAN_POINT ( 'NONE',  ( 130.8568914410475372, 34.05028731879791337, 0.000000000000000000 ) ) ;
#26256=CARTESIAN_POINT ( 'NONE',  ( -87.13361725327074225, -15.19799821270821560, -15.19799821270861884 ) ) ;
#26257=CARTESIAN_POINT ( 'NONE',  ( -259.2033419157646676, -35.01439189186523748, -21.55415060305881170 ) ) ;
#26259=CARTESIAN_POINT ( 'NONE',  ( -105.2054292635175585, 21.49321519473984665, 5.610018989487960791E-28 ) ) ;
#26260=EDGE_LOOP ( 'NONE', ( #8924, #6210, #5847, #20684 ) ) ;
#26263=CARTESIAN_POINT ( 'NONE',  ( -5.866564133101632272, 23.09290806363617676, 42.46617576964622742 ) ) ;
#26266=( BOUNDED_SURFACE ( )  B_SPLINE_SURFACE ( 3, 3, ( 
 ( #5828, #11941, #18456, #8211, #2238, #373, #13930, #5960, #234, #24330, #6094, #2369, #3977, #14070, #16197, #14201, #16060, #22335, #8077, #12074, #104, #20195, #1843, #1975, #24458, #20593, #26336, #8346, #16467, #7942 ),
 ( #10216, #12336, #2107, #20330, #18322, #24591, #6347, #10081, #20464, #4110, #12209, #4375, #22066, #20067, #9945, #16329, #14335, #18055, #15919, #14466, #18595, #22467, #10346, #22599, #24051, #12465, #10481, #26206, #17125, #2908 ),
 ( #8883, #25256, #19126, #8750, #6879, #4902, #14596, #20861, #2776, #14863, #908, #11016, #23258, #16727, #16866, #18727, #22725, #9021, #21260, #6484, #12605, #5034, #11141, #777, #2645, #22997, #24728, #4504, #7007, #16994 ),
 ( #24998, #10888, #6612, #20734, #13141, #4774, #12878, #18863, #20994, #8477, #644, #19000, #25129, #6751, #14995, #23130, #511, #13012, #15128, #2503, #14730, #21133, #19256, #3032, #8616, #16595, #10614, #24858, #22862, #4639 ),
 ( #12741, #10752, #23884, #13638, #1287, #17759, #3537, #7140, #21764, #9136, #21511, #1167, #9395, #19635, #5661, #11779, #3283, #11381, #5532, #5279, #23505, #25769, #7388, #21632, #17625, #15383, #9654, #7264, #19502, #5159 ),
 ( #23750, #15255, #13384, #3408, #15499, #19760, #11637, #15756, #9270, #17502, #11261, #23385, #1550, #13767, #25388, #13265, #21894, #3671, #1418, #25642, #23629, #25900, #21387, #9519, #3159, #1036, #7519, #15627, #5408, #19380 ),
 ( #17378, #17252, #13509, #25517, #7641, #11509, #24301, #18161, #6069, #3948, #6193, #8315, #15890, #19897, #14171, #26307, #7775, #8186, #10187, #1947, #4081, #20303, #12182, #18429, #22174, #206, #6319, #9787, #1815, #4217 ) ),
 .UNSPECIFIED., .T., .F., .F. ) 
 B_SPLINE_SURFACE_WITH_KNOTS ( ( 4, 3, 4 ),
 ( 4, 2, 2, 2, 2, 2, 2, 2, 2, 2, 2, 2, 2, 2, 4 ),
 ( 0.000000000000000000, 0.5000000000000000000, 1.000000000000000000 ),
 ( 0.000000000000000000, 0.1357259735107005372, 0.1651108541090157700, 0.1944957347073310028, 0.3598804999793158710, 0.3867117631979620773, 0.4135430264166082281, 0.5789277916885930964, 0.6062785021374117456, 0.6336292125862302838, 0.8508620842112317728, 0.8814014469398914198, 0.9119408096685510667, 0.9559704048342755334, 1.000000000000000000 ),
 .UNSPECIFIED. ) 
 GEOMETRIC_REPRESENTATION_ITEM ( )  RATIONAL_B_SPLINE_SURFACE ( (
 ( 1.000000000000000000, 1.000000000000000000, 1.000000000000000000, 1.000000000000000000, 1.000000000000000000, 1.000000000000000000, 1.000000000000000000, 1.000000000000000000, 1.000000000000000000, 1.000000000000000000, 1.000000000000000000, 1.000000000000000000, 1.000000000000000000, 1.000000000000000000, 1.000000000000000000, 1.000000000000000000, 1.000000000000000000, 1.000000000000000000, 1.000000000000000000, 1.000000000000000000, 1.000000000000000000, 1.000000000000000000, 1.000000000000000000, 1.000000000000000000, 1.000000000000000000, 1.000000000000000000, 1.000000000000000000, 1.000000000000000000, 1.000000000000000000, 1.000000000000000000),
 ( 0.3333333333333333703, 0.3333333333333333703, 0.3333333333333333703, 0.3333333333333333703, 0.3333333333333333703, 0.3333333333333333703, 0.3333333333333333703, 0.3333333333333333703, 0.3333333333333333703, 0.3333333333333333703, 0.3333333333333333703, 0.3333333333333333703, 0.3333333333333333703, 0.3333333333333333703, 0.3333333333333333703, 0.3333333333333333703, 0.3333333333333333703, 0.3333333333333333703, 0.3333333333333333703, 0.3333333333333333703, 0.3333333333333333703, 0.3333333333333333703, 0.3333333333333333703, 0.3333333333333333703, 0.3333333333333333703, 0.3333333333333333703, 0.3333333333333333703, 0.3333333333333333703, 0.3333333333333333703, 0.3333333333333333703),
 ( 0.3333333333333333703, 0.3333333333333333703, 0.3333333333333333703, 0.3333333333333333703, 0.3333333333333333703, 0.3333333333333333703, 0.3333333333333333703, 0.3333333333333333703, 0.3333333333333333703, 0.3333333333333333703, 0.3333333333333333703, 0.3333333333333333703, 0.3333333333333333703, 0.3333333333333333703, 0.3333333333333333703, 0.3333333333333333703, 0.3333333333333333703, 0.3333333333333333703, 0.3333333333333333703, 0.3333333333333333703, 0.3333333333333333703, 0.3333333333333333703, 0.3333333333333333703, 0.3333333333333333703, 0.3333333333333333703, 0.3333333333333333703, 0.3333333333333333703, 0.3333333333333333703, 0.3333333333333333703, 0.3333333333333333703),
 ( 1.000000000000000000, 1.000000000000000000, 1.000000000000000000, 1.000000000000000000, 1.000000000000000000, 1.000000000000000000, 1.000000000000000000, 1.000000000000000000, 1.000000000000000000, 1.000000000000000000, 1.000000000000000000, 1.000000000000000000, 1.000000000000000000, 1.000000000000000000, 1.000000000000000000, 1.000000000000000000, 1.000000000000000000, 1.000000000000000000, 1.000000000000000000, 1.000000000000000000, 1.000000000000000000, 1.000000000000000000, 1.000000000000000000, 1.000000000000000000, 1.000000000000000000, 1.000000000000000000, 1.000000000000000000, 1.000000000000000000, 1.000000000000000000, 1.000000000000000000),
 ( 0.3333333333333333703, 0.3333333333333333703, 0.3333333333333333703, 0.3333333333333333703, 0.3333333333333333703, 0.3333333333333333703, 0.3333333333333333703, 0.3333333333333333703, 0.3333333333333333703, 0.3333333333333333703, 0.3333333333333333703, 0.3333333333333333703, 0.3333333333333333703, 0.3333333333333333703, 0.3333333333333333703, 0.3333333333333333703, 0.3333333333333333703, 0.3333333333333333703, 0.3333333333333333703, 0.3333333333333333703, 0.3333333333333333703, 0.3333333333333333703, 0.3333333333333333703, 0.3333333333333333703, 0.3333333333333333703, 0.3333333333333333703, 0.3333333333333333703, 0.3333333333333333703, 0.3333333333333333703, 0.3333333333333333703),
 ( 0.3333333333333333703, 0.3333333333333333703, 0.3333333333333333703, 0.3333333333333333703, 0.3333333333333333703, 0.3333333333333333703, 0.3333333333333333703, 0.3333333333333333703, 0.3333333333333333703, 0.3333333333333333703, 0.3333333333333333703, 0.3333333333333333703, 0.3333333333333333703, 0.3333333333333333703, 0.3333333333333333703, 0.3333333333333333703, 0.3333333333333333703, 0.3333333333333333703, 0.3333333333333333703, 0.3333333333333333703, 0.3333333333333333703, 0.3333333333333333703, 0.3333333333333333703, 0.3333333333333333703, 0.3333333333333333703, 0.3333333333333333703, 0.3333333333333333703, 0.3333333333333333703, 0.3333333333333333703, 0.3333333333333333703),
 ( 1.000000000000000000, 1.000000000000000000, 1.000000000000000000, 1.000000000000000000, 1.000000000000000000, 1.000000000000000000, 1.000000000000000000, 1.000000000000000000, 1.000000000000000000, 1.000000000000000000, 1.000000000000000000, 1.000000000000000000, 1.000000000000000000, 1.000000000000000000, 1.000000000000000000, 1.000000000000000000, 1.000000000000000000, 1.000000000000000000, 1.000000000000000000, 1.000000000000000000, 1.000000000000000000, 1.000000000000000000, 1.000000000000000000, 1.000000000000000000, 1.000000000000000000, 1.000000000000000000, 1.000000000000000000, 1.000000000000000000, 1.000000000000000000, 1.000000000000000000) ) ) 
 REPRESENTATION_ITEM ( '' )  SURFACE ( )  );
#26267=CARTESIAN_POINT ( 'NONE',  ( 200.0000000000000000, -20.00000000000006750, -40.00000000000002132 ) ) ;
#26269=CARTESIAN_POINT ( 'NONE',  ( -110.0737093975992309, 5.042781230404372650, 19.58505513376282536 ) ) ;
#26272=CARTESIAN_POINT ( 'NONE',  ( -93.01741312765912539, -8.169811846367046826, -20.82169463874099335 ) ) ;
#26273=CARTESIAN_POINT ( 'NONE',  ( -259.2033419157646676, -1.473088368616265084E-13, 9.517827891722632216 ) ) ;
#26274=CARTESIAN_POINT ( 'NONE',  ( -259.2033419157646676, -1.473088368616265084E-13, 9.517827891722632216 ) ) ;
#26278=CARTESIAN_POINT ( 'NONE',  ( -4.027137536850113442, -13.82877337592765699, -46.99492183298336556 ) ) ;
#26279=CARTESIAN_POINT ( 'NONE',  ( 184.8905102610680444, -13.49065550809791603, -13.49065550809818781 ) ) ;
#26281=CARTESIAN_POINT ( 'NONE',  ( 14.38125909742183062, -67.30136555898262429, 10.73282306405838682 ) ) ;
#26282=CARTESIAN_POINT ( 'NONE',  ( 170.2234770963711128, -40.00000000000024158, 24.55285855007145202 ) ) ;
#26283=CARTESIAN_POINT ( 'NONE',  ( 14.38125909742181285, -10.73282306404712472, -10.73282306404731301 ) ) ;
#26284=CARTESIAN_POINT ( 'NONE',  ( -208.1127848780264742, -55.00245453010926866, 40.00000000000002132 ) ) ;
#26286=CARTESIAN_POINT ( 'NONE',  ( 19.06497207195982924, -54.19242893257843008, -2.449293598294708485E-15 ) ) ;
#26287=CARTESIAN_POINT ( 'NONE',  ( -110.0730399734196254, 10.33436089318840523, 17.33982166920115375 ) ) ;
#26288=CARTESIAN_POINT ( 'NONE',  ( -259.2033419157646676, 40.00000000000029843, -30.48217210827696988 ) ) ;
#26289=CARTESIAN_POINT ( 'NONE',  ( -280.0000000000000568, 14.14213562373097943, -42.42640687119285303 ) ) ;
#26290=CARTESIAN_POINT ( 'NONE',  ( 184.8905102610680444, 19.07866798485562398, -40.00000000000002132 ) ) ;
#26292=ORIENTED_EDGE ( 'NONE', *, *, #25415, .T. ) ;
#26293=CARTESIAN_POINT ( 'NONE',  ( -91.56559293963834989, -22.67402823373193499, 40.00000000000002132 ) ) ;
#26294=CARTESIAN_POINT ( 'NONE',  ( 170.0000000000001421, 9.369682556672135121, 22.62041470344889760 ) ) ;
#26295=CARTESIAN_POINT ( 'NONE',  ( -192.9588430854690273, -40.00000000000024158, 54.46834944101708231 ) ) ;
#26296=CARTESIAN_POINT ( 'NONE',  ( -105.3755690713226727, -15.38646221621807619, 15.38646221621768362 ) ) ;
#26297=CARTESIAN_POINT ( 'NONE',  ( 163.1118516004056573, -2.556006622855449647E-13, 27.26290988616872824 ) ) ;
#26298=CARTESIAN_POINT ( 'NONE',  ( -190.6721700386037526, -43.63442057298705379, -23.91541588165668131 ) ) ;
#26302=CARTESIAN_POINT ( 'NONE',  ( -198.0356074513804572, 39.15871834505956173, -39.15871834505865223 ) ) ;
#26303=CARTESIAN_POINT ( 'NONE',  ( -100.7734535825088500, -40.53558337403692491, 16.03295912088671571 ) ) ;
#26304=CARTESIAN_POINT ( 'NONE',  ( -110.1011157335593396, 20.18087853521583241, 1.497753828917178565 ) ) ;
#26305=CARTESIAN_POINT ( 'NONE',  ( -135.8532207217289738, -1.208299557080134822E-13, 9.153146818113572891 ) ) ;
#26306=CARTESIAN_POINT ( 'NONE',  ( 136.1360204305621551, -31.79587985999279454, 24.77266263493094911 ) ) ;
#26307=CARTESIAN_POINT ( 'NONE',  ( 0.2972598230769938343, 10.13633138497486286, -10.13633138497461594 ) ) ;
#26308=CARTESIAN_POINT ( 'NONE',  ( -198.0356074513804572, 10.87444709759730088, -10.87444709759707173 ) ) ;
#26309=CARTESIAN_POINT ( 'NONE',  ( -213.1075012329537230, -66.26714140138676612, 9.698598906462487790 ) ) ;
#26311=AXIS2_PLACEMENT_3D ( 'NONE', #4572, #19187, #9074 ) ;
#26313=CARTESIAN_POINT ( 'NONE',  ( 91.82158438592156813, 39.99999999999995737, 22.79471317813484887 ) ) ;
#26314=CARTESIAN_POINT ( 'NONE',  ( 57.59792236341147031, 1.722363176415040886, 1.722363176415060426 ) ) ;
#26315=CARTESIAN_POINT ( 'NONE',  ( 17.24092899315852279, 44.34059580269009615, -18.36647614519047522 ) ) ;
#26316=CARTESIAN_POINT ( 'NONE',  ( -56.48582580120559982, 30.84685318188643777, -40.00000000000002132 ) ) ;
#26319=CARTESIAN_POINT ( 'NONE',  ( -213.1075012329537230, 13.71589010951907994, 0.000000000000000000 ) ) ;
#26320=CARTESIAN_POINT ( 'NONE',  ( -3.524834090818314891, -43.28235980537091621, 17.92814044289653097 ) ) ;
#26321=CARTESIAN_POINT ( 'NONE',  ( -135.8532207217289738, -9.153146818113595984, 40.00000000000002132 ) ) ;
#26323=CARTESIAN_POINT ( 'NONE',  ( -194.4222775679849917, -44.35790405182654439, 24.44979664542841391 ) ) ;
#26325=CARTESIAN_POINT ( 'NONE',  ( 21.45050411887960706, -18.02367319545413693, 43.51299627226052280 ) ) ;
#26326=ADVANCED_FACE ( 'NONE', ( #13330 ), #25626, .T. ) ;
#26328=CARTESIAN_POINT ( 'NONE',  ( 22.92196489052082953, 23.44087486047551394, -42.99364193793545041 ) ) ;
#26332=CARTESIAN_POINT ( 'NONE',  ( -144.0562696876083066, -14.68019673967120120, 29.54283206236174664 ) ) ;
#26333=CARTESIAN_POINT ( 'NONE',  ( 136.1360204305621266, 3.511608612530757068, -3.511608612530642937 ) ) ;
#26334=CARTESIAN_POINT ( 'NONE',  ( 14.38125909742181285, -15.17850393972633505, 0.000000000000000000 ) ) ;
#26335=CARTESIAN_POINT ( 'NONE',  ( -192.9370379451880240, 14.03127537977120909, -48.35015161801996442 ) ) ;
#26336=CARTESIAN_POINT ( 'NONE',  ( 170.2234770963711128, -17.36149277827010096, 17.36149277826970660 ) ) ;
#26338=CARTESIAN_POINT ( 'NONE',  ( 14.38125909742182884, -55.17850393971007605, 40.00000000000002132 ) ) ;
#26339=CARTESIAN_POINT ( 'NONE',  ( 4.995406935893288214, 55.24977328854835434, 2.449293598294708485E-15 ) ) ;
#26340=CARTESIAN_POINT ( 'NONE',  ( -105.3755690713226727, 1.741486606973311632E-13, -18.24025645688352881 ) ) ;
#26341=CARTESIAN_POINT ( 'NONE',  ( -86.96347745069644475, 41.18208027870598187, -15.38646221621779731 ) ) ;
#26344=FACE_OUTER_BOUND ( 'NONE', #19324, .T. ) ;
#26346=CARTESIAN_POINT ( 'NONE',  ( -280.0000000000000568, -14.14213562373108601, 42.42640687119285303 ) ) ;
#26347=CARTESIAN_POINT ( 'NONE',  ( -103.9663809733797990, -8.026122152273305943, 20.15238534308313589 ) ) ;
#26349=ORIENTED_EDGE ( 'NONE', *, *, #7991, .T. ) ;
#26351=CARTESIAN_POINT ( 'NONE',  ( 163.1118516004056573, -9.006482792073960297, -47.56205970284963769 ) ) ;
#26352=CARTESIAN_POINT ( 'NONE',  ( 83.11963132834678447, -24.42551322420066384, -9.001241435739066432 ) ) ;
#26353=CARTESIAN_POINT ( 'NONE',  ( 163.1118516004056573, -40.00000000000003553, 12.73709011382460687 ) ) ;
#26403=COLOUR_RGB('Off White',0.89,0.88,0.83);
#26404=FILL_AREA_STYLE_COLOUR('',#26403);
#26405=FILL_AREA_STYLE('',(#26404));
#26406=SURFACE_STYLE_FILL_AREA(#26405);
#26407=SURFACE_SIDE_STYLE('',(#26406));
#26408=SURFACE_STYLE_USAGE(.BOTH.,#26407);
#26409=PRESENTATION_STYLE_ASSIGNMENT((#26408));
ENDSEC;
END-ISO-10303-21;
